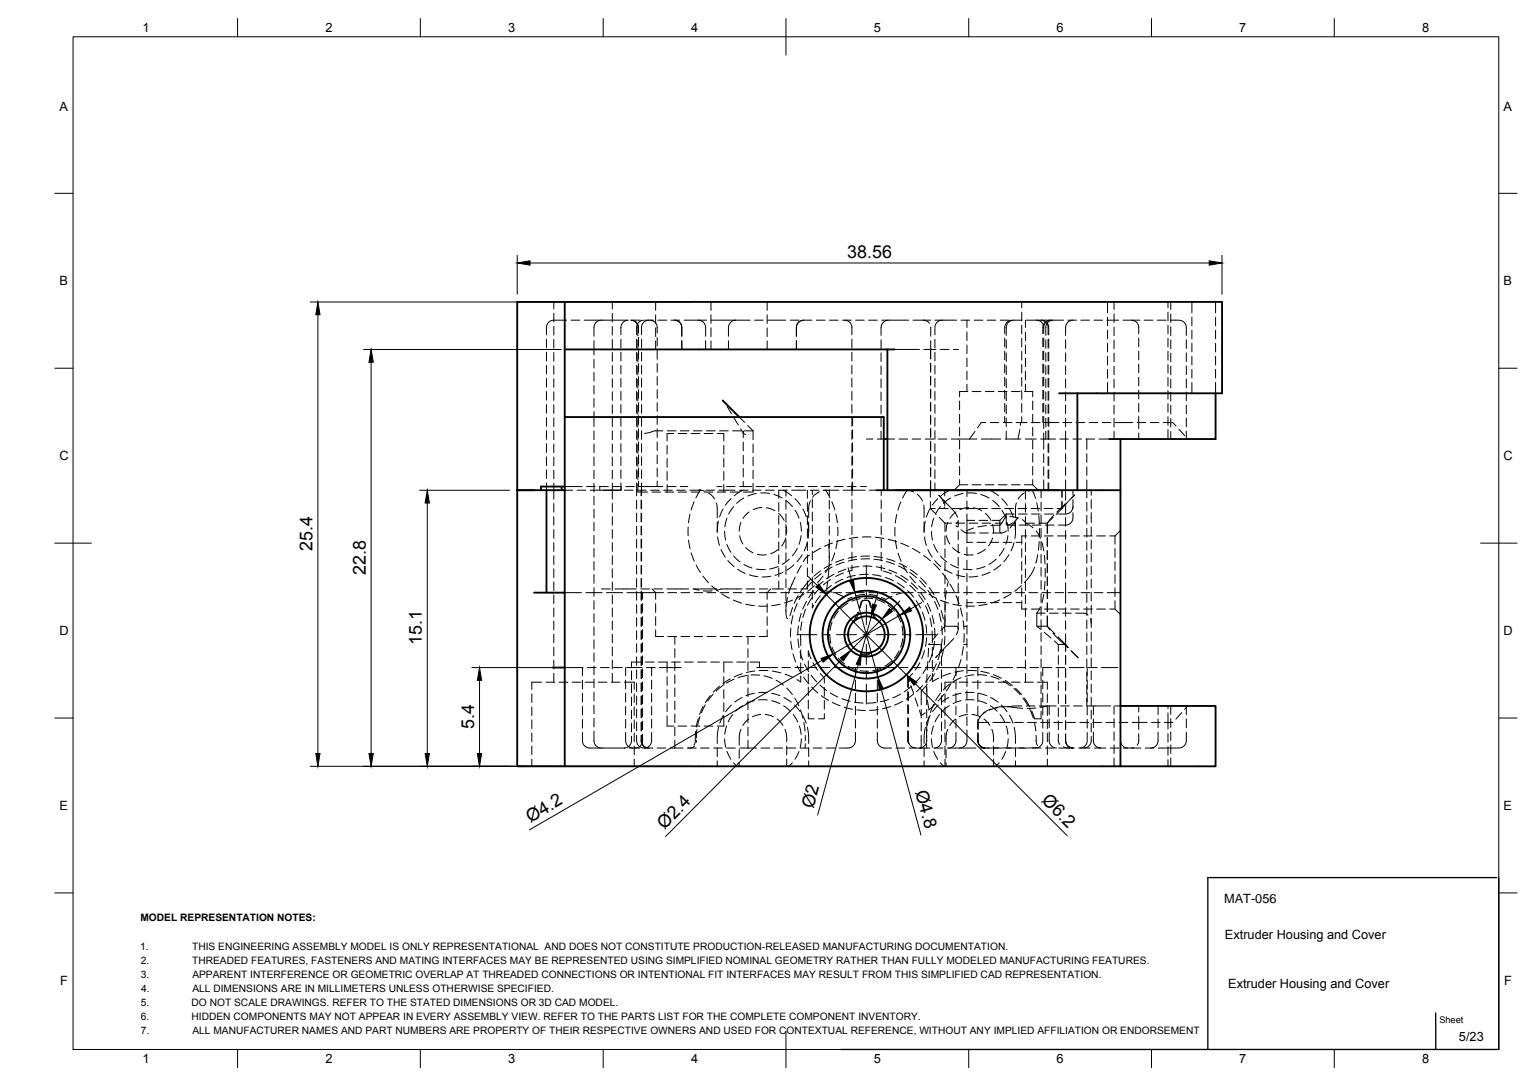
ISO-10303-21;
HEADER;
/* Generated by software containing ST-Developer
 * from STEP Tools, Inc. (www.steptools.com) 
 */

FILE_DESCRIPTION(
/* description */ (''),
/* implementation_level */ '2;1');

FILE_NAME(
/* name */ 'Extruder Housing and Cover.step',
/* time_stamp */ '2026-10-28T16:47:13+01:00',
/* author */ (''),
/* organization */ (''),
/* preprocessor_version */ 'ST-DEVELOPER v20.2',
/* originating_system */ 'Autodesk Translation Framework v15.17.0.0',
/* authorisation */ '');

FILE_SCHEMA (('AUTOMOTIVE_DESIGN { 1 0 10303 214 3 1 1 }'));
ENDSEC;

DATA;
#10=MECHANICAL_DESIGN_GEOMETRIC_PRESENTATION_REPRESENTATION('',(#4569,#4570),#459242);
#135=SPHERICAL_SURFACE('',#96252,3.7);
#136=SPHERICAL_SURFACE('',#96289,0.4);
#137=SPHERICAL_SURFACE('',#96515,3.7);
#138=SPHERICAL_SURFACE('',#96673,2.5);
#139=SPHERICAL_SURFACE('',#96678,2.5);
#140=SPHERICAL_SURFACE('',#96891,0.4);
#141=SPHERICAL_SURFACE('',#96896,0.4);
#156=ELLIPSE('',#96160,1.23559647500717,0.4);
#157=ELLIPSE('',#96173,0.405496303869506,0.4);
#158=ELLIPSE('',#96175,0.680073525436772,0.4);
#159=ELLIPSE('',#96193,0.565685424949236,0.4);
#160=ELLIPSE('',#96250,11.2311262166053,9.2);
#161=ELLIPSE('',#96391,11.2311262166054,9.2);
#162=ELLIPSE('',#96412,0.565685424948761,0.4);
#163=ELLIPSE('',#96519,10.6232449530892,9.2);
#164=ELLIPSE('',#96520,11.2311262166053,9.2);
#165=ELLIPSE('',#96521,11.2311262166053,9.2);
#166=ELLIPSE('',#96562,11.2311262166054,9.2);
#167=ELLIPSE('',#96563,10.6232449530892,9.2);
#168=ELLIPSE('',#96876,12.4909175466738,7.94395207421036);
#169=ELLIPSE('',#97006,2.10877579943506,1.);
#170=ELLIPSE('',#97007,2.46373699895096,1.);
#171=ELLIPSE('',#97009,2.59999999999994,1.3);
#172=ELLIPSE('',#97010,0.230940107675852,0.2);
#173=ELLIPSE('',#97011,0.230940107675852,0.2);
#174=ELLIPSE('',#97015,2.26648083430746,1.3);
#175=ELLIPSE('',#97016,0.24415491775229,0.2);
#176=ELLIPSE('',#97017,0.24415491775229,0.2);
#177=ELLIPSE('',#97027,0.24415491775229,0.2);
#178=ELLIPSE('',#97030,0.24415491775229,0.2);
#179=ELLIPSE('',#97033,0.230940107675851,0.2);
#180=ELLIPSE('',#97035,0.230940107675851,0.2);
#181=ELLIPSE('',#97037,2.59999999999997,1.3);
#182=ELLIPSE('',#97038,2.46373699895092,1.);
#183=ELLIPSE('',#97040,2.10877579943508,1.);
#184=ELLIPSE('',#97042,2.26648083430744,1.3);
#1619=ORIENTED_CLOSED_SHELL('',*,#94627,.F.);
#1620=BREP_WITH_VOIDS('Cover',#94628,(#1619));
#1621=TOROIDAL_SURFACE('',#95348,5.05,0.4);
#1622=TOROIDAL_SURFACE('',#95355,10.4999999997296,0.4);
#1623=TOROIDAL_SURFACE('',#95362,11.6,0.4);
#1624=TOROIDAL_SURFACE('',#95390,3.6,0.4);
#1625=TOROIDAL_SURFACE('',#95404,1.2,0.4);
#1626=TOROIDAL_SURFACE('',#95413,13.6,0.4);
#1627=TOROIDAL_SURFACE('',#95420,3.55,0.4);
#1628=TOROIDAL_SURFACE('',#95445,10.1000000149012,0.4);
#1629=TOROIDAL_SURFACE('',#95463,3.6,0.4);
#1630=TOROIDAL_SURFACE('',#95475,3.55,0.4);
#1631=TOROIDAL_SURFACE('',#95497,10.1000000149012,0.4);
#1632=TOROIDAL_SURFACE('',#95504,4.1,0.4);
#1633=TOROIDAL_SURFACE('',#95508,3.2,0.4);
#1634=TOROIDAL_SURFACE('',#95514,5.80000000000001,0.4);
#1635=TOROIDAL_SURFACE('',#95535,5.2,0.4);
#1636=TOROIDAL_SURFACE('',#95543,5.8,0.4);
#1637=TOROIDAL_SURFACE('',#95547,7.59496173936711,0.4);
#1638=TOROIDAL_SURFACE('',#95556,1.2,0.4);
#1639=TOROIDAL_SURFACE('',#95570,3.5,0.4);
#1640=TOROIDAL_SURFACE('',#95591,9.7949617393671,0.4);
#1641=TOROIDAL_SURFACE('',#95596,3.6,0.4);
#1642=TOROIDAL_SURFACE('',#95603,10.1,0.4);
#1643=TOROIDAL_SURFACE('',#95610,16.9949617393671,0.4);
#1644=TOROIDAL_SURFACE('',#95631,4.,0.4);
#1645=TOROIDAL_SURFACE('',#95639,23.3449617393671,0.4);
#1646=TOROIDAL_SURFACE('',#95643,0.8,0.4);
#1647=TOROIDAL_SURFACE('',#95647,8.2,0.4);
#1648=TOROIDAL_SURFACE('',#95669,19.3949617393671,0.4);
#1649=TOROIDAL_SURFACE('',#95676,10.1,0.4);
#1650=TOROIDAL_SURFACE('',#95699,5.05,0.4);
#1651=TOROIDAL_SURFACE('',#95707,13.,0.4);
#1652=TOROIDAL_SURFACE('',#95716,11.6,0.4);
#1653=TOROIDAL_SURFACE('',#95723,10.4999999997296,0.4);
#1654=TOROIDAL_SURFACE('',#95753,4.,0.4);
#1655=TOROIDAL_SURFACE('',#95760,13.6,0.4);
#1656=TOROIDAL_SURFACE('',#96072,5.05,0.4);
#1657=TOROIDAL_SURFACE('',#96090,11.,0.4);
#1658=TOROIDAL_SURFACE('',#96106,3.6,0.4);
#1659=TOROIDAL_SURFACE('',#96110,2.1,0.4);
#1660=TOROIDAL_SURFACE('',#96116,2.1,0.4);
#1661=TOROIDAL_SURFACE('',#96119,16.9949617393671,0.4);
#1662=TOROIDAL_SURFACE('',#96123,3.6,0.4);
#1663=TOROIDAL_SURFACE('',#96126,9.79496173936711,0.4);
#1664=TOROIDAL_SURFACE('',#96138,11.95,0.4);
#1665=TOROIDAL_SURFACE('',#96145,4.2,0.4);
#1666=TOROIDAL_SURFACE('',#96178,4.2,0.4);
#1667=TOROIDAL_SURFACE('',#96185,25.3449617393673,0.4);
#1668=TOROIDAL_SURFACE('',#96201,4.09750037145961,0.4);
#1669=TOROIDAL_SURFACE('',#96206,3.2,0.4);
#1670=TOROIDAL_SURFACE('',#96209,4.1,0.4);
#1671=TOROIDAL_SURFACE('',#96230,8.8,0.4);
#1672=TOROIDAL_SURFACE('',#96253,4.6,0.4);
#1673=TOROIDAL_SURFACE('',#96263,1.2,0.4);
#1674=TOROIDAL_SURFACE('',#96272,6.1,0.4);
#1675=TOROIDAL_SURFACE('',#96280,5.2,0.4);
#1676=TOROIDAL_SURFACE('',#96286,7.2949617393671,0.4);
#1677=TOROIDAL_SURFACE('',#96310,4.5,0.4);
#1678=TOROIDAL_SURFACE('',#96319,8.2,0.4);
#1679=TOROIDAL_SURFACE('',#96326,19.4949617393671,0.4);
#1680=TOROIDAL_SURFACE('',#96361,4.1,0.4);
#1681=TOROIDAL_SURFACE('',#96365,6.2,0.4);
#1682=TOROIDAL_SURFACE('',#96372,22.1949617393671,0.4);
#1683=TOROIDAL_SURFACE('',#96376,8.8,0.4);
#1684=TOROIDAL_SURFACE('',#96397,12.05,0.4);
#1685=TOROIDAL_SURFACE('',#96404,3.6,0.4);
#1686=TOROIDAL_SURFACE('',#96429,1.2,0.4);
#1687=TOROIDAL_SURFACE('',#96438,8.8,0.4);
#1688=TOROIDAL_SURFACE('',#96450,3.9,0.4);
#1689=TOROIDAL_SURFACE('',#96478,8.8,0.4);
#1690=TOROIDAL_SURFACE('',#96495,3.9,0.4);
#1691=TOROIDAL_SURFACE('',#96506,8.8,0.4);
#1692=TOROIDAL_SURFACE('',#96509,4.0975003714596,0.4);
#1693=TOROIDAL_SURFACE('',#96525,8.8,0.4);
#1694=TOROIDAL_SURFACE('',#96538,3.9,0.4);
#1695=TOROIDAL_SURFACE('',#96884,3.6,0.4);
#1696=TOROIDAL_SURFACE('',#96902,3.6,0.4);
#1697=TOROIDAL_SURFACE('',#96914,4.64877154610377,0.4);
#2221=(
BOUNDED_SURFACE()
B_SPLINE_SURFACE(2,2,((#138725,#138726,#138727,#138728,#138729),(#138730,
#138731,#138732,#138733,#138734),(#138735,#138736,#138737,#138738,#138739)),
 .UNSPECIFIED.,.F.,.F.,.F.)
B_SPLINE_SURFACE_WITH_KNOTS((3,3),(3,2,3),(-1.08356648062379E-15,1.5707963267949),
(-0.78539816339629,0.381098988689,1.54759614077429),.UNSPECIFIED.)
GEOMETRIC_REPRESENTATION_ITEM()
RATIONAL_B_SPLINE_SURFACE(((1.,0.834677941920344,1.,0.834677941920344,1.),
(0.707106781186542,0.590206432838701,0.707106781186542,0.590206432838701,
0.707106781186542),(1.,0.834677941920344,1.,0.834677941920344,1.)))
REPRESENTATION_ITEM('')
SURFACE()
);
#2222=(
BOUNDED_SURFACE()
B_SPLINE_SURFACE(2,2,((#138751,#138752,#138753,#138754,#138755),(#138756,
#138757,#138758,#138759,#138760),(#138761,#138762,#138763,#138764,#138765)),
 .UNSPECIFIED.,.F.,.F.,.F.)
B_SPLINE_SURFACE_WITH_KNOTS((3,3),(3,2,3),(-2.56377862909096E-16,1.5707963267949),
(0.206471222704293,1.13583112104019,2.06519101937609),.UNSPECIFIED.)
GEOMETRIC_REPRESENTATION_ITEM()
RATIONAL_B_SPLINE_SURFACE(((1.,0.89396503791678,1.,0.89396503791678,1.),
(0.707106781186548,0.632128740454645,0.707106781186548,0.632128740454645,
0.707106781186548),(1.,0.89396503791678,1.,0.89396503791678,1.)))
REPRESENTATION_ITEM('')
SURFACE()
);
#2223=(
BOUNDED_SURFACE()
B_SPLINE_SURFACE(2,2,((#138777,#138778,#138779,#138780,#138781),(#138782,
#138783,#138784,#138785,#138786),(#138787,#138788,#138789,#138790,#138791)),
 .UNSPECIFIED.,.F.,.F.,.F.)
B_SPLINE_SURFACE_WITH_KNOTS((3,3),(3,2,3),(-4.13193059734374E-15,1.5707963267949),
(-0.913769759667264,1.11022302462516E-16,0.913769759667264),
 .UNSPECIFIED.)
GEOMETRIC_REPRESENTATION_ITEM()
RATIONAL_B_SPLINE_SURFACE(((1.,0.89743109935827,1.,0.89743109935827,1.),
(0.707106781186553,0.634579616003937,0.707106781186553,0.634579616003937,
0.707106781186553),(1.,0.89743109935827,1.,0.89743109935827,1.)))
REPRESENTATION_ITEM('')
SURFACE()
);
#2224=(
BOUNDED_SURFACE()
B_SPLINE_SURFACE(2,2,((#138803,#138804,#138805),(#138806,#138807,#138808),
(#138809,#138810,#138811)),.UNSPECIFIED.,.F.,.F.,.F.)
B_SPLINE_SURFACE_WITH_KNOTS((3,3),(3,3),(-3.94009957434615E-16,1.5707963267949),
(-2.61567274150278,-1.57079632679301),.UNSPECIFIED.)
GEOMETRIC_REPRESENTATION_ITEM()
RATIONAL_B_SPLINE_SURFACE(((1.,0.866605104543064,1.),(0.707106781186545,
0.612782346033276,0.707106781186545),(1.,0.866605104543064,1.)))
REPRESENTATION_ITEM('')
SURFACE()
);
#2225=(
BOUNDED_SURFACE()
B_SPLINE_SURFACE(2,2,((#138823,#138824,#138825),(#138826,#138827,#138828),
(#138829,#138830,#138831)),.UNSPECIFIED.,.F.,.F.,.F.)
B_SPLINE_SURFACE_WITH_KNOTS((3,3),(3,3),(-1.43399263023479E-17,1.5707963267949),
(-1.57079632679302,-0.785398163396283),.UNSPECIFIED.)
GEOMETRIC_REPRESENTATION_ITEM()
RATIONAL_B_SPLINE_SURFACE(((1.,0.923879532511424,1.),(0.707106781186537,
0.653281482438276,0.707106781186537),(1.,0.923879532511424,1.)))
REPRESENTATION_ITEM('')
SURFACE()
);
#2226=(
BOUNDED_SURFACE()
B_SPLINE_SURFACE(2,2,((#138884,#138885,#138886),(#138887,#138888,#138889),
(#138890,#138891,#138892)),.UNSPECIFIED.,.F.,.F.,.F.)
B_SPLINE_SURFACE_WITH_KNOTS((3,3),(3,3),(-2.92306873924357E-15,1.5707963267949),
(-0.624753868765047,0.624753868765048),.UNSPECIFIED.)
GEOMETRIC_REPRESENTATION_ITEM()
RATIONAL_B_SPLINE_SURFACE(((1.,0.81110710565381,1.),(0.707106781186553,
0.573539334676407,0.707106781186553),(1.,0.81110710565381,1.)))
REPRESENTATION_ITEM('')
SURFACE()
);
#2227=(
BOUNDED_SURFACE()
B_SPLINE_SURFACE(2,2,((#138904,#138905,#138906,#138907,#138908),(#138909,
#138910,#138911,#138912,#138913),(#138914,#138915,#138916,#138917,#138918)),
 .UNSPECIFIED.,.F.,.F.,.F.)
B_SPLINE_SURFACE_WITH_KNOTS((3,3),(3,2,3),(-4.23634106201263E-16,1.5707963267949),
(-0.93774449040515,0.,0.93774449040515),.UNSPECIFIED.)
GEOMETRIC_REPRESENTATION_ITEM()
RATIONAL_B_SPLINE_SURFACE(((1.,0.892078465806108,1.,0.892078465806108,1.),
(0.707106781186543,0.630794732521986,0.707106781186543,0.630794732521986,
0.707106781186543),(1.,0.892078465806108,1.,0.892078465806108,1.)))
REPRESENTATION_ITEM('')
SURFACE()
);
#2228=(
BOUNDED_SURFACE()
B_SPLINE_SURFACE(2,2,((#138930,#138931,#138932),(#138933,#138934,#138935),
(#138936,#138937,#138938)),.UNSPECIFIED.,.F.,.F.,.F.)
B_SPLINE_SURFACE_WITH_KNOTS((3,3),(3,3),(-1.38777878078474E-15,1.5707963267949),
(-1.57079632680232,-0.78539816339745),.UNSPECIFIED.)
GEOMETRIC_REPRESENTATION_ITEM()
RATIONAL_B_SPLINE_SURFACE(((1.,0.923879532509866,1.),(0.707106781186554,
0.653281482437189,0.707106781186554),(1.,0.923879532509866,1.)))
REPRESENTATION_ITEM('')
SURFACE()
);
#2229=(
BOUNDED_SURFACE()
B_SPLINE_SURFACE(2,2,((#138962,#138963,#138964,#138965,#138966),(#138967,
#138968,#138969,#138970,#138971),(#138972,#138973,#138974,#138975,#138976)),
 .UNSPECIFIED.,.F.,.F.,.F.)
B_SPLINE_SURFACE_WITH_KNOTS((3,3),(3,2,3),(-3.22429839320269E-16,1.57079632679491),
(-1.57079632679301,-0.578762685695985,0.413270955399318),.UNSPECIFIED.)
GEOMETRIC_REPRESENTATION_ITEM()
RATIONAL_B_SPLINE_SURFACE(((1.,0.87948523306508,1.,0.87948523306508,1.),
(0.707106781186541,0.621889972253744,0.707106781186541,0.621889972253744,
0.707106781186541),(1.,0.87948523306508,1.,0.87948523306508,1.)))
REPRESENTATION_ITEM('')
SURFACE()
);
#2230=(
BOUNDED_SURFACE()
B_SPLINE_SURFACE(2,2,((#138988,#138989,#138990),(#138991,#138992,#138993),
(#138994,#138995,#138996)),.UNSPECIFIED.,.F.,.F.,.F.)
B_SPLINE_SURFACE_WITH_KNOTS((3,3),(3,3),(-4.80258936466661E-17,1.5707963267949),
(0.338566037798194,1.71521306218255),.UNSPECIFIED.)
GEOMETRIC_REPRESENTATION_ITEM()
RATIONAL_B_SPLINE_SURFACE(((1.,0.772312077486283,1.),(0.707106781186543,
0.546107107182817,0.707106781186543),(1.,0.772312077486283,1.)))
REPRESENTATION_ITEM('')
SURFACE()
);
#2231=(
BOUNDED_SURFACE()
B_SPLINE_SURFACE(2,2,((#139010,#139011,#139012),(#139013,#139014,#139015),
(#139016,#139017,#139018)),.UNSPECIFIED.,.F.,.F.,.F.)
B_SPLINE_SURFACE_WITH_KNOTS((3,3),(3,3),(-2.97223913180379E-15,1.5707963267949),
(0.821121559764502,2.02961305550291),.UNSPECIFIED.)
GEOMETRIC_REPRESENTATION_ITEM()
RATIONAL_B_SPLINE_SURFACE(((1.,0.82293085364046,1.),(0.707106781186547,
0.581899987056804,0.707106781186547),(1.,0.82293085364046,1.)))
REPRESENTATION_ITEM('')
SURFACE()
);
#2232=(
BOUNDED_SURFACE()
B_SPLINE_SURFACE(2,2,((#139080,#139081,#139082),(#139083,#139084,#139085),
(#139086,#139087,#139088)),.UNSPECIFIED.,.F.,.F.,.F.)
B_SPLINE_SURFACE_WITH_KNOTS((3,3),(3,3),(1.36100253158678E-19,1.57079632679491),
(0.135935745545801,1.57038769941725),.UNSPECIFIED.)
GEOMETRIC_REPRESENTATION_ITEM()
RATIONAL_B_SPLINE_SURFACE(((1.,0.753631982435871,1.),(0.707106781186546,
0.532898285299465,0.707106781186546),(1.,0.753631982435871,1.)))
REPRESENTATION_ITEM('')
SURFACE()
);
#2233=(
BOUNDED_SURFACE()
B_SPLINE_SURFACE(2,2,((#139100,#139101,#139102,#139103,#139104),(#139105,
#139106,#139107,#139108,#139109),(#139110,#139111,#139112,#139113,#139114)),
 .UNSPECIFIED.,.F.,.F.,.F.)
B_SPLINE_SURFACE_WITH_KNOTS((3,3),(3,2,3),(-3.39617731412459E-16,1.570796326795),
(1.57038769941725,2.35599017650376,3.14159265359003),.UNSPECIFIED.)
GEOMETRIC_REPRESENTATION_ITEM()
RATIONAL_B_SPLINE_SURFACE(((1.,0.92384043395866,1.,0.92384043395866,1.),
(0.707106781186508,0.653253835586454,0.707106781186508,0.653253835586454,
0.707106781186508),(1.,0.92384043395866,1.,0.92384043395866,1.)))
REPRESENTATION_ITEM('')
SURFACE()
);
#2234=(
BOUNDED_SURFACE()
B_SPLINE_SURFACE(2,2,((#139126,#139127,#139128,#139129,#139130),(#139131,
#139132,#139133,#139134,#139135),(#139136,#139137,#139138,#139139,#139140)),
 .UNSPECIFIED.,.F.,.F.,.F.)
B_SPLINE_SURFACE_WITH_KNOTS((3,3),(3,2,3),(-3.35182484084685E-16,1.5707963267949),
(-3.14159265359013,-2.16753947400706,-1.19348629442367),.UNSPECIFIED.)
GEOMETRIC_REPRESENTATION_ITEM()
RATIONAL_B_SPLINE_SURFACE(((1.,0.883728319944576,1.,0.883728319944576,1.),
(0.707106781186538,0.624890287759396,0.707106781186538,0.624890287759396,
0.707106781186538),(1.,0.883728319944576,1.,0.883728319944576,1.)))
REPRESENTATION_ITEM('')
SURFACE()
);
#2235=(
BOUNDED_SURFACE()
B_SPLINE_SURFACE(2,2,((#139152,#139153,#139154),(#139155,#139156,#139157),
(#139158,#139159,#139160)),.UNSPECIFIED.,.F.,.F.,.F.)
B_SPLINE_SURFACE_WITH_KNOTS((3,3),(3,3),(-2.40560064119055E-16,1.5707963267949),
(-2.36148733561698,-1.11197959808688),.UNSPECIFIED.)
GEOMETRIC_REPRESENTATION_ITEM()
RATIONAL_B_SPLINE_SURFACE(((1.,0.81110710565381,1.),(0.707106781186542,
0.573539334676398,0.707106781186542),(1.,0.81110710565381,1.)))
REPRESENTATION_ITEM('')
SURFACE()
);
#2236=(
BOUNDED_SURFACE()
B_SPLINE_SURFACE(2,2,((#139172,#139173,#139174),(#139175,#139176,#139177),
(#139178,#139179,#139180)),.UNSPECIFIED.,.F.,.F.,.F.)
B_SPLINE_SURFACE_WITH_KNOTS((3,3),(3,3),(-3.67871583187674E-16,1.5707963267949),
(-1.11197959808689,0.13308724141338),.UNSPECIFIED.)
GEOMETRIC_REPRESENTATION_ITEM()
RATIONAL_B_SPLINE_SURFACE(((1.,0.812403840463596,1.),(0.707106781186548,
0.574456264653803,0.707106781186548),(1.,0.812403840463596,1.)))
REPRESENTATION_ITEM('')
SURFACE()
);
#2237=(
BOUNDED_SURFACE()
B_SPLINE_SURFACE(2,2,((#139189,#139190,#139191),(#139192,#139193,#139194),
(#139195,#139196,#139197)),.UNSPECIFIED.,.F.,.F.,.F.)
B_SPLINE_SURFACE_WITH_KNOTS((3,3),(3,3),(-3.62332867476797E-16,1.5707963267949),
(-0.379047751698848,0.883627629924469),.UNSPECIFIED.)
GEOMETRIC_REPRESENTATION_ITEM()
RATIONAL_B_SPLINE_SURFACE(((1.,0.8072386920689,1.),(0.707106781186543,0.570803953198074,
0.707106781186543),(1.,0.8072386920689,1.)))
REPRESENTATION_ITEM('')
SURFACE()
);
#2238=(
BOUNDED_SURFACE()
B_SPLINE_SURFACE(2,2,((#139234,#139235,#139236),(#139237,#139238,#139239),
(#139240,#139241,#139242)),.UNSPECIFIED.,.F.,.F.,.F.)
B_SPLINE_SURFACE_WITH_KNOTS((3,3),(3,3),(-2.78610200478756E-15,1.5707963267949),
(-1.57120495417254,-0.136753000301094),.UNSPECIFIED.)
GEOMETRIC_REPRESENTATION_ITEM()
RATIONAL_B_SPLINE_SURFACE(((1.,0.753631982435872,1.),(0.707106781186546,
0.532898285299465,0.707106781186546),(1.,0.753631982435872,1.)))
REPRESENTATION_ITEM('')
SURFACE()
);
#2239=(
BOUNDED_SURFACE()
B_SPLINE_SURFACE(2,2,((#139254,#139255,#139256),(#139257,#139258,#139259),
(#139260,#139261,#139262)),.UNSPECIFIED.,.F.,.F.,.F.)
B_SPLINE_SURFACE_WITH_KNOTS((3,3),(3,3),(2.55184415889316E-16,1.5707963267949),
(-0.59217173005856,0.724821492103155),.UNSPECIFIED.)
GEOMETRIC_REPRESENTATION_ITEM()
RATIONAL_B_SPLINE_SURFACE(((1.,0.790913091470082,1.),(0.707106781186549,
0.559260010307712,0.707106781186549),(1.,0.790913091470082,1.)))
REPRESENTATION_ITEM('')
SURFACE()
);
#2240=(
BOUNDED_SURFACE()
B_SPLINE_SURFACE(2,2,((#139292,#139293,#139294,#139295,#139296),(#139297,
#139298,#139299,#139300,#139301),(#139302,#139303,#139304,#139305,#139306)),
 .UNSPECIFIED.,.F.,.F.,.F.)
B_SPLINE_SURFACE_WITH_KNOTS((3,3),(3,2,3),(-3.35271616303555E-16,1.57079632679502),
(1.26610367277728,2.20384816318377,3.14159265359003),.UNSPECIFIED.)
GEOMETRIC_REPRESENTATION_ITEM()
RATIONAL_B_SPLINE_SURFACE(((1.,0.892078465805831,1.,0.892078465805831,1.),
(0.707106781186508,0.630794732521759,0.707106781186508,0.630794732521759,
0.707106781186508),(1.,0.892078465805831,1.,0.892078465805831,1.)))
REPRESENTATION_ITEM('')
SURFACE()
);
#2241=(
BOUNDED_SURFACE()
B_SPLINE_SURFACE(2,2,((#139318,#139319,#139320),(#139321,#139322,#139323),
(#139324,#139325,#139326)),.UNSPECIFIED.,.F.,.F.,.F.)
B_SPLINE_SURFACE_WITH_KNOTS((3,3),(3,3),(-3.10863177296109E-15,1.5707963267949),
(-3.14159265359013,-1.57120495417254),.UNSPECIFIED.)
GEOMETRIC_REPRESENTATION_ITEM()
RATIONAL_B_SPLINE_SURFACE(((1.,0.707251238021515,1.),(0.707106781186534,
0.500102146407585,0.707106781186534),(1.,0.707251238021515,1.)))
REPRESENTATION_ITEM('')
SURFACE()
);
#2242=(
BOUNDED_SURFACE()
B_SPLINE_SURFACE(2,2,((#139373,#139374,#139375,#139376,#139377),(#139378,
#139379,#139380,#139381,#139382),(#139383,#139384,#139385,#139386,#139387)),
 .UNSPECIFIED.,.F.,.F.,.F.)
B_SPLINE_SURFACE_WITH_KNOTS((3,3),(3,2,3),(-3.79723113300163E-16,1.5707963267949),
(-2.21649908067713,-1.20577137048503,-0.195043660292926),.UNSPECIFIED.)
GEOMETRIC_REPRESENTATION_ITEM()
RATIONAL_B_SPLINE_SURFACE(((1.,0.874998380695011,1.,0.874998380695011,1.),
(0.707106781186542,0.618717288516686,0.707106781186542,0.618717288516686,
0.707106781186542),(1.,0.874998380695011,1.,0.874998380695011,1.)))
REPRESENTATION_ITEM('')
SURFACE()
);
#2243=(
BOUNDED_SURFACE()
B_SPLINE_SURFACE(2,2,((#139405,#139406,#139407,#139408,#139409),(#139410,
#139411,#139412,#139413,#139414),(#139415,#139416,#139417,#139418,#139419)),
 .UNSPECIFIED.,.F.,.F.,.F.)
B_SPLINE_SURFACE_WITH_KNOTS((3,3),(3,2,3),(-2.33769771306233E-15,1.5707963267949),
(-0.139437550001727,0.715679388398409,1.57079632679678),.UNSPECIFIED.)
GEOMETRIC_REPRESENTATION_ITEM()
RATIONAL_B_SPLINE_SURFACE(((1.,0.909980842363504,1.,0.909980842363504,1.),
(0.707106781186545,0.643453624385078,0.707106781186545,0.643453624385078,
0.707106781186545),(1.,0.909980842363504,1.,0.909980842363504,1.)))
REPRESENTATION_ITEM('')
SURFACE()
);
#2244=(
BOUNDED_SURFACE()
B_SPLINE_SURFACE(2,2,((#139443,#139444,#139445),(#139446,#139447,#139448),
(#139449,#139450,#139451)),.UNSPECIFIED.,.F.,.F.,.F.)
B_SPLINE_SURFACE_WITH_KNOTS((3,3),(3,3),(1.38777878078144E-17,1.5707963267949),
(0.785398163397444,1.5707963267949),.UNSPECIFIED.)
GEOMETRIC_REPRESENTATION_ITEM()
RATIONAL_B_SPLINE_SURFACE(((1.,0.923879532511286,1.),(0.707106781186537,
0.653281482438178,0.707106781186537),(1.,0.923879532511286,1.)))
REPRESENTATION_ITEM('')
SURFACE()
);
#2245=(
BOUNDED_SURFACE()
B_SPLINE_SURFACE(2,2,((#139463,#139464,#139465,#139466,#139467),(#139468,
#139469,#139470,#139471,#139472),(#139473,#139474,#139475,#139476,#139477)),
 .UNSPECIFIED.,.F.,.F.,.F.)
B_SPLINE_SURFACE_WITH_KNOTS((3,3),(3,2,3),(-2.76514922070703E-15,1.5707963267949),
(-1.03943004137575,0.,1.03943004137575),.UNSPECIFIED.)
GEOMETRIC_REPRESENTATION_ITEM()
RATIONAL_B_SPLINE_SURFACE(((1.,0.867960744996435,1.,0.867960744996435,1.),
(0.707106781186546,0.613740928590705,0.707106781186546,0.613740928590705,
0.707106781186546),(1.,0.867960744996435,1.,0.867960744996435,1.)))
REPRESENTATION_ITEM('')
SURFACE()
);
#2246=(
BOUNDED_SURFACE()
B_SPLINE_SURFACE(2,2,((#139489,#139490,#139491,#139492,#139493),(#139494,
#139495,#139496,#139497,#139498),(#139499,#139500,#139501,#139502,#139503)),
 .UNSPECIFIED.,.F.,.F.,.F.)
B_SPLINE_SURFACE_WITH_KNOTS((3,3),(3,2,3),(-4.15746516061636E-16,1.5707963267949),
(-1.31482537730283,-2.22044604925031E-16,1.31482537730283),
 .UNSPECIFIED.)
GEOMETRIC_REPRESENTATION_ITEM()
RATIONAL_B_SPLINE_SURFACE(((1.,0.791575909743,1.,0.791575909743,1.),(0.707106781186554,
0.559728693603191,0.707106781186554,0.559728693603191,0.707106781186554),
(1.,0.791575909743,1.,0.791575909743,1.)))
REPRESENTATION_ITEM('')
SURFACE()
);
#2247=(
BOUNDED_SURFACE()
B_SPLINE_SURFACE(2,2,((#139558,#139559,#139560,#139561,#139562),(#139563,
#139564,#139565,#139566,#139567),(#139568,#139569,#139570,#139571,#139572)),
 .UNSPECIFIED.,.F.,.F.,.F.)
B_SPLINE_SURFACE_WITH_KNOTS((3,3),(3,2,3),(-2.46171489419642E-16,1.5707963267949),
(-2.81803077212777,-1.86696066691245,-0.915890561697128),.UNSPECIFIED.)
GEOMETRIC_REPRESENTATION_ITEM()
RATIONAL_B_SPLINE_SURFACE(((1.,0.889047894212165,1.,0.889047894212165,1.),
(0.707106781186546,0.628651794797041,0.707106781186546,0.628651794797041,
0.707106781186546),(1.,0.889047894212165,1.,0.889047894212165,1.)))
REPRESENTATION_ITEM('')
SURFACE()
);
#2248=(
BOUNDED_SURFACE()
B_SPLINE_SURFACE(2,2,((#139584,#139585,#139586),(#139587,#139588,#139589),
(#139590,#139591,#139592)),.UNSPECIFIED.,.F.,.F.,.F.)
B_SPLINE_SURFACE_WITH_KNOTS((3,3),(3,3),(-4.20649046086306E-17,1.5707963267949),
(-1.66612611099672,-0.292748166464849),.UNSPECIFIED.)
GEOMETRIC_REPRESENTATION_ITEM()
RATIONAL_B_SPLINE_SURFACE(((1.,0.773349375865919,1.),(0.707106781186547,
0.546840587901175,0.707106781186547),(1.,0.773349375865919,1.)))
REPRESENTATION_ITEM('')
SURFACE()
);
#2249=(
BOUNDED_SURFACE()
B_SPLINE_SURFACE(2,2,((#139604,#139605,#139606,#139607,#139608),(#139609,
#139610,#139611,#139612,#139613),(#139614,#139615,#139616,#139617,#139618)),
 .UNSPECIFIED.,.F.,.F.,.F.)
B_SPLINE_SURFACE_WITH_KNOTS((3,3),(3,2,3),(-2.33310191252187E-15,1.5707963267949),
(-0.0602957815162571,0.75525027264115,1.57079632679678),.UNSPECIFIED.)
GEOMETRIC_REPRESENTATION_ITEM()
RATIONAL_B_SPLINE_SURFACE(((1.,0.918006240075228,1.,0.918006240075228,1.),
(0.707106781186546,0.649128437528759,0.707106781186546,0.649128437528759,
0.707106781186546),(1.,0.918006240075228,1.,0.918006240075228,1.)))
REPRESENTATION_ITEM('')
SURFACE()
);
#2250=(
BOUNDED_SURFACE()
B_SPLINE_SURFACE(2,2,((#139630,#139631,#139632),(#139633,#139634,#139635),
(#139636,#139637,#139638)),.UNSPECIFIED.,.F.,.F.,.F.)
B_SPLINE_SURFACE_WITH_KNOTS((3,3),(3,3),(-4.40596164996656E-16,1.5707963267949),
(1.57079632679678,3.04334701619792),.UNSPECIFIED.)
GEOMETRIC_REPRESENTATION_ITEM()
RATIONAL_B_SPLINE_SURFACE(((1.,0.740974920563651,1.),(0.707106781186542,
0.523948391019717,0.707106781186542),(1.,0.740974920563651,1.)))
REPRESENTATION_ITEM('')
SURFACE()
);
#2251=(
BOUNDED_SURFACE()
B_SPLINE_SURFACE(2,2,((#139673,#139674,#139675),(#139676,#139677,#139678),
(#139679,#139680,#139681)),.UNSPECIFIED.,.F.,.F.,.F.)
B_SPLINE_SURFACE_WITH_KNOTS((3,3),(3,3),(-3.19704967403774E-16,1.5707963267949),
(-0.873151522554683,-0.203094574416464),.UNSPECIFIED.)
GEOMETRIC_REPRESENTATION_ITEM()
RATIONAL_B_SPLINE_SURFACE(((1.,0.944400947853729,1.),(0.707106781186549,
0.667792314386376,0.707106781186549),(1.,0.944400947853729,1.)))
REPRESENTATION_ITEM('')
SURFACE()
);
#2252=(
BOUNDED_SURFACE()
B_SPLINE_SURFACE(2,2,((#139705,#139706,#139707),(#139708,#139709,#139710),
(#139711,#139712,#139713)),.UNSPECIFIED.,.F.,.F.,.F.)
B_SPLINE_SURFACE_WITH_KNOTS((3,3),(3,3),(-5.55723799297029E-15,1.5707963267949),
(-1.5533380622009,-0.0271380096021075),.UNSPECIFIED.)
GEOMETRIC_REPRESENTATION_ITEM()
RATIONAL_B_SPLINE_SURFACE(((1.,0.722696856670203,1.),(0.707106781186542,
0.511023848093699,0.707106781186542),(1.,0.722696856670203,1.)))
REPRESENTATION_ITEM('')
SURFACE()
);
#2253=(
BOUNDED_SURFACE()
B_SPLINE_SURFACE(2,2,((#139725,#139726,#139727,#139728,#139729),(#139730,
#139731,#139732,#139733,#139734),(#139735,#139736,#139737,#139738,#139739)),
 .UNSPECIFIED.,.F.,.F.,.F.)
B_SPLINE_SURFACE_WITH_KNOTS((3,3),(3,2,3),(1.04083408558608E-17,1.5707963267949),
(-0.027138009602113,0.771829158596392,1.5707963267949),.UNSPECIFIED.)
GEOMETRIC_REPRESENTATION_ITEM()
RATIONAL_B_SPLINE_SURFACE(((1.,0.921261973001208,1.,0.921261973001208,1.),
(0.707106781186546,0.651430588358451,0.707106781186546,0.651430588358451,
0.707106781186546),(1.,0.921261973001208,1.,0.921261973001208,1.)))
REPRESENTATION_ITEM('')
SURFACE()
);
#2254=(
BOUNDED_SURFACE()
B_SPLINE_SURFACE(2,2,((#139751,#139752,#139753),(#139754,#139755,#139756),
(#139757,#139758,#139759)),.UNSPECIFIED.,.F.,.F.,.F.)
B_SPLINE_SURFACE_WITH_KNOTS((3,3),(3,3),(-3.04212300157278E-16,1.5707963267949),
(1.5707963267949,2.35619449019235),.UNSPECIFIED.)
GEOMETRIC_REPRESENTATION_ITEM()
RATIONAL_B_SPLINE_SURFACE(((1.,0.923879532511286,1.),(0.707106781186548,
0.653281482438189,0.707106781186548),(1.,0.923879532511286,1.)))
REPRESENTATION_ITEM('')
SURFACE()
);
#2255=(
BOUNDED_SURFACE()
B_SPLINE_SURFACE(2,2,((#139771,#139772,#139773),(#139774,#139775,#139776),
(#139777,#139778,#139779)),.UNSPECIFIED.,.F.,.F.,.F.)
B_SPLINE_SURFACE_WITH_KNOTS((3,3),(3,3),(-4.44307714369147E-16,1.5707963267949),
(-0.411322268457341,0.411322268457339),.UNSPECIFIED.)
GEOMETRIC_REPRESENTATION_ITEM()
RATIONAL_B_SPLINE_SURFACE(((1.,0.9165929526849,1.),(0.707106781186543,0.648129092431289,
0.707106781186543),(1.,0.9165929526849,1.)))
REPRESENTATION_ITEM('')
SURFACE()
);
#2256=(
BOUNDED_SURFACE()
B_SPLINE_SURFACE(2,2,((#139791,#139792,#139793),(#139794,#139795,#139796),
(#139797,#139798,#139799)),.UNSPECIFIED.,.F.,.F.,.F.)
B_SPLINE_SURFACE_WITH_KNOTS((3,3),(3,3),(-3.09236869201824E-15,1.57079632679491),
(-0.743192726042517,0.743192726042517),.UNSPECIFIED.)
GEOMETRIC_REPRESENTATION_ITEM()
RATIONAL_B_SPLINE_SURFACE(((1.,0.736311982025157,1.),(0.707106781186541,
0.520651195558891,0.707106781186541),(1.,0.736311982025157,1.)))
REPRESENTATION_ITEM('')
SURFACE()
);
#2257=(
BOUNDED_SURFACE()
B_SPLINE_SURFACE(2,2,((#139811,#139812,#139813,#139814,#139815),(#139816,
#139817,#139818,#139819,#139820),(#139821,#139822,#139823,#139824,#139825)),
 .UNSPECIFIED.,.F.,.F.,.F.)
B_SPLINE_SURFACE_WITH_KNOTS((3,3),(3,2,3),(-3.88201214029742E-16,1.5707963267949),
(-2.21206449869477,-1.24517592036125,-0.278287342027729),.UNSPECIFIED.)
GEOMETRIC_REPRESENTATION_ITEM()
RATIONAL_B_SPLINE_SURFACE(((1.,0.885399163650358,1.,0.885399163650358,1.),
(0.70710678118654,0.626071752674059,0.70710678118654,0.626071752674059,
0.70710678118654),(1.,0.885399163650358,1.,0.885399163650358,1.)))
REPRESENTATION_ITEM('')
SURFACE()
);
#2258=(
BOUNDED_SURFACE()
B_SPLINE_SURFACE(2,2,((#139876,#139877,#139878,#139879,#139880),(#139881,
#139882,#139883,#139884,#139885),(#139886,#139887,#139888,#139889,#139890)),
 .UNSPECIFIED.,.F.,.F.,.F.)
B_SPLINE_SURFACE_WITH_KNOTS((3,3),(3,2,3),(-3.2009740160607E-15,1.5707963267949),
(-2.81763962832209,-1.47992684575006,-0.142214063178028),.UNSPECIFIED.)
GEOMETRIC_REPRESENTATION_ITEM()
RATIONAL_B_SPLINE_SURFACE(((1.,0.784531318155132,1.,0.784531318155132,1.),
(0.707106781186547,0.554747415120714,0.707106781186547,0.554747415120714,
0.707106781186547),(1.,0.784531318155132,1.,0.784531318155132,1.)))
REPRESENTATION_ITEM('')
SURFACE()
);
#2259=(
BOUNDED_SURFACE()
B_SPLINE_SURFACE(2,2,((#139908,#139909,#139910),(#139911,#139912,#139913),
(#139914,#139915,#139916)),.UNSPECIFIED.,.F.,.F.,.F.)
B_SPLINE_SURFACE_WITH_KNOTS((3,3),(3,3),(-9.43679832250494E-16,1.5707963267949),
(-4.54149544011533E-19,1.07849707504375),.UNSPECIFIED.)
GEOMETRIC_REPRESENTATION_ITEM()
RATIONAL_B_SPLINE_SURFACE(((1.,0.858094793061586,1.),(0.707106781186537,
0.606764647074706,0.707106781186537),(1.,0.858094793061586,1.)))
REPRESENTATION_ITEM('')
SURFACE()
);
#2260=(
BOUNDED_SURFACE()
B_SPLINE_SURFACE(2,2,((#139928,#139929,#139930,#139931,#139932),(#139933,
#139934,#139935,#139936,#139937),(#139938,#139939,#139940,#139941,#139942)),
 .UNSPECIFIED.,.F.,.F.,.F.)
B_SPLINE_SURFACE_WITH_KNOTS((3,3),(3,2,3),(-1.37198715633005E-15,1.5707963267949),
(-0.913769759667265,0.,0.913769759667266),.UNSPECIFIED.)
GEOMETRIC_REPRESENTATION_ITEM()
RATIONAL_B_SPLINE_SURFACE(((1.,0.89743109935827,1.,0.89743109935827,1.),
(0.707106781186543,0.634579616003927,0.707106781186543,0.634579616003927,
0.707106781186543),(1.,0.89743109935827,1.,0.89743109935827,1.)))
REPRESENTATION_ITEM('')
SURFACE()
);
#2261=(
BOUNDED_SURFACE()
B_SPLINE_SURFACE(2,2,((#139954,#139955,#139956,#139957,#139958),(#139959,
#139960,#139961,#139962,#139963),(#139964,#139965,#139966,#139967,#139968)),
 .UNSPECIFIED.,.F.,.F.,.F.)
B_SPLINE_SURFACE_WITH_KNOTS((3,3),(3,2,3),(-5.97388390143348E-15,1.5707963267949),
(-0.929359898335899,0.,0.929359898335898),.UNSPECIFIED.)
GEOMETRIC_REPRESENTATION_ITEM()
RATIONAL_B_SPLINE_SURFACE(((1.,0.89396503791678,1.,0.89396503791678,1.),
(0.707106781186544,0.632128740454641,0.707106781186544,0.632128740454641,
0.707106781186544),(1.,0.89396503791678,1.,0.89396503791678,1.)))
REPRESENTATION_ITEM('')
SURFACE()
);
#2262=(
BOUNDED_SURFACE()
B_SPLINE_SURFACE(2,2,((#140011,#140012,#140013),(#140014,#140015,#140016),
(#140017,#140018,#140019)),.UNSPECIFIED.,.F.,.F.,.F.)
B_SPLINE_SURFACE_WITH_KNOTS((3,3),(3,3),(-2.44248335016468E-15,1.5707963267949),
(-1.38777878078145E-17,1.5707963267949),.UNSPECIFIED.)
GEOMETRIC_REPRESENTATION_ITEM()
RATIONAL_B_SPLINE_SURFACE(((1.,0.707106781186547,1.),(0.707106781186554,
0.500000000000004,0.707106781186554),(1.,0.707106781186547,1.)))
REPRESENTATION_ITEM('')
SURFACE()
);
#2263=(
BOUNDED_SURFACE()
B_SPLINE_SURFACE(2,2,((#140031,#140032,#140033,#140034,#140035),(#140036,
#140037,#140038,#140039,#140040),(#140041,#140042,#140043,#140044,#140045)),
 .UNSPECIFIED.,.F.,.F.,.F.)
B_SPLINE_SURFACE_WITH_KNOTS((3,3),(3,2,3),(-2.87162691077515E-16,1.5707963267949),
(-1.06707356455707,0.,1.06707356455707),.UNSPECIFIED.)
GEOMETRIC_REPRESENTATION_ITEM()
RATIONAL_B_SPLINE_SURFACE(((1.,0.86101371653255,1.,0.86101371653255,1.),
(0.707106781186543,0.608828637654794,0.707106781186543,0.608828637654794,
0.707106781186543),(1.,0.86101371653255,1.,0.86101371653255,1.)))
REPRESENTATION_ITEM('')
SURFACE()
);
#2264=(
BOUNDED_SURFACE()
B_SPLINE_SURFACE(2,2,((#140057,#140058,#140059,#140060,#140061),(#140062,
#140063,#140064,#140065,#140066),(#140067,#140068,#140069,#140070,#140071)),
 .UNSPECIFIED.,.F.,.F.,.F.)
B_SPLINE_SURFACE_WITH_KNOTS((3,3),(3,2,3),(-3.12052122059803E-16,1.5707963267949),
(-0.937275919666155,0.,0.937275919666154),.UNSPECIFIED.)
GEOMETRIC_REPRESENTATION_ITEM()
RATIONAL_B_SPLINE_SURFACE(((1.,0.892184310318489,1.,0.892184310318489,1.),
(0.707106781186544,0.630869575894443,0.707106781186544,0.630869575894443,
0.707106781186544),(1.,0.892184310318489,1.,0.892184310318489,1.)))
REPRESENTATION_ITEM('')
SURFACE()
);
#2265=(
BOUNDED_SURFACE()
B_SPLINE_SURFACE(2,2,((#140083,#140084,#140085,#140086,#140087),(#140088,
#140089,#140090,#140091,#140092),(#140093,#140094,#140095,#140096,#140097)),
 .UNSPECIFIED.,.F.,.F.,.F.)
B_SPLINE_SURFACE_WITH_KNOTS((3,3),(3,2,3),(-2.44248335016467E-15,1.5707963267949),
(-1.94884750401252,-0.974423752006261,1.12987552192351E-32),
 .UNSPECIFIED.)
GEOMETRIC_REPRESENTATION_ITEM()
RATIONAL_B_SPLINE_SURFACE(((1.,0.883641590777673,1.,0.883641590777673,1.),
(0.707106781186542,0.624828960977356,0.707106781186542,0.624828960977356,
0.707106781186542),(1.,0.883641590777673,1.,0.883641590777673,1.)))
REPRESENTATION_ITEM('')
SURFACE()
);
#2266=(
BOUNDED_SURFACE()
B_SPLINE_SURFACE(2,2,((#141085,#141086,#141087,#141088,#141089),(#141090,
#141091,#141092,#141093,#141094),(#141095,#141096,#141097,#141098,#141099)),
 .UNSPECIFIED.,.F.,.F.,.F.)
B_SPLINE_SURFACE_WITH_KNOTS((3,3),(3,2,3),(-4.40321821990384E-16,1.5707963267949),
(-1.1664971520853,0.,1.16649715208529),.UNSPECIFIED.)
GEOMETRIC_REPRESENTATION_ITEM()
RATIONAL_B_SPLINE_SURFACE(((1.,0.834677941920342,1.,0.834677941920342,1.),
(0.707106781186555,0.590206432838712,0.707106781186555,0.590206432838712,
0.707106781186555),(1.,0.834677941920342,1.,0.834677941920342,1.)))
REPRESENTATION_ITEM('')
SURFACE()
);
#2267=(
BOUNDED_SURFACE()
B_SPLINE_SURFACE(2,2,((#141108,#141109,#141110),(#141111,#141112,#141113),
(#141114,#141115,#141116)),.UNSPECIFIED.,.F.,.F.,.F.)
B_SPLINE_SURFACE_WITH_KNOTS((3,3),(3,3),(-3.04212300157654E-16,1.5707963267949),
(-2.35619449019351,-1.57079632679678),.UNSPECIFIED.)
GEOMETRIC_REPRESENTATION_ITEM()
RATIONAL_B_SPLINE_SURFACE(((1.,0.923879532511424,1.),(0.707106781186556,
0.653281482438293,0.707106781186556),(1.,0.923879532511424,1.)))
REPRESENTATION_ITEM('')
SURFACE()
);
#2268=(
BOUNDED_SURFACE()
B_SPLINE_SURFACE(2,2,((#141128,#141129,#141130,#141131,#141132),(#141133,
#141134,#141135,#141136,#141137),(#141138,#141139,#141140,#141141,#141142)),
 .UNSPECIFIED.,.F.,.F.,.F.)
B_SPLINE_SURFACE_WITH_KNOTS((3,3),(3,2,3),(1.38777878069775E-17,1.5707963267949),
(-1.57079632679678,-0.570510447746883,0.429775431304741),.UNSPECIFIED.)
GEOMETRIC_REPRESENTATION_ITEM()
RATIONAL_B_SPLINE_SURFACE(((1.,0.877514024066407,1.,0.877514024066407,1.),
(0.70710678118655,0.620496117003654,0.70710678118655,0.620496117003654,
0.70710678118655),(1.,0.877514024066407,1.,0.877514024066407,1.)))
REPRESENTATION_ITEM('')
SURFACE()
);
#2269=(
BOUNDED_SURFACE()
B_SPLINE_SURFACE(2,2,((#141154,#141155,#141156,#141157,#141158),(#141159,
#141160,#141161,#141162,#141163),(#141164,#141165,#141166,#141167,#141168)),
 .UNSPECIFIED.,.F.,.F.,.F.)
B_SPLINE_SURFACE_WITH_KNOTS((3,3),(3,2,3),(-2.04068455613418E-16,1.5707963267949),
(0.317238733765724,1.23836023442364,2.15948173508156),.UNSPECIFIED.)
GEOMETRIC_REPRESENTATION_ITEM()
RATIONAL_B_SPLINE_SURFACE(((1.,0.895803412613763,1.,0.895803412613763,1.),
(0.707106781186556,0.63342866766925,0.707106781186556,0.63342866766925,
0.707106781186556),(1.,0.895803412613763,1.,0.895803412613763,1.)))
REPRESENTATION_ITEM('')
SURFACE()
);
#2270=(
BOUNDED_SURFACE()
B_SPLINE_SURFACE(2,2,((#141344,#141345,#141346,#141347,#141348),(#141349,
#141350,#141351,#141352,#141353),(#141354,#141355,#141356,#141357,#141358)),
 .UNSPECIFIED.,.F.,.F.,.F.)
B_SPLINE_SURFACE_WITH_KNOTS((3,3),(3,2,3),(-2.00928091613498E-16,1.5707963267949),
(0.492169594955417,1.33946582626418,2.18676205757294),.UNSPECIFIED.)
GEOMETRIC_REPRESENTATION_ITEM()
RATIONAL_B_SPLINE_SURFACE(((1.,0.911595310291363,1.,0.911595310291363,1.),
(0.707106781186556,0.644595225604885,0.707106781186556,0.644595225604885,
0.707106781186556),(1.,0.911595310291363,1.,0.911595310291363,1.)))
REPRESENTATION_ITEM('')
SURFACE()
);
#2271=(
BOUNDED_SURFACE()
B_SPLINE_SURFACE(2,2,((#141547,#141548,#141549),(#141550,#141551,#141552),
(#141553,#141554,#141555)),.UNSPECIFIED.,.F.,.F.,.F.)
B_SPLINE_SURFACE_WITH_KNOTS((3,3),(3,3),(-3.40404913931651E-16,1.5707963267949),
(1.57079632679491,3.14159265358979),.UNSPECIFIED.)
GEOMETRIC_REPRESENTATION_ITEM()
RATIONAL_B_SPLINE_SURFACE(((1.,0.707106781186554,1.),(0.707106781186545,
0.500000000000003,0.707106781186545),(1.,0.707106781186554,1.)))
REPRESENTATION_ITEM('')
SURFACE()
);
#2272=(
BOUNDED_SURFACE()
B_SPLINE_SURFACE(2,2,((#141662,#141663,#141664,#141665,#141666),(#141667,
#141668,#141669,#141670,#141671),(#141672,#141673,#141674,#141675,#141676)),
 .UNSPECIFIED.,.F.,.F.,.F.)
B_SPLINE_SURFACE_WITH_KNOTS((3,3),(3,2,3),(9.65265731632566E-18,1.5707963267949),
(-1.57306506263583,-0.715832961083556,0.141399140468717),.UNSPECIFIED.)
GEOMETRIC_REPRESENTATION_ITEM()
RATIONAL_B_SPLINE_SURFACE(((1.,0.909541807036257,1.,0.909541807036257,1.),
(0.707106781186556,0.643143179528011,0.707106781186556,0.643143179528011,
0.707106781186556),(1.,0.909541807036257,1.,0.909541807036257,1.)))
REPRESENTATION_ITEM('')
SURFACE()
);
#2273=(
BOUNDED_SURFACE()
B_SPLINE_SURFACE(2,2,((#141688,#141689,#141690),(#141691,#141692,#141693),
(#141694,#141695,#141696)),.UNSPECIFIED.,.F.,.F.,.F.)
B_SPLINE_SURFACE_WITH_KNOTS((3,3),(3,3),(-1.07735048008271E-14,1.57079632679491),
(0.133494798627492,1.57079632679493),.UNSPECIFIED.)
GEOMETRIC_REPRESENTATION_ITEM()
RATIONAL_B_SPLINE_SURFACE(((1.,0.752694710045445,1.),(0.707106781186546,
0.532235533636375,0.707106781186546),(1.,0.752694710045445,1.)))
REPRESENTATION_ITEM('')
SURFACE()
);
#2274=(
BOUNDED_SURFACE()
B_SPLINE_SURFACE(2,2,((#141811,#141812,#141813),(#141814,#141815,#141816),
(#141817,#141818,#141819)),.UNSPECIFIED.,.F.,.F.,.F.)
B_SPLINE_SURFACE_WITH_KNOTS((3,3),(3,3),(-7.12649760132934E-17,1.20783157419784),
(0.404259769435194,1.75111622640166),.UNSPECIFIED.)
GEOMETRIC_REPRESENTATION_ITEM()
RATIONAL_B_SPLINE_SURFACE(((1.,0.781688182176695,1.),(0.823118273259482,
0.643421826740624,0.823118273259482),(1.,0.781688182176695,1.)))
REPRESENTATION_ITEM('')
SURFACE()
);
#2275=(
BOUNDED_SURFACE()
B_SPLINE_SURFACE(2,2,((#141851,#141852,#141853),(#141854,#141855,#141856),
(#141857,#141858,#141859)),.UNSPECIFIED.,.F.,.F.,.F.)
B_SPLINE_SURFACE_WITH_KNOTS((3,3),(3,3),(-3.40404913931651E-16,1.5707963267949),
(1.5707963267949,3.14159265358979),.UNSPECIFIED.)
GEOMETRIC_REPRESENTATION_ITEM()
RATIONAL_B_SPLINE_SURFACE(((1.,0.707106781186548,1.),(0.707106781186553,
0.500000000000004,0.707106781186553),(1.,0.707106781186548,1.)))
REPRESENTATION_ITEM('')
SURFACE()
);
#2276=(
BOUNDED_SURFACE()
B_SPLINE_SURFACE(2,2,((#141867,#141868,#141869),(#141870,#141871,#141872),
(#141873,#141874,#141875)),.UNSPECIFIED.,.F.,.F.,.F.)
B_SPLINE_SURFACE_WITH_KNOTS((3,3),(3,3),(-3.38850230422209E-16,1.5707963267949),
(-3.14159265358979,-1.5707963267949),.UNSPECIFIED.)
GEOMETRIC_REPRESENTATION_ITEM()
RATIONAL_B_SPLINE_SURFACE(((1.,0.707106781186548,1.),(0.707106781186553,
0.500000000000004,0.707106781186553),(1.,0.707106781186548,1.)))
REPRESENTATION_ITEM('')
SURFACE()
);
#2277=(
BOUNDED_SURFACE()
B_SPLINE_SURFACE(2,2,((#141883,#141884,#141885),(#141886,#141887,#141888),
(#141889,#141890,#141891)),.UNSPECIFIED.,.F.,.F.,.F.)
B_SPLINE_SURFACE_WITH_KNOTS((3,3),(3,3),(1.04083408558608E-17,1.5707963267949),
(-1.5707963267949,-1.21122148599942),.UNSPECIFIED.)
GEOMETRIC_REPRESENTATION_ITEM()
RATIONAL_B_SPLINE_SURFACE(((1.,0.983881728593355,1.),(0.707106781186553,
0.69570944217391,0.707106781186553),(1.,0.983881728593355,1.)))
REPRESENTATION_ITEM('')
SURFACE()
);
#2278=(
BOUNDED_SURFACE()
B_SPLINE_SURFACE(2,2,((#142040,#142041,#142042,#142043,#142044),(#142045,
#142046,#142047,#142048,#142049),(#142050,#142051,#142052,#142053,#142054)),
 .UNSPECIFIED.,.F.,.F.,.F.)
B_SPLINE_SURFACE_WITH_KNOTS((3,3),(3,2,3),(-3.26817438467699E-16,1.5707963267949),
(-0.0112409050907196,1.17247679255081,2.35619449019235),.UNSPECIFIED.)
GEOMETRIC_REPRESENTATION_ITEM()
RATIONAL_B_SPLINE_SURFACE(((1.,0.829905053082259,1.,0.829905053082259,1.),
(0.70710678118655,0.586831490775449,0.70710678118655,0.586831490775449,
0.70710678118655),(1.,0.829905053082259,1.,0.829905053082259,1.)))
REPRESENTATION_ITEM('')
SURFACE()
);
#2279=(
BOUNDED_SURFACE()
B_SPLINE_SURFACE(2,2,((#142078,#142079,#142080,#142081,#142082),(#142083,
#142084,#142085,#142086,#142087),(#142088,#142089,#142090,#142091,#142092)),
 .UNSPECIFIED.,.F.,.F.,.F.)
B_SPLINE_SURFACE_WITH_KNOTS((3,3),(3,2,3),(-4.37390637964367E-16,1.5707963267949),
(-0.858171546837339,1.11022302462516E-16,0.85817154683734),
 .UNSPECIFIED.)
GEOMETRIC_REPRESENTATION_ITEM()
RATIONAL_B_SPLINE_SURFACE(((1.,0.909346484128941,1.,0.909346484128941,1.),
(0.70710678118655,0.643005065375722,0.70710678118655,0.643005065375722,
0.70710678118655),(1.,0.909346484128941,1.,0.909346484128941,1.)))
REPRESENTATION_ITEM('')
SURFACE()
);
#2280=(
BOUNDED_SURFACE()
B_SPLINE_SURFACE(2,2,((#142107,#142108,#142109,#142110,#142111),(#142112,
#142113,#142114,#142115,#142116),(#142117,#142118,#142119,#142120,#142121)),
 .UNSPECIFIED.,.F.,.F.,.F.)
B_SPLINE_SURFACE_WITH_KNOTS((3,3),(3,2,3),(-3.23084773091812E-16,1.5707963267949),
(-2.9253611858372,-1.9555154025201,-0.98566961920299),.UNSPECIFIED.)
GEOMETRIC_REPRESENTATION_ITEM()
RATIONAL_B_SPLINE_SURFACE(((1.,0.884710895031854,1.,0.884710895031854,1.),
(0.707106781186556,0.625585073266651,0.707106781186556,0.625585073266651,
0.707106781186556),(1.,0.884710895031854,1.,0.884710895031854,1.)))
REPRESENTATION_ITEM('')
SURFACE()
);
#2281=(
BOUNDED_SURFACE()
B_SPLINE_SURFACE(2,2,((#142179,#142180,#142181),(#142182,#142183,#142184),
(#142185,#142186,#142187)),.UNSPECIFIED.,.F.,.F.,.F.)
B_SPLINE_SURFACE_WITH_KNOTS((3,3),(3,3),(-3.40404913931651E-16,1.5707963267949),
(1.5707963267949,3.14159265358979),.UNSPECIFIED.)
GEOMETRIC_REPRESENTATION_ITEM()
RATIONAL_B_SPLINE_SURFACE(((1.,0.707106781186548,1.),(0.70710678118655,
0.500000000000002,0.70710678118655),(1.,0.707106781186548,1.)))
REPRESENTATION_ITEM('')
SURFACE()
);
#2282=(
BOUNDED_SURFACE()
B_SPLINE_SURFACE(2,2,((#142205,#142206,#142207,#142208,#142209),(#142210,
#142211,#142212,#142213,#142214),(#142215,#142216,#142217,#142218,#142219)),
 .UNSPECIFIED.,.F.,.F.,.F.)
B_SPLINE_SURFACE_WITH_KNOTS((3,3),(3,2,3),(-3.38916221447103E-16,1.5707963267949),
(-0.993480418549077,0.,0.993480418549077),.UNSPECIFIED.)
GEOMETRIC_REPRESENTATION_ITEM()
RATIONAL_B_SPLINE_SURFACE(((1.,0.879140723351448,1.,0.879140723351448,1.),
(0.707106781186546,0.621646367099054,0.707106781186546,0.621646367099054,
0.707106781186546),(1.,0.879140723351448,1.,0.879140723351448,1.)))
REPRESENTATION_ITEM('')
SURFACE()
);
#2283=(
BOUNDED_SURFACE()
B_SPLINE_SURFACE(2,2,((#142237,#142238,#142239,#142240,#142241),(#142242,
#142243,#142244,#142245,#142246),(#142247,#142248,#142249,#142250,#142251)),
 .UNSPECIFIED.,.F.,.F.,.F.)
B_SPLINE_SURFACE_WITH_KNOTS((3,3),(3,2,3),(-1.80387197830009E-16,1.5707963267949),
(-2.1740397470008,-1.03404943345041,0.105940880099987),.UNSPECIFIED.)
GEOMETRIC_REPRESENTATION_ITEM()
RATIONAL_B_SPLINE_SURFACE(((1.,0.841903588711717,1.,0.841903588711717,1.),
(0.707106781186553,0.59531573668335,0.707106781186553,0.59531573668335,
0.707106781186553),(1.,0.841903588711717,1.,0.841903588711717,1.)))
REPRESENTATION_ITEM('')
SURFACE()
);
#2284=(
BOUNDED_SURFACE()
B_SPLINE_SURFACE(2,2,((#142263,#142264,#142265),(#142266,#142267,#142268),
(#142269,#142270,#142271)),.UNSPECIFIED.,.F.,.F.,.F.)
B_SPLINE_SURFACE_WITH_KNOTS((3,3),(3,3),(3.04212300157275E-16,1.5707963267949),
(-0.0419015857269754,0.785398163397452),.UNSPECIFIED.)
GEOMETRIC_REPRESENTATION_ITEM()
RATIONAL_B_SPLINE_SURFACE(((1.,0.915659843255931,1.),(0.707106781186539,
0.647469284426472,0.707106781186539),(1.,0.915659843255931,1.)))
REPRESENTATION_ITEM('')
SURFACE()
);
#2285=(
BOUNDED_SURFACE()
B_SPLINE_SURFACE(2,2,((#142283,#142284,#142285),(#142286,#142287,#142288),
(#142289,#142290,#142291)),.UNSPECIFIED.,.F.,.F.,.F.)
B_SPLINE_SURFACE_WITH_KNOTS((3,3),(3,3),(-1.43399263032023E-17,1.5707963267949),
(0.78539816339745,1.5707963267949),.UNSPECIFIED.)
GEOMETRIC_REPRESENTATION_ITEM()
RATIONAL_B_SPLINE_SURFACE(((1.,0.923879532511287,1.),(0.707106781186552,
0.653281482438192,0.707106781186552),(1.,0.923879532511287,1.)))
REPRESENTATION_ITEM('')
SURFACE()
);
#2286=(
BOUNDED_SURFACE()
B_SPLINE_SURFACE(2,2,((#142330,#142331,#142332),(#142333,#142334,#142335),
(#142336,#142337,#142338)),.UNSPECIFIED.,.F.,.F.,.F.)
B_SPLINE_SURFACE_WITH_KNOTS((3,3),(3,3),(1.04083408558608E-17,1.5707963267949),
(-1.5707963267949,2.95409308984431E-16),.UNSPECIFIED.)
GEOMETRIC_REPRESENTATION_ITEM()
RATIONAL_B_SPLINE_SURFACE(((1.,0.707106781186547,1.),(0.707106781186553,
0.500000000000004,0.707106781186553),(1.,0.707106781186547,1.)))
REPRESENTATION_ITEM('')
SURFACE()
);
#2287=(
BOUNDED_SURFACE()
B_SPLINE_SURFACE(2,2,((#142350,#142351,#142352),(#142353,#142354,#142355),
(#142356,#142357,#142358)),.UNSPECIFIED.,.F.,.F.,.F.)
B_SPLINE_SURFACE_WITH_KNOTS((3,3),(3,3),(-1.0408340855861E-17,1.5707963267949),
(-2.76167977375508E-15,1.5707963267949),.UNSPECIFIED.)
GEOMETRIC_REPRESENTATION_ITEM()
RATIONAL_B_SPLINE_SURFACE(((1.,0.707106781186546,1.),(0.707106781186553,
0.500000000000003,0.707106781186553),(1.,0.707106781186546,1.)))
REPRESENTATION_ITEM('')
SURFACE()
);
#2288=(
BOUNDED_SURFACE()
B_SPLINE_SURFACE(2,2,((#142382,#142383,#142384,#142385,#142386),(#142387,
#142388,#142389,#142390,#142391),(#142392,#142393,#142394,#142395,#142396)),
 .UNSPECIFIED.,.F.,.F.,.F.)
B_SPLINE_SURFACE_WITH_KNOTS((3,3),(3,2,3),(-3.33132048898093E-16,1.5707963267949),
(-1.09723005759692,0.,1.09723005759692),.UNSPECIFIED.)
GEOMETRIC_REPRESENTATION_ITEM()
RATIONAL_B_SPLINE_SURFACE(((1.,0.85324761095477,1.,0.85324761095477,1.),
(0.707106781186558,0.603337171737348,0.707106781186558,0.603337171737348,
0.707106781186558),(1.,0.85324761095477,1.,0.85324761095477,1.)))
REPRESENTATION_ITEM('')
SURFACE()
);
#2289=(
BOUNDED_SURFACE()
B_SPLINE_SURFACE(2,2,((#142414,#142415,#142416),(#142417,#142418,#142419),
(#142420,#142421,#142422)),.UNSPECIFIED.,.F.,.F.,.F.)
B_SPLINE_SURFACE_WITH_KNOTS((3,3),(3,3),(-1.07755746139668E-16,1.5707963267949),
(-1.93037116759037,-1.5707963267949),.UNSPECIFIED.)
GEOMETRIC_REPRESENTATION_ITEM()
RATIONAL_B_SPLINE_SURFACE(((1.,0.983881728593356,1.),(0.707106781186554,
0.695709442173911,0.707106781186554),(1.,0.983881728593356,1.)))
REPRESENTATION_ITEM('')
SURFACE()
);
#2290=(
BOUNDED_SURFACE()
B_SPLINE_SURFACE(2,2,((#142555,#142556,#142557,#142558,#142559),(#142560,
#142561,#142562,#142563,#142564),(#142565,#142566,#142567,#142568,#142569)),
 .UNSPECIFIED.,.F.,.F.,.F.)
B_SPLINE_SURFACE_WITH_KNOTS((3,3),(3,2,3),(-3.36658337620736E-16,1.5707963267949),
(-0.939955765746386,-1.11022302462516E-16,0.939955765746385),
 .UNSPECIFIED.)
GEOMETRIC_REPRESENTATION_ITEM()
RATIONAL_B_SPLINE_SURFACE(((1.,0.891578304520668,1.,0.891578304520668,1.),
(0.707106781186548,0.63044106508537,0.707106781186548,0.63044106508537,
0.707106781186548),(1.,0.891578304520668,1.,0.891578304520668,1.)))
REPRESENTATION_ITEM('')
SURFACE()
);
#2291=(
BOUNDED_SURFACE()
B_SPLINE_SURFACE(2,2,((#142581,#142582,#142583,#142584,#142585),(#142586,
#142587,#142588,#142589,#142590),(#142591,#142592,#142593,#142594,#142595)),
 .UNSPECIFIED.,.F.,.F.,.F.)
B_SPLINE_SURFACE_WITH_KNOTS((3,3),(3,2,3),(-1.55728298388104E-16,1.5707963267949),
(-1.94810635916574,-0.974053179581248,1.68810521070105E-12),
 .UNSPECIFIED.)
GEOMETRIC_REPRESENTATION_ITEM()
RATIONAL_B_SPLINE_SURFACE(((1.,0.883728319944464,1.,0.883728319944464,1.),
(0.707106781186545,0.624890287759324,0.707106781186545,0.624890287759324,
0.707106781186545),(1.,0.883728319944464,1.,0.883728319944464,1.)))
REPRESENTATION_ITEM('')
SURFACE()
);
#2292=(
BOUNDED_SURFACE()
B_SPLINE_SURFACE(2,2,((#142747,#142748,#142749,#142750,#142751),(#142752,
#142753,#142754,#142755,#142756),(#142757,#142758,#142759,#142760,#142761)),
 .UNSPECIFIED.,.F.,.F.,.F.)
B_SPLINE_SURFACE_WITH_KNOTS((3,3),(3,2,3),(-2.28159225117958E-16,1.5707963267949),
(-2.35619449019236,-1.53123643686414,-0.706278383535922),.UNSPECIFIED.)
GEOMETRIC_REPRESENTATION_ITEM()
RATIONAL_B_SPLINE_SURFACE(((1.,0.916129842560975,1.,0.916129842560975,1.),
(0.707106781186559,0.64780162412224,0.707106781186559,0.64780162412224,
0.707106781186559),(1.,0.916129842560975,1.,0.916129842560975,1.)))
REPRESENTATION_ITEM('')
SURFACE()
);
#2293=(
BOUNDED_SURFACE()
B_SPLINE_SURFACE(2,2,((#142773,#142774,#142775,#142776,#142777),(#142778,
#142779,#142780,#142781,#142782),(#142783,#142784,#142785,#142786,#142787)),
 .UNSPECIFIED.,.F.,.F.,.F.)
B_SPLINE_SURFACE_WITH_KNOTS((3,3),(3,2,3),(1.54818837825044E-16,1.5707963267949),
(-0.663590463352779,0.191803543921911,1.0471975511966),.UNSPECIFIED.)
GEOMETRIC_REPRESENTATION_ITEM()
RATIONAL_B_SPLINE_SURFACE(((1.,0.909923390286242,1.,0.909923390286242,1.),
(0.70710678118655,0.643412999631658,0.70710678118655,0.643412999631658,
0.70710678118655),(1.,0.909923390286242,1.,0.909923390286242,1.)))
REPRESENTATION_ITEM('')
SURFACE()
);
#2294=(
BOUNDED_SURFACE()
B_SPLINE_SURFACE(2,2,((#142799,#142800,#142801),(#142802,#142803,#142804),
(#142805,#142806,#142807)),.UNSPECIFIED.,.F.,.F.,.F.)
B_SPLINE_SURFACE_WITH_KNOTS((3,3),(3,3),(-2.38131079176154E-16,1.5707963267949),
(1.0471975511966,2.32096244656348),.UNSPECIFIED.)
GEOMETRIC_REPRESENTATION_ITEM()
RATIONAL_B_SPLINE_SURFACE(((1.,0.803953645065829,1.),(0.707106781186556,
0.568481074185697,0.707106781186556),(1.,0.803953645065829,1.)))
REPRESENTATION_ITEM('')
SURFACE()
);
#2295=(
BOUNDED_SURFACE()
B_SPLINE_SURFACE(2,2,((#142821,#142822,#142823),(#142824,#142825,#142826),
(#142827,#142828,#142829)),.UNSPECIFIED.,.F.,.F.,.F.)
B_SPLINE_SURFACE_WITH_KNOTS((3,3),(3,3),(-1.75550993291529E-16,1.5707963267949),
(0.820630207026316,2.0943951023932),.UNSPECIFIED.)
GEOMETRIC_REPRESENTATION_ITEM()
RATIONAL_B_SPLINE_SURFACE(((1.,0.803953645065829,1.),(0.707106781186554,
0.568481074185696,0.707106781186554),(1.,0.803953645065829,1.)))
REPRESENTATION_ITEM('')
SURFACE()
);
#2296=(
BOUNDED_SURFACE()
B_SPLINE_SURFACE(2,2,((#142841,#142842,#142843,#142844,#142845),(#142846,
#142847,#142848,#142849,#142850),(#142851,#142852,#142853,#142854,#142855)),
 .UNSPECIFIED.,.F.,.F.,.F.)
B_SPLINE_SURFACE_WITH_KNOTS((3,3),(3,2,3),(-4.26771686360733E-16,1.5707963267949),
(-1.30899693899481,0.,1.30899693899481),.UNSPECIFIED.)
GEOMETRIC_REPRESENTATION_ITEM()
RATIONAL_B_SPLINE_SURFACE(((1.,0.793353340291521,1.,0.793353340291521,1.),
(0.707106781186554,0.560985526797139,0.707106781186554,0.560985526797139,
0.707106781186554),(1.,0.793353340291521,1.,0.793353340291521,1.)))
REPRESENTATION_ITEM('')
SURFACE()
);
#2297=(
BOUNDED_SURFACE()
B_SPLINE_SURFACE(2,2,((#142926,#142927,#142928),(#142929,#142930,#142931),
(#142932,#142933,#142934)),.UNSPECIFIED.,.F.,.F.,.F.)
B_SPLINE_SURFACE_WITH_KNOTS((3,3),(3,3),(-1.04083408558608E-17,1.5707963267949),
(1.24587053304372,1.5707963267949),.UNSPECIFIED.)
GEOMETRIC_REPRESENTATION_ITEM()
RATIONAL_B_SPLINE_SURFACE(((1.,0.986831905268789,1.),(0.707106781186553,
0.697795532106808,0.707106781186553),(1.,0.986831905268789,1.)))
REPRESENTATION_ITEM('')
SURFACE()
);
#2298=(
BOUNDED_SURFACE()
B_SPLINE_SURFACE(2,2,((#142946,#142947,#142948),(#142949,#142950,#142951),
(#142952,#142953,#142954)),.UNSPECIFIED.,.F.,.F.,.F.)
B_SPLINE_SURFACE_WITH_KNOTS((3,3),(3,3),(-3.40404913931651E-16,1.5707963267949),
(1.5707963267949,3.14159265358979),.UNSPECIFIED.)
GEOMETRIC_REPRESENTATION_ITEM()
RATIONAL_B_SPLINE_SURFACE(((1.,0.707106781186548,1.),(0.707106781186553,
0.500000000000004,0.707106781186553),(1.,0.707106781186548,1.)))
REPRESENTATION_ITEM('')
SURFACE()
);
#2299=(
BOUNDED_SURFACE()
B_SPLINE_SURFACE(2,2,((#142966,#142967,#142968),(#142969,#142970,#142971),
(#142972,#142973,#142974)),.UNSPECIFIED.,.F.,.F.,.F.)
B_SPLINE_SURFACE_WITH_KNOTS((3,3),(3,3),(-3.33074211398212E-16,1.5707963267949),
(-3.14159265358979,-1.86782775822291),.UNSPECIFIED.)
GEOMETRIC_REPRESENTATION_ITEM()
RATIONAL_B_SPLINE_SURFACE(((1.,0.80395364506583,1.),(0.707106781186555,
0.568481074185697,0.707106781186555),(1.,0.80395364506583,1.)))
REPRESENTATION_ITEM('')
SURFACE()
);
#2300=(
BOUNDED_SURFACE()
B_SPLINE_SURFACE(2,2,((#142983,#142984,#142985),(#142986,#142987,#142988),
(#142989,#142990,#142991)),.UNSPECIFIED.,.F.,.F.,.F.)
B_SPLINE_SURFACE_WITH_KNOTS((3,3),(3,3),(-3.32755772175793E-16,1.5707963267949),
(-0.636882447683443,0.636882447683442),.UNSPECIFIED.)
GEOMETRIC_REPRESENTATION_ITEM()
RATIONAL_B_SPLINE_SURFACE(((1.,0.803953645065828,1.),(0.707106781186554,
0.568481074185695,0.707106781186554),(1.,0.803953645065828,1.)))
REPRESENTATION_ITEM('')
SURFACE()
);
#2301=(
BOUNDED_SURFACE()
B_SPLINE_SURFACE(2,2,((#143003,#143004,#143005,#143006,#143007),(#143008,
#143009,#143010,#143011,#143012),(#143013,#143014,#143015,#143016,#143017)),
 .UNSPECIFIED.,.F.,.F.,.F.)
B_SPLINE_SURFACE_WITH_KNOTS((3,3),(3,2,3),(-1.64312426003188E-16,1.5707963267949),
(-2.0943951023932,-1.23900109511851,-0.383607087843824),.UNSPECIFIED.)
GEOMETRIC_REPRESENTATION_ITEM()
RATIONAL_B_SPLINE_SURFACE(((1.,0.909923390286242,1.,0.909923390286242,1.),
(0.707106781186545,0.643412999631653,0.707106781186545,0.643412999631653,
0.707106781186545),(1.,0.909923390286242,1.,0.909923390286242,1.)))
REPRESENTATION_ITEM('')
SURFACE()
);
#2302=(
BOUNDED_SURFACE()
B_SPLINE_SURFACE(2,2,((#143187,#143188,#143189,#143190,#143191),(#143192,
#143193,#143194,#143195,#143196),(#143197,#143198,#143199,#143200,#143201)),
 .UNSPECIFIED.,.F.,.F.,.F.)
B_SPLINE_SURFACE_WITH_KNOTS((3,3),(3,2,3),(-3.04971088561005E-16,1.5707963267949),
(-2.75798556574597,-1.90259155847128,-1.0471975511966),.UNSPECIFIED.)
GEOMETRIC_REPRESENTATION_ITEM()
RATIONAL_B_SPLINE_SURFACE(((1.,0.909923390286243,1.,0.909923390286243,1.),
(0.707106781186553,0.643412999631661,0.707106781186553,0.643412999631661,
0.707106781186553),(1.,0.909923390286243,1.,0.909923390286243,1.)))
REPRESENTATION_ITEM('')
SURFACE()
);
#2303=(
BOUNDED_SURFACE()
B_SPLINE_SURFACE(2,2,((#143213,#143214,#143215),(#143216,#143217,#143218),
(#143219,#143220,#143221)),.UNSPECIFIED.,.F.,.F.,.F.)
B_SPLINE_SURFACE_WITH_KNOTS((3,3),(3,3),(1.72872884261539E-16,1.5707963267949),
(-1.0471975511966,0.226567344170284),.UNSPECIFIED.)
GEOMETRIC_REPRESENTATION_ITEM()
RATIONAL_B_SPLINE_SURFACE(((1.,0.803953645065828,1.),(0.707106781186554,
0.568481074185695,0.707106781186554),(1.,0.803953645065828,1.)))
REPRESENTATION_ITEM('')
SURFACE()
);
#2304=(
BOUNDED_SURFACE()
B_SPLINE_SURFACE(2,2,((#143230,#143231,#143232),(#143233,#143234,#143235),
(#143236,#143237,#143238)),.UNSPECIFIED.,.F.,.F.,.F.)
B_SPLINE_SURFACE_WITH_KNOTS((3,3),(3,3),(1.0220704756512E-16,1.5707963267949),
(-1.27376489536688,1.38777878078145E-17),.UNSPECIFIED.)
GEOMETRIC_REPRESENTATION_ITEM()
RATIONAL_B_SPLINE_SURFACE(((1.,0.80395364506583,1.),(0.707106781186553,
0.568481074185696,0.707106781186553),(1.,0.80395364506583,1.)))
REPRESENTATION_ITEM('')
SURFACE()
);
#2305=(
BOUNDED_SURFACE()
B_SPLINE_SURFACE(2,2,((#143250,#143251,#143252),(#143253,#143254,#143255),
(#143256,#143257,#143258)),.UNSPECIFIED.,.F.,.F.,.F.)
B_SPLINE_SURFACE_WITH_KNOTS((3,3),(3,3),(-1.04083408558608E-17,1.5707963267949),
(-6.80011602582909E-16,1.5707963267949),.UNSPECIFIED.)
GEOMETRIC_REPRESENTATION_ITEM()
RATIONAL_B_SPLINE_SURFACE(((1.,0.707106781186547,1.),(0.707106781186555,
0.500000000000005,0.707106781186555),(1.,0.707106781186547,1.)))
REPRESENTATION_ITEM('')
SURFACE()
);
#2306=(
BOUNDED_SURFACE()
B_SPLINE_SURFACE(2,2,((#143270,#143271,#143272),(#143273,#143274,#143275),
(#143276,#143277,#143278)),.UNSPECIFIED.,.F.,.F.,.F.)
B_SPLINE_SURFACE_WITH_KNOTS((3,3),(3,3),(-1.16510060523539E-16,1.5707963267949),
(1.5707963267949,1.89572212054608),.UNSPECIFIED.)
GEOMETRIC_REPRESENTATION_ITEM()
RATIONAL_B_SPLINE_SURFACE(((1.,0.986831905268789,1.),(0.707106781186554,
0.697795532106808,0.707106781186554),(1.,0.986831905268789,1.)))
REPRESENTATION_ITEM('')
SURFACE()
);
#4089=(
BOUNDED_CURVE()
B_SPLINE_CURVE(2,(#140599,#140600,#140601),.UNSPECIFIED.,.F.,.F.)
B_SPLINE_CURVE_WITH_KNOTS((3,3),(0.,0.128077890591623),.UNSPECIFIED.)
CURVE()
GEOMETRIC_REPRESENTATION_ITEM()
RATIONAL_B_SPLINE_CURVE((1.,1.00129982111734,1.))
REPRESENTATION_ITEM('')
);
#4090=(
BOUNDED_CURVE()
B_SPLINE_CURVE(2,(#140616,#140617,#140618),.UNSPECIFIED.,.F.,.F.)
B_SPLINE_CURVE_WITH_KNOTS((3,3),(0.000362946931860339,0.146205519527569),
 .UNSPECIFIED.)
CURVE()
GEOMETRIC_REPRESENTATION_ITEM()
RATIONAL_B_SPLINE_CURVE((1.00000258096586,1.0005198467923,1.00000237765636))
REPRESENTATION_ITEM('')
);
#4091=(
BOUNDED_CURVE()
B_SPLINE_CURVE(2,(#141526,#141527,#141528),.UNSPECIFIED.,.F.,.F.)
B_SPLINE_CURVE_WITH_KNOTS((3,3),(0.00319674958924355,0.00384559926899821),
 .UNSPECIFIED.)
CURVE()
GEOMETRIC_REPRESENTATION_ITEM()
RATIONAL_B_SPLINE_CURVE((1.00001174504467,1.00001239664656,1.00001282889535))
REPRESENTATION_ITEM('')
);
#4092=(
BOUNDED_CURVE()
B_SPLINE_CURVE(2,(#141532,#141533,#141534),.UNSPECIFIED.,.F.,.F.)
B_SPLINE_CURVE_WITH_KNOTS((3,3),(0.235117374689744,0.605037926847431),
 .UNSPECIFIED.)
CURVE()
GEOMETRIC_REPRESENTATION_ITEM()
RATIONAL_B_SPLINE_CURVE((1.05233383959897,1.08689092491703,1.10064057896449))
REPRESENTATION_ITEM('')
);
#4093=(
BOUNDED_CURVE()
B_SPLINE_CURVE(2,(#141570,#141571,#141572),.UNSPECIFIED.,.F.,.F.)
B_SPLINE_CURVE_WITH_KNOTS((3,3),(1.57192299052648,2.14887151832575),
 .UNSPECIFIED.)
CURVE()
GEOMETRIC_REPRESENTATION_ITEM()
RATIONAL_B_SPLINE_CURVE((6.65976698144355,7.49223785412377,8.17335038631666))
REPRESENTATION_ITEM('')
);
#4094=(
BOUNDED_CURVE()
B_SPLINE_CURVE(2,(#141613,#141614,#141615),.UNSPECIFIED.,.F.,.F.)
B_SPLINE_CURVE_WITH_KNOTS((3,3),(0.270860367343992,0.325892472320335),
 .UNSPECIFIED.)
CURVE()
GEOMETRIC_REPRESENTATION_ITEM()
RATIONAL_B_SPLINE_CURVE((1.54730126785002,1.59219194080314,1.63273127384522))
REPRESENTATION_ITEM('')
);
#4095=(
BOUNDED_CURVE()
B_SPLINE_CURVE(2,(#141631,#141632,#141633),.UNSPECIFIED.,.F.,.F.)
B_SPLINE_CURVE_WITH_KNOTS((3,3),(0.,0.29854563440631),.UNSPECIFIED.)
CURVE()
GEOMETRIC_REPRESENTATION_ITEM()
RATIONAL_B_SPLINE_CURVE((1.,1.04264499839507,1.))
REPRESENTATION_ITEM('')
);
#4096=(
BOUNDED_CURVE()
B_SPLINE_CURVE(2,(#141725,#141726,#141727,#141728),.UNSPECIFIED.,.F.,.F.)
B_SPLINE_CURVE_WITH_KNOTS((3,1,3),(1.66167847180388,2.26230069355391,2.27651444205068),
 .UNSPECIFIED.)
CURVE()
GEOMETRIC_REPRESENTATION_ITEM()
RATIONAL_B_SPLINE_CURVE((6.5568621272732,7.34757944538262,7.99897023989561,
8.01394260001255))
REPRESENTATION_ITEM('')
);
#4097=(
BOUNDED_CURVE()
B_SPLINE_CURVE(2,(#143650,#143651,#143652),.UNSPECIFIED.,.F.,.F.)
B_SPLINE_CURVE_WITH_KNOTS((3,3),(0.,0.28311686851659),.UNSPECIFIED.)
CURVE()
GEOMETRIC_REPRESENTATION_ITEM()
RATIONAL_B_SPLINE_CURVE((1.,1.06870093790198,1.))
REPRESENTATION_ITEM('')
);
#4098=(
BOUNDED_CURVE()
B_SPLINE_CURVE(2,(#143653,#143654,#143655),.UNSPECIFIED.,.F.,.F.)
B_SPLINE_CURVE_WITH_KNOTS((3,3),(0.,0.283116868518929),.UNSPECIFIED.)
CURVE()
GEOMETRIC_REPRESENTATION_ITEM()
RATIONAL_B_SPLINE_CURVE((1.,1.0687009379036,1.))
REPRESENTATION_ITEM('')
);
#4099=(
BOUNDED_CURVE()
B_SPLINE_CURVE(2,(#143729,#143730,#143731),.UNSPECIFIED.,.F.,.F.)
B_SPLINE_CURVE_WITH_KNOTS((3,3),(0.185737456128969,0.362789547470562),
 .UNSPECIFIED.)
CURVE()
GEOMETRIC_REPRESENTATION_ITEM()
RATIONAL_B_SPLINE_CURVE((1.,1.13683142662591,1.01279688953851))
REPRESENTATION_ITEM('')
);
#4100=(
BOUNDED_CURVE()
B_SPLINE_CURVE(2,(#143745,#143746,#143747),.UNSPECIFIED.,.F.,.F.)
B_SPLINE_CURVE_WITH_KNOTS((3,3),(0.00868536478737642,0.185737456128969),
 .UNSPECIFIED.)
CURVE()
GEOMETRIC_REPRESENTATION_ITEM()
RATIONAL_B_SPLINE_CURVE((1.01279688953851,1.13683142662591,1.))
REPRESENTATION_ITEM('')
);
#4101=(
BOUNDED_CURVE()
B_SPLINE_CURVE(2,(#143752,#143753,#143754),.UNSPECIFIED.,.F.,.F.)
B_SPLINE_CURVE_WITH_KNOTS((3,3),(0.,0.0101246152898397),.UNSPECIFIED.)
CURVE()
GEOMETRIC_REPRESENTATION_ITEM()
RATIONAL_B_SPLINE_CURVE((1.,1.01194504282515,1.023099278064))
REPRESENTATION_ITEM('')
);
#4102=(
BOUNDED_CURVE()
B_SPLINE_CURVE(2,(#143755,#143756,#143757),.UNSPECIFIED.,.F.,.F.)
B_SPLINE_CURVE_WITH_KNOTS((3,3),(0.29573730439733,0.30586191968717),
 .UNSPECIFIED.)
CURVE()
GEOMETRIC_REPRESENTATION_ITEM()
RATIONAL_B_SPLINE_CURVE((1.02309927806399,1.01194504282515,1.))
REPRESENTATION_ITEM('')
);
#4103=(
BOUNDED_CURVE()
B_SPLINE_CURVE(2,(#143761,#143762,#143763),.UNSPECIFIED.,.F.,.F.)
B_SPLINE_CURVE_WITH_KNOTS((3,3),(0.185737456128969,0.362789547470561),
 .UNSPECIFIED.)
CURVE()
GEOMETRIC_REPRESENTATION_ITEM()
RATIONAL_B_SPLINE_CURVE((1.,1.13683142662589,1.01279688953851))
REPRESENTATION_ITEM('')
);
#4104=(
BOUNDED_CURVE()
B_SPLINE_CURVE(2,(#143777,#143778,#143779),.UNSPECIFIED.,.F.,.F.)
B_SPLINE_CURVE_WITH_KNOTS((3,3),(0.00868536478737701,0.18573745612897),
 .UNSPECIFIED.)
CURVE()
GEOMETRIC_REPRESENTATION_ITEM()
RATIONAL_B_SPLINE_CURVE((1.01279688953851,1.13683142662591,1.))
REPRESENTATION_ITEM('')
);
#4105=(
BOUNDED_CURVE()
B_SPLINE_CURVE(2,(#143784,#143785,#143786),.UNSPECIFIED.,.F.,.F.)
B_SPLINE_CURVE_WITH_KNOTS((3,3),(0.,0.0101246152898398),.UNSPECIFIED.)
CURVE()
GEOMETRIC_REPRESENTATION_ITEM()
RATIONAL_B_SPLINE_CURVE((1.,1.01194504282515,1.023099278064))
REPRESENTATION_ITEM('')
);
#4106=(
BOUNDED_CURVE()
B_SPLINE_CURVE(2,(#143787,#143788,#143789),.UNSPECIFIED.,.F.,.F.)
B_SPLINE_CURVE_WITH_KNOTS((3,3),(0.29573730439733,0.30586191968717),
 .UNSPECIFIED.)
CURVE()
GEOMETRIC_REPRESENTATION_ITEM()
RATIONAL_B_SPLINE_CURVE((1.023099278064,1.01194504282515,1.))
REPRESENTATION_ITEM('')
);
#4107=(
BOUNDED_CURVE()
B_SPLINE_CURVE(2,(#143926,#143927,#143928),.UNSPECIFIED.,.F.,.F.)
B_SPLINE_CURVE_WITH_KNOTS((3,3),(0.281942572226475,0.665668068688164),
 .UNSPECIFIED.)
CURVE()
GEOMETRIC_REPRESENTATION_ITEM()
RATIONAL_B_SPLINE_CURVE((1.10320422134355,1.12183288632099,1.))
REPRESENTATION_ITEM('')
);
#4108=(
BOUNDED_CURVE()
B_SPLINE_CURVE(2,(#143930,#143931,#143932),.UNSPECIFIED.,.F.,.F.)
B_SPLINE_CURVE_WITH_KNOTS((3,3),(0.,0.283207139377398),.UNSPECIFIED.)
CURVE()
GEOMETRIC_REPRESENTATION_ITEM()
RATIONAL_B_SPLINE_CURVE((1.,1.06875639213164,1.00010378144267))
REPRESENTATION_ITEM('')
);
#4109=(
BOUNDED_CURVE()
B_SPLINE_CURVE(2,(#144536,#144537,#144538),.UNSPECIFIED.,.F.,.F.)
B_SPLINE_CURVE_WITH_KNOTS((3,3),(0.,0.128077890592173),.UNSPECIFIED.)
CURVE()
GEOMETRIC_REPRESENTATION_ITEM()
RATIONAL_B_SPLINE_CURVE((1.,1.001299821138,1.))
REPRESENTATION_ITEM('')
);
#4110=(
BOUNDED_CURVE()
B_SPLINE_CURVE(2,(#144636,#144637,#144638),.UNSPECIFIED.,.F.,.F.)
B_SPLINE_CURVE_WITH_KNOTS((3,3),(0.,0.0065572501027407),.UNSPECIFIED.)
CURVE()
GEOMETRIC_REPRESENTATION_ITEM()
RATIONAL_B_SPLINE_CURVE((1.,1.00078068132504,1.00149559186922))
REPRESENTATION_ITEM('')
);
#4111=(
BOUNDED_CURVE()
B_SPLINE_CURVE(2,(#144967,#144968,#144969),.UNSPECIFIED.,.F.,.F.)
B_SPLINE_CURVE_WITH_KNOTS((3,3),(0.000566681709996598,0.146427783245033),
 .UNSPECIFIED.)
CURVE()
GEOMETRIC_REPRESENTATION_ITEM()
RATIONAL_B_SPLINE_CURVE((1.00000402002378,1.00051937724566,1.))
REPRESENTATION_ITEM('')
);
#4407=SHAPE_REPRESENTATION_RELATIONSHIP('SRR','None',#459332,#4428);
#4428=ADVANCED_BREP_SHAPE_REPRESENTATION('',(#4450,#1620),#459221);
#4450=MANIFOLD_SOLID_BREP('Body',#94626);
#4569=STYLED_ITEM('',(#459505),#4450);
#4570=STYLED_ITEM('',(#459505),#1620);
#4672=CONICAL_SURFACE('',#95787,2.35,0.785398163397448);
#4673=CONICAL_SURFACE('',#95933,17.8449617393671,0.785398163397452);
#4674=CONICAL_SURFACE('',#95988,4.45,0.785398163397449);
#4675=CONICAL_SURFACE('',#96034,8.94496173936711,0.785398163397449);
#4676=CONICAL_SURFACE('',#96037,2.15,0.785398163397448);
#4677=CONICAL_SURFACE('',#96648,1.70000000000068,0.785398163409378);
#4678=CONICAL_SURFACE('',#96655,1.70000000000068,0.785398163385518);
#4679=CONICAL_SURFACE('',#96656,3.3,0.785398163405255);
#4680=CONICAL_SURFACE('',#96688,1.7,0.785398163397448);
#4681=CONICAL_SURFACE('',#96694,1.7,0.785398163397448);
#4682=CONICAL_SURFACE('',#96712,3.3,0.785398163417184);
#4683=CONICAL_SURFACE('',#96758,3.025,0.785398163397444);
#4684=CONICAL_SURFACE('',#96777,3.95,0.78539816339745);
#4685=CONICAL_SURFACE('',#96784,2.25,0.982793723247329);
#4686=CONICAL_SURFACE('',#96794,2.15000000000002,0.78539816339767);
#4687=CONICAL_SURFACE('',#96823,4.45,0.785398163397449);
#4688=CONICAL_SURFACE('',#96825,4.45,0.785398163397449);
#4689=CONICAL_SURFACE('',#96840,8.94496173936711,0.78539816339745);
#4690=CONICAL_SURFACE('',#96849,3.625,0.483447001567199);
#4691=CONICAL_SURFACE('',#96853,1.1,0.588002603547571);
#4692=CONICAL_SURFACE('',#96856,4.43137084989847,0.78539816339745);
#4693=CONICAL_SURFACE('',#96858,4.43137084989847,0.78539816339745);
#4694=CONICAL_SURFACE('',#96860,4.43137084989847,0.78539816339745);
#4695=CONICAL_SURFACE('',#96871,2.75,0.785398163397449);
#4696=CONICAL_SURFACE('',#96872,2.75,0.785398163397449);
#4697=CONICAL_SURFACE('',#96910,3.2,0.785398163397448);
#4698=CONICAL_SURFACE('',#96934,17.8449617393671,0.785398163397452);
#4699=CONICAL_SURFACE('',#96987,3.15,0.785398163397448);
#4700=CONICAL_SURFACE('',#97073,4.68747748340553,0.483447001567199);
#4701=CONICAL_SURFACE('',#97074,4.325,0.785398163397448);
#5126=FACE_BOUND('',#12581,.T.);
#5127=FACE_BOUND('',#12584,.T.);
#5128=FACE_BOUND('',#12585,.T.);
#5129=FACE_BOUND('',#12590,.T.);
#5130=FACE_BOUND('',#12591,.T.);
#5131=FACE_BOUND('',#12592,.T.);
#5132=FACE_BOUND('',#12593,.T.);
#5133=FACE_BOUND('',#12594,.T.);
#5134=FACE_BOUND('',#12605,.T.);
#5135=FACE_BOUND('',#12648,.T.);
#5136=FACE_BOUND('',#12676,.T.);
#5137=FACE_BOUND('',#12677,.T.);
#5138=FACE_BOUND('',#12689,.T.);
#5139=FACE_BOUND('',#12708,.T.);
#5140=FACE_BOUND('',#12768,.T.);
#5141=FACE_BOUND('',#12943,.T.);
#5142=FACE_BOUND('',#12965,.T.);
#5143=FACE_BOUND('',#12969,.T.);
#5144=FACE_BOUND('',#13002,.T.);
#5145=FACE_BOUND('',#13027,.T.);
#5146=FACE_BOUND('',#13029,.T.);
#5147=FACE_BOUND('',#13030,.T.);
#5148=FACE_BOUND('',#13031,.T.);
#5149=FACE_BOUND('',#13045,.T.);
#5150=FACE_BOUND('',#13069,.T.);
#5151=FACE_BOUND('',#13071,.T.);
#5152=FACE_BOUND('',#13080,.T.);
#5153=FACE_BOUND('',#13083,.T.);
#5154=FACE_BOUND('',#13089,.T.);
#5155=FACE_BOUND('',#13123,.T.);
#5156=FACE_BOUND('',#13130,.T.);
#5157=FACE_BOUND('',#13147,.T.);
#5158=FACE_BOUND('',#13199,.T.);
#5159=FACE_BOUND('',#13213,.T.);
#5160=FACE_BOUND('',#13214,.T.);
#5161=FACE_BOUND('',#13215,.T.);
#5352=PLANE('',#95379);
#5353=PLANE('',#95382);
#5354=PLANE('',#95383);
#5355=PLANE('',#95427);
#5356=PLANE('',#95443);
#5357=PLANE('',#95444);
#5358=PLANE('',#95483);
#5359=PLANE('',#95490);
#5360=PLANE('',#95525);
#5361=PLANE('',#95530);
#5362=PLANE('',#95533);
#5363=PLANE('',#95534);
#5364=PLANE('',#95580);
#5365=PLANE('',#95587);
#5366=PLANE('',#95590);
#5367=PLANE('',#95625);
#5368=PLANE('',#95630);
#5369=PLANE('',#95684);
#5370=PLANE('',#95698);
#5371=PLANE('',#95741);
#5372=PLANE('',#95772);
#5373=PLANE('',#95773);
#5374=PLANE('',#95791);
#5375=PLANE('',#95795);
#5376=PLANE('',#95799);
#5377=PLANE('',#95817);
#5378=PLANE('',#95836);
#5379=PLANE('',#95839);
#5380=PLANE('',#95840);
#5381=PLANE('',#95860);
#5382=PLANE('',#95865);
#5383=PLANE('',#95866);
#5384=PLANE('',#95877);
#5385=PLANE('',#95880);
#5386=PLANE('',#95894);
#5387=PLANE('',#95895);
#5388=PLANE('',#95899);
#5389=PLANE('',#95901);
#5390=PLANE('',#95915);
#5391=PLANE('',#95917);
#5392=PLANE('',#95918);
#5393=PLANE('',#95923);
#5394=PLANE('',#95925);
#5395=PLANE('',#95932);
#5396=PLANE('',#95935);
#5397=PLANE('',#95936);
#5398=PLANE('',#95938);
#5399=PLANE('',#95945);
#5400=PLANE('',#95951);
#5401=PLANE('',#95958);
#5402=PLANE('',#95966);
#5403=PLANE('',#95968);
#5404=PLANE('',#95973);
#5405=PLANE('',#95981);
#5406=PLANE('',#95993);
#5407=PLANE('',#95995);
#5408=PLANE('',#95997);
#5409=PLANE('',#95998);
#5410=PLANE('',#96002);
#5411=PLANE('',#96007);
#5412=PLANE('',#96012);
#5413=PLANE('',#96015);
#5414=PLANE('',#96016);
#5415=PLANE('',#96025);
#5416=PLANE('',#96031);
#5417=PLANE('',#96039);
#5418=PLANE('',#96041);
#5419=PLANE('',#96043);
#5420=PLANE('',#96044);
#5421=PLANE('',#96046);
#5422=PLANE('',#96047);
#5423=PLANE('',#96055);
#5424=PLANE('',#96071);
#5425=PLANE('',#96105);
#5426=PLANE('',#96134);
#5427=PLANE('',#96137);
#5428=PLANE('',#96157);
#5429=PLANE('',#96159);
#5430=PLANE('',#96165);
#5431=PLANE('',#96170);
#5432=PLANE('',#96176);
#5433=PLANE('',#96177);
#5434=PLANE('',#96195);
#5435=PLANE('',#96197);
#5436=PLANE('',#96200);
#5437=PLANE('',#96213);
#5438=PLANE('',#96238);
#5439=PLANE('',#96241);
#5440=PLANE('',#96244);
#5441=PLANE('',#96291);
#5442=PLANE('',#96294);
#5443=PLANE('',#96301);
#5444=PLANE('',#96343);
#5445=PLANE('',#96346);
#5446=PLANE('',#96347);
#5447=PLANE('',#96395);
#5448=PLANE('',#96396);
#5449=PLANE('',#96417);
#5450=PLANE('',#96422);
#5451=PLANE('',#96473);
#5452=PLANE('',#96476);
#5453=PLANE('',#96477);
#5454=PLANE('',#96512);
#5455=PLANE('',#96524);
#5456=PLANE('',#96553);
#5457=PLANE('',#96556);
#5458=PLANE('',#96565);
#5459=PLANE('',#96568);
#5460=PLANE('',#96578);
#5461=PLANE('',#96579);
#5462=PLANE('',#96594);
#5463=PLANE('',#96598);
#5464=PLANE('',#96605);
#5465=PLANE('',#96618);
#5466=PLANE('',#96621);
#5467=PLANE('',#96645);
#5468=PLANE('',#96652);
#5469=PLANE('',#96657);
#5470=PLANE('',#96660);
#5471=PLANE('',#96663);
#5472=PLANE('',#96667);
#5473=PLANE('',#96668);
#5474=PLANE('',#96672);
#5475=PLANE('',#96683);
#5476=PLANE('',#96687);
#5477=PLANE('',#96689);
#5478=PLANE('',#96693);
#5479=PLANE('',#96695);
#5480=PLANE('',#96696);
#5481=PLANE('',#96698);
#5482=PLANE('',#96699);
#5483=PLANE('',#96702);
#5484=PLANE('',#96704);
#5485=PLANE('',#96707);
#5486=PLANE('',#96714);
#5487=PLANE('',#96717);
#5488=PLANE('',#96723);
#5489=PLANE('',#96732);
#5490=PLANE('',#96734);
#5491=PLANE('',#96739);
#5492=PLANE('',#96744);
#5493=PLANE('',#96752);
#5494=PLANE('',#96753);
#5495=PLANE('',#96780);
#5496=PLANE('',#96810);
#5497=PLANE('',#96818);
#5498=PLANE('',#96829);
#5499=PLANE('',#96831);
#5500=PLANE('',#96838);
#5501=PLANE('',#96839);
#5502=PLANE('',#96848);
#5503=PLANE('',#96850);
#5504=PLANE('',#96861);
#5505=PLANE('',#96875);
#5506=PLANE('',#96879);
#5507=PLANE('',#96880);
#5508=PLANE('',#96916);
#5509=PLANE('',#96923);
#5510=PLANE('',#96930);
#5511=PLANE('',#96937);
#5512=PLANE('',#96944);
#5513=PLANE('',#96947);
#5514=PLANE('',#96951);
#5515=PLANE('',#96954);
#5516=PLANE('',#96957);
#5517=PLANE('',#96960);
#5518=PLANE('',#96968);
#5519=PLANE('',#96984);
#5520=PLANE('',#96988);
#5521=PLANE('',#96989);
#5522=PLANE('',#97008);
#5523=PLANE('',#97012);
#5524=PLANE('',#97013);
#5525=PLANE('',#97014);
#5526=PLANE('',#97018);
#5527=PLANE('',#97031);
#5528=PLANE('',#97036);
#5529=PLANE('',#97041);
#5530=PLANE('',#97047);
#5531=PLANE('',#97056);
#5532=PLANE('',#97062);
#5533=PLANE('',#97064);
#5534=PLANE('',#97068);
#5535=PLANE('',#97070);
#5536=PLANE('',#97071);
#5537=PLANE('',#97075);
#5538=PLANE('',#97076);
#5539=PLANE('',#97077);
#5540=PLANE('',#97081);
#5541=PLANE('',#97083);
#5542=PLANE('',#97085);
#5543=PLANE('',#97089);
#5544=PLANE('',#97090);
#5545=PLANE('',#97091);
#5546=PLANE('',#97092);
#6205=B_SPLINE_SURFACE_WITH_KNOTS('',3,3,((#140119,#140120,#140121,#140122,
#140123,#140124,#140125,#140126,#140127),(#140128,#140129,#140130,#140131,
#140132,#140133,#140134,#140135,#140136),(#140137,#140138,#140139,#140140,
#140141,#140142,#140143,#140144,#140145),(#140146,#140147,#140148,#140149,
#140150,#140151,#140152,#140153,#140154),(#140155,#140156,#140157,#140158,
#140159,#140160,#140161,#140162,#140163)),.UNSPECIFIED.,.F.,.F.,.F.,(4,
1,4),(4,1,1,1,1,1,4),(0.,0.571428571428571,1.),(0.461365642517441,0.594297668650691,
0.72722969478394,0.793695707850564,0.860161720917189,0.893394727450501,
0.926627733983813),.UNSPECIFIED.);
#6206=B_SPLINE_SURFACE_WITH_KNOTS('',3,3,((#140218,#140219,#140220,#140221,
#140222,#140223),(#140224,#140225,#140226,#140227,#140228,#140229),(#140230,
#140231,#140232,#140233,#140234,#140235),(#140236,#140237,#140238,#140239,
#140240,#140241)),.UNSPECIFIED.,.F.,.F.,.F.,(4,4),(4,1,1,4),(0.,1.),(8.11743420200643E-14,
0.0357756929344898,0.0596261548907622,0.0834766168470346),.UNSPECIFIED.);
#6207=B_SPLINE_SURFACE_WITH_KNOTS('',3,3,((#140256,#140257,#140258,#140259,
#140260,#140261,#140262),(#140263,#140264,#140265,#140266,#140267,#140268,
#140269),(#140270,#140271,#140272,#140273,#140274,#140275,#140276),(#140277,
#140278,#140279,#140280,#140281,#140282,#140283),(#140284,#140285,#140286,
#140287,#140288,#140289,#140290)),.UNSPECIFIED.,.F.,.F.,.F.,(4,1,4),(4,
1,1,1,4),(0.,0.571428571428571,1.),(0.,0.0576772753326012,0.115354550665202,
0.173031825997804,0.403740927328209),.UNSPECIFIED.);
#6208=B_SPLINE_SURFACE_WITH_KNOTS('',3,3,((#144750,#144751,#144752,#144753,
#144754),(#144755,#144756,#144757,#144758,#144759),(#144760,#144761,#144762,
#144763,#144764),(#144765,#144766,#144767,#144768,#144769),(#144770,#144771,
#144772,#144773,#144774)),.UNSPECIFIED.,.F.,.F.,.F.,(4,1,4),(4,1,4),(0.,
0.5,1.),(0.,0.0637546478056962,0.148760844879958),.UNSPECIFIED.);
#6209=B_SPLINE_SURFACE_WITH_KNOTS('',3,3,((#144837,#144838,#144839,#144840,
#144841,#144842,#144843,#144844,#144845,#144846,#144847,#144848,#144849),
(#144850,#144851,#144852,#144853,#144854,#144855,#144856,#144857,#144858,
#144859,#144860,#144861,#144862),(#144863,#144864,#144865,#144866,#144867,
#144868,#144869,#144870,#144871,#144872,#144873,#144874,#144875),(#144876,
#144877,#144878,#144879,#144880,#144881,#144882,#144883,#144884,#144885,
#144886,#144887,#144888),(#144889,#144890,#144891,#144892,#144893,#144894,
#144895,#144896,#144897,#144898,#144899,#144900,#144901)),.UNSPECIFIED.,
 .F.,.F.,.F.,(4,1,4),(4,1,1,1,1,1,1,1,1,1,4),(0.,0.5,1.),(-0.195457271730056,
-0.191966963306305,-0.188476654882554,-0.181496038035052,-0.167534804340048,
-0.13961233695004,-0.125651103255036,-0.111689869560032,-0.0837674021700239,
-0.0558449347800159,0.),.UNSPECIFIED.);
#6210=B_SPLINE_SURFACE_WITH_KNOTS('',3,3,((#145209,#145210,#145211,#145212),
(#145213,#145214,#145215,#145216),(#145217,#145218,#145219,#145220),(#145221,
#145222,#145223,#145224)),.UNSPECIFIED.,.F.,.F.,.F.,(4,4),(4,4),(0.,1.),
(-0.185221475089327,0.29949531162374),.UNSPECIFIED.);
#6211=B_SPLINE_SURFACE_WITH_KNOTS('',3,3,((#145225,#145226,#145227,#145228),
(#145229,#145230,#145231,#145232),(#145233,#145234,#145235,#145236),(#145237,
#145238,#145239,#145240)),.UNSPECIFIED.,.F.,.F.,.F.,(4,4),(4,4),(0.,1.),
(-0.35010463104534,0.22917017018593),.UNSPECIFIED.);
#6212=B_SPLINE_SURFACE_WITH_KNOTS('',3,3,((#145242,#145243,#145244,#145245,
#145246,#145247),(#145248,#145249,#145250,#145251,#145252,#145253),(#145254,
#145255,#145256,#145257,#145258,#145259),(#145260,#145261,#145262,#145263,
#145264,#145265)),.UNSPECIFIED.,.F.,.F.,.F.,(4,4),(4,1,1,4),(0.,1.),(-0.346299380282928,
-0.321815335614959,-0.312633818864471,-0.303452302113982),.UNSPECIFIED.);
#6213=B_SPLINE_SURFACE_WITH_KNOTS('',3,3,((#145274,#145275,#145276,#145277,
#145278),(#145279,#145280,#145281,#145282,#145283),(#145284,#145285,#145286,
#145287,#145288),(#145289,#145290,#145291,#145292,#145293)),
 .UNSPECIFIED.,.F.,.F.,.F.,(4,4),(4,1,4),(0.,1.),(-0.700638140826161,-0.192826413836344,
0.484255888816744),.UNSPECIFIED.);
#6214=B_SPLINE_SURFACE_WITH_KNOTS('',3,3,((#145297,#145298,#145299,#145300,
#145301),(#145302,#145303,#145304,#145305,#145306),(#145307,#145308,#145309,
#145310,#145311),(#145312,#145313,#145314,#145315,#145316)),
 .UNSPECIFIED.,.F.,.F.,.F.,(4,4),(4,1,4),(0.,1.),(-0.780128599420792,-0.0310350531663454,
0.53078510652449),.UNSPECIFIED.);
#6585=FACE_OUTER_BOUND('',#12406,.T.);
#6586=FACE_OUTER_BOUND('',#12407,.T.);
#6587=FACE_OUTER_BOUND('',#12408,.T.);
#6588=FACE_OUTER_BOUND('',#12409,.T.);
#6589=FACE_OUTER_BOUND('',#12410,.T.);
#6590=FACE_OUTER_BOUND('',#12411,.T.);
#6591=FACE_OUTER_BOUND('',#12412,.T.);
#6592=FACE_OUTER_BOUND('',#12413,.T.);
#6593=FACE_OUTER_BOUND('',#12414,.T.);
#6594=FACE_OUTER_BOUND('',#12415,.T.);
#6595=FACE_OUTER_BOUND('',#12416,.T.);
#6596=FACE_OUTER_BOUND('',#12417,.T.);
#6597=FACE_OUTER_BOUND('',#12418,.T.);
#6598=FACE_OUTER_BOUND('',#12419,.T.);
#6599=FACE_OUTER_BOUND('',#12420,.T.);
#6600=FACE_OUTER_BOUND('',#12421,.T.);
#6601=FACE_OUTER_BOUND('',#12422,.T.);
#6602=FACE_OUTER_BOUND('',#12423,.T.);
#6603=FACE_OUTER_BOUND('',#12424,.T.);
#6604=FACE_OUTER_BOUND('',#12425,.T.);
#6605=FACE_OUTER_BOUND('',#12426,.T.);
#6606=FACE_OUTER_BOUND('',#12427,.T.);
#6607=FACE_OUTER_BOUND('',#12428,.T.);
#6608=FACE_OUTER_BOUND('',#12429,.T.);
#6609=FACE_OUTER_BOUND('',#12430,.T.);
#6610=FACE_OUTER_BOUND('',#12431,.T.);
#6611=FACE_OUTER_BOUND('',#12432,.T.);
#6612=FACE_OUTER_BOUND('',#12433,.T.);
#6613=FACE_OUTER_BOUND('',#12434,.T.);
#6614=FACE_OUTER_BOUND('',#12435,.T.);
#6615=FACE_OUTER_BOUND('',#12436,.T.);
#6616=FACE_OUTER_BOUND('',#12437,.T.);
#6617=FACE_OUTER_BOUND('',#12438,.T.);
#6618=FACE_OUTER_BOUND('',#12439,.T.);
#6619=FACE_OUTER_BOUND('',#12440,.T.);
#6620=FACE_OUTER_BOUND('',#12441,.T.);
#6621=FACE_OUTER_BOUND('',#12442,.T.);
#6622=FACE_OUTER_BOUND('',#12443,.T.);
#6623=FACE_OUTER_BOUND('',#12444,.T.);
#6624=FACE_OUTER_BOUND('',#12445,.T.);
#6625=FACE_OUTER_BOUND('',#12446,.T.);
#6626=FACE_OUTER_BOUND('',#12447,.T.);
#6627=FACE_OUTER_BOUND('',#12448,.T.);
#6628=FACE_OUTER_BOUND('',#12449,.T.);
#6629=FACE_OUTER_BOUND('',#12450,.T.);
#6630=FACE_OUTER_BOUND('',#12451,.T.);
#6631=FACE_OUTER_BOUND('',#12452,.T.);
#6632=FACE_OUTER_BOUND('',#12453,.T.);
#6633=FACE_OUTER_BOUND('',#12454,.T.);
#6634=FACE_OUTER_BOUND('',#12455,.T.);
#6635=FACE_OUTER_BOUND('',#12456,.T.);
#6636=FACE_OUTER_BOUND('',#12457,.T.);
#6637=FACE_OUTER_BOUND('',#12458,.T.);
#6638=FACE_OUTER_BOUND('',#12459,.T.);
#6639=FACE_OUTER_BOUND('',#12460,.T.);
#6640=FACE_OUTER_BOUND('',#12461,.T.);
#6641=FACE_OUTER_BOUND('',#12462,.T.);
#6642=FACE_OUTER_BOUND('',#12463,.T.);
#6643=FACE_OUTER_BOUND('',#12464,.T.);
#6644=FACE_OUTER_BOUND('',#12465,.T.);
#6645=FACE_OUTER_BOUND('',#12466,.T.);
#6646=FACE_OUTER_BOUND('',#12467,.T.);
#6647=FACE_OUTER_BOUND('',#12468,.T.);
#6648=FACE_OUTER_BOUND('',#12469,.T.);
#6649=FACE_OUTER_BOUND('',#12470,.T.);
#6650=FACE_OUTER_BOUND('',#12471,.T.);
#6651=FACE_OUTER_BOUND('',#12472,.T.);
#6652=FACE_OUTER_BOUND('',#12473,.T.);
#6653=FACE_OUTER_BOUND('',#12474,.T.);
#6654=FACE_OUTER_BOUND('',#12475,.T.);
#6655=FACE_OUTER_BOUND('',#12476,.T.);
#6656=FACE_OUTER_BOUND('',#12477,.T.);
#6657=FACE_OUTER_BOUND('',#12478,.T.);
#6658=FACE_OUTER_BOUND('',#12479,.T.);
#6659=FACE_OUTER_BOUND('',#12480,.T.);
#6660=FACE_OUTER_BOUND('',#12481,.T.);
#6661=FACE_OUTER_BOUND('',#12482,.T.);
#6662=FACE_OUTER_BOUND('',#12483,.T.);
#6663=FACE_OUTER_BOUND('',#12484,.T.);
#6664=FACE_OUTER_BOUND('',#12485,.T.);
#6665=FACE_OUTER_BOUND('',#12486,.T.);
#6666=FACE_OUTER_BOUND('',#12487,.T.);
#6667=FACE_OUTER_BOUND('',#12488,.T.);
#6668=FACE_OUTER_BOUND('',#12489,.T.);
#6669=FACE_OUTER_BOUND('',#12490,.T.);
#6670=FACE_OUTER_BOUND('',#12491,.T.);
#6671=FACE_OUTER_BOUND('',#12492,.T.);
#6672=FACE_OUTER_BOUND('',#12493,.T.);
#6673=FACE_OUTER_BOUND('',#12494,.T.);
#6674=FACE_OUTER_BOUND('',#12495,.T.);
#6675=FACE_OUTER_BOUND('',#12496,.T.);
#6676=FACE_OUTER_BOUND('',#12497,.T.);
#6677=FACE_OUTER_BOUND('',#12498,.T.);
#6678=FACE_OUTER_BOUND('',#12499,.T.);
#6679=FACE_OUTER_BOUND('',#12500,.T.);
#6680=FACE_OUTER_BOUND('',#12501,.T.);
#6681=FACE_OUTER_BOUND('',#12502,.T.);
#6682=FACE_OUTER_BOUND('',#12503,.T.);
#6683=FACE_OUTER_BOUND('',#12504,.T.);
#6684=FACE_OUTER_BOUND('',#12505,.T.);
#6685=FACE_OUTER_BOUND('',#12506,.T.);
#6686=FACE_OUTER_BOUND('',#12507,.T.);
#6687=FACE_OUTER_BOUND('',#12508,.T.);
#6688=FACE_OUTER_BOUND('',#12509,.T.);
#6689=FACE_OUTER_BOUND('',#12510,.T.);
#6690=FACE_OUTER_BOUND('',#12511,.T.);
#6691=FACE_OUTER_BOUND('',#12512,.T.);
#6692=FACE_OUTER_BOUND('',#12513,.T.);
#6693=FACE_OUTER_BOUND('',#12514,.T.);
#6694=FACE_OUTER_BOUND('',#12515,.T.);
#6695=FACE_OUTER_BOUND('',#12516,.T.);
#6696=FACE_OUTER_BOUND('',#12517,.T.);
#6697=FACE_OUTER_BOUND('',#12518,.T.);
#6698=FACE_OUTER_BOUND('',#12519,.T.);
#6699=FACE_OUTER_BOUND('',#12520,.T.);
#6700=FACE_OUTER_BOUND('',#12521,.T.);
#6701=FACE_OUTER_BOUND('',#12522,.T.);
#6702=FACE_OUTER_BOUND('',#12523,.T.);
#6703=FACE_OUTER_BOUND('',#12524,.T.);
#6704=FACE_OUTER_BOUND('',#12525,.T.);
#6705=FACE_OUTER_BOUND('',#12526,.T.);
#6706=FACE_OUTER_BOUND('',#12527,.T.);
#6707=FACE_OUTER_BOUND('',#12528,.T.);
#6708=FACE_OUTER_BOUND('',#12529,.T.);
#6709=FACE_OUTER_BOUND('',#12530,.T.);
#6710=FACE_OUTER_BOUND('',#12531,.T.);
#6711=FACE_OUTER_BOUND('',#12532,.T.);
#6712=FACE_OUTER_BOUND('',#12533,.T.);
#6713=FACE_OUTER_BOUND('',#12534,.T.);
#6714=FACE_OUTER_BOUND('',#12535,.T.);
#6715=FACE_OUTER_BOUND('',#12536,.T.);
#6716=FACE_OUTER_BOUND('',#12537,.T.);
#6717=FACE_OUTER_BOUND('',#12538,.T.);
#6718=FACE_OUTER_BOUND('',#12539,.T.);
#6719=FACE_OUTER_BOUND('',#12540,.T.);
#6720=FACE_OUTER_BOUND('',#12541,.T.);
#6721=FACE_OUTER_BOUND('',#12542,.T.);
#6722=FACE_OUTER_BOUND('',#12543,.T.);
#6723=FACE_OUTER_BOUND('',#12544,.T.);
#6724=FACE_OUTER_BOUND('',#12545,.T.);
#6725=FACE_OUTER_BOUND('',#12546,.T.);
#6726=FACE_OUTER_BOUND('',#12547,.T.);
#6727=FACE_OUTER_BOUND('',#12548,.T.);
#6728=FACE_OUTER_BOUND('',#12549,.T.);
#6729=FACE_OUTER_BOUND('',#12550,.T.);
#6730=FACE_OUTER_BOUND('',#12551,.T.);
#6731=FACE_OUTER_BOUND('',#12552,.T.);
#6732=FACE_OUTER_BOUND('',#12553,.T.);
#6733=FACE_OUTER_BOUND('',#12554,.T.);
#6734=FACE_OUTER_BOUND('',#12555,.T.);
#6735=FACE_OUTER_BOUND('',#12556,.T.);
#6736=FACE_OUTER_BOUND('',#12557,.T.);
#6737=FACE_OUTER_BOUND('',#12558,.T.);
#6738=FACE_OUTER_BOUND('',#12559,.T.);
#6739=FACE_OUTER_BOUND('',#12560,.T.);
#6740=FACE_OUTER_BOUND('',#12561,.T.);
#6741=FACE_OUTER_BOUND('',#12562,.T.);
#6742=FACE_OUTER_BOUND('',#12563,.T.);
#6743=FACE_OUTER_BOUND('',#12564,.T.);
#6744=FACE_OUTER_BOUND('',#12565,.T.);
#6745=FACE_OUTER_BOUND('',#12566,.T.);
#6746=FACE_OUTER_BOUND('',#12567,.T.);
#6747=FACE_OUTER_BOUND('',#12568,.T.);
#6748=FACE_OUTER_BOUND('',#12569,.T.);
#6749=FACE_OUTER_BOUND('',#12570,.T.);
#6750=FACE_OUTER_BOUND('',#12571,.T.);
#6751=FACE_OUTER_BOUND('',#12572,.T.);
#6752=FACE_OUTER_BOUND('',#12573,.T.);
#6753=FACE_OUTER_BOUND('',#12574,.T.);
#6754=FACE_OUTER_BOUND('',#12575,.T.);
#6755=FACE_OUTER_BOUND('',#12576,.T.);
#6756=FACE_OUTER_BOUND('',#12577,.T.);
#6757=FACE_OUTER_BOUND('',#12578,.T.);
#6758=FACE_OUTER_BOUND('',#12579,.T.);
#6759=FACE_OUTER_BOUND('',#12580,.T.);
#6760=FACE_OUTER_BOUND('',#12582,.T.);
#6761=FACE_OUTER_BOUND('',#12583,.T.);
#6762=FACE_OUTER_BOUND('',#12586,.T.);
#6763=FACE_OUTER_BOUND('',#12587,.T.);
#6764=FACE_OUTER_BOUND('',#12588,.T.);
#6765=FACE_OUTER_BOUND('',#12589,.T.);
#6766=FACE_OUTER_BOUND('',#12595,.T.);
#6767=FACE_OUTER_BOUND('',#12596,.T.);
#6768=FACE_OUTER_BOUND('',#12597,.T.);
#6769=FACE_OUTER_BOUND('',#12598,.T.);
#6770=FACE_OUTER_BOUND('',#12599,.T.);
#6771=FACE_OUTER_BOUND('',#12600,.T.);
#6772=FACE_OUTER_BOUND('',#12601,.T.);
#6773=FACE_OUTER_BOUND('',#12602,.T.);
#6774=FACE_OUTER_BOUND('',#12603,.T.);
#6775=FACE_OUTER_BOUND('',#12604,.T.);
#6776=FACE_OUTER_BOUND('',#12606,.T.);
#6777=FACE_OUTER_BOUND('',#12607,.T.);
#6778=FACE_OUTER_BOUND('',#12608,.T.);
#6779=FACE_OUTER_BOUND('',#12609,.T.);
#6780=FACE_OUTER_BOUND('',#12610,.T.);
#6781=FACE_OUTER_BOUND('',#12611,.T.);
#6782=FACE_OUTER_BOUND('',#12612,.T.);
#6783=FACE_OUTER_BOUND('',#12613,.T.);
#6784=FACE_OUTER_BOUND('',#12614,.T.);
#6785=FACE_OUTER_BOUND('',#12615,.T.);
#6786=FACE_OUTER_BOUND('',#12616,.T.);
#6787=FACE_OUTER_BOUND('',#12617,.T.);
#6788=FACE_OUTER_BOUND('',#12618,.T.);
#6789=FACE_OUTER_BOUND('',#12619,.T.);
#6790=FACE_OUTER_BOUND('',#12620,.T.);
#6791=FACE_OUTER_BOUND('',#12621,.T.);
#6792=FACE_OUTER_BOUND('',#12622,.T.);
#6793=FACE_OUTER_BOUND('',#12623,.T.);
#6794=FACE_OUTER_BOUND('',#12624,.T.);
#6795=FACE_OUTER_BOUND('',#12625,.T.);
#6796=FACE_OUTER_BOUND('',#12626,.T.);
#6797=FACE_OUTER_BOUND('',#12627,.T.);
#6798=FACE_OUTER_BOUND('',#12628,.T.);
#6799=FACE_OUTER_BOUND('',#12629,.T.);
#6800=FACE_OUTER_BOUND('',#12630,.T.);
#6801=FACE_OUTER_BOUND('',#12631,.T.);
#6802=FACE_OUTER_BOUND('',#12632,.T.);
#6803=FACE_OUTER_BOUND('',#12633,.T.);
#6804=FACE_OUTER_BOUND('',#12634,.T.);
#6805=FACE_OUTER_BOUND('',#12635,.T.);
#6806=FACE_OUTER_BOUND('',#12636,.T.);
#6807=FACE_OUTER_BOUND('',#12637,.T.);
#6808=FACE_OUTER_BOUND('',#12638,.T.);
#6809=FACE_OUTER_BOUND('',#12639,.T.);
#6810=FACE_OUTER_BOUND('',#12640,.T.);
#6811=FACE_OUTER_BOUND('',#12641,.T.);
#6812=FACE_OUTER_BOUND('',#12642,.T.);
#6813=FACE_OUTER_BOUND('',#12643,.T.);
#6814=FACE_OUTER_BOUND('',#12644,.T.);
#6815=FACE_OUTER_BOUND('',#12645,.T.);
#6816=FACE_OUTER_BOUND('',#12646,.T.);
#6817=FACE_OUTER_BOUND('',#12647,.T.);
#6818=FACE_OUTER_BOUND('',#12649,.T.);
#6819=FACE_OUTER_BOUND('',#12650,.T.);
#6820=FACE_OUTER_BOUND('',#12651,.T.);
#6821=FACE_OUTER_BOUND('',#12652,.T.);
#6822=FACE_OUTER_BOUND('',#12653,.T.);
#6823=FACE_OUTER_BOUND('',#12654,.T.);
#6824=FACE_OUTER_BOUND('',#12655,.T.);
#6825=FACE_OUTER_BOUND('',#12656,.T.);
#6826=FACE_OUTER_BOUND('',#12657,.T.);
#6827=FACE_OUTER_BOUND('',#12658,.T.);
#6828=FACE_OUTER_BOUND('',#12659,.T.);
#6829=FACE_OUTER_BOUND('',#12660,.T.);
#6830=FACE_OUTER_BOUND('',#12661,.T.);
#6831=FACE_OUTER_BOUND('',#12662,.T.);
#6832=FACE_OUTER_BOUND('',#12663,.T.);
#6833=FACE_OUTER_BOUND('',#12664,.T.);
#6834=FACE_OUTER_BOUND('',#12665,.T.);
#6835=FACE_OUTER_BOUND('',#12666,.T.);
#6836=FACE_OUTER_BOUND('',#12667,.T.);
#6837=FACE_OUTER_BOUND('',#12668,.T.);
#6838=FACE_OUTER_BOUND('',#12669,.T.);
#6839=FACE_OUTER_BOUND('',#12670,.T.);
#6840=FACE_OUTER_BOUND('',#12671,.T.);
#6841=FACE_OUTER_BOUND('',#12672,.T.);
#6842=FACE_OUTER_BOUND('',#12673,.T.);
#6843=FACE_OUTER_BOUND('',#12674,.T.);
#6844=FACE_OUTER_BOUND('',#12675,.T.);
#6845=FACE_OUTER_BOUND('',#12678,.T.);
#6846=FACE_OUTER_BOUND('',#12679,.T.);
#6847=FACE_OUTER_BOUND('',#12680,.T.);
#6848=FACE_OUTER_BOUND('',#12681,.T.);
#6849=FACE_OUTER_BOUND('',#12682,.T.);
#6850=FACE_OUTER_BOUND('',#12683,.T.);
#6851=FACE_OUTER_BOUND('',#12684,.T.);
#6852=FACE_OUTER_BOUND('',#12685,.T.);
#6853=FACE_OUTER_BOUND('',#12686,.T.);
#6854=FACE_OUTER_BOUND('',#12687,.T.);
#6855=FACE_OUTER_BOUND('',#12688,.T.);
#6856=FACE_OUTER_BOUND('',#12690,.T.);
#6857=FACE_OUTER_BOUND('',#12691,.T.);
#6858=FACE_OUTER_BOUND('',#12692,.T.);
#6859=FACE_OUTER_BOUND('',#12693,.T.);
#6860=FACE_OUTER_BOUND('',#12694,.T.);
#6861=FACE_OUTER_BOUND('',#12695,.T.);
#6862=FACE_OUTER_BOUND('',#12696,.T.);
#6863=FACE_OUTER_BOUND('',#12697,.T.);
#6864=FACE_OUTER_BOUND('',#12698,.T.);
#6865=FACE_OUTER_BOUND('',#12699,.T.);
#6866=FACE_OUTER_BOUND('',#12700,.T.);
#6867=FACE_OUTER_BOUND('',#12701,.T.);
#6868=FACE_OUTER_BOUND('',#12702,.T.);
#6869=FACE_OUTER_BOUND('',#12703,.T.);
#6870=FACE_OUTER_BOUND('',#12704,.T.);
#6871=FACE_OUTER_BOUND('',#12705,.T.);
#6872=FACE_OUTER_BOUND('',#12706,.T.);
#6873=FACE_OUTER_BOUND('',#12707,.T.);
#6874=FACE_OUTER_BOUND('',#12709,.T.);
#6875=FACE_OUTER_BOUND('',#12710,.T.);
#6876=FACE_OUTER_BOUND('',#12711,.T.);
#6877=FACE_OUTER_BOUND('',#12712,.T.);
#6878=FACE_OUTER_BOUND('',#12713,.T.);
#6879=FACE_OUTER_BOUND('',#12714,.T.);
#6880=FACE_OUTER_BOUND('',#12715,.T.);
#6881=FACE_OUTER_BOUND('',#12716,.T.);
#6882=FACE_OUTER_BOUND('',#12717,.T.);
#6883=FACE_OUTER_BOUND('',#12718,.T.);
#6884=FACE_OUTER_BOUND('',#12719,.T.);
#6885=FACE_OUTER_BOUND('',#12720,.T.);
#6886=FACE_OUTER_BOUND('',#12721,.T.);
#6887=FACE_OUTER_BOUND('',#12722,.T.);
#6888=FACE_OUTER_BOUND('',#12723,.T.);
#6889=FACE_OUTER_BOUND('',#12724,.T.);
#6890=FACE_OUTER_BOUND('',#12725,.T.);
#6891=FACE_OUTER_BOUND('',#12726,.T.);
#6892=FACE_OUTER_BOUND('',#12727,.T.);
#6893=FACE_OUTER_BOUND('',#12728,.T.);
#6894=FACE_OUTER_BOUND('',#12729,.T.);
#6895=FACE_OUTER_BOUND('',#12730,.T.);
#6896=FACE_OUTER_BOUND('',#12731,.T.);
#6897=FACE_OUTER_BOUND('',#12732,.T.);
#6898=FACE_OUTER_BOUND('',#12733,.T.);
#6899=FACE_OUTER_BOUND('',#12734,.T.);
#6900=FACE_OUTER_BOUND('',#12735,.T.);
#6901=FACE_OUTER_BOUND('',#12736,.T.);
#6902=FACE_OUTER_BOUND('',#12737,.T.);
#6903=FACE_OUTER_BOUND('',#12738,.T.);
#6904=FACE_OUTER_BOUND('',#12739,.T.);
#6905=FACE_OUTER_BOUND('',#12740,.T.);
#6906=FACE_OUTER_BOUND('',#12741,.T.);
#6907=FACE_OUTER_BOUND('',#12742,.T.);
#6908=FACE_OUTER_BOUND('',#12743,.T.);
#6909=FACE_OUTER_BOUND('',#12744,.T.);
#6910=FACE_OUTER_BOUND('',#12745,.T.);
#6911=FACE_OUTER_BOUND('',#12746,.T.);
#6912=FACE_OUTER_BOUND('',#12747,.T.);
#6913=FACE_OUTER_BOUND('',#12748,.T.);
#6914=FACE_OUTER_BOUND('',#12749,.T.);
#6915=FACE_OUTER_BOUND('',#12750,.T.);
#6916=FACE_OUTER_BOUND('',#12751,.T.);
#6917=FACE_OUTER_BOUND('',#12752,.T.);
#6918=FACE_OUTER_BOUND('',#12753,.T.);
#6919=FACE_OUTER_BOUND('',#12754,.T.);
#6920=FACE_OUTER_BOUND('',#12755,.T.);
#6921=FACE_OUTER_BOUND('',#12756,.T.);
#6922=FACE_OUTER_BOUND('',#12757,.T.);
#6923=FACE_OUTER_BOUND('',#12758,.T.);
#6924=FACE_OUTER_BOUND('',#12759,.T.);
#6925=FACE_OUTER_BOUND('',#12760,.T.);
#6926=FACE_OUTER_BOUND('',#12761,.T.);
#6927=FACE_OUTER_BOUND('',#12762,.T.);
#6928=FACE_OUTER_BOUND('',#12763,.T.);
#6929=FACE_OUTER_BOUND('',#12764,.T.);
#6930=FACE_OUTER_BOUND('',#12765,.T.);
#6931=FACE_OUTER_BOUND('',#12766,.T.);
#6932=FACE_OUTER_BOUND('',#12767,.T.);
#6933=FACE_OUTER_BOUND('',#12769,.T.);
#6934=FACE_OUTER_BOUND('',#12770,.T.);
#6935=FACE_OUTER_BOUND('',#12771,.T.);
#6936=FACE_OUTER_BOUND('',#12772,.T.);
#6937=FACE_OUTER_BOUND('',#12773,.T.);
#6938=FACE_OUTER_BOUND('',#12774,.T.);
#6939=FACE_OUTER_BOUND('',#12775,.T.);
#6940=FACE_OUTER_BOUND('',#12776,.T.);
#6941=FACE_OUTER_BOUND('',#12777,.T.);
#6942=FACE_OUTER_BOUND('',#12778,.T.);
#6943=FACE_OUTER_BOUND('',#12779,.T.);
#6944=FACE_OUTER_BOUND('',#12780,.T.);
#6945=FACE_OUTER_BOUND('',#12781,.T.);
#6946=FACE_OUTER_BOUND('',#12782,.T.);
#6947=FACE_OUTER_BOUND('',#12783,.T.);
#6948=FACE_OUTER_BOUND('',#12784,.T.);
#6949=FACE_OUTER_BOUND('',#12785,.T.);
#6950=FACE_OUTER_BOUND('',#12786,.T.);
#6951=FACE_OUTER_BOUND('',#12787,.T.);
#6952=FACE_OUTER_BOUND('',#12788,.T.);
#6953=FACE_OUTER_BOUND('',#12789,.T.);
#6954=FACE_OUTER_BOUND('',#12790,.T.);
#6955=FACE_OUTER_BOUND('',#12791,.T.);
#6956=FACE_OUTER_BOUND('',#12792,.T.);
#6957=FACE_OUTER_BOUND('',#12793,.T.);
#6958=FACE_OUTER_BOUND('',#12794,.T.);
#6959=FACE_OUTER_BOUND('',#12795,.T.);
#6960=FACE_OUTER_BOUND('',#12796,.T.);
#6961=FACE_OUTER_BOUND('',#12797,.T.);
#6962=FACE_OUTER_BOUND('',#12798,.T.);
#6963=FACE_OUTER_BOUND('',#12799,.T.);
#6964=FACE_OUTER_BOUND('',#12800,.T.);
#6965=FACE_OUTER_BOUND('',#12801,.T.);
#6966=FACE_OUTER_BOUND('',#12802,.T.);
#6967=FACE_OUTER_BOUND('',#12803,.T.);
#6968=FACE_OUTER_BOUND('',#12804,.T.);
#6969=FACE_OUTER_BOUND('',#12805,.T.);
#6970=FACE_OUTER_BOUND('',#12806,.T.);
#6971=FACE_OUTER_BOUND('',#12807,.T.);
#6972=FACE_OUTER_BOUND('',#12808,.T.);
#6973=FACE_OUTER_BOUND('',#12809,.T.);
#6974=FACE_OUTER_BOUND('',#12810,.T.);
#6975=FACE_OUTER_BOUND('',#12811,.T.);
#6976=FACE_OUTER_BOUND('',#12812,.T.);
#6977=FACE_OUTER_BOUND('',#12813,.T.);
#6978=FACE_OUTER_BOUND('',#12814,.T.);
#6979=FACE_OUTER_BOUND('',#12815,.T.);
#6980=FACE_OUTER_BOUND('',#12816,.T.);
#6981=FACE_OUTER_BOUND('',#12817,.T.);
#6982=FACE_OUTER_BOUND('',#12818,.T.);
#6983=FACE_OUTER_BOUND('',#12819,.T.);
#6984=FACE_OUTER_BOUND('',#12820,.T.);
#6985=FACE_OUTER_BOUND('',#12821,.T.);
#6986=FACE_OUTER_BOUND('',#12822,.T.);
#6987=FACE_OUTER_BOUND('',#12823,.T.);
#6988=FACE_OUTER_BOUND('',#12824,.T.);
#6989=FACE_OUTER_BOUND('',#12825,.T.);
#6990=FACE_OUTER_BOUND('',#12826,.T.);
#6991=FACE_OUTER_BOUND('',#12827,.T.);
#6992=FACE_OUTER_BOUND('',#12828,.T.);
#6993=FACE_OUTER_BOUND('',#12829,.T.);
#6994=FACE_OUTER_BOUND('',#12830,.T.);
#6995=FACE_OUTER_BOUND('',#12831,.T.);
#6996=FACE_OUTER_BOUND('',#12832,.T.);
#6997=FACE_OUTER_BOUND('',#12833,.T.);
#6998=FACE_OUTER_BOUND('',#12834,.T.);
#6999=FACE_OUTER_BOUND('',#12835,.T.);
#7000=FACE_OUTER_BOUND('',#12836,.T.);
#7001=FACE_OUTER_BOUND('',#12837,.T.);
#7002=FACE_OUTER_BOUND('',#12838,.T.);
#7003=FACE_OUTER_BOUND('',#12839,.T.);
#7004=FACE_OUTER_BOUND('',#12840,.T.);
#7005=FACE_OUTER_BOUND('',#12841,.T.);
#7006=FACE_OUTER_BOUND('',#12842,.T.);
#7007=FACE_OUTER_BOUND('',#12843,.T.);
#7008=FACE_OUTER_BOUND('',#12844,.T.);
#7009=FACE_OUTER_BOUND('',#12845,.T.);
#7010=FACE_OUTER_BOUND('',#12846,.T.);
#7011=FACE_OUTER_BOUND('',#12847,.T.);
#7012=FACE_OUTER_BOUND('',#12848,.T.);
#7013=FACE_OUTER_BOUND('',#12849,.T.);
#7014=FACE_OUTER_BOUND('',#12850,.T.);
#7015=FACE_OUTER_BOUND('',#12851,.T.);
#7016=FACE_OUTER_BOUND('',#12852,.T.);
#7017=FACE_OUTER_BOUND('',#12853,.T.);
#7018=FACE_OUTER_BOUND('',#12854,.T.);
#7019=FACE_OUTER_BOUND('',#12855,.T.);
#7020=FACE_OUTER_BOUND('',#12856,.T.);
#7021=FACE_OUTER_BOUND('',#12857,.T.);
#7022=FACE_OUTER_BOUND('',#12858,.T.);
#7023=FACE_OUTER_BOUND('',#12859,.T.);
#7024=FACE_OUTER_BOUND('',#12860,.T.);
#7025=FACE_OUTER_BOUND('',#12861,.T.);
#7026=FACE_OUTER_BOUND('',#12862,.T.);
#7027=FACE_OUTER_BOUND('',#12863,.T.);
#7028=FACE_OUTER_BOUND('',#12864,.T.);
#7029=FACE_OUTER_BOUND('',#12865,.T.);
#7030=FACE_OUTER_BOUND('',#12866,.T.);
#7031=FACE_OUTER_BOUND('',#12867,.T.);
#7032=FACE_OUTER_BOUND('',#12868,.T.);
#7033=FACE_OUTER_BOUND('',#12869,.T.);
#7034=FACE_OUTER_BOUND('',#12870,.T.);
#7035=FACE_OUTER_BOUND('',#12871,.T.);
#7036=FACE_OUTER_BOUND('',#12872,.T.);
#7037=FACE_OUTER_BOUND('',#12873,.T.);
#7038=FACE_OUTER_BOUND('',#12874,.T.);
#7039=FACE_OUTER_BOUND('',#12875,.T.);
#7040=FACE_OUTER_BOUND('',#12876,.T.);
#7041=FACE_OUTER_BOUND('',#12877,.T.);
#7042=FACE_OUTER_BOUND('',#12878,.T.);
#7043=FACE_OUTER_BOUND('',#12879,.T.);
#7044=FACE_OUTER_BOUND('',#12880,.T.);
#7045=FACE_OUTER_BOUND('',#12881,.T.);
#7046=FACE_OUTER_BOUND('',#12882,.T.);
#7047=FACE_OUTER_BOUND('',#12883,.T.);
#7048=FACE_OUTER_BOUND('',#12884,.T.);
#7049=FACE_OUTER_BOUND('',#12885,.T.);
#7050=FACE_OUTER_BOUND('',#12886,.T.);
#7051=FACE_OUTER_BOUND('',#12887,.T.);
#7052=FACE_OUTER_BOUND('',#12888,.T.);
#7053=FACE_OUTER_BOUND('',#12889,.T.);
#7054=FACE_OUTER_BOUND('',#12890,.T.);
#7055=FACE_OUTER_BOUND('',#12891,.T.);
#7056=FACE_OUTER_BOUND('',#12892,.T.);
#7057=FACE_OUTER_BOUND('',#12893,.T.);
#7058=FACE_OUTER_BOUND('',#12894,.T.);
#7059=FACE_OUTER_BOUND('',#12895,.T.);
#7060=FACE_OUTER_BOUND('',#12896,.T.);
#7061=FACE_OUTER_BOUND('',#12897,.T.);
#7062=FACE_OUTER_BOUND('',#12898,.T.);
#7063=FACE_OUTER_BOUND('',#12899,.T.);
#7064=FACE_OUTER_BOUND('',#12900,.T.);
#7065=FACE_OUTER_BOUND('',#12901,.T.);
#7066=FACE_OUTER_BOUND('',#12902,.T.);
#7067=FACE_OUTER_BOUND('',#12903,.T.);
#7068=FACE_OUTER_BOUND('',#12904,.T.);
#7069=FACE_OUTER_BOUND('',#12905,.T.);
#7070=FACE_OUTER_BOUND('',#12906,.T.);
#7071=FACE_OUTER_BOUND('',#12907,.T.);
#7072=FACE_OUTER_BOUND('',#12908,.T.);
#7073=FACE_OUTER_BOUND('',#12909,.T.);
#7074=FACE_OUTER_BOUND('',#12910,.T.);
#7075=FACE_OUTER_BOUND('',#12911,.T.);
#7076=FACE_OUTER_BOUND('',#12912,.T.);
#7077=FACE_OUTER_BOUND('',#12913,.T.);
#7078=FACE_OUTER_BOUND('',#12914,.T.);
#7079=FACE_OUTER_BOUND('',#12915,.T.);
#7080=FACE_OUTER_BOUND('',#12916,.T.);
#7081=FACE_OUTER_BOUND('',#12917,.T.);
#7082=FACE_OUTER_BOUND('',#12918,.T.);
#7083=FACE_OUTER_BOUND('',#12919,.T.);
#7084=FACE_OUTER_BOUND('',#12920,.T.);
#7085=FACE_OUTER_BOUND('',#12921,.T.);
#7086=FACE_OUTER_BOUND('',#12922,.T.);
#7087=FACE_OUTER_BOUND('',#12923,.T.);
#7088=FACE_OUTER_BOUND('',#12924,.T.);
#7089=FACE_OUTER_BOUND('',#12925,.T.);
#7090=FACE_OUTER_BOUND('',#12926,.T.);
#7091=FACE_OUTER_BOUND('',#12927,.T.);
#7092=FACE_OUTER_BOUND('',#12928,.T.);
#7093=FACE_OUTER_BOUND('',#12929,.T.);
#7094=FACE_OUTER_BOUND('',#12930,.T.);
#7095=FACE_OUTER_BOUND('',#12931,.T.);
#7096=FACE_OUTER_BOUND('',#12932,.T.);
#7097=FACE_OUTER_BOUND('',#12933,.T.);
#7098=FACE_OUTER_BOUND('',#12934,.T.);
#7099=FACE_OUTER_BOUND('',#12935,.T.);
#7100=FACE_OUTER_BOUND('',#12936,.T.);
#7101=FACE_OUTER_BOUND('',#12937,.T.);
#7102=FACE_OUTER_BOUND('',#12938,.T.);
#7103=FACE_OUTER_BOUND('',#12939,.T.);
#7104=FACE_OUTER_BOUND('',#12940,.T.);
#7105=FACE_OUTER_BOUND('',#12941,.T.);
#7106=FACE_OUTER_BOUND('',#12942,.T.);
#7107=FACE_OUTER_BOUND('',#12944,.T.);
#7108=FACE_OUTER_BOUND('',#12945,.T.);
#7109=FACE_OUTER_BOUND('',#12946,.T.);
#7110=FACE_OUTER_BOUND('',#12947,.T.);
#7111=FACE_OUTER_BOUND('',#12948,.T.);
#7112=FACE_OUTER_BOUND('',#12949,.T.);
#7113=FACE_OUTER_BOUND('',#12950,.T.);
#7114=FACE_OUTER_BOUND('',#12951,.T.);
#7115=FACE_OUTER_BOUND('',#12952,.T.);
#7116=FACE_OUTER_BOUND('',#12953,.T.);
#7117=FACE_OUTER_BOUND('',#12954,.T.);
#7118=FACE_OUTER_BOUND('',#12955,.T.);
#7119=FACE_OUTER_BOUND('',#12956,.T.);
#7120=FACE_OUTER_BOUND('',#12957,.T.);
#7121=FACE_OUTER_BOUND('',#12958,.T.);
#7122=FACE_OUTER_BOUND('',#12959,.T.);
#7123=FACE_OUTER_BOUND('',#12960,.T.);
#7124=FACE_OUTER_BOUND('',#12961,.T.);
#7125=FACE_OUTER_BOUND('',#12962,.T.);
#7126=FACE_OUTER_BOUND('',#12963,.T.);
#7127=FACE_OUTER_BOUND('',#12964,.T.);
#7128=FACE_OUTER_BOUND('',#12966,.T.);
#7129=FACE_OUTER_BOUND('',#12967,.T.);
#7130=FACE_OUTER_BOUND('',#12968,.T.);
#7131=FACE_OUTER_BOUND('',#12970,.T.);
#7132=FACE_OUTER_BOUND('',#12971,.T.);
#7133=FACE_OUTER_BOUND('',#12972,.T.);
#7134=FACE_OUTER_BOUND('',#12973,.T.);
#7135=FACE_OUTER_BOUND('',#12974,.T.);
#7136=FACE_OUTER_BOUND('',#12975,.T.);
#7137=FACE_OUTER_BOUND('',#12976,.T.);
#7138=FACE_OUTER_BOUND('',#12977,.T.);
#7139=FACE_OUTER_BOUND('',#12978,.T.);
#7140=FACE_OUTER_BOUND('',#12979,.T.);
#7141=FACE_OUTER_BOUND('',#12980,.T.);
#7142=FACE_OUTER_BOUND('',#12981,.T.);
#7143=FACE_OUTER_BOUND('',#12982,.T.);
#7144=FACE_OUTER_BOUND('',#12983,.T.);
#7145=FACE_OUTER_BOUND('',#12984,.T.);
#7146=FACE_OUTER_BOUND('',#12985,.T.);
#7147=FACE_OUTER_BOUND('',#12986,.T.);
#7148=FACE_OUTER_BOUND('',#12987,.T.);
#7149=FACE_OUTER_BOUND('',#12988,.T.);
#7150=FACE_OUTER_BOUND('',#12989,.T.);
#7151=FACE_OUTER_BOUND('',#12990,.T.);
#7152=FACE_OUTER_BOUND('',#12991,.T.);
#7153=FACE_OUTER_BOUND('',#12992,.T.);
#7154=FACE_OUTER_BOUND('',#12993,.T.);
#7155=FACE_OUTER_BOUND('',#12994,.T.);
#7156=FACE_OUTER_BOUND('',#12995,.T.);
#7157=FACE_OUTER_BOUND('',#12996,.T.);
#7158=FACE_OUTER_BOUND('',#12997,.T.);
#7159=FACE_OUTER_BOUND('',#12998,.T.);
#7160=FACE_OUTER_BOUND('',#12999,.T.);
#7161=FACE_OUTER_BOUND('',#13000,.T.);
#7162=FACE_OUTER_BOUND('',#13001,.T.);
#7163=FACE_OUTER_BOUND('',#13003,.T.);
#7164=FACE_OUTER_BOUND('',#13004,.T.);
#7165=FACE_OUTER_BOUND('',#13005,.T.);
#7166=FACE_OUTER_BOUND('',#13006,.T.);
#7167=FACE_OUTER_BOUND('',#13007,.T.);
#7168=FACE_OUTER_BOUND('',#13008,.T.);
#7169=FACE_OUTER_BOUND('',#13009,.T.);
#7170=FACE_OUTER_BOUND('',#13010,.T.);
#7171=FACE_OUTER_BOUND('',#13011,.T.);
#7172=FACE_OUTER_BOUND('',#13012,.T.);
#7173=FACE_OUTER_BOUND('',#13013,.T.);
#7174=FACE_OUTER_BOUND('',#13014,.T.);
#7175=FACE_OUTER_BOUND('',#13015,.T.);
#7176=FACE_OUTER_BOUND('',#13016,.T.);
#7177=FACE_OUTER_BOUND('',#13017,.T.);
#7178=FACE_OUTER_BOUND('',#13018,.T.);
#7179=FACE_OUTER_BOUND('',#13019,.T.);
#7180=FACE_OUTER_BOUND('',#13020,.T.);
#7181=FACE_OUTER_BOUND('',#13021,.T.);
#7182=FACE_OUTER_BOUND('',#13022,.T.);
#7183=FACE_OUTER_BOUND('',#13023,.T.);
#7184=FACE_OUTER_BOUND('',#13024,.T.);
#7185=FACE_OUTER_BOUND('',#13025,.T.);
#7186=FACE_OUTER_BOUND('',#13026,.T.);
#7187=FACE_OUTER_BOUND('',#13028,.T.);
#7188=FACE_OUTER_BOUND('',#13032,.T.);
#7189=FACE_OUTER_BOUND('',#13033,.T.);
#7190=FACE_OUTER_BOUND('',#13034,.T.);
#7191=FACE_OUTER_BOUND('',#13035,.T.);
#7192=FACE_OUTER_BOUND('',#13036,.T.);
#7193=FACE_OUTER_BOUND('',#13037,.T.);
#7194=FACE_OUTER_BOUND('',#13038,.T.);
#7195=FACE_OUTER_BOUND('',#13039,.T.);
#7196=FACE_OUTER_BOUND('',#13040,.T.);
#7197=FACE_OUTER_BOUND('',#13041,.T.);
#7198=FACE_OUTER_BOUND('',#13042,.T.);
#7199=FACE_OUTER_BOUND('',#13043,.T.);
#7200=FACE_OUTER_BOUND('',#13044,.T.);
#7201=FACE_OUTER_BOUND('',#13046,.T.);
#7202=FACE_OUTER_BOUND('',#13047,.T.);
#7203=FACE_OUTER_BOUND('',#13048,.T.);
#7204=FACE_OUTER_BOUND('',#13049,.T.);
#7205=FACE_OUTER_BOUND('',#13050,.T.);
#7206=FACE_OUTER_BOUND('',#13051,.T.);
#7207=FACE_OUTER_BOUND('',#13052,.T.);
#7208=FACE_OUTER_BOUND('',#13053,.T.);
#7209=FACE_OUTER_BOUND('',#13054,.T.);
#7210=FACE_OUTER_BOUND('',#13055,.T.);
#7211=FACE_OUTER_BOUND('',#13056,.T.);
#7212=FACE_OUTER_BOUND('',#13057,.T.);
#7213=FACE_OUTER_BOUND('',#13058,.T.);
#7214=FACE_OUTER_BOUND('',#13059,.T.);
#7215=FACE_OUTER_BOUND('',#13060,.T.);
#7216=FACE_OUTER_BOUND('',#13061,.T.);
#7217=FACE_OUTER_BOUND('',#13062,.T.);
#7218=FACE_OUTER_BOUND('',#13063,.T.);
#7219=FACE_OUTER_BOUND('',#13064,.T.);
#7220=FACE_OUTER_BOUND('',#13065,.T.);
#7221=FACE_OUTER_BOUND('',#13066,.T.);
#7222=FACE_OUTER_BOUND('',#13067,.T.);
#7223=FACE_OUTER_BOUND('',#13068,.T.);
#7224=FACE_OUTER_BOUND('',#13070,.T.);
#7225=FACE_OUTER_BOUND('',#13072,.T.);
#7226=FACE_OUTER_BOUND('',#13073,.T.);
#7227=FACE_OUTER_BOUND('',#13074,.T.);
#7228=FACE_OUTER_BOUND('',#13075,.T.);
#7229=FACE_OUTER_BOUND('',#13076,.T.);
#7230=FACE_OUTER_BOUND('',#13077,.T.);
#7231=FACE_OUTER_BOUND('',#13078,.T.);
#7232=FACE_OUTER_BOUND('',#13079,.T.);
#7233=FACE_OUTER_BOUND('',#13081,.T.);
#7234=FACE_OUTER_BOUND('',#13082,.T.);
#7235=FACE_OUTER_BOUND('',#13084,.T.);
#7236=FACE_OUTER_BOUND('',#13085,.T.);
#7237=FACE_OUTER_BOUND('',#13086,.T.);
#7238=FACE_OUTER_BOUND('',#13087,.T.);
#7239=FACE_OUTER_BOUND('',#13088,.T.);
#7240=FACE_OUTER_BOUND('',#13090,.T.);
#7241=FACE_OUTER_BOUND('',#13091,.T.);
#7242=FACE_OUTER_BOUND('',#13092,.T.);
#7243=FACE_OUTER_BOUND('',#13093,.T.);
#7244=FACE_OUTER_BOUND('',#13094,.T.);
#7245=FACE_OUTER_BOUND('',#13095,.T.);
#7246=FACE_OUTER_BOUND('',#13096,.T.);
#7247=FACE_OUTER_BOUND('',#13097,.T.);
#7248=FACE_OUTER_BOUND('',#13098,.T.);
#7249=FACE_OUTER_BOUND('',#13099,.T.);
#7250=FACE_OUTER_BOUND('',#13100,.T.);
#7251=FACE_OUTER_BOUND('',#13101,.T.);
#7252=FACE_OUTER_BOUND('',#13102,.T.);
#7253=FACE_OUTER_BOUND('',#13103,.T.);
#7254=FACE_OUTER_BOUND('',#13104,.T.);
#7255=FACE_OUTER_BOUND('',#13105,.T.);
#7256=FACE_OUTER_BOUND('',#13106,.T.);
#7257=FACE_OUTER_BOUND('',#13107,.T.);
#7258=FACE_OUTER_BOUND('',#13108,.T.);
#7259=FACE_OUTER_BOUND('',#13109,.T.);
#7260=FACE_OUTER_BOUND('',#13110,.T.);
#7261=FACE_OUTER_BOUND('',#13111,.T.);
#7262=FACE_OUTER_BOUND('',#13112,.T.);
#7263=FACE_OUTER_BOUND('',#13113,.T.);
#7264=FACE_OUTER_BOUND('',#13114,.T.);
#7265=FACE_OUTER_BOUND('',#13115,.T.);
#7266=FACE_OUTER_BOUND('',#13116,.T.);
#7267=FACE_OUTER_BOUND('',#13117,.T.);
#7268=FACE_OUTER_BOUND('',#13118,.T.);
#7269=FACE_OUTER_BOUND('',#13119,.T.);
#7270=FACE_OUTER_BOUND('',#13120,.T.);
#7271=FACE_OUTER_BOUND('',#13121,.T.);
#7272=FACE_OUTER_BOUND('',#13122,.T.);
#7273=FACE_OUTER_BOUND('',#13124,.T.);
#7274=FACE_OUTER_BOUND('',#13125,.T.);
#7275=FACE_OUTER_BOUND('',#13126,.T.);
#7276=FACE_OUTER_BOUND('',#13127,.T.);
#7277=FACE_OUTER_BOUND('',#13128,.T.);
#7278=FACE_OUTER_BOUND('',#13129,.T.);
#7279=FACE_OUTER_BOUND('',#13131,.T.);
#7280=FACE_OUTER_BOUND('',#13132,.T.);
#7281=FACE_OUTER_BOUND('',#13133,.T.);
#7282=FACE_OUTER_BOUND('',#13134,.T.);
#7283=FACE_OUTER_BOUND('',#13135,.T.);
#7284=FACE_OUTER_BOUND('',#13136,.T.);
#7285=FACE_OUTER_BOUND('',#13137,.T.);
#7286=FACE_OUTER_BOUND('',#13138,.T.);
#7287=FACE_OUTER_BOUND('',#13139,.T.);
#7288=FACE_OUTER_BOUND('',#13140,.T.);
#7289=FACE_OUTER_BOUND('',#13141,.T.);
#7290=FACE_OUTER_BOUND('',#13142,.T.);
#7291=FACE_OUTER_BOUND('',#13143,.T.);
#7292=FACE_OUTER_BOUND('',#13144,.T.);
#7293=FACE_OUTER_BOUND('',#13145,.T.);
#7294=FACE_OUTER_BOUND('',#13146,.T.);
#7295=FACE_OUTER_BOUND('',#13148,.T.);
#7296=FACE_OUTER_BOUND('',#13149,.T.);
#7297=FACE_OUTER_BOUND('',#13150,.T.);
#7298=FACE_OUTER_BOUND('',#13151,.T.);
#7299=FACE_OUTER_BOUND('',#13152,.T.);
#7300=FACE_OUTER_BOUND('',#13153,.T.);
#7301=FACE_OUTER_BOUND('',#13154,.T.);
#7302=FACE_OUTER_BOUND('',#13155,.T.);
#7303=FACE_OUTER_BOUND('',#13156,.T.);
#7304=FACE_OUTER_BOUND('',#13157,.T.);
#7305=FACE_OUTER_BOUND('',#13158,.T.);
#7306=FACE_OUTER_BOUND('',#13159,.T.);
#7307=FACE_OUTER_BOUND('',#13160,.T.);
#7308=FACE_OUTER_BOUND('',#13161,.T.);
#7309=FACE_OUTER_BOUND('',#13162,.T.);
#7310=FACE_OUTER_BOUND('',#13163,.T.);
#7311=FACE_OUTER_BOUND('',#13164,.T.);
#7312=FACE_OUTER_BOUND('',#13165,.T.);
#7313=FACE_OUTER_BOUND('',#13166,.T.);
#7314=FACE_OUTER_BOUND('',#13167,.T.);
#7315=FACE_OUTER_BOUND('',#13168,.T.);
#7316=FACE_OUTER_BOUND('',#13169,.T.);
#7317=FACE_OUTER_BOUND('',#13170,.T.);
#7318=FACE_OUTER_BOUND('',#13171,.T.);
#7319=FACE_OUTER_BOUND('',#13172,.T.);
#7320=FACE_OUTER_BOUND('',#13173,.T.);
#7321=FACE_OUTER_BOUND('',#13174,.T.);
#7322=FACE_OUTER_BOUND('',#13175,.T.);
#7323=FACE_OUTER_BOUND('',#13176,.T.);
#7324=FACE_OUTER_BOUND('',#13177,.T.);
#7325=FACE_OUTER_BOUND('',#13178,.T.);
#7326=FACE_OUTER_BOUND('',#13179,.T.);
#7327=FACE_OUTER_BOUND('',#13180,.T.);
#7328=FACE_OUTER_BOUND('',#13181,.T.);
#7329=FACE_OUTER_BOUND('',#13182,.T.);
#7330=FACE_OUTER_BOUND('',#13183,.T.);
#7331=FACE_OUTER_BOUND('',#13184,.T.);
#7332=FACE_OUTER_BOUND('',#13185,.T.);
#7333=FACE_OUTER_BOUND('',#13186,.T.);
#7334=FACE_OUTER_BOUND('',#13187,.T.);
#7335=FACE_OUTER_BOUND('',#13188,.T.);
#7336=FACE_OUTER_BOUND('',#13189,.T.);
#7337=FACE_OUTER_BOUND('',#13190,.T.);
#7338=FACE_OUTER_BOUND('',#13191,.T.);
#7339=FACE_OUTER_BOUND('',#13192,.T.);
#7340=FACE_OUTER_BOUND('',#13193,.T.);
#7341=FACE_OUTER_BOUND('',#13194,.T.);
#7342=FACE_OUTER_BOUND('',#13195,.T.);
#7343=FACE_OUTER_BOUND('',#13196,.T.);
#7344=FACE_OUTER_BOUND('',#13197,.T.);
#7345=FACE_OUTER_BOUND('',#13198,.T.);
#7346=FACE_OUTER_BOUND('',#13200,.T.);
#7347=FACE_OUTER_BOUND('',#13201,.T.);
#7348=FACE_OUTER_BOUND('',#13202,.T.);
#7349=FACE_OUTER_BOUND('',#13203,.T.);
#7350=FACE_OUTER_BOUND('',#13204,.T.);
#7351=FACE_OUTER_BOUND('',#13205,.T.);
#7352=FACE_OUTER_BOUND('',#13206,.T.);
#7353=FACE_OUTER_BOUND('',#13207,.T.);
#7354=FACE_OUTER_BOUND('',#13208,.T.);
#7355=FACE_OUTER_BOUND('',#13209,.T.);
#7356=FACE_OUTER_BOUND('',#13210,.T.);
#7357=FACE_OUTER_BOUND('',#13211,.T.);
#7358=FACE_OUTER_BOUND('',#13212,.T.);
#7359=FACE_OUTER_BOUND('',#13216,.T.);
#7360=FACE_OUTER_BOUND('',#13217,.T.);
#7361=FACE_OUTER_BOUND('',#13218,.T.);
#7362=FACE_OUTER_BOUND('',#13219,.T.);
#7363=FACE_OUTER_BOUND('',#13220,.T.);
#12406=EDGE_LOOP('',(#59316,#59317,#59318,#59319));
#12407=EDGE_LOOP('',(#59320,#59321,#59322,#59323));
#12408=EDGE_LOOP('',(#59324,#59325,#59326,#59327));
#12409=EDGE_LOOP('',(#59328,#59329,#59330,#59331));
#12410=EDGE_LOOP('',(#59332,#59333,#59334,#59335));
#12411=EDGE_LOOP('',(#59336,#59337,#59338,#59339));
#12412=EDGE_LOOP('',(#59340,#59341,#59342,#59343));
#12413=EDGE_LOOP('',(#59344,#59345,#59346,#59347));
#12414=EDGE_LOOP('',(#59348,#59349,#59350,#59351));
#12415=EDGE_LOOP('',(#59352,#59353,#59354,#59355));
#12416=EDGE_LOOP('',(#59356,#59357,#59358,#59359,#59360,#59361,#59362,#59363,
#59364,#59365));
#12417=EDGE_LOOP('',(#59366,#59367,#59368,#59369));
#12418=EDGE_LOOP('',(#59370,#59371,#59372,#59373));
#12419=EDGE_LOOP('',(#59374,#59375,#59376,#59377));
#12420=EDGE_LOOP('',(#59378,#59379,#59380,#59381));
#12421=EDGE_LOOP('',(#59382,#59383,#59384,#59385,#59386,#59387,#59388,#59389,
#59390,#59391));
#12422=EDGE_LOOP('',(#59392,#59393,#59394,#59395));
#12423=EDGE_LOOP('',(#59396,#59397,#59398,#59399));
#12424=EDGE_LOOP('',(#59400,#59401,#59402,#59403));
#12425=EDGE_LOOP('',(#59404,#59405,#59406,#59407));
#12426=EDGE_LOOP('',(#59408,#59409,#59410,#59411));
#12427=EDGE_LOOP('',(#59412,#59413,#59414,#59415));
#12428=EDGE_LOOP('',(#59416,#59417,#59418,#59419));
#12429=EDGE_LOOP('',(#59420,#59421,#59422,#59423));
#12430=EDGE_LOOP('',(#59424,#59425,#59426,#59427));
#12431=EDGE_LOOP('',(#59428,#59429,#59430,#59431));
#12432=EDGE_LOOP('',(#59432,#59433,#59434,#59435));
#12433=EDGE_LOOP('',(#59436,#59437,#59438,#59439));
#12434=EDGE_LOOP('',(#59440,#59441,#59442,#59443,#59444));
#12435=EDGE_LOOP('',(#59445,#59446,#59447,#59448));
#12436=EDGE_LOOP('',(#59449,#59450,#59451,#59452));
#12437=EDGE_LOOP('',(#59453,#59454,#59455,#59456));
#12438=EDGE_LOOP('',(#59457,#59458,#59459,#59460));
#12439=EDGE_LOOP('',(#59461,#59462,#59463,#59464));
#12440=EDGE_LOOP('',(#59465,#59466,#59467,#59468,#59469,#59470,#59471,#59472,
#59473,#59474,#59475,#59476,#59477,#59478,#59479,#59480));
#12441=EDGE_LOOP('',(#59481,#59482,#59483,#59484));
#12442=EDGE_LOOP('',(#59485,#59486,#59487,#59488));
#12443=EDGE_LOOP('',(#59489,#59490,#59491,#59492,#59493,#59494,#59495,#59496,
#59497,#59498,#59499,#59500,#59501,#59502));
#12444=EDGE_LOOP('',(#59503,#59504,#59505,#59506));
#12445=EDGE_LOOP('',(#59507,#59508,#59509,#59510));
#12446=EDGE_LOOP('',(#59511,#59512,#59513,#59514));
#12447=EDGE_LOOP('',(#59515,#59516,#59517,#59518));
#12448=EDGE_LOOP('',(#59519,#59520,#59521,#59522));
#12449=EDGE_LOOP('',(#59523,#59524,#59525,#59526));
#12450=EDGE_LOOP('',(#59527,#59528,#59529,#59530));
#12451=EDGE_LOOP('',(#59531,#59532,#59533,#59534));
#12452=EDGE_LOOP('',(#59535,#59536,#59537,#59538));
#12453=EDGE_LOOP('',(#59539,#59540,#59541,#59542));
#12454=EDGE_LOOP('',(#59543,#59544,#59545,#59546));
#12455=EDGE_LOOP('',(#59547,#59548,#59549,#59550));
#12456=EDGE_LOOP('',(#59551,#59552,#59553,#59554,#59555,#59556));
#12457=EDGE_LOOP('',(#59557,#59558,#59559,#59560));
#12458=EDGE_LOOP('',(#59561,#59562,#59563,#59564));
#12459=EDGE_LOOP('',(#59565,#59566,#59567,#59568));
#12460=EDGE_LOOP('',(#59569,#59570,#59571,#59572));
#12461=EDGE_LOOP('',(#59573,#59574,#59575,#59576,#59577,#59578,#59579,#59580,
#59581,#59582,#59583,#59584));
#12462=EDGE_LOOP('',(#59585,#59586,#59587,#59588));
#12463=EDGE_LOOP('',(#59589,#59590,#59591,#59592));
#12464=EDGE_LOOP('',(#59593,#59594,#59595,#59596));
#12465=EDGE_LOOP('',(#59597,#59598,#59599,#59600));
#12466=EDGE_LOOP('',(#59601,#59602,#59603,#59604));
#12467=EDGE_LOOP('',(#59605,#59606,#59607,#59608));
#12468=EDGE_LOOP('',(#59609,#59610,#59611,#59612));
#12469=EDGE_LOOP('',(#59613,#59614,#59615,#59616));
#12470=EDGE_LOOP('',(#59617,#59618,#59619,#59620));
#12471=EDGE_LOOP('',(#59621,#59622,#59623,#59624));
#12472=EDGE_LOOP('',(#59625,#59626,#59627,#59628));
#12473=EDGE_LOOP('',(#59629,#59630,#59631,#59632,#59633,#59634));
#12474=EDGE_LOOP('',(#59635,#59636,#59637,#59638));
#12475=EDGE_LOOP('',(#59639,#59640,#59641,#59642));
#12476=EDGE_LOOP('',(#59643,#59644,#59645,#59646));
#12477=EDGE_LOOP('',(#59647,#59648,#59649,#59650));
#12478=EDGE_LOOP('',(#59651,#59652,#59653,#59654,#59655,#59656));
#12479=EDGE_LOOP('',(#59657,#59658,#59659,#59660,#59661,#59662,#59663,#59664,
#59665,#59666,#59667));
#12480=EDGE_LOOP('',(#59668,#59669,#59670,#59671));
#12481=EDGE_LOOP('',(#59672,#59673,#59674,#59675));
#12482=EDGE_LOOP('',(#59676,#59677,#59678,#59679));
#12483=EDGE_LOOP('',(#59680,#59681,#59682,#59683));
#12484=EDGE_LOOP('',(#59684,#59685,#59686,#59687));
#12485=EDGE_LOOP('',(#59688,#59689,#59690,#59691));
#12486=EDGE_LOOP('',(#59692,#59693,#59694,#59695));
#12487=EDGE_LOOP('',(#59696,#59697,#59698,#59699));
#12488=EDGE_LOOP('',(#59700,#59701,#59702,#59703));
#12489=EDGE_LOOP('',(#59704,#59705,#59706,#59707));
#12490=EDGE_LOOP('',(#59708,#59709,#59710,#59711));
#12491=EDGE_LOOP('',(#59712,#59713,#59714,#59715));
#12492=EDGE_LOOP('',(#59716,#59717,#59718,#59719));
#12493=EDGE_LOOP('',(#59720,#59721,#59722,#59723));
#12494=EDGE_LOOP('',(#59724,#59725,#59726,#59727));
#12495=EDGE_LOOP('',(#59728,#59729,#59730,#59731));
#12496=EDGE_LOOP('',(#59732,#59733,#59734,#59735));
#12497=EDGE_LOOP('',(#59736,#59737,#59738,#59739));
#12498=EDGE_LOOP('',(#59740,#59741,#59742,#59743));
#12499=EDGE_LOOP('',(#59744,#59745,#59746,#59747));
#12500=EDGE_LOOP('',(#59748,#59749,#59750,#59751));
#12501=EDGE_LOOP('',(#59752,#59753,#59754,#59755,#59756,#59757,#59758,#59759,
#59760,#59761,#59762,#59763,#59764,#59765));
#12502=EDGE_LOOP('',(#59766,#59767,#59768,#59769));
#12503=EDGE_LOOP('',(#59770,#59771,#59772,#59773));
#12504=EDGE_LOOP('',(#59774,#59775,#59776,#59777));
#12505=EDGE_LOOP('',(#59778,#59779,#59780,#59781));
#12506=EDGE_LOOP('',(#59782,#59783,#59784,#59785));
#12507=EDGE_LOOP('',(#59786,#59787,#59788,#59789));
#12508=EDGE_LOOP('',(#59790,#59791,#59792,#59793));
#12509=EDGE_LOOP('',(#59794,#59795,#59796,#59797));
#12510=EDGE_LOOP('',(#59798,#59799,#59800,#59801));
#12511=EDGE_LOOP('',(#59802,#59803,#59804,#59805));
#12512=EDGE_LOOP('',(#59806,#59807,#59808,#59809));
#12513=EDGE_LOOP('',(#59810,#59811,#59812,#59813));
#12514=EDGE_LOOP('',(#59814,#59815,#59816,#59817));
#12515=EDGE_LOOP('',(#59818,#59819,#59820,#59821));
#12516=EDGE_LOOP('',(#59822,#59823,#59824,#59825,#59826,#59827,#59828,#59829,
#59830));
#12517=EDGE_LOOP('',(#59831,#59832,#59833,#59834));
#12518=EDGE_LOOP('',(#59835,#59836,#59837,#59838));
#12519=EDGE_LOOP('',(#59839,#59840,#59841,#59842));
#12520=EDGE_LOOP('',(#59843,#59844,#59845,#59846));
#12521=EDGE_LOOP('',(#59847,#59848,#59849,#59850));
#12522=EDGE_LOOP('',(#59851,#59852,#59853,#59854));
#12523=EDGE_LOOP('',(#59855,#59856,#59857,#59858));
#12524=EDGE_LOOP('',(#59859,#59860,#59861,#59862));
#12525=EDGE_LOOP('',(#59863,#59864,#59865,#59866));
#12526=EDGE_LOOP('',(#59867,#59868,#59869,#59870));
#12527=EDGE_LOOP('',(#59871,#59872,#59873,#59874));
#12528=EDGE_LOOP('',(#59875,#59876,#59877,#59878));
#12529=EDGE_LOOP('',(#59879,#59880,#59881,#59882));
#12530=EDGE_LOOP('',(#59883,#59884,#59885,#59886));
#12531=EDGE_LOOP('',(#59887,#59888,#59889,#59890));
#12532=EDGE_LOOP('',(#59891,#59892,#59893,#59894));
#12533=EDGE_LOOP('',(#59895,#59896,#59897,#59898));
#12534=EDGE_LOOP('',(#59899,#59900,#59901,#59902));
#12535=EDGE_LOOP('',(#59903,#59904,#59905,#59906));
#12536=EDGE_LOOP('',(#59907,#59908,#59909,#59910));
#12537=EDGE_LOOP('',(#59911,#59912,#59913,#59914));
#12538=EDGE_LOOP('',(#59915,#59916,#59917,#59918));
#12539=EDGE_LOOP('',(#59919,#59920,#59921,#59922));
#12540=EDGE_LOOP('',(#59923,#59924,#59925,#59926,#59927,#59928));
#12541=EDGE_LOOP('',(#59929,#59930,#59931,#59932,#59933,#59934,#59935,#59936,
#59937,#59938,#59939,#59940,#59941,#59942,#59943,#59944));
#12542=EDGE_LOOP('',(#59945,#59946,#59947,#59948));
#12543=EDGE_LOOP('',(#59949,#59950,#59951,#59952));
#12544=EDGE_LOOP('',(#59953,#59954,#59955,#59956));
#12545=EDGE_LOOP('',(#59957,#59958,#59959,#59960));
#12546=EDGE_LOOP('',(#59961,#59962,#59963,#59964));
#12547=EDGE_LOOP('',(#59965,#59966,#59967,#59968));
#12548=EDGE_LOOP('',(#59969,#59970,#59971,#59972));
#12549=EDGE_LOOP('',(#59973,#59974,#59975,#59976));
#12550=EDGE_LOOP('',(#59977,#59978,#59979,#59980));
#12551=EDGE_LOOP('',(#59981,#59982,#59983,#59984,#59985,#59986,#59987,#59988));
#12552=EDGE_LOOP('',(#59989,#59990,#59991,#59992));
#12553=EDGE_LOOP('',(#59993,#59994,#59995,#59996));
#12554=EDGE_LOOP('',(#59997,#59998,#59999,#60000));
#12555=EDGE_LOOP('',(#60001,#60002,#60003,#60004));
#12556=EDGE_LOOP('',(#60005,#60006,#60007,#60008,#60009,#60010,#60011,#60012,
#60013));
#12557=EDGE_LOOP('',(#60014,#60015,#60016,#60017));
#12558=EDGE_LOOP('',(#60018,#60019,#60020,#60021));
#12559=EDGE_LOOP('',(#60022,#60023,#60024,#60025));
#12560=EDGE_LOOP('',(#60026,#60027,#60028,#60029));
#12561=EDGE_LOOP('',(#60030,#60031,#60032,#60033));
#12562=EDGE_LOOP('',(#60034,#60035,#60036,#60037));
#12563=EDGE_LOOP('',(#60038,#60039,#60040,#60041));
#12564=EDGE_LOOP('',(#60042,#60043,#60044,#60045));
#12565=EDGE_LOOP('',(#60046,#60047,#60048,#60049));
#12566=EDGE_LOOP('',(#60050,#60051,#60052,#60053));
#12567=EDGE_LOOP('',(#60054,#60055,#60056,#60057));
#12568=EDGE_LOOP('',(#60058,#60059,#60060,#60061));
#12569=EDGE_LOOP('',(#60062,#60063,#60064,#60065,#60066,#60067,#60068,#60069));
#12570=EDGE_LOOP('',(#60070,#60071,#60072,#60073));
#12571=EDGE_LOOP('',(#60074,#60075,#60076,#60077));
#12572=EDGE_LOOP('',(#60078,#60079,#60080,#60081));
#12573=EDGE_LOOP('',(#60082,#60083,#60084,#60085));
#12574=EDGE_LOOP('',(#60086,#60087,#60088,#60089,#60090,#60091,#60092,#60093,
#60094,#60095,#60096,#60097,#60098,#60099,#60100,#60101,#60102,#60103));
#12575=EDGE_LOOP('',(#60104,#60105,#60106,#60107,#60108,#60109));
#12576=EDGE_LOOP('',(#60110,#60111,#60112,#60113));
#12577=EDGE_LOOP('',(#60114,#60115,#60116,#60117,#60118,#60119,#60120,#60121,
#60122,#60123,#60124,#60125,#60126,#60127));
#12578=EDGE_LOOP('',(#60128,#60129,#60130,#60131,#60132,#60133));
#12579=EDGE_LOOP('',(#60134,#60135,#60136,#60137));
#12580=EDGE_LOOP('',(#60138,#60139,#60140,#60141,#60142,#60143,#60144,#60145,
#60146,#60147,#60148,#60149,#60150,#60151,#60152,#60153,#60154,#60155,#60156,
#60157,#60158,#60159,#60160,#60161,#60162,#60163,#60164,#60165,#60166,#60167,
#60168,#60169));
#12581=EDGE_LOOP('',(#60170));
#12582=EDGE_LOOP('',(#60171,#60172,#60173,#60174));
#12583=EDGE_LOOP('',(#60175,#60176,#60177,#60178,#60179,#60180,#60181,#60182,
#60183,#60184,#60185,#60186,#60187,#60188,#60189,#60190,#60191,#60192,#60193,
#60194,#60195,#60196,#60197));
#12584=EDGE_LOOP('',(#60198,#60199,#60200,#60201,#60202,#60203,#60204,#60205,
#60206,#60207,#60208,#60209,#60210,#60211));
#12585=EDGE_LOOP('',(#60212));
#12586=EDGE_LOOP('',(#60213,#60214,#60215,#60216,#60217,#60218));
#12587=EDGE_LOOP('',(#60219,#60220,#60221,#60222));
#12588=EDGE_LOOP('',(#60223,#60224,#60225,#60226));
#12589=EDGE_LOOP('',(#60227,#60228,#60229,#60230,#60231,#60232,#60233,#60234,
#60235,#60236,#60237,#60238,#60239,#60240,#60241,#60242,#60243,#60244,#60245,
#60246,#60247,#60248,#60249,#60250,#60251,#60252));
#12590=EDGE_LOOP('',(#60253));
#12591=EDGE_LOOP('',(#60254,#60255,#60256,#60257));
#12592=EDGE_LOOP('',(#60258));
#12593=EDGE_LOOP('',(#60259));
#12594=EDGE_LOOP('',(#60260));
#12595=EDGE_LOOP('',(#60261,#60262,#60263,#60264));
#12596=EDGE_LOOP('',(#60265,#60266,#60267,#60268,#60269,#60270));
#12597=EDGE_LOOP('',(#60271,#60272,#60273,#60274));
#12598=EDGE_LOOP('',(#60275,#60276,#60277,#60278));
#12599=EDGE_LOOP('',(#60279,#60280,#60281,#60282,#60283,#60284));
#12600=EDGE_LOOP('',(#60285,#60286,#60287,#60288,#60289,#60290,#60291,#60292,
#60293,#60294,#60295,#60296,#60297,#60298,#60299,#60300,#60301,#60302,#60303,
#60304,#60305,#60306,#60307,#60308,#60309));
#12601=EDGE_LOOP('',(#60310,#60311,#60312,#60313));
#12602=EDGE_LOOP('',(#60314,#60315,#60316,#60317));
#12603=EDGE_LOOP('',(#60318,#60319,#60320,#60321));
#12604=EDGE_LOOP('',(#60322,#60323,#60324,#60325,#60326,#60327,#60328,#60329,
#60330,#60331,#60332,#60333,#60334,#60335,#60336,#60337,#60338,#60339,#60340,
#60341,#60342,#60343,#60344,#60345,#60346,#60347,#60348,#60349,#60350,#60351,
#60352,#60353));
#12605=EDGE_LOOP('',(#60354));
#12606=EDGE_LOOP('',(#60355,#60356,#60357,#60358));
#12607=EDGE_LOOP('',(#60359,#60360,#60361,#60362));
#12608=EDGE_LOOP('',(#60363,#60364,#60365,#60366,#60367,#60368));
#12609=EDGE_LOOP('',(#60369,#60370,#60371,#60372));
#12610=EDGE_LOOP('',(#60373,#60374,#60375,#60376));
#12611=EDGE_LOOP('',(#60377,#60378,#60379,#60380));
#12612=EDGE_LOOP('',(#60381,#60382,#60383,#60384));
#12613=EDGE_LOOP('',(#60385,#60386,#60387,#60388));
#12614=EDGE_LOOP('',(#60389,#60390,#60391,#60392));
#12615=EDGE_LOOP('',(#60393,#60394,#60395,#60396));
#12616=EDGE_LOOP('',(#60397,#60398,#60399,#60400));
#12617=EDGE_LOOP('',(#60401,#60402,#60403,#60404));
#12618=EDGE_LOOP('',(#60405,#60406,#60407,#60408));
#12619=EDGE_LOOP('',(#60409,#60410,#60411,#60412));
#12620=EDGE_LOOP('',(#60413,#60414,#60415,#60416));
#12621=EDGE_LOOP('',(#60417,#60418,#60419,#60420,#60421,#60422));
#12622=EDGE_LOOP('',(#60423,#60424,#60425,#60426));
#12623=EDGE_LOOP('',(#60427,#60428,#60429,#60430));
#12624=EDGE_LOOP('',(#60431,#60432,#60433,#60434));
#12625=EDGE_LOOP('',(#60435,#60436,#60437,#60438));
#12626=EDGE_LOOP('',(#60439,#60440,#60441,#60442,#60443,#60444,#60445,#60446));
#12627=EDGE_LOOP('',(#60447,#60448,#60449,#60450));
#12628=EDGE_LOOP('',(#60451,#60452,#60453,#60454));
#12629=EDGE_LOOP('',(#60455,#60456,#60457,#60458));
#12630=EDGE_LOOP('',(#60459,#60460,#60461,#60462));
#12631=EDGE_LOOP('',(#60463,#60464,#60465,#60466,#60467,#60468));
#12632=EDGE_LOOP('',(#60469,#60470,#60471,#60472));
#12633=EDGE_LOOP('',(#60473,#60474,#60475,#60476));
#12634=EDGE_LOOP('',(#60477,#60478,#60479,#60480));
#12635=EDGE_LOOP('',(#60481,#60482,#60483,#60484));
#12636=EDGE_LOOP('',(#60485,#60486,#60487,#60488));
#12637=EDGE_LOOP('',(#60489,#60490,#60491,#60492));
#12638=EDGE_LOOP('',(#60493,#60494,#60495,#60496));
#12639=EDGE_LOOP('',(#60497,#60498,#60499,#60500,#60501,#60502));
#12640=EDGE_LOOP('',(#60503,#60504,#60505,#60506));
#12641=EDGE_LOOP('',(#60507,#60508,#60509,#60510,#60511,#60512));
#12642=EDGE_LOOP('',(#60513,#60514,#60515,#60516));
#12643=EDGE_LOOP('',(#60517,#60518,#60519,#60520,#60521,#60522,#60523,#60524));
#12644=EDGE_LOOP('',(#60525,#60526,#60527,#60528));
#12645=EDGE_LOOP('',(#60529,#60530,#60531,#60532,#60533));
#12646=EDGE_LOOP('',(#60534,#60535,#60536,#60537,#60538));
#12647=EDGE_LOOP('',(#60539));
#12648=EDGE_LOOP('',(#60540));
#12649=EDGE_LOOP('',(#60541,#60542,#60543,#60544));
#12650=EDGE_LOOP('',(#60545,#60546,#60547,#60548));
#12651=EDGE_LOOP('',(#60549,#60550,#60551,#60552,#60553,#60554,#60555,#60556,
#60557));
#12652=EDGE_LOOP('',(#60558,#60559,#60560,#60561,#60562,#60563));
#12653=EDGE_LOOP('',(#60564,#60565,#60566,#60567));
#12654=EDGE_LOOP('',(#60568,#60569,#60570,#60571));
#12655=EDGE_LOOP('',(#60572,#60573,#60574,#60575));
#12656=EDGE_LOOP('',(#60576,#60577,#60578,#60579));
#12657=EDGE_LOOP('',(#60580,#60581,#60582,#60583));
#12658=EDGE_LOOP('',(#60584,#60585,#60586,#60587));
#12659=EDGE_LOOP('',(#60588,#60589,#60590,#60591));
#12660=EDGE_LOOP('',(#60592,#60593,#60594,#60595));
#12661=EDGE_LOOP('',(#60596,#60597,#60598,#60599,#60600,#60601));
#12662=EDGE_LOOP('',(#60602,#60603,#60604,#60605));
#12663=EDGE_LOOP('',(#60606,#60607,#60608,#60609));
#12664=EDGE_LOOP('',(#60610,#60611,#60612,#60613));
#12665=EDGE_LOOP('',(#60614,#60615,#60616,#60617));
#12666=EDGE_LOOP('',(#60618,#60619,#60620,#60621));
#12667=EDGE_LOOP('',(#60622,#60623,#60624,#60625));
#12668=EDGE_LOOP('',(#60626,#60627,#60628,#60629));
#12669=EDGE_LOOP('',(#60630,#60631,#60632,#60633));
#12670=EDGE_LOOP('',(#60634,#60635,#60636,#60637));
#12671=EDGE_LOOP('',(#60638,#60639,#60640,#60641));
#12672=EDGE_LOOP('',(#60642,#60643,#60644,#60645));
#12673=EDGE_LOOP('',(#60646,#60647,#60648,#60649));
#12674=EDGE_LOOP('',(#60650,#60651,#60652,#60653,#60654,#60655));
#12675=EDGE_LOOP('',(#60656,#60657,#60658,#60659,#60660,#60661,#60662,#60663,
#60664,#60665,#60666,#60667,#60668,#60669,#60670,#60671,#60672));
#12676=EDGE_LOOP('',(#60673,#60674,#60675,#60676,#60677,#60678,#60679,#60680));
#12677=EDGE_LOOP('',(#60681));
#12678=EDGE_LOOP('',(#60682,#60683,#60684,#60685,#60686));
#12679=EDGE_LOOP('',(#60687,#60688,#60689,#60690));
#12680=EDGE_LOOP('',(#60691,#60692,#60693,#60694));
#12681=EDGE_LOOP('',(#60695,#60696,#60697,#60698));
#12682=EDGE_LOOP('',(#60699,#60700,#60701,#60702));
#12683=EDGE_LOOP('',(#60703,#60704,#60705,#60706));
#12684=EDGE_LOOP('',(#60707,#60708,#60709,#60710));
#12685=EDGE_LOOP('',(#60711,#60712,#60713,#60714,#60715,#60716));
#12686=EDGE_LOOP('',(#60717));
#12687=EDGE_LOOP('',(#60718,#60719,#60720,#60721));
#12688=EDGE_LOOP('',(#60722));
#12689=EDGE_LOOP('',(#60723));
#12690=EDGE_LOOP('',(#60724,#60725,#60726,#60727));
#12691=EDGE_LOOP('',(#60728,#60729,#60730,#60731));
#12692=EDGE_LOOP('',(#60732,#60733,#60734,#60735));
#12693=EDGE_LOOP('',(#60736,#60737,#60738,#60739));
#12694=EDGE_LOOP('',(#60740,#60741,#60742,#60743));
#12695=EDGE_LOOP('',(#60744,#60745,#60746,#60747));
#12696=EDGE_LOOP('',(#60748,#60749,#60750,#60751));
#12697=EDGE_LOOP('',(#60752,#60753,#60754,#60755));
#12698=EDGE_LOOP('',(#60756));
#12699=EDGE_LOOP('',(#60757,#60758,#60759,#60760));
#12700=EDGE_LOOP('',(#60761,#60762,#60763,#60764));
#12701=EDGE_LOOP('',(#60765,#60766,#60767,#60768));
#12702=EDGE_LOOP('',(#60769,#60770,#60771,#60772));
#12703=EDGE_LOOP('',(#60773,#60774,#60775,#60776));
#12704=EDGE_LOOP('',(#60777,#60778,#60779,#60780));
#12705=EDGE_LOOP('',(#60781,#60782,#60783,#60784));
#12706=EDGE_LOOP('',(#60785,#60786,#60787,#60788));
#12707=EDGE_LOOP('',(#60789,#60790,#60791,#60792,#60793,#60794,#60795,#60796,
#60797,#60798,#60799,#60800,#60801,#60802));
#12708=EDGE_LOOP('',(#60803,#60804,#60805,#60806));
#12709=EDGE_LOOP('',(#60807,#60808,#60809,#60810,#60811));
#12710=EDGE_LOOP('',(#60812,#60813,#60814,#60815));
#12711=EDGE_LOOP('',(#60816,#60817,#60818,#60819));
#12712=EDGE_LOOP('',(#60820,#60821,#60822,#60823));
#12713=EDGE_LOOP('',(#60824,#60825,#60826,#60827));
#12714=EDGE_LOOP('',(#60828,#60829,#60830,#60831,#60832,#60833,#60834,#60835));
#12715=EDGE_LOOP('',(#60836,#60837,#60838,#60839));
#12716=EDGE_LOOP('',(#60840,#60841,#60842,#60843));
#12717=EDGE_LOOP('',(#60844,#60845,#60846,#60847));
#12718=EDGE_LOOP('',(#60848,#60849,#60850,#60851,#60852,#60853));
#12719=EDGE_LOOP('',(#60854,#60855,#60856,#60857));
#12720=EDGE_LOOP('',(#60858,#60859,#60860));
#12721=EDGE_LOOP('',(#60861,#60862,#60863,#60864));
#12722=EDGE_LOOP('',(#60865,#60866,#60867));
#12723=EDGE_LOOP('',(#60868,#60869,#60870,#60871));
#12724=EDGE_LOOP('',(#60872,#60873,#60874,#60875));
#12725=EDGE_LOOP('',(#60876,#60877,#60878,#60879));
#12726=EDGE_LOOP('',(#60880,#60881,#60882,#60883,#60884,#60885,#60886,#60887,
#60888,#60889,#60890,#60891,#60892,#60893,#60894,#60895,#60896,#60897,#60898,
#60899));
#12727=EDGE_LOOP('',(#60900,#60901,#60902,#60903));
#12728=EDGE_LOOP('',(#60904,#60905,#60906,#60907));
#12729=EDGE_LOOP('',(#60908,#60909,#60910,#60911,#60912,#60913));
#12730=EDGE_LOOP('',(#60914,#60915,#60916,#60917));
#12731=EDGE_LOOP('',(#60918,#60919,#60920,#60921));
#12732=EDGE_LOOP('',(#60922,#60923,#60924,#60925));
#12733=EDGE_LOOP('',(#60926,#60927,#60928,#60929));
#12734=EDGE_LOOP('',(#60930,#60931,#60932,#60933));
#12735=EDGE_LOOP('',(#60934,#60935,#60936,#60937));
#12736=EDGE_LOOP('',(#60938,#60939,#60940,#60941));
#12737=EDGE_LOOP('',(#60942,#60943,#60944,#60945));
#12738=EDGE_LOOP('',(#60946,#60947,#60948,#60949));
#12739=EDGE_LOOP('',(#60950,#60951,#60952,#60953));
#12740=EDGE_LOOP('',(#60954,#60955,#60956,#60957));
#12741=EDGE_LOOP('',(#60958,#60959,#60960,#60961,#60962,#60963));
#12742=EDGE_LOOP('',(#60964,#60965,#60966,#60967,#60968,#60969,#60970,#60971));
#12743=EDGE_LOOP('',(#60972,#60973,#60974,#60975));
#12744=EDGE_LOOP('',(#60976,#60977,#60978,#60979));
#12745=EDGE_LOOP('',(#60980,#60981,#60982,#60983));
#12746=EDGE_LOOP('',(#60984,#60985,#60986,#60987));
#12747=EDGE_LOOP('',(#60988,#60989,#60990,#60991));
#12748=EDGE_LOOP('',(#60992,#60993,#60994,#60995));
#12749=EDGE_LOOP('',(#60996,#60997,#60998,#60999));
#12750=EDGE_LOOP('',(#61000,#61001,#61002,#61003));
#12751=EDGE_LOOP('',(#61004,#61005,#61006,#61007));
#12752=EDGE_LOOP('',(#61008,#61009,#61010,#61011));
#12753=EDGE_LOOP('',(#61012,#61013,#61014,#61015));
#12754=EDGE_LOOP('',(#61016,#61017,#61018,#61019));
#12755=EDGE_LOOP('',(#61020,#61021,#61022,#61023,#61024,#61025,#61026,#61027));
#12756=EDGE_LOOP('',(#61028,#61029,#61030,#61031,#61032));
#12757=EDGE_LOOP('',(#61033,#61034,#61035,#61036));
#12758=EDGE_LOOP('',(#61037,#61038,#61039,#61040,#61041,#61042,#61043));
#12759=EDGE_LOOP('',(#61044,#61045,#61046,#61047,#61048,#61049,#61050,#61051,
#61052,#61053,#61054,#61055,#61056));
#12760=EDGE_LOOP('',(#61057,#61058,#61059,#61060));
#12761=EDGE_LOOP('',(#61061,#61062,#61063,#61064,#61065,#61066,#61067));
#12762=EDGE_LOOP('',(#61068,#61069,#61070,#61071));
#12763=EDGE_LOOP('',(#61072,#61073,#61074,#61075,#61076));
#12764=EDGE_LOOP('',(#61077,#61078,#61079,#61080,#61081,#61082,#61083,#61084,
#61085,#61086));
#12765=EDGE_LOOP('',(#61087,#61088,#61089,#61090));
#12766=EDGE_LOOP('',(#61091,#61092,#61093,#61094));
#12767=EDGE_LOOP('',(#61095,#61096,#61097,#61098,#61099,#61100,#61101));
#12768=EDGE_LOOP('',(#61102));
#12769=EDGE_LOOP('',(#61103,#61104,#61105,#61106));
#12770=EDGE_LOOP('',(#61107,#61108,#61109,#61110,#61111,#61112,#61113,#61114,
#61115,#61116,#61117,#61118,#61119,#61120,#61121,#61122));
#12771=EDGE_LOOP('',(#61123,#61124,#61125,#61126,#61127));
#12772=EDGE_LOOP('',(#61128,#61129,#61130,#61131,#61132));
#12773=EDGE_LOOP('',(#61133,#61134,#61135,#61136));
#12774=EDGE_LOOP('',(#61137,#61138,#61139,#61140));
#12775=EDGE_LOOP('',(#61141,#61142,#61143,#61144));
#12776=EDGE_LOOP('',(#61145,#61146,#61147,#61148));
#12777=EDGE_LOOP('',(#61149,#61150,#61151,#61152));
#12778=EDGE_LOOP('',(#61153,#61154,#61155,#61156));
#12779=EDGE_LOOP('',(#61157,#61158,#61159,#61160));
#12780=EDGE_LOOP('',(#61161,#61162,#61163,#61164));
#12781=EDGE_LOOP('',(#61165,#61166,#61167,#61168,#61169,#61170));
#12782=EDGE_LOOP('',(#61171,#61172,#61173,#61174,#61175,#61176,#61177));
#12783=EDGE_LOOP('',(#61178,#61179,#61180,#61181));
#12784=EDGE_LOOP('',(#61182,#61183,#61184,#61185,#61186,#61187));
#12785=EDGE_LOOP('',(#61188,#61189,#61190,#61191,#61192,#61193,#61194,#61195));
#12786=EDGE_LOOP('',(#61196,#61197,#61198));
#12787=EDGE_LOOP('',(#61199,#61200,#61201,#61202));
#12788=EDGE_LOOP('',(#61203,#61204,#61205,#61206,#61207));
#12789=EDGE_LOOP('',(#61208,#61209,#61210,#61211,#61212,#61213,#61214,#61215,
#61216));
#12790=EDGE_LOOP('',(#61217,#61218,#61219,#61220));
#12791=EDGE_LOOP('',(#61221,#61222,#61223,#61224));
#12792=EDGE_LOOP('',(#61225,#61226,#61227,#61228));
#12793=EDGE_LOOP('',(#61229,#61230,#61231,#61232));
#12794=EDGE_LOOP('',(#61233,#61234,#61235,#61236));
#12795=EDGE_LOOP('',(#61237,#61238,#61239,#61240));
#12796=EDGE_LOOP('',(#61241,#61242,#61243,#61244));
#12797=EDGE_LOOP('',(#61245,#61246,#61247,#61248,#61249,#61250));
#12798=EDGE_LOOP('',(#61251,#61252,#61253,#61254));
#12799=EDGE_LOOP('',(#61255,#61256,#61257,#61258));
#12800=EDGE_LOOP('',(#61259,#61260,#61261,#61262));
#12801=EDGE_LOOP('',(#61263,#61264,#61265,#61266));
#12802=EDGE_LOOP('',(#61267,#61268,#61269,#61270));
#12803=EDGE_LOOP('',(#61271,#61272,#61273,#61274));
#12804=EDGE_LOOP('',(#61275,#61276,#61277,#61278));
#12805=EDGE_LOOP('',(#61279,#61280,#61281,#61282));
#12806=EDGE_LOOP('',(#61283,#61284,#61285,#61286,#61287,#61288,#61289,#61290,
#61291,#61292,#61293,#61294,#61295,#61296,#61297));
#12807=EDGE_LOOP('',(#61298,#61299,#61300));
#12808=EDGE_LOOP('',(#61301,#61302,#61303,#61304));
#12809=EDGE_LOOP('',(#61305,#61306,#61307,#61308));
#12810=EDGE_LOOP('',(#61309,#61310,#61311,#61312));
#12811=EDGE_LOOP('',(#61313,#61314,#61315,#61316));
#12812=EDGE_LOOP('',(#61317,#61318,#61319,#61320));
#12813=EDGE_LOOP('',(#61321,#61322,#61323,#61324));
#12814=EDGE_LOOP('',(#61325,#61326,#61327,#61328));
#12815=EDGE_LOOP('',(#61329,#61330,#61331,#61332));
#12816=EDGE_LOOP('',(#61333,#61334,#61335,#61336));
#12817=EDGE_LOOP('',(#61337,#61338,#61339,#61340));
#12818=EDGE_LOOP('',(#61341,#61342,#61343,#61344));
#12819=EDGE_LOOP('',(#61345,#61346,#61347));
#12820=EDGE_LOOP('',(#61348,#61349,#61350,#61351));
#12821=EDGE_LOOP('',(#61352,#61353,#61354,#61355));
#12822=EDGE_LOOP('',(#61356,#61357,#61358,#61359));
#12823=EDGE_LOOP('',(#61360,#61361,#61362,#61363));
#12824=EDGE_LOOP('',(#61364,#61365,#61366,#61367));
#12825=EDGE_LOOP('',(#61368,#61369,#61370,#61371));
#12826=EDGE_LOOP('',(#61372,#61373,#61374,#61375,#61376,#61377,#61378,#61379,
#61380,#61381,#61382));
#12827=EDGE_LOOP('',(#61383,#61384,#61385,#61386));
#12828=EDGE_LOOP('',(#61387,#61388,#61389,#61390));
#12829=EDGE_LOOP('',(#61391,#61392,#61393,#61394));
#12830=EDGE_LOOP('',(#61395,#61396,#61397,#61398));
#12831=EDGE_LOOP('',(#61399,#61400,#61401,#61402));
#12832=EDGE_LOOP('',(#61403,#61404,#61405,#61406));
#12833=EDGE_LOOP('',(#61407,#61408,#61409,#61410));
#12834=EDGE_LOOP('',(#61411,#61412,#61413,#61414));
#12835=EDGE_LOOP('',(#61415,#61416,#61417,#61418));
#12836=EDGE_LOOP('',(#61419,#61420,#61421,#61422));
#12837=EDGE_LOOP('',(#61423,#61424,#61425,#61426));
#12838=EDGE_LOOP('',(#61427,#61428,#61429,#61430));
#12839=EDGE_LOOP('',(#61431,#61432,#61433,#61434));
#12840=EDGE_LOOP('',(#61435,#61436,#61437,#61438));
#12841=EDGE_LOOP('',(#61439,#61440,#61441,#61442));
#12842=EDGE_LOOP('',(#61443,#61444,#61445,#61446));
#12843=EDGE_LOOP('',(#61447,#61448,#61449,#61450));
#12844=EDGE_LOOP('',(#61451,#61452,#61453,#61454));
#12845=EDGE_LOOP('',(#61455,#61456,#61457,#61458,#61459,#61460,#61461,#61462,
#61463,#61464,#61465,#61466));
#12846=EDGE_LOOP('',(#61467,#61468,#61469,#61470));
#12847=EDGE_LOOP('',(#61471,#61472,#61473,#61474));
#12848=EDGE_LOOP('',(#61475,#61476,#61477,#61478));
#12849=EDGE_LOOP('',(#61479,#61480,#61481,#61482));
#12850=EDGE_LOOP('',(#61483,#61484,#61485,#61486));
#12851=EDGE_LOOP('',(#61487,#61488,#61489,#61490));
#12852=EDGE_LOOP('',(#61491,#61492,#61493,#61494));
#12853=EDGE_LOOP('',(#61495,#61496,#61497,#61498));
#12854=EDGE_LOOP('',(#61499,#61500,#61501,#61502));
#12855=EDGE_LOOP('',(#61503,#61504,#61505,#61506));
#12856=EDGE_LOOP('',(#61507,#61508,#61509,#61510));
#12857=EDGE_LOOP('',(#61511,#61512,#61513,#61514));
#12858=EDGE_LOOP('',(#61515,#61516,#61517,#61518));
#12859=EDGE_LOOP('',(#61519,#61520,#61521,#61522,#61523,#61524));
#12860=EDGE_LOOP('',(#61525,#61526,#61527,#61528,#61529,#61530,#61531,#61532,
#61533,#61534,#61535));
#12861=EDGE_LOOP('',(#61536,#61537,#61538,#61539));
#12862=EDGE_LOOP('',(#61540,#61541,#61542,#61543));
#12863=EDGE_LOOP('',(#61544,#61545,#61546,#61547,#61548,#61549,#61550,#61551,
#61552,#61553,#61554));
#12864=EDGE_LOOP('',(#61555,#61556,#61557,#61558));
#12865=EDGE_LOOP('',(#61559,#61560,#61561,#61562));
#12866=EDGE_LOOP('',(#61563,#61564,#61565,#61566));
#12867=EDGE_LOOP('',(#61567,#61568,#61569,#61570));
#12868=EDGE_LOOP('',(#61571,#61572,#61573,#61574));
#12869=EDGE_LOOP('',(#61575,#61576,#61577,#61578,#61579,#61580));
#12870=EDGE_LOOP('',(#61581,#61582,#61583,#61584));
#12871=EDGE_LOOP('',(#61585,#61586,#61587,#61588,#61589,#61590,#61591,#61592,
#61593,#61594));
#12872=EDGE_LOOP('',(#61595,#61596,#61597,#61598));
#12873=EDGE_LOOP('',(#61599,#61600,#61601,#61602,#61603,#61604));
#12874=EDGE_LOOP('',(#61605,#61606,#61607,#61608,#61609,#61610,#61611,#61612,
#61613,#61614,#61615,#61616,#61617,#61618));
#12875=EDGE_LOOP('',(#61619,#61620,#61621,#61622));
#12876=EDGE_LOOP('',(#61623,#61624,#61625,#61626));
#12877=EDGE_LOOP('',(#61627,#61628,#61629,#61630));
#12878=EDGE_LOOP('',(#61631,#61632,#61633,#61634));
#12879=EDGE_LOOP('',(#61635,#61636,#61637,#61638));
#12880=EDGE_LOOP('',(#61639,#61640,#61641,#61642));
#12881=EDGE_LOOP('',(#61643,#61644,#61645,#61646));
#12882=EDGE_LOOP('',(#61647,#61648,#61649,#61650));
#12883=EDGE_LOOP('',(#61651,#61652,#61653,#61654,#61655));
#12884=EDGE_LOOP('',(#61656,#61657,#61658,#61659));
#12885=EDGE_LOOP('',(#61660,#61661,#61662,#61663));
#12886=EDGE_LOOP('',(#61664,#61665,#61666,#61667));
#12887=EDGE_LOOP('',(#61668,#61669,#61670,#61671));
#12888=EDGE_LOOP('',(#61672,#61673,#61674,#61675,#61676,#61677,#61678,#61679,
#61680,#61681,#61682,#61683,#61684,#61685,#61686,#61687));
#12889=EDGE_LOOP('',(#61688,#61689,#61690,#61691));
#12890=EDGE_LOOP('',(#61692,#61693,#61694,#61695));
#12891=EDGE_LOOP('',(#61696,#61697,#61698,#61699));
#12892=EDGE_LOOP('',(#61700,#61701,#61702,#61703));
#12893=EDGE_LOOP('',(#61704,#61705,#61706,#61707,#61708,#61709,#61710,#61711,
#61712,#61713,#61714,#61715));
#12894=EDGE_LOOP('',(#61716,#61717,#61718,#61719));
#12895=EDGE_LOOP('',(#61720,#61721,#61722,#61723));
#12896=EDGE_LOOP('',(#61724,#61725,#61726,#61727));
#12897=EDGE_LOOP('',(#61728,#61729,#61730,#61731));
#12898=EDGE_LOOP('',(#61732,#61733,#61734,#61735));
#12899=EDGE_LOOP('',(#61736,#61737,#61738,#61739));
#12900=EDGE_LOOP('',(#61740,#61741,#61742,#61743));
#12901=EDGE_LOOP('',(#61744,#61745,#61746,#61747));
#12902=EDGE_LOOP('',(#61748,#61749,#61750,#61751));
#12903=EDGE_LOOP('',(#61752,#61753,#61754,#61755));
#12904=EDGE_LOOP('',(#61756,#61757,#61758,#61759));
#12905=EDGE_LOOP('',(#61760,#61761,#61762,#61763,#61764,#61765));
#12906=EDGE_LOOP('',(#61766,#61767,#61768,#61769));
#12907=EDGE_LOOP('',(#61770,#61771,#61772,#61773));
#12908=EDGE_LOOP('',(#61774,#61775));
#12909=EDGE_LOOP('',(#61776,#61777,#61778,#61779,#61780,#61781,#61782,#61783,
#61784,#61785,#61786,#61787,#61788,#61789,#61790,#61791,#61792,#61793,#61794,
#61795,#61796,#61797,#61798,#61799));
#12910=EDGE_LOOP('',(#61800,#61801,#61802,#61803,#61804,#61805,#61806,#61807,
#61808,#61809,#61810,#61811));
#12911=EDGE_LOOP('',(#61812,#61813,#61814,#61815));
#12912=EDGE_LOOP('',(#61816,#61817,#61818,#61819));
#12913=EDGE_LOOP('',(#61820,#61821,#61822,#61823));
#12914=EDGE_LOOP('',(#61824,#61825,#61826,#61827));
#12915=EDGE_LOOP('',(#61828,#61829,#61830,#61831));
#12916=EDGE_LOOP('',(#61832,#61833,#61834,#61835));
#12917=EDGE_LOOP('',(#61836,#61837,#61838,#61839));
#12918=EDGE_LOOP('',(#61840,#61841,#61842,#61843));
#12919=EDGE_LOOP('',(#61844,#61845,#61846,#61847));
#12920=EDGE_LOOP('',(#61848,#61849,#61850,#61851));
#12921=EDGE_LOOP('',(#61852,#61853,#61854,#61855));
#12922=EDGE_LOOP('',(#61856,#61857,#61858,#61859));
#12923=EDGE_LOOP('',(#61860,#61861,#61862,#61863));
#12924=EDGE_LOOP('',(#61864,#61865,#61866,#61867));
#12925=EDGE_LOOP('',(#61868,#61869,#61870,#61871,#61872,#61873,#61874,#61875,
#61876,#61877,#61878,#61879,#61880,#61881,#61882));
#12926=EDGE_LOOP('',(#61883,#61884,#61885,#61886,#61887,#61888,#61889,#61890,
#61891,#61892));
#12927=EDGE_LOOP('',(#61893,#61894,#61895,#61896));
#12928=EDGE_LOOP('',(#61897,#61898,#61899,#61900));
#12929=EDGE_LOOP('',(#61901,#61902,#61903,#61904));
#12930=EDGE_LOOP('',(#61905,#61906,#61907,#61908));
#12931=EDGE_LOOP('',(#61909,#61910,#61911,#61912));
#12932=EDGE_LOOP('',(#61913,#61914,#61915,#61916));
#12933=EDGE_LOOP('',(#61917,#61918,#61919,#61920,#61921,#61922,#61923,#61924));
#12934=EDGE_LOOP('',(#61925,#61926,#61927,#61928));
#12935=EDGE_LOOP('',(#61929,#61930,#61931,#61932));
#12936=EDGE_LOOP('',(#61933,#61934,#61935,#61936));
#12937=EDGE_LOOP('',(#61937,#61938,#61939,#61940));
#12938=EDGE_LOOP('',(#61941,#61942,#61943,#61944));
#12939=EDGE_LOOP('',(#61945,#61946,#61947,#61948));
#12940=EDGE_LOOP('',(#61949,#61950,#61951,#61952));
#12941=EDGE_LOOP('',(#61953,#61954,#61955,#61956));
#12942=EDGE_LOOP('',(#61957));
#12943=EDGE_LOOP('',(#61958));
#12944=EDGE_LOOP('',(#61959,#61960,#61961,#61962));
#12945=EDGE_LOOP('',(#61963,#61964,#61965,#61966));
#12946=EDGE_LOOP('',(#61967,#61968,#61969,#61970,#61971,#61972,#61973,#61974,
#61975,#61976));
#12947=EDGE_LOOP('',(#61977,#61978,#61979,#61980));
#12948=EDGE_LOOP('',(#61981,#61982,#61983,#61984));
#12949=EDGE_LOOP('',(#61985,#61986,#61987,#61988));
#12950=EDGE_LOOP('',(#61989,#61990,#61991,#61992));
#12951=EDGE_LOOP('',(#61993,#61994,#61995,#61996));
#12952=EDGE_LOOP('',(#61997,#61998,#61999,#62000));
#12953=EDGE_LOOP('',(#62001,#62002,#62003,#62004));
#12954=EDGE_LOOP('',(#62005,#62006,#62007,#62008));
#12955=EDGE_LOOP('',(#62009,#62010,#62011,#62012));
#12956=EDGE_LOOP('',(#62013,#62014,#62015,#62016));
#12957=EDGE_LOOP('',(#62017,#62018,#62019,#62020));
#12958=EDGE_LOOP('',(#62021,#62022,#62023,#62024));
#12959=EDGE_LOOP('',(#62025,#62026,#62027,#62028));
#12960=EDGE_LOOP('',(#62029,#62030,#62031,#62032));
#12961=EDGE_LOOP('',(#62033,#62034,#62035,#62036));
#12962=EDGE_LOOP('',(#62037,#62038,#62039,#62040));
#12963=EDGE_LOOP('',(#62041,#62042,#62043,#62044));
#12964=EDGE_LOOP('',(#62045,#62046));
#12965=EDGE_LOOP('',(#62047));
#12966=EDGE_LOOP('',(#62048,#62049,#62050,#62051));
#12967=EDGE_LOOP('',(#62052,#62053,#62054,#62055));
#12968=EDGE_LOOP('',(#62056,#62057));
#12969=EDGE_LOOP('',(#62058));
#12970=EDGE_LOOP('',(#62059,#62060,#62061,#62062));
#12971=EDGE_LOOP('',(#62063,#62064,#62065,#62066));
#12972=EDGE_LOOP('',(#62067,#62068,#62069,#62070,#62071,#62072));
#12973=EDGE_LOOP('',(#62073,#62074,#62075,#62076,#62077,#62078));
#12974=EDGE_LOOP('',(#62079,#62080,#62081,#62082));
#12975=EDGE_LOOP('',(#62083,#62084,#62085,#62086,#62087));
#12976=EDGE_LOOP('',(#62088,#62089,#62090,#62091));
#12977=EDGE_LOOP('',(#62092,#62093,#62094,#62095));
#12978=EDGE_LOOP('',(#62096,#62097,#62098,#62099,#62100));
#12979=EDGE_LOOP('',(#62101,#62102,#62103,#62104));
#12980=EDGE_LOOP('',(#62105,#62106,#62107,#62108,#62109));
#12981=EDGE_LOOP('',(#62110,#62111,#62112,#62113));
#12982=EDGE_LOOP('',(#62114,#62115,#62116,#62117,#62118));
#12983=EDGE_LOOP('',(#62119,#62120,#62121,#62122));
#12984=EDGE_LOOP('',(#62123,#62124,#62125,#62126));
#12985=EDGE_LOOP('',(#62127,#62128,#62129,#62130));
#12986=EDGE_LOOP('',(#62131,#62132,#62133,#62134));
#12987=EDGE_LOOP('',(#62135,#62136,#62137,#62138,#62139,#62140));
#12988=EDGE_LOOP('',(#62141,#62142,#62143,#62144));
#12989=EDGE_LOOP('',(#62145,#62146,#62147,#62148));
#12990=EDGE_LOOP('',(#62149,#62150,#62151,#62152));
#12991=EDGE_LOOP('',(#62153,#62154,#62155,#62156,#62157,#62158));
#12992=EDGE_LOOP('',(#62159,#62160,#62161,#62162));
#12993=EDGE_LOOP('',(#62163,#62164,#62165,#62166));
#12994=EDGE_LOOP('',(#62167,#62168,#62169,#62170,#62171,#62172));
#12995=EDGE_LOOP('',(#62173,#62174,#62175,#62176));
#12996=EDGE_LOOP('',(#62177,#62178,#62179,#62180));
#12997=EDGE_LOOP('',(#62181,#62182,#62183,#62184));
#12998=EDGE_LOOP('',(#62185,#62186,#62187,#62188));
#12999=EDGE_LOOP('',(#62189,#62190,#62191,#62192));
#13000=EDGE_LOOP('',(#62193,#62194,#62195,#62196,#62197,#62198));
#13001=EDGE_LOOP('',(#62199));
#13002=EDGE_LOOP('',(#62200));
#13003=EDGE_LOOP('',(#62201,#62202,#62203,#62204));
#13004=EDGE_LOOP('',(#62205,#62206,#62207,#62208,#62209));
#13005=EDGE_LOOP('',(#62210,#62211,#62212,#62213));
#13006=EDGE_LOOP('',(#62214,#62215,#62216,#62217));
#13007=EDGE_LOOP('',(#62218,#62219,#62220,#62221,#62222,#62223,#62224,#62225));
#13008=EDGE_LOOP('',(#62226,#62227,#62228,#62229,#62230,#62231));
#13009=EDGE_LOOP('',(#62232,#62233,#62234,#62235,#62236,#62237));
#13010=EDGE_LOOP('',(#62238,#62239,#62240,#62241));
#13011=EDGE_LOOP('',(#62242,#62243,#62244,#62245));
#13012=EDGE_LOOP('',(#62246,#62247,#62248,#62249));
#13013=EDGE_LOOP('',(#62250,#62251,#62252,#62253,#62254,#62255));
#13014=EDGE_LOOP('',(#62256,#62257,#62258,#62259));
#13015=EDGE_LOOP('',(#62260,#62261,#62262,#62263,#62264));
#13016=EDGE_LOOP('',(#62265,#62266,#62267,#62268));
#13017=EDGE_LOOP('',(#62269,#62270,#62271,#62272,#62273,#62274,#62275,#62276,
#62277,#62278,#62279,#62280));
#13018=EDGE_LOOP('',(#62281,#62282,#62283,#62284));
#13019=EDGE_LOOP('',(#62285,#62286,#62287,#62288));
#13020=EDGE_LOOP('',(#62289,#62290,#62291,#62292,#62293,#62294,#62295,#62296,
#62297,#62298));
#13021=EDGE_LOOP('',(#62299,#62300,#62301,#62302));
#13022=EDGE_LOOP('',(#62303,#62304,#62305,#62306,#62307,#62308,#62309,#62310,
#62311,#62312));
#13023=EDGE_LOOP('',(#62313,#62314,#62315,#62316));
#13024=EDGE_LOOP('',(#62317,#62318,#62319,#62320));
#13025=EDGE_LOOP('',(#62321,#62322,#62323,#62324));
#13026=EDGE_LOOP('',(#62325,#62326,#62327,#62328,#62329,#62330,#62331,#62332,
#62333,#62334,#62335,#62336,#62337,#62338,#62339,#62340,#62341,#62342,#62343,
#62344,#62345,#62346,#62347,#62348,#62349,#62350,#62351,#62352,#62353,#62354,
#62355,#62356,#62357,#62358,#62359,#62360,#62361,#62362,#62363,#62364,#62365,
#62366,#62367,#62368,#62369,#62370,#62371));
#13027=EDGE_LOOP('',(#62372));
#13028=EDGE_LOOP('',(#62373,#62374,#62375,#62376,#62377,#62378,#62379,#62380,
#62381,#62382,#62383,#62384,#62385,#62386));
#13029=EDGE_LOOP('',(#62387));
#13030=EDGE_LOOP('',(#62388));
#13031=EDGE_LOOP('',(#62389));
#13032=EDGE_LOOP('',(#62390,#62391,#62392,#62393));
#13033=EDGE_LOOP('',(#62394,#62395,#62396,#62397));
#13034=EDGE_LOOP('',(#62398,#62399,#62400,#62401,#62402,#62403,#62404));
#13035=EDGE_LOOP('',(#62405,#62406,#62407,#62408,#62409));
#13036=EDGE_LOOP('',(#62410,#62411,#62412,#62413));
#13037=EDGE_LOOP('',(#62414,#62415,#62416,#62417,#62418));
#13038=EDGE_LOOP('',(#62419,#62420,#62421,#62422,#62423));
#13039=EDGE_LOOP('',(#62424,#62425,#62426,#62427));
#13040=EDGE_LOOP('',(#62428,#62429,#62430,#62431,#62432,#62433,#62434));
#13041=EDGE_LOOP('',(#62435,#62436,#62437,#62438));
#13042=EDGE_LOOP('',(#62439,#62440,#62441,#62442,#62443,#62444));
#13043=EDGE_LOOP('',(#62445,#62446,#62447,#62448));
#13044=EDGE_LOOP('',(#62449));
#13045=EDGE_LOOP('',(#62450));
#13046=EDGE_LOOP('',(#62451,#62452,#62453,#62454));
#13047=EDGE_LOOP('',(#62455,#62456,#62457,#62458));
#13048=EDGE_LOOP('',(#62459,#62460,#62461,#62462));
#13049=EDGE_LOOP('',(#62463,#62464,#62465,#62466));
#13050=EDGE_LOOP('',(#62467,#62468,#62469,#62470));
#13051=EDGE_LOOP('',(#62471,#62472,#62473,#62474));
#13052=EDGE_LOOP('',(#62475,#62476,#62477,#62478));
#13053=EDGE_LOOP('',(#62479,#62480,#62481,#62482));
#13054=EDGE_LOOP('',(#62483,#62484,#62485,#62486));
#13055=EDGE_LOOP('',(#62487,#62488,#62489,#62490));
#13056=EDGE_LOOP('',(#62491,#62492,#62493,#62494));
#13057=EDGE_LOOP('',(#62495,#62496,#62497,#62498));
#13058=EDGE_LOOP('',(#62499,#62500,#62501,#62502));
#13059=EDGE_LOOP('',(#62503,#62504,#62505,#62506));
#13060=EDGE_LOOP('',(#62507,#62508,#62509,#62510,#62511,#62512,#62513));
#13061=EDGE_LOOP('',(#62514,#62515,#62516,#62517));
#13062=EDGE_LOOP('',(#62518,#62519,#62520,#62521));
#13063=EDGE_LOOP('',(#62522,#62523,#62524,#62525,#62526,#62527));
#13064=EDGE_LOOP('',(#62528,#62529,#62530,#62531));
#13065=EDGE_LOOP('',(#62532,#62533,#62534));
#13066=EDGE_LOOP('',(#62535,#62536,#62537,#62538,#62539));
#13067=EDGE_LOOP('',(#62540,#62541,#62542,#62543));
#13068=EDGE_LOOP('',(#62544));
#13069=EDGE_LOOP('',(#62545));
#13070=EDGE_LOOP('',(#62546));
#13071=EDGE_LOOP('',(#62547));
#13072=EDGE_LOOP('',(#62548,#62549,#62550,#62551));
#13073=EDGE_LOOP('',(#62552,#62553,#62554,#62555));
#13074=EDGE_LOOP('',(#62556));
#13075=EDGE_LOOP('',(#62557));
#13076=EDGE_LOOP('',(#62558,#62559,#62560,#62561,#62562));
#13077=EDGE_LOOP('',(#62563,#62564,#62565,#62566));
#13078=EDGE_LOOP('',(#62567,#62568,#62569,#62570));
#13079=EDGE_LOOP('',(#62571));
#13080=EDGE_LOOP('',(#62572));
#13081=EDGE_LOOP('',(#62573,#62574,#62575,#62576));
#13082=EDGE_LOOP('',(#62577));
#13083=EDGE_LOOP('',(#62578));
#13084=EDGE_LOOP('',(#62579,#62580,#62581,#62582,#62583));
#13085=EDGE_LOOP('',(#62584,#62585,#62586,#62587));
#13086=EDGE_LOOP('',(#62588,#62589,#62590,#62591,#62592,#62593,#62594));
#13087=EDGE_LOOP('',(#62595,#62596,#62597,#62598,#62599,#62600));
#13088=EDGE_LOOP('',(#62601));
#13089=EDGE_LOOP('',(#62602));
#13090=EDGE_LOOP('',(#62603,#62604,#62605,#62606));
#13091=EDGE_LOOP('',(#62607,#62608,#62609,#62610,#62611,#62612,#62613,#62614));
#13092=EDGE_LOOP('',(#62615,#62616,#62617,#62618,#62619,#62620,#62621,#62622));
#13093=EDGE_LOOP('',(#62623,#62624,#62625));
#13094=EDGE_LOOP('',(#62626,#62627,#62628,#62629));
#13095=EDGE_LOOP('',(#62630,#62631,#62632,#62633));
#13096=EDGE_LOOP('',(#62634,#62635,#62636,#62637));
#13097=EDGE_LOOP('',(#62638,#62639,#62640,#62641,#62642));
#13098=EDGE_LOOP('',(#62643,#62644,#62645,#62646));
#13099=EDGE_LOOP('',(#62647,#62648,#62649,#62650));
#13100=EDGE_LOOP('',(#62651,#62652,#62653,#62654));
#13101=EDGE_LOOP('',(#62655,#62656,#62657,#62658));
#13102=EDGE_LOOP('',(#62659,#62660,#62661,#62662,#62663,#62664,#62665,#62666,
#62667));
#13103=EDGE_LOOP('',(#62668,#62669,#62670,#62671));
#13104=EDGE_LOOP('',(#62672,#62673,#62674));
#13105=EDGE_LOOP('',(#62675,#62676,#62677,#62678));
#13106=EDGE_LOOP('',(#62679,#62680,#62681));
#13107=EDGE_LOOP('',(#62682,#62683,#62684,#62685));
#13108=EDGE_LOOP('',(#62686,#62687,#62688,#62689));
#13109=EDGE_LOOP('',(#62690,#62691,#62692,#62693));
#13110=EDGE_LOOP('',(#62694,#62695,#62696,#62697));
#13111=EDGE_LOOP('',(#62698,#62699,#62700,#62701,#62702,#62703,#62704,#62705,
#62706));
#13112=EDGE_LOOP('',(#62707,#62708,#62709,#62710));
#13113=EDGE_LOOP('',(#62711,#62712,#62713,#62714,#62715,#62716,#62717,#62718));
#13114=EDGE_LOOP('',(#62719,#62720,#62721,#62722,#62723,#62724,#62725,#62726,
#62727,#62728,#62729,#62730,#62731));
#13115=EDGE_LOOP('',(#62732,#62733,#62734,#62735));
#13116=EDGE_LOOP('',(#62736,#62737,#62738,#62739));
#13117=EDGE_LOOP('',(#62740,#62741,#62742,#62743));
#13118=EDGE_LOOP('',(#62744,#62745,#62746,#62747));
#13119=EDGE_LOOP('',(#62748,#62749,#62750,#62751));
#13120=EDGE_LOOP('',(#62752,#62753,#62754,#62755));
#13121=EDGE_LOOP('',(#62756,#62757,#62758,#62759));
#13122=EDGE_LOOP('',(#62760,#62761,#62762,#62763,#62764,#62765));
#13123=EDGE_LOOP('',(#62766));
#13124=EDGE_LOOP('',(#62767,#62768,#62769,#62770));
#13125=EDGE_LOOP('',(#62771,#62772,#62773,#62774));
#13126=EDGE_LOOP('',(#62775,#62776,#62777,#62778));
#13127=EDGE_LOOP('',(#62779,#62780,#62781,#62782));
#13128=EDGE_LOOP('',(#62783,#62784,#62785,#62786,#62787,#62788,#62789));
#13129=EDGE_LOOP('',(#62790,#62791,#62792,#62793,#62794,#62795,#62796,#62797,
#62798,#62799,#62800,#62801,#62802,#62803,#62804,#62805,#62806,#62807,#62808,
#62809,#62810,#62811,#62812));
#13130=EDGE_LOOP('',(#62813));
#13131=EDGE_LOOP('',(#62814,#62815,#62816,#62817));
#13132=EDGE_LOOP('',(#62818,#62819,#62820,#62821));
#13133=EDGE_LOOP('',(#62822,#62823,#62824,#62825));
#13134=EDGE_LOOP('',(#62826,#62827,#62828,#62829));
#13135=EDGE_LOOP('',(#62830,#62831,#62832,#62833));
#13136=EDGE_LOOP('',(#62834,#62835,#62836,#62837));
#13137=EDGE_LOOP('',(#62838,#62839,#62840,#62841,#62842,#62843,#62844,#62845));
#13138=EDGE_LOOP('',(#62846,#62847,#62848,#62849));
#13139=EDGE_LOOP('',(#62850,#62851,#62852,#62853));
#13140=EDGE_LOOP('',(#62854,#62855,#62856,#62857));
#13141=EDGE_LOOP('',(#62858,#62859,#62860,#62861,#62862,#62863,#62864,#62865,
#62866,#62867,#62868,#62869,#62870,#62871,#62872,#62873,#62874,#62875,#62876));
#13142=EDGE_LOOP('',(#62877,#62878,#62879,#62880));
#13143=EDGE_LOOP('',(#62881,#62882,#62883,#62884));
#13144=EDGE_LOOP('',(#62885,#62886,#62887,#62888));
#13145=EDGE_LOOP('',(#62889,#62890,#62891,#62892));
#13146=EDGE_LOOP('',(#62893,#62894,#62895,#62896,#62897,#62898,#62899,#62900,
#62901,#62902,#62903,#62904,#62905,#62906,#62907,#62908,#62909,#62910,#62911,
#62912,#62913,#62914,#62915,#62916,#62917,#62918,#62919,#62920,#62921,#62922,
#62923,#62924,#62925,#62926,#62927,#62928));
#13147=EDGE_LOOP('',(#62929));
#13148=EDGE_LOOP('',(#62930,#62931,#62932,#62933));
#13149=EDGE_LOOP('',(#62934,#62935,#62936,#62937,#62938,#62939,#62940,#62941));
#13150=EDGE_LOOP('',(#62942,#62943,#62944,#62945));
#13151=EDGE_LOOP('',(#62946,#62947,#62948,#62949,#62950));
#13152=EDGE_LOOP('',(#62951,#62952,#62953,#62954,#62955,#62956,#62957,#62958,
#62959,#62960,#62961,#62962,#62963,#62964,#62965,#62966,#62967,#62968));
#13153=EDGE_LOOP('',(#62969,#62970,#62971,#62972,#62973,#62974,#62975));
#13154=EDGE_LOOP('',(#62976,#62977,#62978,#62979));
#13155=EDGE_LOOP('',(#62980,#62981,#62982,#62983,#62984,#62985,#62986,#62987,
#62988,#62989,#62990,#62991,#62992,#62993,#62994,#62995,#62996,#62997,#62998,
#62999,#63000,#63001,#63002,#63003,#63004,#63005,#63006,#63007,#63008,#63009,
#63010,#63011,#63012,#63013,#63014,#63015,#63016,#63017,#63018,#63019,#63020,
#63021,#63022,#63023,#63024,#63025,#63026,#63027,#63028,#63029));
#13156=EDGE_LOOP('',(#63030,#63031,#63032,#63033));
#13157=EDGE_LOOP('',(#63034,#63035,#63036,#63037,#63038,#63039,#63040,#63041,
#63042));
#13158=EDGE_LOOP('',(#63043,#63044,#63045,#63046,#63047));
#13159=EDGE_LOOP('',(#63048,#63049,#63050,#63051));
#13160=EDGE_LOOP('',(#63052,#63053,#63054,#63055));
#13161=EDGE_LOOP('',(#63056,#63057,#63058,#63059,#63060,#63061));
#13162=EDGE_LOOP('',(#63062,#63063,#63064,#63065));
#13163=EDGE_LOOP('',(#63066,#63067,#63068,#63069));
#13164=EDGE_LOOP('',(#63070,#63071,#63072,#63073,#63074));
#13165=EDGE_LOOP('',(#63075,#63076,#63077,#63078));
#13166=EDGE_LOOP('',(#63079,#63080,#63081,#63082));
#13167=EDGE_LOOP('',(#63083,#63084,#63085,#63086));
#13168=EDGE_LOOP('',(#63087,#63088,#63089,#63090));
#13169=EDGE_LOOP('',(#63091,#63092,#63093,#63094));
#13170=EDGE_LOOP('',(#63095,#63096,#63097,#63098));
#13171=EDGE_LOOP('',(#63099,#63100,#63101,#63102,#63103));
#13172=EDGE_LOOP('',(#63104,#63105,#63106,#63107,#63108));
#13173=EDGE_LOOP('',(#63109,#63110,#63111,#63112,#63113));
#13174=EDGE_LOOP('',(#63114,#63115,#63116,#63117,#63118));
#13175=EDGE_LOOP('',(#63119,#63120,#63121,#63122));
#13176=EDGE_LOOP('',(#63123,#63124,#63125,#63126));
#13177=EDGE_LOOP('',(#63127,#63128,#63129,#63130,#63131,#63132));
#13178=EDGE_LOOP('',(#63133,#63134,#63135,#63136));
#13179=EDGE_LOOP('',(#63137,#63138,#63139,#63140));
#13180=EDGE_LOOP('',(#63141,#63142,#63143,#63144));
#13181=EDGE_LOOP('',(#63145,#63146,#63147,#63148));
#13182=EDGE_LOOP('',(#63149,#63150,#63151,#63152));
#13183=EDGE_LOOP('',(#63153,#63154,#63155,#63156));
#13184=EDGE_LOOP('',(#63157,#63158,#63159,#63160));
#13185=EDGE_LOOP('',(#63161,#63162,#63163,#63164));
#13186=EDGE_LOOP('',(#63165,#63166,#63167,#63168));
#13187=EDGE_LOOP('',(#63169,#63170,#63171,#63172,#63173,#63174,#63175,#63176,
#63177,#63178,#63179,#63180,#63181,#63182,#63183,#63184,#63185,#63186,#63187,
#63188,#63189,#63190,#63191,#63192));
#13188=EDGE_LOOP('',(#63193,#63194,#63195,#63196));
#13189=EDGE_LOOP('',(#63197,#63198,#63199,#63200));
#13190=EDGE_LOOP('',(#63201,#63202,#63203,#63204));
#13191=EDGE_LOOP('',(#63205,#63206,#63207,#63208));
#13192=EDGE_LOOP('',(#63209,#63210,#63211,#63212));
#13193=EDGE_LOOP('',(#63213,#63214,#63215,#63216));
#13194=EDGE_LOOP('',(#63217,#63218,#63219,#63220,#63221,#63222,#63223));
#13195=EDGE_LOOP('',(#63224,#63225,#63226,#63227));
#13196=EDGE_LOOP('',(#63228,#63229,#63230,#63231));
#13197=EDGE_LOOP('',(#63232,#63233,#63234,#63235,#63236,#63237,#63238,#63239,
#63240,#63241,#63242));
#13198=EDGE_LOOP('',(#63243,#63244,#63245,#63246,#63247,#63248,#63249,#63250));
#13199=EDGE_LOOP('',(#63251));
#13200=EDGE_LOOP('',(#63252,#63253,#63254,#63255,#63256,#63257));
#13201=EDGE_LOOP('',(#63258,#63259,#63260,#63261));
#13202=EDGE_LOOP('',(#63262,#63263,#63264,#63265,#63266,#63267,#63268,#63269));
#13203=EDGE_LOOP('',(#63270,#63271,#63272,#63273,#63274,#63275,#63276,#63277,
#63278));
#13204=EDGE_LOOP('',(#63279,#63280,#63281,#63282,#63283));
#13205=EDGE_LOOP('',(#63284,#63285,#63286,#63287,#63288));
#13206=EDGE_LOOP('',(#63289,#63290,#63291,#63292,#63293,#63294));
#13207=EDGE_LOOP('',(#63295,#63296,#63297,#63298));
#13208=EDGE_LOOP('',(#63299,#63300,#63301,#63302,#63303,#63304));
#13209=EDGE_LOOP('',(#63305,#63306,#63307,#63308));
#13210=EDGE_LOOP('',(#63309,#63310,#63311,#63312,#63313,#63314));
#13211=EDGE_LOOP('',(#63315,#63316,#63317,#63318,#63319,#63320,#63321,#63322,
#63323));
#13212=EDGE_LOOP('',(#63324,#63325,#63326,#63327,#63328,#63329,#63330,#63331,
#63332,#63333,#63334,#63335,#63336,#63337,#63338,#63339,#63340,#63341,#63342,
#63343,#63344,#63345,#63346,#63347,#63348,#63349,#63350,#63351,#63352,#63353,
#63354,#63355,#63356,#63357,#63358,#63359,#63360,#63361,#63362,#63363,#63364,
#63365,#63366,#63367,#63368,#63369));
#13213=EDGE_LOOP('',(#63370));
#13214=EDGE_LOOP('',(#63371));
#13215=EDGE_LOOP('',(#63372));
#13216=EDGE_LOOP('',(#63373,#63374,#63375,#63376));
#13217=EDGE_LOOP('',(#63377,#63378,#63379,#63380,#63381,#63382,#63383,#63384,
#63385,#63386,#63387,#63388,#63389,#63390,#63391,#63392,#63393,#63394));
#13218=EDGE_LOOP('',(#63395,#63396,#63397,#63398));
#13219=EDGE_LOOP('',(#63399,#63400,#63401,#63402,#63403,#63404,#63405,#63406));
#13220=EDGE_LOOP('',(#63407,#63408,#63409,#63410,#63411,#63412,#63413,#63414,
#63415,#63416,#63417,#63418,#63419,#63420,#63421,#63422,#63423,#63424,#63425));
#18355=CIRCLE('',#95343,0.4);
#18356=CIRCLE('',#95344,0.4);
#18357=CIRCLE('',#95345,0.4);
#18358=CIRCLE('',#95346,0.8);
#18359=CIRCLE('',#95347,0.4);
#18360=CIRCLE('',#95349,0.4);
#18361=CIRCLE('',#95350,4.65);
#18362=CIRCLE('',#95351,5.05);
#18363=CIRCLE('',#95352,0.400000000000001);
#18364=CIRCLE('',#95353,0.8);
#18365=CIRCLE('',#95354,0.4);
#18366=CIRCLE('',#95356,0.400000000000002);
#18367=CIRCLE('',#95357,10.0999999997296);
#18368=CIRCLE('',#95358,10.4999999997296);
#18369=CIRCLE('',#95359,0.4);
#18370=CIRCLE('',#95360,0.8);
#18371=CIRCLE('',#95361,0.4);
#18372=CIRCLE('',#95363,0.4);
#18373=CIRCLE('',#95364,12.);
#18374=CIRCLE('',#95365,11.6);
#18375=CIRCLE('',#95366,0.4);
#18376=CIRCLE('',#95367,0.8);
#18377=CIRCLE('',#95368,0.4);
#18378=CIRCLE('',#95370,0.4);
#18379=CIRCLE('',#95371,0.8);
#18380=CIRCLE('',#95372,0.4);
#18381=CIRCLE('',#95374,12.);
#18382=CIRCLE('',#95375,12.);
#18383=CIRCLE('',#95376,12.);
#18384=CIRCLE('',#95378,0.8);
#18385=CIRCLE('',#95381,0.8);
#18386=CIRCLE('',#95385,0.399999999999998);
#18387=CIRCLE('',#95386,0.400000000000001);
#18388=CIRCLE('',#95387,0.4);
#18389=CIRCLE('',#95388,0.6);
#18390=CIRCLE('',#95389,0.2);
#18391=CIRCLE('',#95391,0.4);
#18392=CIRCLE('',#95392,3.2);
#18393=CIRCLE('',#95393,3.6);
#18394=CIRCLE('',#95394,0.4);
#18395=CIRCLE('',#95395,0.8);
#18396=CIRCLE('',#95396,0.4);
#18397=CIRCLE('',#95398,0.4);
#18398=CIRCLE('',#95399,0.399999999999999);
#18399=CIRCLE('',#95400,0.8);
#18400=CIRCLE('',#95401,0.4);
#18401=CIRCLE('',#95403,0.4);
#18402=CIRCLE('',#95405,0.4);
#18403=CIRCLE('',#95406,0.8);
#18404=CIRCLE('',#95407,1.2);
#18405=CIRCLE('',#95409,0.4);
#18406=CIRCLE('',#95410,0.399999999999999);
#18407=CIRCLE('',#95411,0.8);
#18408=CIRCLE('',#95412,0.4);
#18409=CIRCLE('',#95414,0.399999999999999);
#18410=CIRCLE('',#95415,13.2);
#18411=CIRCLE('',#95416,13.6);
#18412=CIRCLE('',#95417,0.4);
#18413=CIRCLE('',#95418,0.6);
#18414=CIRCLE('',#95419,0.2);
#18415=CIRCLE('',#95421,0.4);
#18416=CIRCLE('',#95422,3.15);
#18417=CIRCLE('',#95423,3.15);
#18418=CIRCLE('',#95424,3.55);
#18419=CIRCLE('',#95425,0.8);
#18420=CIRCLE('',#95426,0.4);
#18421=CIRCLE('',#95429,0.8);
#18422=CIRCLE('',#95431,13.2);
#18423=CIRCLE('',#95433,0.6);
#18424=CIRCLE('',#95435,3.15);
#18425=CIRCLE('',#95436,3.15);
#18426=CIRCLE('',#95437,3.15);
#18427=CIRCLE('',#95438,3.15);
#18428=CIRCLE('',#95439,3.15);
#18429=CIRCLE('',#95440,3.15);
#18430=CIRCLE('',#95442,0.8);
#18431=CIRCLE('',#95446,0.4);
#18432=CIRCLE('',#95447,10.1000000149012);
#18433=CIRCLE('',#95448,0.4);
#18434=CIRCLE('',#95449,9.70000001490116);
#18435=CIRCLE('',#95450,0.4);
#18436=CIRCLE('',#95451,0.6);
#18437=CIRCLE('',#95452,0.2);
#18438=CIRCLE('',#95454,0.399999999999999);
#18439=CIRCLE('',#95455,0.399999999999999);
#18440=CIRCLE('',#95456,0.6);
#18441=CIRCLE('',#95457,0.2);
#18442=CIRCLE('',#95459,0.4);
#18443=CIRCLE('',#95460,0.4);
#18444=CIRCLE('',#95461,0.6);
#18445=CIRCLE('',#95462,0.2);
#18446=CIRCLE('',#95464,0.4);
#18447=CIRCLE('',#95465,3.2);
#18448=CIRCLE('',#95466,3.6);
#18449=CIRCLE('',#95467,0.400000000000001);
#18450=CIRCLE('',#95468,0.6);
#18451=CIRCLE('',#95469,0.2);
#18452=CIRCLE('',#95471,0.4);
#18453=CIRCLE('',#95472,0.4);
#18454=CIRCLE('',#95473,0.6);
#18455=CIRCLE('',#95474,0.2);
#18456=CIRCLE('',#95476,0.399999999999999);
#18457=CIRCLE('',#95477,3.55);
#18458=CIRCLE('',#95478,0.6);
#18459=CIRCLE('',#95479,0.2);
#18460=CIRCLE('',#95481,0.6);
#18461=CIRCLE('',#95482,0.6);
#18462=CIRCLE('',#95485,0.6);
#18463=CIRCLE('',#95487,0.6);
#18464=CIRCLE('',#95489,9.70000001490116);
#18465=CIRCLE('',#95492,0.400000000000001);
#18466=CIRCLE('',#95493,0.399999999999999);
#18467=CIRCLE('',#95494,0.399999999999999);
#18468=CIRCLE('',#95495,0.6);
#18469=CIRCLE('',#95496,0.2);
#18470=CIRCLE('',#95498,0.4);
#18471=CIRCLE('',#95499,9.70000001490116);
#18472=CIRCLE('',#95500,10.1000000149012);
#18473=CIRCLE('',#95501,0.4);
#18474=CIRCLE('',#95502,0.6);
#18475=CIRCLE('',#95503,0.2);
#18476=CIRCLE('',#95505,0.4);
#18477=CIRCLE('',#95506,3.7);
#18478=CIRCLE('',#95507,4.1);
#18479=CIRCLE('',#95509,0.399999999999999);
#18480=CIRCLE('',#95510,3.6);
#18481=CIRCLE('',#95511,3.2);
#18482=CIRCLE('',#95513,0.4);
#18483=CIRCLE('',#95515,0.399999999999999);
#18484=CIRCLE('',#95516,5.40000000000001);
#18485=CIRCLE('',#95517,5.80000000000001);
#18486=CIRCLE('',#95518,0.4);
#18487=CIRCLE('',#95519,0.6);
#18488=CIRCLE('',#95520,0.2);
#18489=CIRCLE('',#95522,0.4);
#18490=CIRCLE('',#95523,0.6);
#18491=CIRCLE('',#95524,0.2);
#18492=CIRCLE('',#95527,5.40000000000001);
#18493=CIRCLE('',#95529,0.6);
#18494=CIRCLE('',#95532,0.6);
#18495=CIRCLE('',#95536,0.4);
#18496=CIRCLE('',#95537,5.2);
#18497=CIRCLE('',#95538,0.4);
#18498=CIRCLE('',#95539,4.8);
#18499=CIRCLE('',#95540,0.4);
#18500=CIRCLE('',#95541,0.6);
#18501=CIRCLE('',#95542,0.2);
#18502=CIRCLE('',#95544,0.399999999999999);
#18503=CIRCLE('',#95545,5.4);
#18504=CIRCLE('',#95546,5.8);
#18505=CIRCLE('',#95548,0.4);
#18506=CIRCLE('',#95549,7.99496173936711);
#18507=CIRCLE('',#95550,7.59496173936711);
#18508=CIRCLE('',#95551,0.4);
#18509=CIRCLE('',#95552,0.8);
#18510=CIRCLE('',#95553,0.4);
#18511=CIRCLE('',#95555,0.4);
#18512=CIRCLE('',#95557,0.4);
#18513=CIRCLE('',#95558,0.8);
#18514=CIRCLE('',#95559,1.2);
#18515=CIRCLE('',#95561,0.4);
#18516=CIRCLE('',#95562,0.4);
#18517=CIRCLE('',#95563,0.8);
#18518=CIRCLE('',#95564,0.4);
#18519=CIRCLE('',#95566,0.4);
#18520=CIRCLE('',#95567,0.4);
#18521=CIRCLE('',#95568,0.6);
#18522=CIRCLE('',#95569,0.2);
#18523=CIRCLE('',#95571,0.4);
#18524=CIRCLE('',#95572,3.1);
#18525=CIRCLE('',#95573,3.5);
#18526=CIRCLE('',#95574,0.400000000000001);
#18527=CIRCLE('',#95575,0.800000000000001);
#18528=CIRCLE('',#95576,0.400000000000001);
#18529=CIRCLE('',#95579,0.8);
#18530=CIRCLE('',#95582,0.6);
#18531=CIRCLE('',#95584,3.1);
#18532=CIRCLE('',#95586,0.800000000000001);
#18533=CIRCLE('',#95589,4.8);
#18534=CIRCLE('',#95592,0.400000000000002);
#18535=CIRCLE('',#95593,9.79496173936711);
#18536=CIRCLE('',#95594,0.400000000000001);
#18537=CIRCLE('',#95595,9.3949617393671);
#18538=CIRCLE('',#95597,0.4);
#18539=CIRCLE('',#95598,4.);
#18540=CIRCLE('',#95599,3.6);
#18541=CIRCLE('',#95600,0.4);
#18542=CIRCLE('',#95601,0.6);
#18543=CIRCLE('',#95602,0.2);
#18544=CIRCLE('',#95604,0.4);
#18545=CIRCLE('',#95605,9.7);
#18546=CIRCLE('',#95606,10.1);
#18547=CIRCLE('',#95607,0.400000000000001);
#18548=CIRCLE('',#95608,0.6);
#18549=CIRCLE('',#95609,0.2);
#18550=CIRCLE('',#95611,0.400000000000001);
#18551=CIRCLE('',#95612,17.3949617393671);
#18552=CIRCLE('',#95613,16.9949617393671);
#18553=CIRCLE('',#95614,0.4);
#18554=CIRCLE('',#95615,0.8);
#18555=CIRCLE('',#95616,0.4);
#18556=CIRCLE('',#95618,0.4);
#18557=CIRCLE('',#95619,0.8);
#18558=CIRCLE('',#95620,0.4);
#18559=CIRCLE('',#95622,17.3949617393671);
#18560=CIRCLE('',#95624,0.8);
#18561=CIRCLE('',#95627,0.8);
#18562=CIRCLE('',#95629,9.3949617393671);
#18563=CIRCLE('',#95632,0.400000000000001);
#18564=CIRCLE('',#95633,4.);
#18565=CIRCLE('',#95634,0.4);
#18566=CIRCLE('',#95635,3.6);
#18567=CIRCLE('',#95636,0.400000000000003);
#18568=CIRCLE('',#95637,0.8);
#18569=CIRCLE('',#95638,0.4);
#18570=CIRCLE('',#95640,0.399999999999998);
#18571=CIRCLE('',#95641,23.7449617393671);
#18572=CIRCLE('',#95642,23.3449617393671);
#18573=CIRCLE('',#95644,0.400000000000003);
#18574=CIRCLE('',#95645,0.4);
#18575=CIRCLE('',#95646,0.8);
#18576=CIRCLE('',#95648,0.4);
#18577=CIRCLE('',#95649,7.8);
#18578=CIRCLE('',#95650,8.2);
#18579=CIRCLE('',#95651,0.399999999999998);
#18580=CIRCLE('',#95652,0.8);
#18581=CIRCLE('',#95653,0.4);
#18582=CIRCLE('',#95655,0.4);
#18583=CIRCLE('',#95656,0.4);
#18584=CIRCLE('',#95657,0.6);
#18585=CIRCLE('',#95658,0.2);
#18586=CIRCLE('',#95660,0.4);
#18587=CIRCLE('',#95661,0.4);
#18588=CIRCLE('',#95662,0.8);
#18589=CIRCLE('',#95663,0.4);
#18590=CIRCLE('',#95665,0.4);
#18591=CIRCLE('',#95666,0.4);
#18592=CIRCLE('',#95667,0.8);
#18593=CIRCLE('',#95668,0.4);
#18594=CIRCLE('',#95670,0.4);
#18595=CIRCLE('',#95671,18.9949617393671);
#18596=CIRCLE('',#95672,19.3949617393671);
#18597=CIRCLE('',#95673,0.399999999999999);
#18598=CIRCLE('',#95674,0.6);
#18599=CIRCLE('',#95675,0.2);
#18600=CIRCLE('',#95677,0.4);
#18601=CIRCLE('',#95678,9.7);
#18602=CIRCLE('',#95679,10.1);
#18603=CIRCLE('',#95680,0.6);
#18604=CIRCLE('',#95681,0.2);
#18605=CIRCLE('',#95683,0.8);
#18606=CIRCLE('',#95686,0.8);
#18607=CIRCLE('',#95688,18.9949617393671);
#18608=CIRCLE('',#95690,0.6);
#18609=CIRCLE('',#95692,9.7);
#18610=CIRCLE('',#95694,0.6);
#18611=CIRCLE('',#95696,3.6);
#18612=CIRCLE('',#95697,3.6);
#18613=CIRCLE('',#95700,0.4);
#18614=CIRCLE('',#95701,5.05);
#18615=CIRCLE('',#95702,0.4);
#18616=CIRCLE('',#95703,4.65);
#18617=CIRCLE('',#95704,0.399999999999998);
#18618=CIRCLE('',#95705,0.8);
#18619=CIRCLE('',#95706,0.4);
#18620=CIRCLE('',#95708,0.400000000000001);
#18621=CIRCLE('',#95709,13.4);
#18622=CIRCLE('',#95710,13.);
#18623=CIRCLE('',#95712,0.4);
#18624=CIRCLE('',#95713,0.4);
#18625=CIRCLE('',#95714,0.8);
#18626=CIRCLE('',#95715,0.4);
#18627=CIRCLE('',#95717,0.4);
#18628=CIRCLE('',#95718,12.);
#18629=CIRCLE('',#95719,11.6);
#18630=CIRCLE('',#95720,0.4);
#18631=CIRCLE('',#95721,0.8);
#18632=CIRCLE('',#95722,0.4);
#18633=CIRCLE('',#95724,0.400000000000002);
#18634=CIRCLE('',#95725,10.0999999997296);
#18635=CIRCLE('',#95726,10.4999999997296);
#18636=CIRCLE('',#95727,0.8);
#18637=CIRCLE('',#95728,0.4);
#18638=CIRCLE('',#95730,12.);
#18639=CIRCLE('',#95731,12.);
#18640=CIRCLE('',#95732,12.);
#18641=CIRCLE('',#95734,0.8);
#18642=CIRCLE('',#95736,10.0999999997296);
#18643=CIRCLE('',#95738,0.8);
#18644=CIRCLE('',#95740,4.65);
#18645=CIRCLE('',#95743,0.4);
#18646=CIRCLE('',#95744,0.4);
#18647=CIRCLE('',#95745,0.399999999999999);
#18648=CIRCLE('',#95746,0.6);
#18649=CIRCLE('',#95747,0.2);
#18650=CIRCLE('',#95749,0.4);
#18651=CIRCLE('',#95750,0.4);
#18652=CIRCLE('',#95751,0.6);
#18653=CIRCLE('',#95752,0.2);
#18654=CIRCLE('',#95754,0.399999999999999);
#18655=CIRCLE('',#95755,3.6);
#18656=CIRCLE('',#95756,4.);
#18657=CIRCLE('',#95757,0.4);
#18658=CIRCLE('',#95758,0.6);
#18659=CIRCLE('',#95759,0.2);
#18660=CIRCLE('',#95761,0.4);
#18661=CIRCLE('',#95762,13.2);
#18662=CIRCLE('',#95763,13.6);
#18663=CIRCLE('',#95764,0.6);
#18664=CIRCLE('',#95765,0.2);
#18665=CIRCLE('',#95767,0.6);
#18666=CIRCLE('',#95769,13.2);
#18667=CIRCLE('',#95771,0.6);
#18668=CIRCLE('',#95774,0.200000000000001);
#18669=CIRCLE('',#95775,0.2);
#18670=CIRCLE('',#95777,0.4);
#18671=CIRCLE('',#95779,8.5);
#18672=CIRCLE('',#95780,8.5);
#18673=CIRCLE('',#95781,8.5);
#18674=CIRCLE('',#95782,8.5);
#18675=CIRCLE('',#95783,8.5);
#18676=CIRCLE('',#95784,8.5);
#18677=CIRCLE('',#95785,8.5);
#18678=CIRCLE('',#95786,8.5);
#18679=CIRCLE('',#95789,0.4);
#18680=CIRCLE('',#95790,0.4);
#18681=CIRCLE('',#95792,0.8);
#18682=CIRCLE('',#95793,0.8);
#18683=CIRCLE('',#95794,0.6);
#18684=CIRCLE('',#95797,0.8);
#18685=CIRCLE('',#95798,0.8);
#18686=CIRCLE('',#95800,4.2);
#18687=CIRCLE('',#95801,0.4);
#18688=CIRCLE('',#95802,0.79999999999745);
#18689=CIRCLE('',#95803,0.6);
#18690=CIRCLE('',#95804,0.6);
#18691=CIRCLE('',#95805,3.2);
#18692=CIRCLE('',#95806,10.45);
#18693=CIRCLE('',#95807,3.43614417320658);
#18694=CIRCLE('',#95808,0.6);
#18695=CIRCLE('',#95809,3.2);
#18696=CIRCLE('',#95810,0.8);
#18697=CIRCLE('',#95811,0.8);
#18698=CIRCLE('',#95812,0.8);
#18699=CIRCLE('',#95813,3.60000000004514);
#18700=CIRCLE('',#95814,1.6);
#18701=CIRCLE('',#95816,4.2);
#18702=CIRCLE('',#95818,4.);
#18703=CIRCLE('',#95819,0.8);
#18704=CIRCLE('',#95820,0.8);
#18705=CIRCLE('',#95821,8.4949617393671);
#18706=CIRCLE('',#95822,4.9);
#18707=CIRCLE('',#95823,0.8);
#18708=CIRCLE('',#95824,0.6);
#18709=CIRCLE('',#95825,9.70000001490116);
#18710=CIRCLE('',#95826,0.6);
#18711=CIRCLE('',#95827,3.7);
#18712=CIRCLE('',#95828,3.6);
#18713=CIRCLE('',#95829,0.4);
#18714=CIRCLE('',#95830,0.8);
#18715=CIRCLE('',#95831,0.6);
#18716=CIRCLE('',#95832,5.4);
#18717=CIRCLE('',#95833,7.99496173936711);
#18718=CIRCLE('',#95834,0.8);
#18719=CIRCLE('',#95835,1.55);
#18720=CIRCLE('',#95838,0.8);
#18721=CIRCLE('',#95841,4.);
#18722=CIRCLE('',#95842,3.60000000004514);
#18723=CIRCLE('',#95843,0.8);
#18724=CIRCLE('',#95844,0.8);
#18725=CIRCLE('',#95845,0.8);
#18726=CIRCLE('',#95846,0.8);
#18727=CIRCLE('',#95847,1.58);
#18728=CIRCLE('',#95848,3.25);
#18729=CIRCLE('',#95849,3.25);
#18730=CIRCLE('',#95850,10.9);
#18731=CIRCLE('',#95851,0.8);
#18732=CIRCLE('',#95852,0.8);
#18733=CIRCLE('',#95853,0.8);
#18734=CIRCLE('',#95854,1.6);
#18735=CIRCLE('',#95855,1.6);
#18736=CIRCLE('',#95856,1.6);
#18737=CIRCLE('',#95857,1.55);
#18738=CIRCLE('',#95858,3.05);
#18739=CIRCLE('',#95862,0.8);
#18740=CIRCLE('',#95864,0.8);
#18741=CIRCLE('',#95867,1.);
#18742=CIRCLE('',#95868,2.);
#18743=CIRCLE('',#95869,7.8);
#18744=CIRCLE('',#95870,0.8);
#18745=CIRCLE('',#95871,0.6);
#18746=CIRCLE('',#95872,100.);
#18747=CIRCLE('',#95873,0.8);
#18748=CIRCLE('',#95874,18.2949617393671);
#18749=CIRCLE('',#95876,0.8);
#18750=CIRCLE('',#95879,0.8);
#18751=CIRCLE('',#95881,0.8);
#18752=CIRCLE('',#95882,4.65);
#18753=CIRCLE('',#95883,0.8);
#18754=CIRCLE('',#95884,10.0999999997296);
#18755=CIRCLE('',#95885,0.8);
#18756=CIRCLE('',#95886,3.75);
#18757=CIRCLE('',#95887,0.8);
#18758=CIRCLE('',#95888,13.4);
#18759=CIRCLE('',#95889,0.8);
#18760=CIRCLE('',#95890,0.4);
#18761=CIRCLE('',#95891,3.05);
#18762=CIRCLE('',#95903,0.6);
#18763=CIRCLE('',#95905,9.7);
#18764=CIRCLE('',#95907,0.6);
#18765=CIRCLE('',#95909,23.7449617393671);
#18766=CIRCLE('',#95911,0.4);
#18767=CIRCLE('',#95913,7.8);
#18768=CIRCLE('',#95919,17.3949617393671);
#18769=CIRCLE('',#95920,9.3949617393671);
#18770=CIRCLE('',#95934,17.3949617393671);
#18771=CIRCLE('',#95939,0.79999999999745);
#18772=CIRCLE('',#95940,0.6);
#18773=CIRCLE('',#95941,0.6);
#18774=CIRCLE('',#95946,1.55);
#18775=CIRCLE('',#95948,3.43614417320658);
#18776=CIRCLE('',#95950,10.45);
#18777=CIRCLE('',#95952,0.6);
#18778=CIRCLE('',#95955,100.);
#18779=CIRCLE('',#95957,0.8);
#18780=CIRCLE('',#95960,0.6);
#18781=CIRCLE('',#95962,3.6);
#18782=CIRCLE('',#95976,0.6);
#18783=CIRCLE('',#95982,0.8);
#18784=CIRCLE('',#95983,2.);
#18785=CIRCLE('',#95984,1.);
#18786=CIRCLE('',#95985,0.4);
#18787=CIRCLE('',#95986,3.75);
#18788=CIRCLE('',#95987,2.3);
#18789=CIRCLE('',#95989,4.);
#18790=CIRCLE('',#95990,4.);
#18791=CIRCLE('',#95999,1.6);
#18792=CIRCLE('',#96001,1.6);
#18793=CIRCLE('',#96003,2.);
#18794=CIRCLE('',#96006,3.25);
#18795=CIRCLE('',#96009,3.25);
#18796=CIRCLE('',#96011,1.6);
#18797=CIRCLE('',#96014,1.6);
#18798=CIRCLE('',#96017,1.55);
#18799=CIRCLE('',#96020,2.);
#18800=CIRCLE('',#96022,1.58);
#18801=CIRCLE('',#96024,2.);
#18802=CIRCLE('',#96027,10.9);
#18803=CIRCLE('',#96030,1.);
#18804=CIRCLE('',#96032,2.);
#18805=CIRCLE('',#96033,1.);
#18806=CIRCLE('',#96048,11.65);
#18807=CIRCLE('',#96049,6.4499999999938);
#18808=CIRCLE('',#96053,0.8);
#18809=CIRCLE('',#96054,0.8);
#18810=CIRCLE('',#96056,5.);
#18811=CIRCLE('',#96057,0.8);
#18812=CIRCLE('',#96058,0.8);
#18813=CIRCLE('',#96059,0.4);
#18814=CIRCLE('',#96060,10.6);
#18815=CIRCLE('',#96061,0.4);
#18816=CIRCLE('',#96062,0.8);
#18817=CIRCLE('',#96063,0.8);
#18818=CIRCLE('',#96064,0.4);
#18819=CIRCLE('',#96065,10.);
#18820=CIRCLE('',#96066,0.8);
#18821=CIRCLE('',#96068,5.);
#18822=CIRCLE('',#96070,0.8);
#18823=CIRCLE('',#96073,0.4);
#18824=CIRCLE('',#96074,5.05);
#18825=CIRCLE('',#96075,0.4);
#18826=CIRCLE('',#96076,4.65);
#18827=CIRCLE('',#96077,0.4);
#18828=CIRCLE('',#96078,0.8);
#18829=CIRCLE('',#96079,0.4);
#18830=CIRCLE('',#96081,0.4);
#18831=CIRCLE('',#96082,0.4);
#18832=CIRCLE('',#96083,0.8);
#18833=CIRCLE('',#96084,0.4);
#18834=CIRCLE('',#96086,0.4);
#18835=CIRCLE('',#96087,0.4);
#18836=CIRCLE('',#96088,0.8);
#18837=CIRCLE('',#96089,0.4);
#18838=CIRCLE('',#96091,0.399999999999996);
#18839=CIRCLE('',#96092,10.6);
#18840=CIRCLE('',#96093,11.);
#18841=CIRCLE('',#96094,0.6);
#18842=CIRCLE('',#96095,0.2);
#18843=CIRCLE('',#96097,0.8);
#18844=CIRCLE('',#96099,10.6);
#18845=CIRCLE('',#96101,0.6);
#18846=CIRCLE('',#96103,4.64999999999989);
#18847=CIRCLE('',#96104,4.64999999999989);
#18848=CIRCLE('',#96107,3.6);
#18849=CIRCLE('',#96108,0.4);
#18850=CIRCLE('',#96109,4.);
#18851=CIRCLE('',#96111,2.1);
#18852=CIRCLE('',#96112,0.4);
#18853=CIRCLE('',#96113,2.5);
#18854=CIRCLE('',#96115,0.4);
#18855=CIRCLE('',#96117,2.5);
#18856=CIRCLE('',#96118,2.1);
#18857=CIRCLE('',#96120,16.9949617393671);
#18858=CIRCLE('',#96121,0.4);
#18859=CIRCLE('',#96122,17.3949617393671);
#18860=CIRCLE('',#96124,4.);
#18861=CIRCLE('',#96125,3.6);
#18862=CIRCLE('',#96127,9.3949617393671);
#18863=CIRCLE('',#96128,9.79496173936711);
#18864=CIRCLE('',#96131,4.);
#18865=CIRCLE('',#96133,9.3949617393671);
#18866=CIRCLE('',#96136,17.3949617393671);
#18867=CIRCLE('',#96139,11.95);
#18868=CIRCLE('',#96140,0.399999999999996);
#18869=CIRCLE('',#96141,11.55);
#18870=CIRCLE('',#96142,0.4);
#18871=CIRCLE('',#96143,0.599999999999999);
#18872=CIRCLE('',#96144,0.199999999999999);
#18873=CIRCLE('',#96146,4.2);
#18874=CIRCLE('',#96147,3.8);
#18875=CIRCLE('',#96148,4.2);
#18876=CIRCLE('',#96150,11.55);
#18877=CIRCLE('',#96153,3.8);
#18878=CIRCLE('',#96154,3.8);
#18879=CIRCLE('',#96156,0.4);
#18880=CIRCLE('',#96158,0.2);
#18881=CIRCLE('',#96161,0.4);
#18882=CIRCLE('',#96162,0.4);
#18883=CIRCLE('',#96163,0.6);
#18884=CIRCLE('',#96166,0.4);
#18885=CIRCLE('',#96167,2.85);
#18886=CIRCLE('',#96168,1.65);
#18887=CIRCLE('',#96171,4.64877154610377);
#18888=CIRCLE('',#96179,4.2);
#18889=CIRCLE('',#96180,0.4);
#18890=CIRCLE('',#96181,3.8);
#18891=CIRCLE('',#96182,0.4);
#18892=CIRCLE('',#96183,0.6);
#18893=CIRCLE('',#96184,0.2);
#18894=CIRCLE('',#96186,0.400000000000005);
#18895=CIRCLE('',#96187,24.9449617393673);
#18896=CIRCLE('',#96188,25.3449617393673);
#18897=CIRCLE('',#96189,0.4);
#18898=CIRCLE('',#96190,0.6);
#18899=CIRCLE('',#96191,0.2);
#18900=CIRCLE('',#96196,3.6);
#18901=CIRCLE('',#96199,3.8);
#18902=CIRCLE('',#96202,3.69774423765867);
#18903=CIRCLE('',#96203,4.09750037145961);
#18904=CIRCLE('',#96204,0.4);
#18905=CIRCLE('',#96205,0.600000000000001);
#18906=CIRCLE('',#96207,0.4);
#18907=CIRCLE('',#96208,3.6);
#18908=CIRCLE('',#96210,4.1);
#18909=CIRCLE('',#96211,0.4);
#18910=CIRCLE('',#96212,3.7);
#18911=CIRCLE('',#96214,8.8);
#18912=CIRCLE('',#96215,0.2);
#18913=CIRCLE('',#96216,0.2);
#18914=CIRCLE('',#96217,0.2);
#18915=CIRCLE('',#96219,0.4);
#18916=CIRCLE('',#96220,0.4);
#18917=CIRCLE('',#96221,0.6);
#18918=CIRCLE('',#96223,0.4);
#18919=CIRCLE('',#96224,0.4);
#18920=CIRCLE('',#96225,0.6);
#18921=CIRCLE('',#96227,0.4);
#18922=CIRCLE('',#96228,0.4);
#18923=CIRCLE('',#96229,0.6);
#18924=CIRCLE('',#96231,9.2);
#18925=CIRCLE('',#96233,0.600000000000001);
#18926=CIRCLE('',#96235,3.6);
#18927=CIRCLE('',#96237,3.7);
#18928=CIRCLE('',#96240,0.6);
#18929=CIRCLE('',#96243,0.6);
#18930=CIRCLE('',#96246,0.6);
#18931=CIRCLE('',#96248,9.2);
#18932=CIRCLE('',#96249,9.2);
#18933=CIRCLE('',#96251,9.2);
#18934=CIRCLE('',#96254,0.399999999999999);
#18935=CIRCLE('',#96255,4.6);
#18936=CIRCLE('',#96256,0.399999999999996);
#18937=CIRCLE('',#96257,4.2);
#18938=CIRCLE('',#96258,0.4);
#18939=CIRCLE('',#96259,0.800000000000001);
#18940=CIRCLE('',#96260,0.400000000000001);
#18941=CIRCLE('',#96262,0.4);
#18942=CIRCLE('',#96264,0.4);
#18943=CIRCLE('',#96265,0.8);
#18944=CIRCLE('',#96266,1.2);
#18945=CIRCLE('',#96268,0.4);
#18946=CIRCLE('',#96269,0.4);
#18947=CIRCLE('',#96270,0.8);
#18948=CIRCLE('',#96271,0.4);
#18949=CIRCLE('',#96273,0.400000000000001);
#18950=CIRCLE('',#96274,6.1);
#18951=CIRCLE('',#96275,0.4);
#18952=CIRCLE('',#96276,5.7);
#18953=CIRCLE('',#96277,0.4);
#18954=CIRCLE('',#96278,0.6);
#18955=CIRCLE('',#96279,0.2);
#18956=CIRCLE('',#96281,0.4);
#18957=CIRCLE('',#96282,4.8);
#18958=CIRCLE('',#96283,5.2);
#18959=CIRCLE('',#96285,0.4);
#18960=CIRCLE('',#96287,7.69496173936711);
#18961=CIRCLE('',#96288,7.2949617393671);
#18962=CIRCLE('',#96290,0.399999999999999);
#18963=CIRCLE('',#96293,0.8);
#18964=CIRCLE('',#96296,0.8);
#18965=CIRCLE('',#96298,7.69496173936711);
#18966=CIRCLE('',#96300,5.7);
#18967=CIRCLE('',#96303,0.400000000000003);
#18968=CIRCLE('',#96304,0.4);
#18969=CIRCLE('',#96305,0.400000000000005);
#18970=CIRCLE('',#96306,0.6);
#18971=CIRCLE('',#96307,0.2);
#18972=CIRCLE('',#96309,0.4);
#18973=CIRCLE('',#96311,0.400000000000005);
#18974=CIRCLE('',#96312,4.1);
#18975=CIRCLE('',#96313,4.5);
#18976=CIRCLE('',#96314,0.400000000000005);
#18977=CIRCLE('',#96315,0.6);
#18978=CIRCLE('',#96316,0.2);
#18979=CIRCLE('',#96318,0.4);
#18980=CIRCLE('',#96320,0.4);
#18981=CIRCLE('',#96321,7.8);
#18982=CIRCLE('',#96322,8.2);
#18983=CIRCLE('',#96323,0.4);
#18984=CIRCLE('',#96324,0.6);
#18985=CIRCLE('',#96325,0.2);
#18986=CIRCLE('',#96327,0.399999999999996);
#18987=CIRCLE('',#96328,19.0949617393671);
#18988=CIRCLE('',#96329,19.4949617393671);
#18989=CIRCLE('',#96330,0.4);
#18990=CIRCLE('',#96331,0.8);
#18991=CIRCLE('',#96332,0.4);
#18992=CIRCLE('',#96334,0.4);
#18993=CIRCLE('',#96335,0.8);
#18994=CIRCLE('',#96336,0.4);
#18995=CIRCLE('',#96338,0.6);
#18996=CIRCLE('',#96340,19.0949617393671);
#18997=CIRCLE('',#96342,0.8);
#18998=CIRCLE('',#96345,0.8);
#18999=CIRCLE('',#96349,0.4);
#19000=CIRCLE('',#96350,0.4);
#19001=CIRCLE('',#96351,0.4);
#19002=CIRCLE('',#96352,0.6);
#19003=CIRCLE('',#96353,0.2);
#19004=CIRCLE('',#96355,0.4);
#19005=CIRCLE('',#96356,0.4);
#19006=CIRCLE('',#96357,0.6);
#19007=CIRCLE('',#96358,0.2);
#19008=CIRCLE('',#96360,0.4);
#19009=CIRCLE('',#96362,0.4);
#19010=CIRCLE('',#96363,3.7);
#19011=CIRCLE('',#96364,4.1);
#19012=CIRCLE('',#96366,0.4);
#19013=CIRCLE('',#96367,6.6);
#19014=CIRCLE('',#96368,6.2);
#19015=CIRCLE('',#96369,0.4);
#19016=CIRCLE('',#96370,0.6);
#19017=CIRCLE('',#96371,0.2);
#19018=CIRCLE('',#96373,0.4);
#19019=CIRCLE('',#96374,22.5949617393671);
#19020=CIRCLE('',#96375,22.1949617393671);
#19021=CIRCLE('',#96377,0.4);
#19022=CIRCLE('',#96378,9.2);
#19023=CIRCLE('',#96379,8.8);
#19024=CIRCLE('',#96380,0.6);
#19025=CIRCLE('',#96381,0.2);
#19026=CIRCLE('',#96383,6.6);
#19027=CIRCLE('',#96385,0.6);
#19028=CIRCLE('',#96387,22.5949617393671);
#19029=CIRCLE('',#96388,22.5949617393671);
#19030=CIRCLE('',#96390,9.2);
#19031=CIRCLE('',#96392,9.2);
#19032=CIRCLE('',#96394,0.6);
#19033=CIRCLE('',#96398,12.05);
#19034=CIRCLE('',#96399,0.400000000000005);
#19035=CIRCLE('',#96400,11.65);
#19036=CIRCLE('',#96401,0.4);
#19037=CIRCLE('',#96402,0.6);
#19038=CIRCLE('',#96403,0.2);
#19039=CIRCLE('',#96405,0.4);
#19040=CIRCLE('',#96406,3.2);
#19041=CIRCLE('',#96407,3.6);
#19042=CIRCLE('',#96408,0.4);
#19043=CIRCLE('',#96409,0.6);
#19044=CIRCLE('',#96410,0.2);
#19045=CIRCLE('',#96414,0.4);
#19046=CIRCLE('',#96416,0.6);
#19047=CIRCLE('',#96418,3.7);
#19048=CIRCLE('',#96419,3.6);
#19049=CIRCLE('',#96420,4.1);
#19050=CIRCLE('',#96424,11.65);
#19051=CIRCLE('',#96425,11.65);
#19052=CIRCLE('',#96427,0.399999999999998);
#19053=CIRCLE('',#96428,0.4);
#19054=CIRCLE('',#96430,0.4);
#19055=CIRCLE('',#96431,0.8);
#19056=CIRCLE('',#96432,1.2);
#19057=CIRCLE('',#96434,0.4);
#19058=CIRCLE('',#96435,0.4);
#19059=CIRCLE('',#96436,0.6);
#19060=CIRCLE('',#96437,0.2);
#19061=CIRCLE('',#96439,0.4);
#19062=CIRCLE('',#96440,9.2);
#19063=CIRCLE('',#96441,8.8);
#19064=CIRCLE('',#96442,0.4);
#19065=CIRCLE('',#96443,0.6);
#19066=CIRCLE('',#96444,0.2);
#19067=CIRCLE('',#96446,0.4);
#19068=CIRCLE('',#96447,0.4);
#19069=CIRCLE('',#96448,0.6);
#19070=CIRCLE('',#96449,0.2);
#19071=CIRCLE('',#96451,0.4);
#19072=CIRCLE('',#96452,3.5);
#19073=CIRCLE('',#96453,3.5);
#19074=CIRCLE('',#96454,3.9);
#19075=CIRCLE('',#96455,0.4);
#19076=CIRCLE('',#96456,0.6);
#19077=CIRCLE('',#96457,0.2);
#19078=CIRCLE('',#96459,0.4);
#19079=CIRCLE('',#96460,0.800000000000001);
#19080=CIRCLE('',#96461,0.400000000000001);
#19081=CIRCLE('',#96463,0.6);
#19082=CIRCLE('',#96465,3.5);
#19083=CIRCLE('',#96466,3.5);
#19084=CIRCLE('',#96467,3.5);
#19085=CIRCLE('',#96468,3.5);
#19086=CIRCLE('',#96469,3.5);
#19087=CIRCLE('',#96470,3.5);
#19088=CIRCLE('',#96472,0.6);
#19089=CIRCLE('',#96475,0.800000000000001);
#19090=CIRCLE('',#96479,8.8);
#19091=CIRCLE('',#96480,0.4);
#19092=CIRCLE('',#96481,9.2);
#19093=CIRCLE('',#96482,0.4);
#19094=CIRCLE('',#96483,0.6);
#19095=CIRCLE('',#96484,0.2);
#19096=CIRCLE('',#96486,0.4);
#19097=CIRCLE('',#96487,0.4);
#19098=CIRCLE('',#96488,0.6);
#19099=CIRCLE('',#96489,0.2);
#19100=CIRCLE('',#96491,0.4);
#19101=CIRCLE('',#96492,0.4);
#19102=CIRCLE('',#96493,0.6);
#19103=CIRCLE('',#96494,0.2);
#19104=CIRCLE('',#96496,0.4);
#19105=CIRCLE('',#96497,3.9);
#19106=CIRCLE('',#96498,0.4);
#19107=CIRCLE('',#96499,0.6);
#19108=CIRCLE('',#96500,0.2);
#19109=CIRCLE('',#96502,0.4);
#19110=CIRCLE('',#96503,0.4);
#19111=CIRCLE('',#96504,0.6);
#19112=CIRCLE('',#96505,0.2);
#19113=CIRCLE('',#96507,9.2);
#19114=CIRCLE('',#96508,8.8);
#19115=CIRCLE('',#96510,3.69774423765867);
#19116=CIRCLE('',#96511,4.0975003714596);
#19117=CIRCLE('',#96514,0.6);
#19118=CIRCLE('',#96517,9.2);
#19119=CIRCLE('',#96518,9.2);
#19120=CIRCLE('',#96522,9.2);
#19121=CIRCLE('',#96523,9.2);
#19122=CIRCLE('',#96526,0.4);
#19123=CIRCLE('',#96527,8.8);
#19124=CIRCLE('',#96528,0.4);
#19125=CIRCLE('',#96529,9.2);
#19126=CIRCLE('',#96530,0.4);
#19127=CIRCLE('',#96531,0.6);
#19128=CIRCLE('',#96532,0.2);
#19129=CIRCLE('',#96534,0.4);
#19130=CIRCLE('',#96535,0.4);
#19131=CIRCLE('',#96536,0.6);
#19132=CIRCLE('',#96537,0.2);
#19133=CIRCLE('',#96539,0.4);
#19134=CIRCLE('',#96540,3.9);
#19135=CIRCLE('',#96541,0.4);
#19136=CIRCLE('',#96542,0.6);
#19137=CIRCLE('',#96543,0.2);
#19138=CIRCLE('',#96545,0.4);
#19139=CIRCLE('',#96546,0.4);
#19140=CIRCLE('',#96547,0.6);
#19141=CIRCLE('',#96548,0.2);
#19142=CIRCLE('',#96550,0.4);
#19143=CIRCLE('',#96551,0.6);
#19144=CIRCLE('',#96552,0.2);
#19145=CIRCLE('',#96555,0.6);
#19146=CIRCLE('',#96558,0.6);
#19147=CIRCLE('',#96560,9.2);
#19148=CIRCLE('',#96561,9.2);
#19149=CIRCLE('',#96564,9.2);
#19150=CIRCLE('',#96567,0.8);
#19151=CIRCLE('',#96570,0.6);
#19152=CIRCLE('',#96572,0.6);
#19153=CIRCLE('',#96574,3.2);
#19154=CIRCLE('',#96576,0.399999999999999);
#19155=CIRCLE('',#96577,0.399999999999999);
#19156=CIRCLE('',#96581,0.4);
#19157=CIRCLE('',#96582,0.4);
#19158=CIRCLE('',#96584,0.6);
#19159=CIRCLE('',#96586,0.8);
#19160=CIRCLE('',#96587,0.8);
#19161=CIRCLE('',#96589,0.8);
#19162=CIRCLE('',#96590,0.8);
#19163=CIRCLE('',#96592,3.43614417320659);
#19164=CIRCLE('',#96593,3.43614417320659);
#19165=CIRCLE('',#96596,3.60000000004514);
#19166=CIRCLE('',#96597,3.60000000004514);
#19167=CIRCLE('',#96599,2.8);
#19168=CIRCLE('',#96600,1.6);
#19169=CIRCLE('',#96602,1.6);
#19170=CIRCLE('',#96604,2.8);
#19171=CIRCLE('',#96607,0.4);
#19172=CIRCLE('',#96609,4.2);
#19173=CIRCLE('',#96611,0.800000000000001);
#19174=CIRCLE('',#96613,0.4);
#19175=CIRCLE('',#96614,0.4);
#19176=CIRCLE('',#96616,0.8);
#19177=CIRCLE('',#96617,0.8);
#19178=CIRCLE('',#96620,0.6);
#19179=CIRCLE('',#96623,4.);
#19180=CIRCLE('',#96624,4.);
#19181=CIRCLE('',#96626,0.8);
#19182=CIRCLE('',#96627,0.8);
#19183=CIRCLE('',#96629,4.2);
#19184=CIRCLE('',#96630,4.2);
#19185=CIRCLE('',#96632,1.55);
#19186=CIRCLE('',#96633,1.55);
#19187=CIRCLE('',#96635,0.4);
#19188=CIRCLE('',#96636,0.4);
#19189=CIRCLE('',#96638,0.75);
#19190=CIRCLE('',#96639,0.75);
#19191=CIRCLE('',#96643,1.3);
#19192=CIRCLE('',#96644,1.3);
#19193=CIRCLE('',#96646,2.5);
#19194=CIRCLE('',#96647,2.10000000000135);
#19195=CIRCLE('',#96650,1.3);
#19196=CIRCLE('',#96651,1.3);
#19197=CIRCLE('',#96653,2.5);
#19198=CIRCLE('',#96654,2.10000000000135);
#19199=CIRCLE('',#96658,2.09999999998101);
#19200=CIRCLE('',#96659,2.5);
#19201=CIRCLE('',#96661,2.09999999998101);
#19202=CIRCLE('',#96662,2.5);
#19203=CIRCLE('',#96665,2.5);
#19204=CIRCLE('',#96666,2.5);
#19205=CIRCLE('',#96670,2.5);
#19206=CIRCLE('',#96671,2.5);
#19207=CIRCLE('',#96674,2.5);
#19208=CIRCLE('',#96675,2.5);
#19209=CIRCLE('',#96677,2.5);
#19210=CIRCLE('',#96679,2.5);
#19211=CIRCLE('',#96680,2.5);
#19212=CIRCLE('',#96682,2.5);
#19213=CIRCLE('',#96685,1.3);
#19214=CIRCLE('',#96686,1.3);
#19215=CIRCLE('',#96691,1.3);
#19216=CIRCLE('',#96692,1.3);
#19217=CIRCLE('',#96701,0.6);
#19218=CIRCLE('',#96703,11.55);
#19219=CIRCLE('',#96706,3.6);
#19220=CIRCLE('',#96708,2.);
#19221=CIRCLE('',#96709,1.);
#19222=CIRCLE('',#96711,2.);
#19223=CIRCLE('',#96713,4.1);
#19224=CIRCLE('',#96716,0.6);
#19225=CIRCLE('',#96718,3.7);
#19226=CIRCLE('',#96721,0.6);
#19227=CIRCLE('',#96722,0.6);
#19228=CIRCLE('',#96724,0.6);
#19229=CIRCLE('',#96725,5.79999999999998);
#19230=CIRCLE('',#96727,0.6);
#19231=CIRCLE('',#96729,5.79999999999998);
#19232=CIRCLE('',#96731,0.6);
#19233=CIRCLE('',#96736,11.55);
#19234=CIRCLE('',#96738,0.6);
#19235=CIRCLE('',#96741,10.45);
#19236=CIRCLE('',#96742,10.45);
#19237=CIRCLE('',#96743,10.45);
#19238=CIRCLE('',#96746,10.35);
#19239=CIRCLE('',#96747,10.35);
#19240=CIRCLE('',#96748,10.35);
#19241=CIRCLE('',#96755,0.6);
#19242=CIRCLE('',#96757,0.599999999999999);
#19243=CIRCLE('',#96759,2.85);
#19244=CIRCLE('',#96760,3.2);
#19245=CIRCLE('',#96762,2.8);
#19246=CIRCLE('',#96763,2.8);
#19247=CIRCLE('',#96765,3.6);
#19248=CIRCLE('',#96766,3.6);
#19249=CIRCLE('',#96770,0.6);
#19250=CIRCLE('',#96772,6.4499999999938);
#19251=CIRCLE('',#96774,1.);
#19252=CIRCLE('',#96776,11.65);
#19253=CIRCLE('',#96778,4.15);
#19254=CIRCLE('',#96779,3.75);
#19255=CIRCLE('',#96781,2.4);
#19256=CIRCLE('',#96783,4.15);
#19257=CIRCLE('',#96785,2.1);
#19258=CIRCLE('',#96787,2.8);
#19259=CIRCLE('',#96788,2.8);
#19260=CIRCLE('',#96791,1.6);
#19261=CIRCLE('',#96792,1.6);
#19262=CIRCLE('',#96795,2.30000000000004);
#19263=CIRCLE('',#96796,2.);
#19264=CIRCLE('',#96798,2.);
#19265=CIRCLE('',#96800,0.4);
#19266=CIRCLE('',#96801,0.4);
#19267=CIRCLE('',#96803,10.35);
#19268=CIRCLE('',#96804,10.35);
#19269=CIRCLE('',#96806,0.75);
#19270=CIRCLE('',#96807,0.75);
#19271=CIRCLE('',#96809,10.);
#19272=CIRCLE('',#96812,0.4);
#19273=CIRCLE('',#96814,2.5);
#19274=CIRCLE('',#96816,3.1);
#19275=CIRCLE('',#96817,3.1);
#19276=CIRCLE('',#96820,2.5);
#19277=CIRCLE('',#96822,0.6);
#19278=CIRCLE('',#96824,4.);
#19279=CIRCLE('',#96826,4.9);
#19280=CIRCLE('',#96828,0.6);
#19281=CIRCLE('',#96830,1.55);
#19282=CIRCLE('',#96832,3.05);
#19283=CIRCLE('',#96833,2.);
#19284=CIRCLE('',#96835,1.55);
#19285=CIRCLE('',#96837,2.);
#19286=CIRCLE('',#96841,8.4949617393671);
#19287=CIRCLE('',#96842,9.3949617393671);
#19288=CIRCLE('',#96844,23.7449617393671);
#19289=CIRCLE('',#96845,23.7449617393671);
#19290=CIRCLE('',#96847,1.65);
#19291=CIRCLE('',#96851,2.1);
#19292=CIRCLE('',#96852,1.2);
#19293=CIRCLE('',#96854,1.);
#19294=CIRCLE('',#96855,1.);
#19295=CIRCLE('',#96857,2.8);
#19296=CIRCLE('',#96859,2.8);
#19297=CIRCLE('',#96864,5.35);
#19298=CIRCLE('',#96865,5.35);
#19299=CIRCLE('',#96866,5.35);
#19300=CIRCLE('',#96868,3.3);
#19301=CIRCLE('',#96869,3.3);
#19302=CIRCLE('',#96870,3.3);
#19303=CIRCLE('',#96873,2.2);
#19304=CIRCLE('',#96878,0.75);
#19305=CIRCLE('',#96881,3.6);
#19306=CIRCLE('',#96883,0.5);
#19307=CIRCLE('',#96885,0.4);
#19308=CIRCLE('',#96886,3.2);
#19309=CIRCLE('',#96888,3.2);
#19310=CIRCLE('',#96890,0.4);
#19311=CIRCLE('',#96892,0.400000000000005);
#19312=CIRCLE('',#96893,0.399999999999949);
#19313=CIRCLE('',#96895,0.4);
#19314=CIRCLE('',#96897,0.400000000000001);
#19315=CIRCLE('',#96898,0.4);
#19316=CIRCLE('',#96900,0.4);
#19317=CIRCLE('',#96901,0.400000000000003);
#19318=CIRCLE('',#96904,0.4);
#19319=CIRCLE('',#96906,2.8);
#19320=CIRCLE('',#96909,24.9449617393673);
#19321=CIRCLE('',#96912,0.399999999999997);
#19322=CIRCLE('',#96913,4.3);
#19323=CIRCLE('',#96915,4.3);
#19324=CIRCLE('',#96918,0.6);
#19325=CIRCLE('',#96920,4.1);
#19326=CIRCLE('',#96922,0.6);
#19327=CIRCLE('',#96925,1.);
#19328=CIRCLE('',#96926,1.);
#19329=CIRCLE('',#96928,2.5);
#19330=CIRCLE('',#96929,2.5);
#19331=CIRCLE('',#96932,1.);
#19332=CIRCLE('',#96933,1.);
#19333=CIRCLE('',#96935,17.3949617393671);
#19334=CIRCLE('',#96936,18.2949617393671);
#19335=CIRCLE('',#96938,4.8);
#19336=CIRCLE('',#96939,0.8);
#19337=CIRCLE('',#96941,0.6);
#19338=CIRCLE('',#96943,0.8);
#19339=CIRCLE('',#96946,0.800000000000001);
#19340=CIRCLE('',#96949,0.800000000000003);
#19341=CIRCLE('',#96950,0.8);
#19342=CIRCLE('',#96953,0.8);
#19343=CIRCLE('',#96956,0.8);
#19344=CIRCLE('',#96958,0.8);
#19345=CIRCLE('',#96959,7.8);
#19346=CIRCLE('',#96962,0.8);
#19347=CIRCLE('',#96964,0.8);
#19348=CIRCLE('',#96966,5.25);
#19349=CIRCLE('',#96967,5.25);
#19350=CIRCLE('',#96969,0.4);
#19351=CIRCLE('',#96970,7.8);
#19352=CIRCLE('',#96971,10.45);
#19353=CIRCLE('',#96973,0.4);
#19354=CIRCLE('',#96975,10.45);
#19355=CIRCLE('',#96976,10.45);
#19356=CIRCLE('',#96977,10.45);
#19357=CIRCLE('',#96979,0.4);
#19358=CIRCLE('',#96980,0.4);
#19359=CIRCLE('',#96982,3.05);
#19360=CIRCLE('',#96983,3.05);
#19361=CIRCLE('',#96985,3.25);
#19362=CIRCLE('',#96986,3.25);
#19363=CIRCLE('',#96990,0.2);
#19364=CIRCLE('',#96991,0.2);
#19365=CIRCLE('',#96992,0.6);
#19366=CIRCLE('',#96993,0.6);
#19367=CIRCLE('',#96994,0.6);
#19368=CIRCLE('',#96995,0.2);
#19369=CIRCLE('',#96996,0.2);
#19370=CIRCLE('',#96997,0.6);
#19371=CIRCLE('',#96998,0.6);
#19372=CIRCLE('',#96999,3.7);
#19373=CIRCLE('',#97000,0.4);
#19374=CIRCLE('',#97001,7.8);
#19375=CIRCLE('',#97002,4.8);
#19376=CIRCLE('',#97004,0.6);
#19377=CIRCLE('',#97022,0.2);
#19378=CIRCLE('',#97024,0.2);
#19379=CIRCLE('',#97026,0.2);
#19380=CIRCLE('',#97029,0.2);
#19381=CIRCLE('',#97039,0.299999999999997);
#19382=CIRCLE('',#97044,0.4);
#19383=CIRCLE('',#97049,0.6);
#19384=CIRCLE('',#97051,0.4);
#19385=CIRCLE('',#97053,10.6);
#19386=CIRCLE('',#97055,0.4);
#19387=CIRCLE('',#97057,0.4);
#19388=CIRCLE('',#97058,7.8);
#19389=CIRCLE('',#97060,0.4);
#19390=CIRCLE('',#97079,0.8);
#19391=CIRCLE('',#97080,0.800000000000001);
#19392=CIRCLE('',#97086,0.8);
#19393=CIRCLE('',#97088,0.8);
#23610=B_SPLINE_CURVE_WITH_KNOTS('',3,(#138846,#138847,#138848,#138849,
#138850,#138851,#138852),.UNSPECIFIED.,.F.,.F.,(4,1,1,1,4),(0.,0.0576772753326012,
0.115354550665202,0.173031825997804,0.403740927328209),.UNSPECIFIED.);
#23611=B_SPLINE_CURVE_WITH_KNOTS('',3,(#140166,#140167,#140168,#140169,
#140170,#140171,#140172,#140173,#140174,#140175,#140176,#140177,#140178,
#140179,#140180,#140181,#140182,#140183,#140184,#140185,#140186,#140187,
#140188,#140189,#140190,#140191,#140192,#140193,#140194,#140195,#140196),
 .UNSPECIFIED.,.F.,.F.,(4,3,3,3,3,3,3,3,3,3,4),(0.,0.00461311763943398,
0.0108962108513953,0.0174429809772217,0.0241024188265093,0.025565721040406,
0.0266315692284618,0.0334300723314571,0.0405906131676447,0.0477511540038322,
0.0479851889522872),.UNSPECIFIED.);
#23612=B_SPLINE_CURVE_WITH_KNOTS('',3,(#140198,#140199,#140200,#140201,
#140202,#140203,#140204,#140205,#140206),.UNSPECIFIED.,.F.,.F.,(4,1,1,1,
1,1,4),(0.461365642517441,0.594297668650691,0.72722969478394,0.793695707850564,
0.860161720917189,0.893394727450501,0.926627733983813),.UNSPECIFIED.);
#23613=B_SPLINE_CURVE_WITH_KNOTS('',3,(#140209,#140210,#140211,#140212,
#140213,#140214,#140215,#140216,#140217),.UNSPECIFIED.,.F.,.F.,(4,1,1,1,
1,1,4),(-0.926627733983813,-0.893394727450501,-0.860161720917189,-0.793695707850564,
-0.72722969478394,-0.594297668650691,-0.500154675194955),.UNSPECIFIED.);
#23614=B_SPLINE_CURVE_WITH_KNOTS('',3,(#140244,#140245,#140246,#140247,
#140248,#140249),.UNSPECIFIED.,.F.,.F.,(4,1,1,4),(-0.0834766168470346,-0.0596261548907622,
-0.0357756929344898,-8.11743420200643E-14),.UNSPECIFIED.);
#23615=B_SPLINE_CURVE_WITH_KNOTS('',3,(#140250,#140251,#140252,#140253,
#140254,#140255),.UNSPECIFIED.,.F.,.F.,(4,1,1,4),(8.11743420200643E-14,
0.0357756929344898,0.0596261548907622,0.0834766168470346),.UNSPECIFIED.);
#23616=B_SPLINE_CURVE_WITH_KNOTS('',3,(#140292,#140293,#140294,#140295,
#140296,#140297,#140298,#140299,#140300,#140301,#140302,#140303,#140304,
#140305,#140306,#140307,#140308,#140309,#140310,#140311,#140312,#140313,
#140314,#140315,#140316,#140317,#140318,#140319),.UNSPECIFIED.,.F.,.F.,
(4,3,3,3,3,3,3,3,3,4),(-0.000214859095644161,0.,0.00693142052454231,0.0137691687551713,
0.0194026267134537,0.0225967132655498,0.0291207852027703,0.0354961538326274,
0.0414739990602825,0.0439088685276748),.UNSPECIFIED.);
#23617=B_SPLINE_CURVE_WITH_KNOTS('',3,(#140320,#140321,#140322,#140323,
#140324,#140325,#140326),.UNSPECIFIED.,.F.,.F.,(4,1,1,1,4),(-0.368376389772111,
-0.173031825997804,-0.115354550665202,-0.0576772753326012,0.),
 .UNSPECIFIED.);
#23618=B_SPLINE_CURVE_WITH_KNOTS('',3,(#140341,#140342,#140343,#140344,
#140345,#140346),.UNSPECIFIED.,.F.,.F.,(4,2,4),(2.16893938526046,2.18932185224566,
2.29478437652477),.UNSPECIFIED.);
#23619=B_SPLINE_CURVE_WITH_KNOTS('',3,(#140350,#140351,#140352,#140353,
#140354,#140355,#140356),.UNSPECIFIED.,.F.,.F.,(4,3,4),(1.53576065525224,
1.55048490763555,1.65559071935948),.UNSPECIFIED.);
#23620=B_SPLINE_CURVE_WITH_KNOTS('',3,(#140372,#140373,#140374,#140375,
#140376,#140377),.UNSPECIFIED.,.F.,.F.,(4,2,4),(0.341286253546736,0.361143619795883,
0.363320956651565),.UNSPECIFIED.);
#23621=B_SPLINE_CURVE_WITH_KNOTS('',3,(#140378,#140379,#140380,#140381,
#140382,#140383),.UNSPECIFIED.,.F.,.F.,(4,2,4),(0.313750555620341,0.321428887297588,
0.341286253546736),.UNSPECIFIED.);
#23622=B_SPLINE_CURVE_WITH_KNOTS('',3,(#140980,#140981,#140982,#140983,
#140984,#140985,#140986,#140987,#140988,#140989),.UNSPECIFIED.,.F.,.F.,
(4,2,2,2,4),(1.67380554977791,1.72330946760875,1.82115803507338,1.91900660253801,
1.92968955045032),.UNSPECIFIED.);
#23623=B_SPLINE_CURVE_WITH_KNOTS('',3,(#140991,#140992,#140993,#140994,
#140995,#140996,#140997,#140998),.UNSPECIFIED.,.F.,.F.,(4,2,2,4),(1.16203916326871,
1.24446130754331,1.33480896870603,1.33871262848189),.UNSPECIFIED.);
#23624=B_SPLINE_CURVE_WITH_KNOTS('',3,(#141202,#141203,#141204,#141205,
#141206,#141207,#141208,#141209,#141210,#141211,#141212,#141213,#141214,
#141215),.UNSPECIFIED.,.F.,.F.,(4,2,2,2,2,2,4),(-0.0644438520828007,-0.049420098065367,
-0.0340805324627365,-0.0180381900027908,-0.00905381728536003,0.,0.000302476647115217),
 .UNSPECIFIED.);
#23625=B_SPLINE_CURVE_WITH_KNOTS('',3,(#141224,#141225,#141226,#141227,
#141228,#141229,#141230,#141231,#141232,#141233,#141234,#141235,#141236,
#141237),.UNSPECIFIED.,.F.,.F.,(4,2,2,2,2,2,4),(-0.0645192623114328,-0.0495220659688513,
-0.034197838940368,-0.0181427477062707,-0.00910662411509301,0.,0.000307206838262488),
 .UNSPECIFIED.);
#23626=B_SPLINE_CURVE_WITH_KNOTS('',3,(#141255,#141256,#141257,#141258,
#141259,#141260,#141261,#141262,#141263,#141264,#141265,#141266,#141267,
#141268),.UNSPECIFIED.,.F.,.F.,(4,2,2,2,2,2,4),(-0.076933286852498,-0.0656628947840389,
-0.0527777497222598,-0.0355412965898649,-0.0182549906540077,0.,0.000407112356477986),
 .UNSPECIFIED.);
#23627=B_SPLINE_CURVE_WITH_KNOTS('',3,(#141277,#141278,#141279,#141280,
#141281,#141282,#141283,#141284,#141285,#141286,#141287,#141288,#141289,
#141290,#141291,#141292),.UNSPECIFIED.,.F.,.F.,(4,2,2,2,2,2,2,4),(-0.17484883404941,
-0.17438352547713,-0.154057828687025,-0.134514112676025,-0.113669604374028,
-0.0979724065437587,-0.0842463799815946,-0.0840619732027956),
 .UNSPECIFIED.);
#23628=B_SPLINE_CURVE_WITH_KNOTS('',3,(#141318,#141319,#141320,#141321,
#141322,#141323,#141324,#141325,#141326,#141327,#141328,#141329),
 .UNSPECIFIED.,.F.,.F.,(4,2,2,2,2,4),(-0.000388459955655831,0.,0.0324366524825953,
0.0672148594225315,0.0883338786734475,0.0887070234931564),.UNSPECIFIED.);
#23629=B_SPLINE_CURVE_WITH_KNOTS('',3,(#141336,#141337,#141338,#141339,
#141340,#141341,#141342,#141343),.UNSPECIFIED.,.F.,.F.,(4,2,2,4),(0.209727352355126,
0.221639359053507,0.227267824689401,0.231641458293049),.UNSPECIFIED.);
#23630=B_SPLINE_CURVE_WITH_KNOTS('',3,(#141367,#141368,#141369,#141370,
#141371,#141372),.UNSPECIFIED.,.F.,.F.,(4,2,4),(-0.085422632899438,-0.0599779172305395,
-0.00660946384348909),.UNSPECIFIED.);
#23631=B_SPLINE_CURVE_WITH_KNOTS('',3,(#141376,#141377,#141378,#141379,
#141380,#141381,#141382,#141383,#141384,#141385,#141386,#141387,#141388,
#141389),.UNSPECIFIED.,.F.,.F.,(4,2,2,2,2,2,4),(0.000112134656694737,0.0132030014333664,
0.0271656495376335,0.0434063776045854,0.0557452168635409,0.0681403897390113,
0.0684503648574364),.UNSPECIFIED.);
#23632=B_SPLINE_CURVE_WITH_KNOTS('',3,(#141393,#141394,#141395,#141396,
#141397,#141398),.UNSPECIFIED.,.F.,.F.,(4,2,4),(0.0919390414530091,0.15020057139645,
0.150889093198151),.UNSPECIFIED.);
#23633=B_SPLINE_CURVE_WITH_KNOTS('',3,(#141403,#141404,#141405,#141406),
 .UNSPECIFIED.,.F.,.F.,(4,4),(0.324870734299899,0.389015211548213),
 .UNSPECIFIED.);
#23634=B_SPLINE_CURVE_WITH_KNOTS('',3,(#141410,#141411,#141412,#141413),
 .UNSPECIFIED.,.F.,.F.,(4,4),(1.82536907488932,1.86305287236042),
 .UNSPECIFIED.);
#23635=B_SPLINE_CURVE_WITH_KNOTS('',3,(#141421,#141422,#141423,#141424,
#141425,#141426),.UNSPECIFIED.,.F.,.F.,(4,2,4),(0.746025828133808,0.777852575214063,
0.79046455586539),.UNSPECIFIED.);
#23636=B_SPLINE_CURVE_WITH_KNOTS('',3,(#141428,#141429,#141430,#141431,
#141432,#141433),.UNSPECIFIED.,.F.,.F.,(4,2,4),(0.303437751782123,0.312479563833371,
0.470690179622201),.UNSPECIFIED.);
#23637=B_SPLINE_CURVE_WITH_KNOTS('',3,(#141435,#141436,#141437,#141438,
#141439,#141440,#141441,#141442,#141443,#141444,#141445,#141446,#141447,
#141448),.UNSPECIFIED.,.F.,.F.,(4,2,2,2,2,2,4),(1.16336684881612,1.24052856460303,
1.33090755793504,1.42128655126704,1.51166554459905,1.60204453793105,1.67920625371796),
 .UNSPECIFIED.);
#23638=B_SPLINE_CURVE_WITH_KNOTS('',3,(#141450,#141451,#141452,#141453),
 .UNSPECIFIED.,.F.,.F.,(4,4),(1.24043822694661,1.24960607382757),
 .UNSPECIFIED.);
#23639=B_SPLINE_CURVE_WITH_KNOTS('',3,(#141458,#141459,#141460,#141461,
#141462,#141463,#141464,#141465,#141466,#141467,#141468,#141469),
 .UNSPECIFIED.,.F.,.F.,(4,2,2,2,2,4),(0.10066778259603,0.120892907264577,
0.141118031933124,0.171226798562592,0.201335565192059,0.222479033048159),
 .UNSPECIFIED.);
#23640=B_SPLINE_CURVE_WITH_KNOTS('',3,(#141476,#141477,#141478,#141479,
#141480,#141481,#141482,#141483,#141484,#141485,#141486,#141487,#141488,
#141489,#141490),.UNSPECIFIED.,.F.,.F.,(4,2,2,3,2,2,4),(1.95413674175165,
1.9749623939079,2.06883224877398,2.18440456807724,2.27009756469335,2.3998891015239,
2.43069177712689),.UNSPECIFIED.);
#23641=B_SPLINE_CURVE_WITH_KNOTS('',3,(#141492,#141493,#141494,#141495,
#141496,#141497,#141498,#141499,#141500,#141501,#141502,#141503,#141504,
#141505,#141506),.UNSPECIFIED.,.F.,.F.,(4,2,2,3,2,2,4),(0.132343968988449,
0.206008897163555,0.279486022780957,0.290162010211257,0.448048634858984,
0.517599926787915,0.527299151805233),.UNSPECIFIED.);
#23642=B_SPLINE_CURVE_WITH_KNOTS('',3,(#141536,#141537,#141538,#141539,
#141540,#141541,#141542,#141543),.UNSPECIFIED.,.F.,.F.,(4,2,2,4),(-0.117541017236412,
-0.105671481013589,-0.0875214169518554,-0.0677213667893671),
 .UNSPECIFIED.);
#23643=B_SPLINE_CURVE_WITH_KNOTS('',3,(#141578,#141579,#141580,#141581,
#141582,#141583,#141584,#141585,#141586,#141587,#141588,#141589,#141590,
#141591),.UNSPECIFIED.,.F.,.F.,(4,2,2,2,2,2,4),(0.18312537356055,0.188512137502322,
0.20364370582247,0.220110749285725,0.236577792748981,0.260891780441132,
0.285205768133283),.UNSPECIFIED.);
#23644=B_SPLINE_CURVE_WITH_KNOTS('',3,(#141646,#141647,#141648,#141649,
#141650,#141651,#141652,#141653,#141654,#141655,#141656,#141657,#141658,
#141659,#141660,#141661),.UNSPECIFIED.,.F.,.F.,(4,2,2,2,2,2,2,4),(-0.000477658155061879,
0.,0.0247302092914747,0.0480741684085018,0.0685297927666644,0.0821332220389815,
0.0925411876291308,0.0950579615863738),.UNSPECIFIED.);
#23645=B_SPLINE_CURVE_WITH_KNOTS('',3,(#141733,#141734,#141735,#141736,
#141737,#141738,#141739,#141740,#141741,#141742),.UNSPECIFIED.,.F.,.F.,
(4,2,2,2,4),(0.13732942536332,0.150614929788285,0.166747654183265,0.186151203326564,
0.207424187379634),.UNSPECIFIED.);
#23646=B_SPLINE_CURVE_WITH_KNOTS('',3,(#141751,#141752,#141753,#141754),
 .UNSPECIFIED.,.F.,.F.,(4,4),(0.142599130795278,0.144346706380812),
 .UNSPECIFIED.);
#23647=B_SPLINE_CURVE_WITH_KNOTS('',3,(#141758,#141759,#141760,#141761),
 .UNSPECIFIED.,.F.,.F.,(4,4),(0.00025811192102492,0.00165664283540655),
 .UNSPECIFIED.);
#23648=B_SPLINE_CURVE_WITH_KNOTS('',3,(#141763,#141764,#141765,#141766,
#141767,#141768,#141769,#141770,#141771,#141772,#141773,#141774,#141775,
#141776),.UNSPECIFIED.,.F.,.F.,(4,2,2,2,2,2,4),(-0.000346312484341596,0.,
0.0150312784786187,0.0297106940471177,0.0467215668210816,0.0602423017367392,
0.0722722728378001),.UNSPECIFIED.);
#23649=B_SPLINE_CURVE_WITH_KNOTS('',3,(#141780,#141781,#141782,#141783,
#141784,#141785,#141786,#141787),.UNSPECIFIED.,.F.,.F.,(4,2,2,4),(0.0136627898201133,
0.125132828407067,0.152540787048518,0.156243805314172),.UNSPECIFIED.);
#23650=B_SPLINE_CURVE_WITH_KNOTS('',3,(#141789,#141790,#141791,#141792,
#141793,#141794,#141795,#141796),.UNSPECIFIED.,.F.,.F.,(4,2,2,4),(0.00660661411091279,
0.14470344735553,0.251350868103014,0.347057593360392),.UNSPECIFIED.);
#23651=B_SPLINE_CURVE_WITH_KNOTS('',3,(#141797,#141798,#141799,#141800,
#141801,#141802,#141803,#141804,#141805,#141806,#141807,#141808,#141809,
#141810),.UNSPECIFIED.,.F.,.F.,(4,2,2,2,2,2,4),(-0.107017806276282,-0.0978369539163657,
-0.0882519488889954,-0.0704169759838092,-0.0478776048900307,-0.0237745956474009,
-0.0129771129663482),.UNSPECIFIED.);
#23652=B_SPLINE_CURVE_WITH_KNOTS('',3,(#141904,#141905,#141906,#141907,
#141908,#141909,#141910,#141911,#141912),.UNSPECIFIED.,.F.,.F.,(4,2,3,4),
(0.828293167562194,0.869881225451604,0.954778354838245,0.973139317003065),
 .UNSPECIFIED.);
#23653=B_SPLINE_CURVE_WITH_KNOTS('',3,(#141946,#141947,#141948,#141949,
#141950,#141951,#141952,#141953,#141954,#141955,#141956,#141957,#141958,
#141959,#141960,#141961,#141962,#141963,#141964,#141965,#141966,#141967,
#141968,#141969,#141970),.UNSPECIFIED.,.F.,.F.,(4,2,2,2,2,2,2,2,2,2,3,4),
(1.15977853242372,1.20026581496982,1.28836339099528,1.37646096702074,1.45628348069954,
1.53610599437834,1.61592850805714,1.69575102173595,1.78384859776141,1.87194617378687,
2.04246365813963,2.06103131106925),.UNSPECIFIED.);
#23654=B_SPLINE_CURVE_WITH_KNOTS('',3,(#141982,#141983,#141984,#141985,
#141986,#141987),.UNSPECIFIED.,.F.,.F.,(4,2,4),(0.,0.0366955352357751,0.0584007125994646),
 .UNSPECIFIED.);
#23655=B_SPLINE_CURVE_WITH_KNOTS('',3,(#141989,#141990,#141991,#141992,
#141993,#141994,#141995,#141996,#141997,#141998,#141999,#142000,#142001,
#142002,#142003,#142004,#142005,#142006,#142007,#142008,#142009,#142010,
#142011,#142012),.UNSPECIFIED.,.F.,.F.,(4,2,2,2,2,2,2,2,2,2,2,4),(0.603586482438603,
0.690548157104178,0.7776775531107,0.814909478184255,0.841789702690823,0.855229814944108,
0.868669927197392,0.882110039450676,0.89555015170396,0.922430376210528,
0.959662301284084,0.988423011761695),.UNSPECIFIED.);
#23656=B_SPLINE_CURVE_WITH_KNOTS('',3,(#142014,#142015,#142016,#142017,
#142018,#142019,#142020,#142021,#142022,#142023,#142024,#142025,#142026),
 .UNSPECIFIED.,.F.,.F.,(4,3,3,3,4),(0.,0.00510825104781711,0.00881483564204352,
0.0138582618694087,0.0184324970853374),.UNSPECIFIED.);
#23657=B_SPLINE_CURVE_WITH_KNOTS('',3,(#142451,#142452,#142453,#142454,
#142455,#142456,#142457,#142458,#142459,#142460,#142461,#142462,#142463),
 .UNSPECIFIED.,.F.,.F.,(4,3,3,3,4),(0.,0.00495757901231158,0.00803114212030837,
0.0131782094120615,0.0156274267007913),.UNSPECIFIED.);
#23658=B_SPLINE_CURVE_WITH_KNOTS('',3,(#142465,#142466,#142467,#142468,
#142469,#142470,#142471,#142472,#142473,#142474,#142475,#142476,#142477,
#142478,#142479,#142480,#142481,#142482,#142483,#142484,#142485,#142486,
#142487,#142488,#142489,#142490,#142491,#142492),.UNSPECIFIED.,.F.,.F.,
(4,2,2,2,2,3,2,2,2,2,3,2,4),(1.57820587984966,1.64634748030809,1.68357940538165,
1.71045962988822,1.7238997421415,1.73733985439478,1.75515538094126,1.77739368952689,
1.81480798197786,1.90628850472617,1.92355226704702,1.99122268110966,2.03565025170069),
 .UNSPECIFIED.);
#23659=B_SPLINE_CURVE_WITH_KNOTS('',3,(#142494,#142495,#142496,#142497,
#142498,#142499,#142500,#142501,#142502,#142503,#142504,#142505,#142506,
#142507,#142508,#142509,#142510,#142511,#142512,#142513,#142514,#142515,
#142516,#142517,#142518),.UNSPECIFIED.,.F.,.F.,(4,3,3,3,3,3,3,3,4),(0.,
0.00579507786607313,0.00734016029473464,0.0138775194884377,0.0157142860932645,
0.0230358256114078,0.0255587459307486,0.0326896693983427,0.0375637041363583),
 .UNSPECIFIED.);
#23660=B_SPLINE_CURVE_WITH_KNOTS('',3,(#142541,#142542,#142543,#142544,
#142545,#142546,#142547,#142548,#142549,#142550,#142551,#142552,#142553,
#142554),.UNSPECIFIED.,.F.,.F.,(4,2,2,2,2,2,4),(-0.0758814738778919,-0.0645512346483667,
-0.0515933744670232,-0.0342983873642865,-0.0175181259639588,0.,0.000393270258763866),
 .UNSPECIFIED.);
#23661=B_SPLINE_CURVE_WITH_KNOTS('',3,(#142610,#142611,#142612,#142613),
 .UNSPECIFIED.,.F.,.F.,(4,4),(0.239784037589408,0.24117260623475),
 .UNSPECIFIED.);
#23662=B_SPLINE_CURVE_WITH_KNOTS('',3,(#142639,#142640,#142641,#142642,
#142643,#142644,#142645,#142646,#142647,#142648,#142649,#142650,#142651,
#142652,#142653,#142654,#142655),.UNSPECIFIED.,.F.,.F.,(4,3,2,2,2,2,2,4),
(-0.0128577538036982,0.00567052604397339,0.139467562250634,0.278935124501267,
0.421402366816533,0.563869609131798,0.720032639200108,0.790946603218797),
 .UNSPECIFIED.);
#23663=B_SPLINE_CURVE_WITH_KNOTS('',3,(#142664,#142665,#142666,#142667,
#142668,#142669,#142670,#142671,#142672,#142673),.UNSPECIFIED.,.F.,.F.,
(4,2,2,2,4),(0.603059033985991,0.640749534408183,0.678440034830375,0.716154939786789,
0.753869844743204),.UNSPECIFIED.);
#23664=B_SPLINE_CURVE_WITH_KNOTS('',3,(#142677,#142678,#142679,#142680,
#142681,#142682,#142683,#142684,#142685,#142686,#142687,#142688,#142689,
#142690,#142691,#142692,#142693,#142694),.UNSPECIFIED.,.F.,.F.,(4,2,2,2,
2,2,2,2,4),(0.,0.0939769400668632,0.187953880133726,0.285086724461635,0.382219568789543,
0.485399452153548,0.588579335517553,0.683402310815935,0.778225286114316),
 .UNSPECIFIED.);
#23665=B_SPLINE_CURVE_WITH_KNOTS('',3,(#142698,#142699,#142700,#142701,
#142702,#142703,#142704,#142705,#142706,#142707),.UNSPECIFIED.,.F.,.F.,
(4,2,2,2,4),(-0.168397624102938,-0.121332479144638,-0.074267334186339,-0.0371336670931696,
0.),.UNSPECIFIED.);
#23666=B_SPLINE_CURVE_WITH_KNOTS('',3,(#142713,#142714,#142715,#142716,
#142717,#142718,#142719,#142720,#142721,#142722,#142723,#142724),
 .UNSPECIFIED.,.F.,.F.,(4,2,2,2,2,4),(1.37984672511584,1.40611061616659,
1.50164662943263,1.59718264269866,1.71238091394357,1.79261814476496),
 .UNSPECIFIED.);
#23667=B_SPLINE_CURVE_WITH_KNOTS('',3,(#142912,#142913,#142914,#142915,
#142916,#142917,#142918,#142919,#142920,#142921,#142922,#142923,#142924,
#142925),.UNSPECIFIED.,.F.,.F.,(4,2,2,2,2,2,4),(-0.142919155679814,-0.142584878197208,
-0.131628599743153,-0.109600735717745,-0.0922149909757629,-0.0785268178472592,
-0.0721276294223837),.UNSPECIFIED.);
#23668=B_SPLINE_CURVE_WITH_KNOTS('',3,(#143028,#143029,#143030,#143031,
#143032,#143033,#143034,#143035,#143036,#143037,#143038,#143039,#143040,
#143041),.UNSPECIFIED.,.F.,.F.,(4,2,2,2,2,2,4),(-0.144508400855472,-0.144147613097621,
-0.129519379467225,-0.115275397220758,-0.098017254785151,-0.0843295892561403,
-0.0720738065488153),.UNSPECIFIED.);
#23669=B_SPLINE_CURVE_WITH_KNOTS('',3,(#143046,#143047,#143048,#143049),
 .UNSPECIFIED.,.F.,.F.,(4,4),(0.126555917274389,0.127955709526028),
 .UNSPECIFIED.);
#23670=B_SPLINE_CURVE_WITH_KNOTS('',3,(#143051,#143052,#143053,#143054,
#143055,#143056),.UNSPECIFIED.,.F.,.F.,(4,2,4),(0.12515823369475,0.125586430963453,
0.12655591727435),.UNSPECIFIED.);
#23671=B_SPLINE_CURVE_WITH_KNOTS('',3,(#143068,#143069,#143070,#143071,
#143072,#143073,#143074,#143075,#143076,#143077,#143078,#143079,#143080,
#143081,#143082,#143083,#143084,#143085,#143086,#143087,#143088,#143089,
#143090,#143091,#143092,#143093,#143094,#143095),.UNSPECIFIED.,.F.,.F.,
(4,3,2,2,2,2,2,2,2,2,2,3,4),(1.00649313055325,1.02506097707024,1.19486303676886,
1.28260286113604,1.37034268550322,1.44970888377749,1.52907508205176,1.60844128032603,
1.68780747860031,1.77554730296748,1.86328712733466,2.03308918703329,2.05164843706349),
 .UNSPECIFIED.);
#23672=B_SPLINE_CURVE_WITH_KNOTS('',3,(#143109,#143110,#143111,#143112,
#143113,#143114,#143115,#143116,#143117,#143118,#143119,#143120,#143121,
#143122,#143123,#143124,#143125,#143126,#143127),.UNSPECIFIED.,.F.,.F.,
(4,3,3,3,3,3,4),(0.,0.00601946685722754,0.0114877407859627,0.0130556988279324,
0.0185846512727586,0.0238133106387385,0.0241136037175848),.UNSPECIFIED.);
#23673=B_SPLINE_CURVE_WITH_KNOTS('',3,(#143129,#143130,#143131,#143132,
#143133,#143134,#143135,#143136,#143137,#143138,#143139,#143140,#143141,
#143142),.UNSPECIFIED.,.F.,.F.,(4,2,2,2,2,2,4),(2.23207184191967,2.29687645546178,
2.38015427484409,2.41565949974496,2.44114532275338,2.45388823425759,2.4666311457618),
 .UNSPECIFIED.);
#23674=B_SPLINE_CURVE_WITH_KNOTS('',3,(#143144,#143145,#143146,#143147,
#143148,#143149,#143150,#143151,#143152,#143153,#143154,#143155),
 .UNSPECIFIED.,.F.,.F.,(4,2,2,2,2,4),(2.4666311457618,2.47937405726601,
2.49211696877022,2.51760279177863,2.55310801667951,2.57292617100586),
 .UNSPECIFIED.);
#23675=B_SPLINE_CURVE_WITH_KNOTS('',3,(#143157,#143158,#143159,#143160,
#143161,#143162,#143163),.UNSPECIFIED.,.F.,.F.,(4,3,4),(-2.6313632032836E-5,
0.00282304343927375,0.00571245680678869),.UNSPECIFIED.);
#23676=B_SPLINE_CURVE_WITH_KNOTS('',3,(#143313,#143314,#143315,#143316,
#143317,#143318),.UNSPECIFIED.,.F.,.F.,(4,2,4),(0.,0.0412614986637767,0.0652763436524788),
 .UNSPECIFIED.);
#23677=B_SPLINE_CURVE_WITH_KNOTS('',3,(#143320,#143321,#143322,#143323,
#143324,#143325,#143326,#143327,#143328,#143329,#143330,#143331),
 .UNSPECIFIED.,.F.,.F.,(4,2,2,2,2,4),(1.53706718335664,1.55794389292349,
1.59344911782436,1.61893494083278,1.63167785233699,1.6444207638412),
 .UNSPECIFIED.);
#23678=B_SPLINE_CURVE_WITH_KNOTS('',3,(#143333,#143334,#143335,#143336,
#143337,#143338,#143339,#143340,#143341,#143342,#143343,#143344,#143345,
#143346),.UNSPECIFIED.,.F.,.F.,(4,2,2,2,2,2,4),(1.6444207638412,1.65716367534541,
1.66990658684962,1.69539240985803,1.73089763475891,1.81417545414122,1.90238360165616),
 .UNSPECIFIED.);
#23679=B_SPLINE_CURVE_WITH_KNOTS('',3,(#143348,#143349,#143350,#143351,
#143352,#143353),.UNSPECIFIED.,.F.,.F.,(4,2,4),(0.,0.00532881829401623,
0.0217063037167981),.UNSPECIFIED.);
#23680=B_SPLINE_CURVE_WITH_KNOTS('',3,(#143556,#143557,#143558,#143559,
#143560,#143561,#143562,#143563,#143564,#143565,#143566,#143567,#143568,
#143569,#143570,#143571,#143572,#143573),.UNSPECIFIED.,.F.,.F.,(4,2,2,2,
2,2,2,2,4),(0.,0.0948259003515225,0.189651800703045,0.292563142700536,0.395474484698028,
0.492438634253719,0.589402783809411,0.683398079037316,0.777393374265221),
 .UNSPECIFIED.);
#23681=B_SPLINE_CURVE_WITH_KNOTS('',3,(#143577,#143578,#143579,#143580,
#143581,#143582,#143583,#143584,#143585,#143586,#143587,#143588,#143589,
#143590,#143591,#143592,#143593,#143594),.UNSPECIFIED.,.F.,.F.,(4,2,2,2,
2,2,2,2,4),(0.,0.0944195222117657,0.188839044423531,0.286064822200348,0.383290599977165,
0.488790377679475,0.594290155381785,0.689433686163349,0.784577216944913),
 .UNSPECIFIED.);
#23682=B_SPLINE_CURVE_WITH_KNOTS('',3,(#143600,#143601,#143602,#143603,
#143604,#143605,#143606,#143607,#143608,#143609,#143610,#143611,#143612,
#143613,#143614,#143615,#143616,#143617),.UNSPECIFIED.,.F.,.F.,(4,2,2,2,
2,2,2,2,4),(0.,0.098362147606416,0.196724295212832,0.299373551861381,0.40202280850993,
0.499926681532627,0.597830554555324,0.691757138564027,0.785683722572729),
 .UNSPECIFIED.);
#23683=B_SPLINE_CURVE_WITH_KNOTS('',3,(#143801,#143802,#143803,#143804,
#143805,#143806,#143807,#143808,#143809,#143810),.UNSPECIFIED.,.F.,.F.,
(4,2,2,2,4),(0.189270674477839,0.211763257145919,0.234255839813999,0.258231413480196,
0.282206987146393),.UNSPECIFIED.);
#23684=B_SPLINE_CURVE_WITH_KNOTS('',3,(#143813,#143814,#143815,#143816,
#143817,#143818,#143819,#143820,#143821,#143822,#143823,#143824,#143825,
#143826),.UNSPECIFIED.,.F.,.F.,(4,2,2,2,2,2,4),(0.18925639316843,0.212017765594377,
0.234779138020324,0.258485907400251,0.282192676780179,0.306887761301932,
0.326562144225016),.UNSPECIFIED.);
#23685=B_SPLINE_CURVE_WITH_KNOTS('',3,(#143842,#143843,#143844,#143845,
#143846,#143847,#143848,#143849,#143850,#143851,#143852,#143853,#143854,
#143855),.UNSPECIFIED.,.F.,.F.,(4,2,2,2,2,2,4),(0.241932234759915,0.261279320323699,
0.286037147223808,0.309784118650402,0.333531090076996,0.356299951830059,
0.379068813583121),.UNSPECIFIED.);
#23686=B_SPLINE_CURVE_WITH_KNOTS('',3,(#143875,#143876,#143877,#143878,
#143879,#143880,#143881,#143882,#143883,#143884),.UNSPECIFIED.,.F.,.F.,
(4,2,2,2,4),(0.286037128270882,0.310064366617074,0.334091604963267,0.3565802092733,
0.379068813583334),.UNSPECIFIED.);
#23687=B_SPLINE_CURVE_WITH_KNOTS('',3,(#143886,#143887,#143888,#143889,
#143890,#143891,#143892,#143893,#143894,#143895),.UNSPECIFIED.,.F.,.F.,
(4,2,2,2,4),(1.01847209163261,1.09614224834082,1.21102278725762,1.30659119635196,
1.40215960544631),.UNSPECIFIED.);
#23688=B_SPLINE_CURVE_WITH_KNOTS('',3,(#143909,#143910,#143911,#143912,
#143913,#143914,#143915,#143916,#143917,#143918,#143919,#143920,#143921,
#143922,#143923,#143924,#143925),.UNSPECIFIED.,.F.,.F.,(4,2,2,2,3,2,2,4),
(0.928216827061862,0.932389730285405,0.992769022880904,1.0531483154764,
1.1739069006674,1.2946654858584,1.3550447784539,1.39738911925677),
 .UNSPECIFIED.);
#23689=B_SPLINE_CURVE_WITH_KNOTS('',3,(#143951,#143952,#143953,#143954,
#143955,#143956),.UNSPECIFIED.,.F.,.F.,(4,2,4),(0.104086067281323,0.108489006128221,
0.168304783933614),.UNSPECIFIED.);
#23690=B_SPLINE_CURVE_WITH_KNOTS('',3,(#143958,#143959,#143960,#143961,
#143962,#143963,#143964,#143965,#143966,#143967,#143968,#143969),
 .UNSPECIFIED.,.F.,.F.,(4,2,2,2,2,4),(0.371222277774226,0.439583636064719,
0.595306530197309,0.737554434553936,0.879802338910563,0.949739845591811),
 .UNSPECIFIED.);
#23691=B_SPLINE_CURVE_WITH_KNOTS('',3,(#143970,#143971,#143972,#143973,
#143974,#143975),.UNSPECIFIED.,.F.,.F.,(4,2,4),(0.0529943431633899,0.0577411969641437,
0.162437857102921),.UNSPECIFIED.);
#23692=B_SPLINE_CURVE_WITH_KNOTS('',3,(#143995,#143996,#143997,#143998,
#143999,#144000,#144001,#144002),.UNSPECIFIED.,.F.,.F.,(4,2,2,4),(0.454924391717627,
0.46478463553666,0.487557239675925,0.503332474617141),.UNSPECIFIED.);
#23693=B_SPLINE_CURVE_WITH_KNOTS('',3,(#144013,#144014,#144015,#144016,
#144017,#144018,#144019,#144020,#144021,#144022),.UNSPECIFIED.,.F.,.F.,
(4,2,2,2,4),(0.301557475483223,0.33925269209598,0.376947908708738,0.414656148075488,
0.452364387442238),.UNSPECIFIED.);
#23694=B_SPLINE_CURVE_WITH_KNOTS('',3,(#144024,#144025,#144026,#144027,
#144028,#144029,#144030,#144031),.UNSPECIFIED.,.F.,.F.,(4,2,2,4),(-0.108303883771064,
-0.0753798988372107,-0.0376899494186054,0.),.UNSPECIFIED.);
#23695=B_SPLINE_CURVE_WITH_KNOTS('',3,(#144040,#144041,#144042,#144043,
#144044,#144045,#144046,#144047,#144048,#144049),.UNSPECIFIED.,.F.,.F.,
(4,2,2,2,4),(0.344103183736344,0.381242716027575,0.418382248318806,0.465288723179234,
0.512195198039662),.UNSPECIFIED.);
#23696=B_SPLINE_CURVE_WITH_KNOTS('',3,(#144061,#144062,#144063,#144064,
#144065,#144066,#144067,#144068,#144069,#144070),.UNSPECIFIED.,.F.,.F.,
(4,2,2,2,4),(0.363197033462642,0.4031110869448,0.443025140426958,0.490684930222813,
0.538344720018669),.UNSPECIFIED.);
#23697=B_SPLINE_CURVE_WITH_KNOTS('',3,(#144074,#144075,#144076,#144077,
#144078,#144079,#144080,#144081,#144082,#144083),.UNSPECIFIED.,.F.,.F.,
(4,2,2,2,4),(0.150729427408656,0.188455603969964,0.226181780531272,0.263877644175159,
0.301573507819046),.UNSPECIFIED.);
#23698=B_SPLINE_CURVE_WITH_KNOTS('',3,(#144089,#144090,#144091,#144092,
#144093,#144094,#144095,#144096,#144097,#144098),.UNSPECIFIED.,.F.,.F.,
(4,2,2,2,4),(0.550254856554737,0.59775876613801,0.645262675721284,0.685134618848566,
0.725006561975848),.UNSPECIFIED.);
#23699=B_SPLINE_CURVE_WITH_KNOTS('',3,(#144118,#144119,#144120,#144121,
#144122,#144123,#144124,#144125,#144126,#144127,#144128,#144129,#144130),
 .UNSPECIFIED.,.F.,.F.,(4,2,2,2,3,4),(-0.100223122044128,-0.0800989314803924,
-0.0599747409166565,-0.0299873704583282,0.,0.0243767134003336),
 .UNSPECIFIED.);
#23700=B_SPLINE_CURVE_WITH_KNOTS('',3,(#144138,#144139,#144140,#144141,
#144142,#144143,#144144,#144145,#144146,#144147,#144148,#144149),
 .UNSPECIFIED.,.F.,.F.,(4,2,2,2,2,4),(0.21639017325191,0.239839563382432,
0.26982693384076,0.299814304299088,0.319938494862824,0.34006268542656),
 .UNSPECIFIED.);
#23701=B_SPLINE_CURVE_WITH_KNOTS('',3,(#144156,#144157,#144158,#144159,
#144160,#144161),.UNSPECIFIED.,.F.,.F.,(4,2,4),(1.4463380141481,1.46636753961024,
1.5045533789501),.UNSPECIFIED.);
#23702=B_SPLINE_CURVE_WITH_KNOTS('',3,(#144163,#144164,#144165,#144166),
 .UNSPECIFIED.,.F.,.F.,(4,4),(2.02040063642927,2.03639014323659),
 .UNSPECIFIED.);
#23703=B_SPLINE_CURVE_WITH_KNOTS('',3,(#144169,#144170,#144171,#144172,
#144173,#144174,#144175,#144176,#144177,#144178,#144179,#144180,#144181,
#144182,#144183),.UNSPECIFIED.,.F.,.F.,(4,2,2,2,3,2,4),(0.225773787410195,
0.239394753865059,0.253015720319924,0.273253708378096,0.293491696436268,
0.315181887462217,0.333911176073498),.UNSPECIFIED.);
#23704=B_SPLINE_CURVE_WITH_KNOTS('',3,(#144185,#144186,#144187,#144188,
#144189,#144190,#144191,#144192,#144193,#144194,#144195,#144196,#144197,
#144198,#144199),.UNSPECIFIED.,.F.,.F.,(4,2,2,2,3,2,4),(-0.068263214221219,
-0.0545185069182086,-0.0407737996151983,-0.0203868998075991,0.,0.0215381797259622,
0.0362085650374704),.UNSPECIFIED.);
#23705=B_SPLINE_CURVE_WITH_KNOTS('',3,(#144207,#144208,#144209,#144210,
#144211,#144212,#144213,#144214,#144215,#144216,#144217,#144218,#144219,
#144220,#144221,#144222),.UNSPECIFIED.,.F.,.F.,(4,2,2,2,2,2,2,4),(0.763245415685139,
0.772656167228652,0.890067929002265,1.00747969077588,1.12489145254949,1.2423032143231,
1.34066137334052,1.34318636064082),.UNSPECIFIED.);
#23706=B_SPLINE_CURVE_WITH_KNOTS('',3,(#144234,#144235,#144236,#144237),
 .UNSPECIFIED.,.F.,.F.,(4,4),(1.52365417396437,1.52591840699516),
 .UNSPECIFIED.);
#23707=B_SPLINE_CURVE_WITH_KNOTS('',3,(#144238,#144239,#144240,#144241),
 .UNSPECIFIED.,.F.,.F.,(4,4),(1.80468312171546,1.87869184978489),
 .UNSPECIFIED.);
#23708=B_SPLINE_CURVE_WITH_KNOTS('',3,(#144242,#144243,#144244,#144245),
 .UNSPECIFIED.,.F.,.F.,(4,4),(6.05153047053036,6.12780351388147),
 .UNSPECIFIED.);
#23709=B_SPLINE_CURVE_WITH_KNOTS('',3,(#144249,#144250,#144251,#144252,
#144253,#144254,#144255,#144256,#144257,#144258,#144259,#144260,#144261,
#144262,#144263,#144264),.UNSPECIFIED.,.F.,.F.,(4,2,2,2,2,2,2,4),(0.156606736308253,
0.180805448767024,0.20508734783811,0.217228297373654,0.229369246909197,
0.24151019644474,0.253651145980283,0.264578837334174),.UNSPECIFIED.);
#23710=B_SPLINE_CURVE_WITH_KNOTS('',3,(#144276,#144277,#144278,#144279,
#144280,#144281),.UNSPECIFIED.,.F.,.F.,(4,2,4),(2.05087433026329,2.07604853698334,
2.22480786223231),.UNSPECIFIED.);
#23711=B_SPLINE_CURVE_WITH_KNOTS('',3,(#144283,#144284,#144285,#144286,
#144287,#144288),.UNSPECIFIED.,.F.,.F.,(4,2,4),(3.23765002225092,3.43215209198459,
3.58086556096453),.UNSPECIFIED.);
#23712=B_SPLINE_CURVE_WITH_KNOTS('',3,(#144290,#144291,#144292,#144293,
#144294,#144295,#144296,#144297),.UNSPECIFIED.,.F.,.F.,(4,2,2,4),(0.193941715876439,
0.365833717405826,0.459726527436784,0.496146962294632),.UNSPECIFIED.);
#23713=B_SPLINE_CURVE_WITH_KNOTS('',3,(#144298,#144299,#144300,#144301,
#144302,#144303,#144304,#144305),.UNSPECIFIED.,.F.,.F.,(4,2,2,4),(1.19119064358888,
1.25304900366289,1.35089757112752,1.40777544238509),.UNSPECIFIED.);
#23714=B_SPLINE_CURVE_WITH_KNOTS('',3,(#144308,#144309,#144310,#144311,
#144312,#144313,#144314,#144315,#144316,#144317,#144318,#144319,#144320,
#144321),.UNSPECIFIED.,.F.,.F.,(4,2,2,2,2,2,4),(0.0724967244197842,0.0766714820213276,
0.114986644138398,0.153301806255469,0.19149984850442,0.229697890753371,
0.234669900956502),.UNSPECIFIED.);
#23715=B_SPLINE_CURVE_WITH_KNOTS('',3,(#144327,#144328,#144329,#144330),
 .UNSPECIFIED.,.F.,.F.,(4,4),(1.62317914932141,1.69306789581112),
 .UNSPECIFIED.);
#23716=B_SPLINE_CURVE_WITH_KNOTS('',3,(#144332,#144333,#144334,#144335,
#144336,#144337),.UNSPECIFIED.,.F.,.F.,(4,2,4),(0.410526643667809,0.556855217300137,
0.576452875080128),.UNSPECIFIED.);
#23717=B_SPLINE_CURVE_WITH_KNOTS('',3,(#144338,#144339,#144340,#144341,
#144342,#144343),.UNSPECIFIED.,.F.,.F.,(4,2,4),(0.257017510558728,0.263940899519207,
0.300168261034611),.UNSPECIFIED.);
#23718=B_SPLINE_CURVE_WITH_KNOTS('',3,(#144369,#144370,#144371,#144372,
#144373,#144374,#144375,#144376,#144377,#144378),.UNSPECIFIED.,.F.,.F.,
(4,2,2,2,4),(1.31489350131146,1.33456157653928,1.41236011898755,1.49015866143582,
1.50084837281906),.UNSPECIFIED.);
#23719=B_SPLINE_CURVE_WITH_KNOTS('',3,(#144388,#144389,#144390,#144391,
#144392,#144393,#144394,#144395,#144396,#144397,#144398,#144399,#144400),
 .UNSPECIFIED.,.F.,.F.,(4,3,2,2,2,4),(0.417573720644144,0.440269087673341,
0.470377854302809,0.500486620932276,0.520711745600823,0.540936870269371),
 .UNSPECIFIED.);
#23720=B_SPLINE_CURVE_WITH_KNOTS('',3,(#144455,#144456,#144457,#144458,
#144459,#144460),.UNSPECIFIED.,.F.,.F.,(4,2,4),(1.28130036614749,1.3304475484929,
1.37533827653421),.UNSPECIFIED.);
#23721=B_SPLINE_CURVE_WITH_KNOTS('',3,(#144462,#144463,#144464,#144465,
#144466,#144467,#144468,#144469),.UNSPECIFIED.,.F.,.F.,(4,2,2,4),(0.372364396932915,
0.435374241191316,0.532988843711153,0.599542108482719),.UNSPECIFIED.);
#23722=B_SPLINE_CURVE_WITH_KNOTS('',3,(#144483,#144484,#144485,#144486,
#144487,#144488,#144489,#144490,#144491,#144492,#144493),.UNSPECIFIED.,
 .F.,.F.,(4,2,3,2,4),(-0.149195468638109,-0.0954898081619349,0.,0.105194370875322,
0.138905665786208),.UNSPECIFIED.);
#23723=B_SPLINE_CURVE_WITH_KNOTS('',3,(#144509,#144510,#144511,#144512),
 .UNSPECIFIED.,.F.,.F.,(4,4),(2.8612825744839,2.89469550090435),
 .UNSPECIFIED.);
#23724=B_SPLINE_CURVE_WITH_KNOTS('',3,(#144565,#144566,#144567,#144568,
#144569,#144570),.UNSPECIFIED.,.F.,.F.,(4,2,4),(2.59711974020287,2.67846990390876,
2.74436889115826),.UNSPECIFIED.);
#23725=B_SPLINE_CURVE_WITH_KNOTS('',3,(#144573,#144574,#144575,#144576,
#144577,#144578,#144579,#144580,#144581,#144582,#144583,#144584,#144585),
 .UNSPECIFIED.,.F.,.F.,(4,2,2,2,3,4),(0.3424697429409,0.362070187841933,
0.381670632742966,0.411028407725618,0.440386182708269,0.473071910942229),
 .UNSPECIFIED.);
#23726=B_SPLINE_CURVE_WITH_KNOTS('',3,(#144587,#144588,#144589,#144590,
#144591,#144592),.UNSPECIFIED.,.F.,.F.,(4,2,4),(6.1917354885447,6.24887728986414,
6.34659932277937),.UNSPECIFIED.);
#23727=B_SPLINE_CURVE_WITH_KNOTS('',3,(#144596,#144597,#144598,#144599,
#144600,#144601,#144602,#144603,#144604,#144605,#144606,#144607,#144608),
 .UNSPECIFIED.,.F.,.F.,(4,3,2,2,2,4),(0.40770045386894,0.440386182708269,
0.46974395769092,0.499101732673572,0.518702177574605,0.538302622475638),
 .UNSPECIFIED.);
#23728=B_SPLINE_CURVE_WITH_KNOTS('',3,(#144609,#144610,#144611,#144612),
 .UNSPECIFIED.,.F.,.F.,(4,4),(7.0054188597794,7.15111856184614),
 .UNSPECIFIED.);
#23729=B_SPLINE_CURVE_WITH_KNOTS('',3,(#144618,#144619,#144620,#144621,
#144622,#144623,#144624,#144625,#144626,#144627),.UNSPECIFIED.,.F.,.F.,
(4,2,2,2,4),(0.959941045056019,1.01793558590819,1.10632333107227,1.1957800913699,
1.2405102505028),.UNSPECIFIED.);
#23730=B_SPLINE_CURVE_WITH_KNOTS('',3,(#144650,#144651,#144652,#144653,
#144654,#144655,#144656,#144657,#144658,#144659,#144660,#144661,#144662),
 .UNSPECIFIED.,.F.,.F.,(4,1,1,1,1,1,1,1,1,1,4),(-0.194615646314672,-0.191966963306305,
-0.188476654882554,-0.181496038035052,-0.167534804340048,-0.13961233695004,
-0.125651103255036,-0.111689869560032,-0.0837674021700239,-0.0558449347800159,
0.),.UNSPECIFIED.);
#23731=B_SPLINE_CURVE_WITH_KNOTS('',3,(#144663,#144664,#144665,#144666,
#144667,#144668,#144669,#144670,#144671,#144672,#144673,#144674,#144675,
#144676,#144677,#144678,#144679,#144680,#144681,#144682,#144683),
 .UNSPECIFIED.,.F.,.F.,(4,2,2,2,2,3,2,2,2,4),(-0.184532964552272,-0.110069111897134,
-0.0293037936841922,-0.0146518968420961,-0.00732594842104806,0.,0.00444223893322424,
0.00888447786644848,0.017768955732897,0.0282169626580737),.UNSPECIFIED.);
#23732=B_SPLINE_CURVE_WITH_KNOTS('',3,(#144704,#144705,#144706,#144707,
#144708),.UNSPECIFIED.,.F.,.F.,(4,1,4),(-0.148760844879958,-0.0637546478056962,
0.),.UNSPECIFIED.);
#23733=B_SPLINE_CURVE_WITH_KNOTS('',3,(#144719,#144720,#144721,#144722,
#144723),.UNSPECIFIED.,.F.,.F.,(4,1,4),(0.,0.0637546478056962,0.148760844879958),
 .UNSPECIFIED.);
#23734=B_SPLINE_CURVE_WITH_KNOTS('',3,(#144725,#144726,#144727,#144728,
#144729,#144730,#144731,#144732,#144733,#144734,#144735,#144736),
 .UNSPECIFIED.,.F.,.F.,(4,2,2,2,2,4),(0.125732173566188,0.141264421553229,
0.170878065072357,0.200491708591485,0.260959450514356,0.268438600062818),
 .UNSPECIFIED.);
#23735=B_SPLINE_CURVE_WITH_KNOTS('',3,(#144782,#144783,#144784,#144785,
#144786,#144787,#144788,#144789,#144790,#144791,#144792,#144793),
 .UNSPECIFIED.,.F.,.F.,(4,2,2,2,2,4),(0.449858469158036,0.479607229821293,
0.553740396055668,0.642656295652044,0.695378146353882,0.704137329267106),
 .UNSPECIFIED.);
#23736=B_SPLINE_CURVE_WITH_KNOTS('',3,(#144796,#144797,#144798,#144799,
#144800,#144801,#144802,#144803,#144804,#144805,#144806,#144807,#144808),
 .UNSPECIFIED.,.F.,.F.,(4,3,2,2,2,4),(0.407700454474756,0.44038618270827,
0.469743957690921,0.499101732673573,0.518702177574606,0.538302622475639),
 .UNSPECIFIED.);
#23737=B_SPLINE_CURVE_WITH_KNOTS('',3,(#144814,#144815,#144816,#144817,
#144818,#144819,#144820),.UNSPECIFIED.,.F.,.F.,(4,3,4),(2.40353495487923,
2.40579815042619,2.52067239352636),.UNSPECIFIED.);
#23738=B_SPLINE_CURVE_WITH_KNOTS('',3,(#144823,#144824,#144825,#144826,
#144827,#144828,#144829,#144830,#144831,#144832,#144833,#144834,#144835),
 .UNSPECIFIED.,.F.,.F.,(4,2,2,2,3,4),(0.342469742940901,0.362070187841934,
0.381670632742967,0.411028407725619,0.44038618270827,0.473071910941784),
 .UNSPECIFIED.);
#23739=B_SPLINE_CURVE_WITH_KNOTS('',3,(#144903,#144904,#144905,#144906,
#144907,#144908,#144909),.UNSPECIFIED.,.F.,.F.,(4,3,4),(0.,0.00387940189952665,
0.00751236288843331),.UNSPECIFIED.);
#23740=B_SPLINE_CURVE_WITH_KNOTS('',3,(#144972,#144973,#144974,#144975,
#144976,#144977),.UNSPECIFIED.,.F.,.F.,(4,2,4),(1.82331017716016,1.90750204863416,
2.02800814763992),.UNSPECIFIED.);
#23741=B_SPLINE_CURVE_WITH_KNOTS('',3,(#145072,#145073,#145074,#145075,
#145076,#145077),.UNSPECIFIED.,.F.,.F.,(4,2,4),(2.32014740388574,2.402277537928,
2.48440767197027),.UNSPECIFIED.);
#23742=B_SPLINE_CURVE_WITH_KNOTS('',3,(#145178,#145179,#145180,#145181),
 .UNSPECIFIED.,.F.,.F.,(4,4),(0.,0.00120017992069814),.UNSPECIFIED.);
#23743=B_SPLINE_CURVE_WITH_KNOTS('',3,(#145202,#145203,#145204,#145205),
 .UNSPECIFIED.,.F.,.F.,(4,4),(0.,0.00271678269554457),.UNSPECIFIED.);
#23744=B_SPLINE_CURVE_WITH_KNOTS('',3,(#145267,#145268,#145269,#145270,
#145271,#145272),.UNSPECIFIED.,.F.,.F.,(4,1,1,4),(0.304018832611615,0.312633818864471,
0.321815335614959,0.346299380282928),.UNSPECIFIED.);
#27340=LINE('',#138721,#31142);
#27341=LINE('',#138724,#31143);
#27342=LINE('',#138821,#31144);
#27343=LINE('',#138822,#31145);
#27344=LINE('',#138836,#31146);
#27345=LINE('',#138840,#31147);
#27346=LINE('',#138844,#31148);
#27347=LINE('',#138854,#31149);
#27348=LINE('',#138857,#31150);
#27349=LINE('',#138860,#31151);
#27350=LINE('',#138864,#31152);
#27351=LINE('',#138865,#31153);
#27352=LINE('',#138868,#31154);
#27353=LINE('',#138872,#31155);
#27354=LINE('',#138873,#31156);
#27355=LINE('',#138880,#31157);
#27356=LINE('',#138883,#31158);
#27357=LINE('',#138928,#31159);
#27358=LINE('',#138929,#31160);
#27359=LINE('',#138948,#31161);
#27360=LINE('',#138949,#31162);
#27361=LINE('',#138960,#31163);
#27362=LINE('',#138961,#31164);
#27363=LINE('',#139023,#31165);
#27364=LINE('',#139025,#31166);
#27365=LINE('',#139026,#31167);
#27366=LINE('',#139029,#31168);
#27367=LINE('',#139033,#31169);
#27368=LINE('',#139037,#31170);
#27369=LINE('',#139042,#31171);
#27370=LINE('',#139044,#31172);
#27371=LINE('',#139048,#31173);
#27372=LINE('',#139052,#31174);
#27373=LINE('',#139056,#31175);
#27374=LINE('',#139060,#31176);
#27375=LINE('',#139064,#31177);
#27376=LINE('',#139068,#31178);
#27377=LINE('',#139069,#31179);
#27378=LINE('',#139098,#31180);
#27379=LINE('',#139099,#31181);
#27380=LINE('',#139124,#31182);
#27381=LINE('',#139125,#31183);
#27382=LINE('',#139170,#31184);
#27383=LINE('',#139171,#31185);
#27384=LINE('',#139202,#31186);
#27385=LINE('',#139206,#31187);
#27386=LINE('',#139209,#31188);
#27387=LINE('',#139212,#31189);
#27388=LINE('',#139213,#31190);
#27389=LINE('',#139218,#31191);
#27390=LINE('',#139222,#31192);
#27391=LINE('',#139230,#31193);
#27392=LINE('',#139233,#31194);
#27393=LINE('',#139284,#31195);
#27394=LINE('',#139285,#31196);
#27395=LINE('',#139316,#31197);
#27396=LINE('',#139317,#31198);
#27397=LINE('',#139331,#31199);
#27398=LINE('',#139333,#31200);
#27399=LINE('',#139335,#31201);
#27400=LINE('',#139337,#31202);
#27401=LINE('',#139338,#31203);
#27402=LINE('',#139341,#31204);
#27403=LINE('',#139345,#31205);
#27404=LINE('',#139349,#31206);
#27405=LINE('',#139350,#31207);
#27406=LINE('',#139353,#31208);
#27407=LINE('',#139357,#31209);
#27408=LINE('',#139359,#31210);
#27409=LINE('',#139361,#31211);
#27410=LINE('',#139362,#31212);
#27411=LINE('',#139429,#31213);
#27412=LINE('',#139430,#31214);
#27413=LINE('',#139441,#31215);
#27414=LINE('',#139442,#31216);
#27415=LINE('',#139461,#31217);
#27416=LINE('',#139462,#31218);
#27417=LINE('',#139510,#31219);
#27418=LINE('',#139511,#31220);
#27419=LINE('',#139514,#31221);
#27420=LINE('',#139517,#31222);
#27421=LINE('',#139520,#31223);
#27422=LINE('',#139521,#31224);
#27423=LINE('',#139524,#31225);
#27424=LINE('',#139528,#31226);
#27425=LINE('',#139532,#31227);
#27426=LINE('',#139536,#31228);
#27427=LINE('',#139537,#31229);
#27428=LINE('',#139540,#31230);
#27429=LINE('',#139628,#31231);
#27430=LINE('',#139629,#31232);
#27431=LINE('',#139643,#31233);
#27432=LINE('',#139646,#31234);
#27433=LINE('',#139649,#31235);
#27434=LINE('',#139653,#31236);
#27435=LINE('',#139654,#31237);
#27436=LINE('',#139657,#31238);
#27437=LINE('',#139661,#31239);
#27438=LINE('',#139723,#31240);
#27439=LINE('',#139724,#31241);
#27440=LINE('',#139749,#31242);
#27441=LINE('',#139750,#31243);
#27442=LINE('',#139769,#31244);
#27443=LINE('',#139770,#31245);
#27444=LINE('',#139830,#31246);
#27445=LINE('',#139833,#31247);
#27446=LINE('',#139836,#31248);
#27447=LINE('',#139837,#31249);
#27448=LINE('',#139840,#31250);
#27449=LINE('',#139844,#31251);
#27450=LINE('',#139848,#31252);
#27451=LINE('',#139852,#31253);
#27452=LINE('',#139856,#31254);
#27453=LINE('',#139860,#31255);
#27454=LINE('',#139864,#31256);
#27455=LINE('',#139906,#31257);
#27456=LINE('',#139907,#31258);
#27457=LINE('',#139973,#31259);
#27458=LINE('',#139977,#31260);
#27459=LINE('',#139981,#31261);
#27460=LINE('',#139984,#31262);
#27461=LINE('',#139987,#31263);
#27462=LINE('',#139991,#31264);
#27463=LINE('',#139995,#31265);
#27464=LINE('',#139999,#31266);
#27465=LINE('',#140007,#31267);
#27466=LINE('',#140010,#31268);
#27467=LINE('',#140029,#31269);
#27468=LINE('',#140030,#31270);
#27469=LINE('',#140102,#31271);
#27470=LINE('',#140105,#31272);
#27471=LINE('',#140108,#31273);
#27472=LINE('',#140112,#31274);
#27473=LINE('',#140116,#31275);
#27474=LINE('',#140117,#31276);
#27475=LINE('',#140329,#31277);
#27476=LINE('',#140333,#31278);
#27477=LINE('',#140337,#31279);
#27478=LINE('',#140360,#31280);
#27479=LINE('',#140364,#31281);
#27480=LINE('',#140368,#31282);
#27481=LINE('',#140389,#31283);
#27482=LINE('',#140392,#31284);
#27483=LINE('',#140396,#31285);
#27484=LINE('',#140398,#31286);
#27485=LINE('',#140400,#31287);
#27486=LINE('',#140405,#31288);
#27487=LINE('',#140407,#31289);
#27488=LINE('',#140409,#31290);
#27489=LINE('',#140410,#31291);
#27490=LINE('',#140416,#31292);
#27491=LINE('',#140419,#31293);
#27492=LINE('',#140424,#31294);
#27493=LINE('',#140427,#31295);
#27494=LINE('',#140431,#31296);
#27495=LINE('',#140435,#31297);
#27496=LINE('',#140450,#31298);
#27497=LINE('',#140454,#31299);
#27498=LINE('',#140456,#31300);
#27499=LINE('',#140458,#31301);
#27500=LINE('',#140462,#31302);
#27501=LINE('',#140465,#31303);
#27502=LINE('',#140471,#31304);
#27503=LINE('',#140474,#31305);
#27504=LINE('',#140478,#31306);
#27505=LINE('',#140482,#31307);
#27506=LINE('',#140486,#31308);
#27507=LINE('',#140501,#31309);
#27508=LINE('',#140504,#31310);
#27509=LINE('',#140508,#31311);
#27510=LINE('',#140517,#31312);
#27511=LINE('',#140522,#31313);
#27512=LINE('',#140524,#31314);
#27513=LINE('',#140525,#31315);
#27514=LINE('',#140528,#31316);
#27515=LINE('',#140531,#31317);
#27516=LINE('',#140534,#31318);
#27517=LINE('',#140535,#31319);
#27518=LINE('',#140538,#31320);
#27519=LINE('',#140543,#31321);
#27520=LINE('',#140547,#31322);
#27521=LINE('',#140552,#31323);
#27522=LINE('',#140556,#31324);
#27523=LINE('',#140562,#31325);
#27524=LINE('',#140568,#31326);
#27525=LINE('',#140572,#31327);
#27526=LINE('',#140576,#31328);
#27527=LINE('',#140580,#31329);
#27528=LINE('',#140584,#31330);
#27529=LINE('',#140593,#31331);
#27530=LINE('',#140596,#31332);
#27531=LINE('',#140598,#31333);
#27532=LINE('',#140605,#31334);
#27533=LINE('',#140608,#31335);
#27534=LINE('',#140611,#31336);
#27535=LINE('',#140614,#31337);
#27536=LINE('',#140619,#31338);
#27537=LINE('',#140622,#31339);
#27538=LINE('',#140626,#31340);
#27539=LINE('',#140630,#31341);
#27540=LINE('',#140632,#31342);
#27541=LINE('',#140638,#31343);
#27542=LINE('',#140641,#31344);
#27543=LINE('',#140648,#31345);
#27544=LINE('',#140651,#31346);
#27545=LINE('',#140654,#31347);
#27546=LINE('',#140655,#31348);
#27547=LINE('',#140674,#31349);
#27548=LINE('',#140678,#31350);
#27549=LINE('',#140682,#31351);
#27550=LINE('',#140684,#31352);
#27551=LINE('',#140685,#31353);
#27552=LINE('',#140687,#31354);
#27553=LINE('',#140689,#31355);
#27554=LINE('',#140691,#31356);
#27555=LINE('',#140692,#31357);
#27556=LINE('',#140694,#31358);
#27557=LINE('',#140696,#31359);
#27558=LINE('',#140698,#31360);
#27559=LINE('',#140700,#31361);
#27560=LINE('',#140704,#31362);
#27561=LINE('',#140707,#31363);
#27562=LINE('',#140710,#31364);
#27563=LINE('',#140716,#31365);
#27564=LINE('',#140719,#31366);
#27565=LINE('',#140722,#31367);
#27566=LINE('',#140725,#31368);
#27567=LINE('',#140727,#31369);
#27568=LINE('',#140730,#31370);
#27569=LINE('',#140732,#31371);
#27570=LINE('',#140734,#31372);
#27571=LINE('',#140740,#31373);
#27572=LINE('',#140741,#31374);
#27573=LINE('',#140743,#31375);
#27574=LINE('',#140745,#31376);
#27575=LINE('',#140747,#31377);
#27576=LINE('',#140749,#31378);
#27577=LINE('',#140752,#31379);
#27578=LINE('',#140753,#31380);
#27579=LINE('',#140755,#31381);
#27580=LINE('',#140758,#31382);
#27581=LINE('',#140761,#31383);
#27582=LINE('',#140765,#31384);
#27583=LINE('',#140768,#31385);
#27584=LINE('',#140770,#31386);
#27585=LINE('',#140771,#31387);
#27586=LINE('',#140779,#31388);
#27587=LINE('',#140781,#31389);
#27588=LINE('',#140789,#31390);
#27589=LINE('',#140792,#31391);
#27590=LINE('',#140801,#31392);
#27591=LINE('',#140806,#31393);
#27592=LINE('',#140808,#31394);
#27593=LINE('',#140809,#31395);
#27594=LINE('',#140812,#31396);
#27595=LINE('',#140817,#31397);
#27596=LINE('',#140818,#31398);
#27597=LINE('',#140820,#31399);
#27598=LINE('',#140823,#31400);
#27599=LINE('',#140824,#31401);
#27600=LINE('',#140826,#31402);
#27601=LINE('',#140828,#31403);
#27602=LINE('',#140830,#31404);
#27603=LINE('',#140833,#31405);
#27604=LINE('',#140835,#31406);
#27605=LINE('',#140837,#31407);
#27606=LINE('',#140843,#31408);
#27607=LINE('',#140849,#31409);
#27608=LINE('',#140851,#31410);
#27609=LINE('',#140855,#31411);
#27610=LINE('',#140859,#31412);
#27611=LINE('',#140867,#31413);
#27612=LINE('',#140871,#31414);
#27613=LINE('',#140873,#31415);
#27614=LINE('',#140883,#31416);
#27615=LINE('',#140888,#31417);
#27616=LINE('',#140891,#31418);
#27617=LINE('',#140894,#31419);
#27618=LINE('',#140897,#31420);
#27619=LINE('',#140898,#31421);
#27620=LINE('',#140901,#31422);
#27621=LINE('',#140907,#31423);
#27622=LINE('',#140908,#31424);
#27623=LINE('',#140911,#31425);
#27624=LINE('',#140912,#31426);
#27625=LINE('',#140916,#31427);
#27626=LINE('',#140918,#31428);
#27627=LINE('',#140923,#31429);
#27628=LINE('',#140927,#31430);
#27629=LINE('',#140931,#31431);
#27630=LINE('',#140936,#31432);
#27631=LINE('',#140937,#31433);
#27632=LINE('',#140940,#31434);
#27633=LINE('',#140941,#31435);
#27634=LINE('',#140951,#31436);
#27635=LINE('',#140953,#31437);
#27636=LINE('',#140956,#31438);
#27637=LINE('',#140959,#31439);
#27638=LINE('',#140961,#31440);
#27639=LINE('',#140963,#31441);
#27640=LINE('',#140965,#31442);
#27641=LINE('',#140967,#31443);
#27642=LINE('',#140969,#31444);
#27643=LINE('',#140971,#31445);
#27644=LINE('',#140973,#31446);
#27645=LINE('',#140975,#31447);
#27646=LINE('',#140999,#31448);
#27647=LINE('',#141002,#31449);
#27648=LINE('',#141004,#31450);
#27649=LINE('',#141005,#31451);
#27650=LINE('',#141011,#31452);
#27651=LINE('',#141018,#31453);
#27652=LINE('',#141021,#31454);
#27653=LINE('',#141028,#31455);
#27654=LINE('',#141032,#31456);
#27655=LINE('',#141040,#31457);
#27656=LINE('',#141044,#31458);
#27657=LINE('',#141048,#31459);
#27658=LINE('',#141052,#31460);
#27659=LINE('',#141056,#31461);
#27660=LINE('',#141059,#31462);
#27661=LINE('',#141063,#31463);
#27662=LINE('',#141067,#31464);
#27663=LINE('',#141070,#31465);
#27664=LINE('',#141072,#31466);
#27665=LINE('',#141074,#31467);
#27666=LINE('',#141075,#31468);
#27667=LINE('',#141107,#31469);
#27668=LINE('',#141126,#31470);
#27669=LINE('',#141127,#31471);
#27670=LINE('',#141173,#31472);
#27671=LINE('',#141176,#31473);
#27672=LINE('',#141179,#31474);
#27673=LINE('',#141183,#31475);
#27674=LINE('',#141187,#31476);
#27675=LINE('',#141191,#31477);
#27676=LINE('',#141242,#31478);
#27677=LINE('',#141243,#31479);
#27678=LINE('',#141294,#31480);
#27679=LINE('',#141295,#31481);
#27680=LINE('',#141298,#31482);
#27681=LINE('',#141301,#31483);
#27682=LINE('',#141304,#31484);
#27683=LINE('',#141308,#31485);
#27684=LINE('',#141309,#31486);
#27685=LINE('',#141312,#31487);
#27686=LINE('',#141401,#31488);
#27687=LINE('',#141408,#31489);
#27688=LINE('',#141415,#31490);
#27689=LINE('',#141419,#31491);
#27690=LINE('',#141454,#31492);
#27691=LINE('',#141457,#31493);
#27692=LINE('',#141472,#31494);
#27693=LINE('',#141510,#31495);
#27694=LINE('',#141513,#31496);
#27695=LINE('',#141516,#31497);
#27696=LINE('',#141518,#31498);
#27697=LINE('',#141524,#31499);
#27698=LINE('',#141530,#31500);
#27699=LINE('',#141545,#31501);
#27700=LINE('',#141560,#31502);
#27701=LINE('',#141563,#31503);
#27702=LINE('',#141569,#31504);
#27703=LINE('',#141577,#31505);
#27704=LINE('',#141596,#31506);
#27705=LINE('',#141598,#31507);
#27706=LINE('',#141600,#31508);
#27707=LINE('',#141602,#31509);
#27708=LINE('',#141603,#31510);
#27709=LINE('',#141605,#31511);
#27710=LINE('',#141607,#31512);
#27711=LINE('',#141609,#31513);
#27712=LINE('',#141611,#31514);
#27713=LINE('',#141616,#31515);
#27714=LINE('',#141619,#31516);
#27715=LINE('',#141622,#31517);
#27716=LINE('',#141626,#31518);
#27717=LINE('',#141627,#31519);
#27718=LINE('',#141630,#31520);
#27719=LINE('',#141636,#31521);
#27720=LINE('',#141637,#31522);
#27721=LINE('',#141704,#31523);
#27722=LINE('',#141706,#31524);
#27723=LINE('',#141709,#31525);
#27724=LINE('',#141710,#31526);
#27725=LINE('',#141713,#31527);
#27726=LINE('',#141717,#31528);
#27727=LINE('',#141719,#31529);
#27728=LINE('',#141720,#31530);
#27729=LINE('',#141723,#31531);
#27730=LINE('',#141730,#31532);
#27731=LINE('',#141732,#31533);
#27732=LINE('',#141745,#31534);
#27733=LINE('',#141839,#31535);
#27734=LINE('',#141843,#31536);
#27735=LINE('',#141846,#31537);
#27736=LINE('',#141850,#31538);
#27737=LINE('',#141866,#31539);
#27738=LINE('',#141882,#31540);
#27739=LINE('',#141899,#31541);
#27740=LINE('',#141903,#31542);
#27741=LINE('',#141915,#31543);
#27742=LINE('',#141919,#31544);
#27743=LINE('',#141923,#31545);
#27744=LINE('',#141924,#31546);
#27745=LINE('',#141927,#31547);
#27746=LINE('',#141931,#31548);
#27747=LINE('',#141932,#31549);
#27748=LINE('',#141935,#31550);
#27749=LINE('',#141939,#31551);
#27750=LINE('',#141940,#31552);
#27751=LINE('',#141943,#31553);
#27752=LINE('',#141974,#31554);
#27753=LINE('',#141978,#31555);
#27754=LINE('',#142028,#31556);
#27755=LINE('',#142064,#31557);
#27756=LINE('',#142065,#31558);
#27757=LINE('',#142076,#31559);
#27758=LINE('',#142077,#31560);
#27759=LINE('',#142136,#31561);
#27760=LINE('',#142137,#31562);
#27761=LINE('',#142145,#31563);
#27762=LINE('',#142147,#31564);
#27763=LINE('',#142148,#31565);
#27764=LINE('',#142151,#31566);
#27765=LINE('',#142155,#31567);
#27766=LINE('',#142156,#31568);
#27767=LINE('',#142159,#31569);
#27768=LINE('',#142163,#31570);
#27769=LINE('',#142167,#31571);
#27770=LINE('',#142175,#31572);
#27771=LINE('',#142178,#31573);
#27772=LINE('',#142197,#31574);
#27773=LINE('',#142198,#31575);
#27774=LINE('',#142229,#31576);
#27775=LINE('',#142230,#31577);
#27776=LINE('',#142281,#31578);
#27777=LINE('',#142282,#31579);
#27778=LINE('',#142296,#31580);
#27779=LINE('',#142299,#31581);
#27780=LINE('',#142302,#31582);
#27781=LINE('',#142306,#31583);
#27782=LINE('',#142310,#31584);
#27783=LINE('',#142311,#31585);
#27784=LINE('',#142314,#31586);
#27785=LINE('',#142318,#31587);
#27786=LINE('',#142319,#31588);
#27787=LINE('',#142326,#31589);
#27788=LINE('',#142329,#31590);
#27789=LINE('',#142348,#31591);
#27790=LINE('',#142349,#31592);
#27791=LINE('',#142368,#31593);
#27792=LINE('',#142369,#31594);
#27793=LINE('',#142427,#31595);
#27794=LINE('',#142430,#31596);
#27795=LINE('',#142433,#31597);
#27796=LINE('',#142437,#31598);
#27797=LINE('',#142441,#31599);
#27798=LINE('',#142445,#31600);
#27799=LINE('',#142449,#31601);
#27800=LINE('',#142522,#31602);
#27801=LINE('',#142526,#31603);
#27802=LINE('',#142530,#31604);
#27803=LINE('',#142531,#31605);
#27804=LINE('',#142603,#31606);
#27805=LINE('',#142605,#31607);
#27806=LINE('',#142608,#31608);
#27807=LINE('',#142615,#31609);
#27808=LINE('',#142619,#31610);
#27809=LINE('',#142622,#31611);
#27810=LINE('',#142627,#31612);
#27811=LINE('',#142631,#31613);
#27812=LINE('',#142633,#31614);
#27813=LINE('',#142636,#31615);
#27814=LINE('',#142656,#31616);
#27815=LINE('',#142660,#31617);
#27816=LINE('',#142675,#31618);
#27817=LINE('',#142696,#31619);
#27818=LINE('',#142711,#31620);
#27819=LINE('',#142725,#31621);
#27820=LINE('',#142731,#31622);
#27821=LINE('',#142734,#31623);
#27822=LINE('',#142745,#31624);
#27823=LINE('',#142746,#31625);
#27824=LINE('',#142797,#31626);
#27825=LINE('',#142798,#31627);
#27826=LINE('',#142839,#31628);
#27827=LINE('',#142840,#31629);
#27828=LINE('',#142860,#31630);
#27829=LINE('',#142863,#31631);
#27830=LINE('',#142867,#31632);
#27831=LINE('',#142869,#31633);
#27832=LINE('',#142873,#31634);
#27833=LINE('',#142877,#31635);
#27834=LINE('',#142881,#31636);
#27835=LINE('',#142885,#31637);
#27836=LINE('',#142889,#31638);
#27837=LINE('',#142893,#31639);
#27838=LINE('',#142894,#31640);
#27839=LINE('',#142897,#31641);
#27840=LINE('',#142901,#31642);
#27841=LINE('',#142902,#31643);
#27842=LINE('',#142944,#31644);
#27843=LINE('',#142945,#31645);
#27844=LINE('',#142964,#31646);
#27845=LINE('',#142965,#31647);
#27846=LINE('',#143001,#31648);
#27847=LINE('',#143002,#31649);
#27848=LINE('',#143059,#31650);
#27849=LINE('',#143061,#31651);
#27850=LINE('',#143062,#31652);
#27851=LINE('',#143065,#31653);
#27852=LINE('',#143098,#31654);
#27853=LINE('',#143101,#31655);
#27854=LINE('',#143105,#31656);
#27855=LINE('',#143169,#31657);
#27856=LINE('',#143173,#31658);
#27857=LINE('',#143176,#31659);
#27858=LINE('',#143211,#31660);
#27859=LINE('',#143212,#31661);
#27860=LINE('',#143248,#31662);
#27861=LINE('',#143249,#31663);
#27862=LINE('',#143268,#31664);
#27863=LINE('',#143269,#31665);
#27864=LINE('',#143283,#31666);
#27865=LINE('',#143285,#31667);
#27866=LINE('',#143286,#31668);
#27867=LINE('',#143289,#31669);
#27868=LINE('',#143293,#31670);
#27869=LINE('',#143294,#31671);
#27870=LINE('',#143297,#31672);
#27871=LINE('',#143301,#31673);
#27872=LINE('',#143305,#31674);
#27873=LINE('',#143309,#31675);
#27874=LINE('',#143357,#31676);
#27875=LINE('',#143362,#31677);
#27876=LINE('',#143366,#31678);
#27877=LINE('',#143367,#31679);
#27878=LINE('',#143372,#31680);
#27879=LINE('',#143381,#31681);
#27880=LINE('',#143384,#31682);
#27881=LINE('',#143387,#31683);
#27882=LINE('',#143389,#31684);
#27883=LINE('',#143391,#31685);
#27884=LINE('',#143393,#31686);
#27885=LINE('',#143395,#31687);
#27886=LINE('',#143397,#31688);
#27887=LINE('',#143398,#31689);
#27888=LINE('',#143401,#31690);
#27889=LINE('',#143403,#31691);
#27890=LINE('',#143404,#31692);
#27891=LINE('',#143410,#31693);
#27892=LINE('',#143416,#31694);
#27893=LINE('',#143422,#31695);
#27894=LINE('',#143428,#31696);
#27895=LINE('',#143432,#31697);
#27896=LINE('',#143434,#31698);
#27897=LINE('',#143435,#31699);
#27898=LINE('',#143441,#31700);
#27899=LINE('',#143450,#31701);
#27900=LINE('',#143454,#31702);
#27901=LINE('',#143457,#31703);
#27902=LINE('',#143459,#31704);
#27903=LINE('',#143461,#31705);
#27904=LINE('',#143463,#31706);
#27905=LINE('',#143465,#31707);
#27906=LINE('',#143467,#31708);
#27907=LINE('',#143469,#31709);
#27908=LINE('',#143471,#31710);
#27909=LINE('',#143472,#31711);
#27910=LINE('',#143475,#31712);
#27911=LINE('',#143479,#31713);
#27912=LINE('',#143487,#31714);
#27913=LINE('',#143494,#31715);
#27914=LINE('',#143497,#31716);
#27915=LINE('',#143500,#31717);
#27916=LINE('',#143502,#31718);
#27917=LINE('',#143503,#31719);
#27918=LINE('',#143506,#31720);
#27919=LINE('',#143510,#31721);
#27920=LINE('',#143512,#31722);
#27921=LINE('',#143513,#31723);
#27922=LINE('',#143518,#31724);
#27923=LINE('',#143525,#31725);
#27924=LINE('',#143528,#31726);
#27925=LINE('',#143536,#31727);
#27926=LINE('',#143542,#31728);
#27927=LINE('',#143547,#31729);
#27928=LINE('',#143551,#31730);
#27929=LINE('',#143575,#31731);
#27930=LINE('',#143595,#31732);
#27931=LINE('',#143598,#31733);
#27932=LINE('',#143618,#31734);
#27933=LINE('',#143623,#31735);
#27934=LINE('',#143628,#31736);
#27935=LINE('',#143633,#31737);
#27936=LINE('',#143638,#31738);
#27937=LINE('',#143643,#31739);
#27938=LINE('',#143648,#31740);
#27939=LINE('',#143661,#31741);
#27940=LINE('',#143663,#31742);
#27941=LINE('',#143667,#31743);
#27942=LINE('',#143668,#31744);
#27943=LINE('',#143674,#31745);
#27944=LINE('',#143676,#31746);
#27945=LINE('',#143680,#31747);
#27946=LINE('',#143681,#31748);
#27947=LINE('',#143684,#31749);
#27948=LINE('',#143686,#31750);
#27949=LINE('',#143687,#31751);
#27950=LINE('',#143693,#31752);
#27951=LINE('',#143696,#31753);
#27952=LINE('',#143697,#31754);
#27953=LINE('',#143700,#31755);
#27954=LINE('',#143702,#31756);
#27955=LINE('',#143703,#31757);
#27956=LINE('',#143709,#31758);
#27957=LINE('',#143712,#31759);
#27958=LINE('',#143713,#31760);
#27959=LINE('',#143733,#31761);
#27960=LINE('',#143735,#31762);
#27961=LINE('',#143736,#31763);
#27962=LINE('',#143742,#31764);
#27963=LINE('',#143749,#31765);
#27964=LINE('',#143750,#31766);
#27965=LINE('',#143765,#31767);
#27966=LINE('',#143767,#31768);
#27967=LINE('',#143768,#31769);
#27968=LINE('',#143774,#31770);
#27969=LINE('',#143781,#31771);
#27970=LINE('',#143782,#31772);
#27971=LINE('',#143792,#31773);
#27972=LINE('',#143794,#31774);
#27973=LINE('',#143795,#31775);
#27974=LINE('',#143797,#31776);
#27975=LINE('',#143798,#31777);
#27976=LINE('',#143811,#31778);
#27977=LINE('',#143827,#31779);
#27978=LINE('',#143831,#31780);
#27979=LINE('',#143833,#31781);
#27980=LINE('',#143834,#31782);
#27981=LINE('',#143840,#31783);
#27982=LINE('',#143856,#31784);
#27983=LINE('',#143860,#31785);
#27984=LINE('',#143862,#31786);
#27985=LINE('',#143865,#31787);
#27986=LINE('',#143868,#31788);
#27987=LINE('',#143870,#31789);
#27988=LINE('',#143871,#31790);
#27989=LINE('',#143885,#31791);
#27990=LINE('',#143905,#31792);
#27991=LINE('',#143936,#31793);
#27992=LINE('',#143937,#31794);
#27993=LINE('',#143940,#31795);
#27994=LINE('',#143944,#31796);
#27995=LINE('',#143945,#31797);
#27996=LINE('',#143950,#31798);
#27997=LINE('',#143980,#31799);
#27998=LINE('',#143991,#31800);
#27999=LINE('',#144004,#31801);
#28000=LINE('',#144008,#31802);
#28001=LINE('',#144009,#31803);
#28002=LINE('',#144010,#31804);
#28003=LINE('',#144023,#31805);
#28004=LINE('',#144035,#31806);
#28005=LINE('',#144036,#31807);
#28006=LINE('',#144037,#31808);
#28007=LINE('',#144055,#31809);
#28008=LINE('',#144056,#31810);
#28009=LINE('',#144072,#31811);
#28010=LINE('',#144086,#31812);
#28011=LINE('',#144103,#31813);
#28012=LINE('',#144105,#31814);
#28013=LINE('',#144107,#31815);
#28014=LINE('',#144109,#31816);
#28015=LINE('',#144111,#31817);
#28016=LINE('',#144112,#31818);
#28017=LINE('',#144113,#31819);
#28018=LINE('',#144114,#31820);
#28019=LINE('',#144132,#31821);
#28020=LINE('',#144135,#31822);
#28021=LINE('',#144151,#31823);
#28022=LINE('',#144204,#31824);
#28023=LINE('',#144228,#31825);
#28024=LINE('',#144232,#31826);
#28025=LINE('',#144266,#31827);
#28026=LINE('',#144269,#31828);
#28027=LINE('',#144274,#31829);
#28028=LINE('',#144324,#31830);
#28029=LINE('',#144349,#31831);
#28030=LINE('',#144356,#31832);
#28031=LINE('',#144360,#31833);
#28032=LINE('',#144366,#31834);
#28033=LINE('',#144383,#31835);
#28034=LINE('',#144387,#31836);
#28035=LINE('',#144405,#31837);
#28036=LINE('',#144409,#31838);
#28037=LINE('',#144416,#31839);
#28038=LINE('',#144419,#31840);
#28039=LINE('',#144423,#31841);
#28040=LINE('',#144427,#31842);
#28041=LINE('',#144432,#31843);
#28042=LINE('',#144437,#31844);
#28043=LINE('',#144441,#31845);
#28044=LINE('',#144442,#31846);
#28045=LINE('',#144446,#31847);
#28046=LINE('',#144449,#31848);
#28047=LINE('',#144453,#31849);
#28048=LINE('',#144470,#31850);
#28049=LINE('',#144475,#31851);
#28050=LINE('',#144479,#31852);
#28051=LINE('',#144480,#31853);
#28052=LINE('',#144495,#31854);
#28053=LINE('',#144500,#31855);
#28054=LINE('',#144502,#31856);
#28055=LINE('',#144506,#31857);
#28056=LINE('',#144525,#31858);
#28057=LINE('',#144529,#31859);
#28058=LINE('',#144547,#31860);
#28059=LINE('',#144550,#31861);
#28060=LINE('',#144560,#31862);
#28061=LINE('',#144615,#31863);
#28062=LINE('',#144645,#31864);
#28063=LINE('',#144647,#31865);
#28064=LINE('',#144688,#31866);
#28065=LINE('',#144690,#31867);
#28066=LINE('',#144692,#31868);
#28067=LINE('',#144693,#31869);
#28068=LINE('',#144697,#31870);
#28069=LINE('',#144699,#31871);
#28070=LINE('',#144701,#31872);
#28071=LINE('',#144724,#31873);
#28072=LINE('',#144737,#31874);
#28073=LINE('',#144781,#31875);
#28074=LINE('',#144811,#31876);
#28075=LINE('',#144821,#31877);
#28076=LINE('',#144917,#31878);
#28077=LINE('',#144919,#31879);
#28078=LINE('',#144920,#31880);
#28079=LINE('',#144925,#31881);
#28080=LINE('',#144931,#31882);
#28081=LINE('',#144933,#31883);
#28082=LINE('',#144935,#31884);
#28083=LINE('',#144936,#31885);
#28084=LINE('',#144941,#31886);
#28085=LINE('',#144948,#31887);
#28086=LINE('',#144951,#31888);
#28087=LINE('',#144954,#31889);
#28088=LINE('',#144956,#31890);
#28089=LINE('',#144957,#31891);
#28090=LINE('',#144962,#31892);
#28091=LINE('',#144982,#31893);
#28092=LINE('',#144986,#31894);
#28093=LINE('',#144992,#31895);
#28094=LINE('',#144993,#31896);
#28095=LINE('',#144999,#31897);
#28096=LINE('',#145001,#31898);
#28097=LINE('',#145003,#31899);
#28098=LINE('',#145004,#31900);
#28099=LINE('',#145011,#31901);
#28100=LINE('',#145013,#31902);
#28101=LINE('',#145015,#31903);
#28102=LINE('',#145016,#31904);
#28103=LINE('',#145018,#31905);
#28104=LINE('',#145020,#31906);
#28105=LINE('',#145021,#31907);
#28106=LINE('',#145025,#31908);
#28107=LINE('',#145028,#31909);
#28108=LINE('',#145029,#31910);
#28109=LINE('',#145036,#31911);
#28110=LINE('',#145038,#31912);
#28111=LINE('',#145039,#31913);
#28112=LINE('',#145042,#31914);
#28113=LINE('',#145043,#31915);
#28114=LINE('',#145047,#31916);
#28115=LINE('',#145050,#31917);
#28116=LINE('',#145055,#31918);
#28117=LINE('',#145062,#31919);
#28118=LINE('',#145067,#31920);
#28119=LINE('',#145082,#31921);
#28120=LINE('',#145092,#31922);
#28121=LINE('',#145098,#31923);
#28122=LINE('',#145101,#31924);
#28123=LINE('',#145103,#31925);
#28124=LINE('',#145104,#31926);
#28125=LINE('',#145109,#31927);
#28126=LINE('',#145114,#31928);
#28127=LINE('',#145117,#31929);
#28128=LINE('',#145122,#31930);
#28129=LINE('',#145127,#31931);
#28130=LINE('',#145131,#31932);
#28131=LINE('',#145142,#31933);
#28132=LINE('',#145149,#31934);
#28133=LINE('',#145154,#31935);
#28134=LINE('',#145156,#31936);
#28135=LINE('',#145158,#31937);
#28136=LINE('',#145159,#31938);
#28137=LINE('',#145163,#31939);
#28138=LINE('',#145165,#31940);
#28139=LINE('',#145167,#31941);
#28140=LINE('',#145168,#31942);
#28141=LINE('',#145174,#31943);
#28142=LINE('',#145175,#31944);
#28143=LINE('',#145194,#31945);
#28144=LINE('',#145196,#31946);
#28145=LINE('',#145197,#31947);
#28146=LINE('',#145320,#31948);
#28147=LINE('',#145322,#31949);
#28148=LINE('',#145324,#31950);
#28149=LINE('',#145325,#31951);
#28150=LINE('',#145331,#31952);
#28151=LINE('',#145334,#31953);
#28152=LINE('',#145337,#31954);
#28153=LINE('',#145343,#31955);
#28154=LINE('',#145349,#31956);
#28155=LINE('',#145351,#31957);
#28156=LINE('',#145353,#31958);
#28157=LINE('',#145357,#31959);
#28158=LINE('',#145360,#31960);
#28159=LINE('',#145362,#31961);
#28160=LINE('',#145364,#31962);
#28161=LINE('',#145372,#31963);
#28162=LINE('',#145374,#31964);
#28163=LINE('',#145375,#31965);
#28164=LINE('',#145380,#31966);
#28165=LINE('',#145383,#31967);
#28166=LINE('',#145384,#31968);
#28167=LINE('',#145388,#31969);
#28168=LINE('',#145395,#31970);
#31142=VECTOR('',#106748,10.);
#31143=VECTOR('',#106751,10.);
#31144=VECTOR('',#106804,10.);
#31145=VECTOR('',#106805,10.);
#31146=VECTOR('',#106812,10.);
#31147=VECTOR('',#106815,10.);
#31148=VECTOR('',#106818,10.);
#31149=VECTOR('',#106819,12.);
#31150=VECTOR('',#106822,10.);
#31151=VECTOR('',#106825,10.);
#31152=VECTOR('',#106830,10.);
#31153=VECTOR('',#106831,10.);
#31154=VECTOR('',#106834,10.);
#31155=VECTOR('',#106839,10.);
#31156=VECTOR('',#106840,10.);
#31157=VECTOR('',#106847,10.);
#31158=VECTOR('',#106850,10.);
#31159=VECTOR('',#106875,10.);
#31160=VECTOR('',#106876,10.);
#31161=VECTOR('',#106887,10.);
#31162=VECTOR('',#106888,10.);
#31163=VECTOR('',#106901,10.);
#31164=VECTOR('',#106902,10.);
#31165=VECTOR('',#106939,10.);
#31166=VECTOR('',#106940,10.);
#31167=VECTOR('',#106941,10.);
#31168=VECTOR('',#106944,10.);
#31169=VECTOR('',#106949,10.);
#31170=VECTOR('',#106954,10.);
#31171=VECTOR('',#106961,3.15);
#31172=VECTOR('',#106962,10.);
#31173=VECTOR('',#106965,10.);
#31174=VECTOR('',#106968,10.);
#31175=VECTOR('',#106971,10.);
#31176=VECTOR('',#106974,10.);
#31177=VECTOR('',#106979,10.);
#31178=VECTOR('',#106984,10.);
#31179=VECTOR('',#106985,10.);
#31180=VECTOR('',#107008,10.);
#31181=VECTOR('',#107009,10.);
#31182=VECTOR('',#107020,10.);
#31183=VECTOR('',#107021,10.);
#31184=VECTOR('',#107046,10.);
#31185=VECTOR('',#107047,10.);
#31186=VECTOR('',#107066,10.);
#31187=VECTOR('',#107069,10.);
#31188=VECTOR('',#107072,3.2);
#31189=VECTOR('',#107075,10.);
#31190=VECTOR('',#107076,10.);
#31191=VECTOR('',#107083,10.);
#31192=VECTOR('',#107088,10.);
#31193=VECTOR('',#107097,10.);
#31194=VECTOR('',#107100,10.);
#31195=VECTOR('',#107141,10.);
#31196=VECTOR('',#107142,10.);
#31197=VECTOR('',#107161,10.);
#31198=VECTOR('',#107162,10.);
#31199=VECTOR('',#107169,5.80000000000001);
#31200=VECTOR('',#107170,10.);
#31201=VECTOR('',#107171,10.);
#31202=VECTOR('',#107172,10.);
#31203=VECTOR('',#107173,3.2);
#31204=VECTOR('',#107176,5.80000000000001);
#31205=VECTOR('',#107181,10.);
#31206=VECTOR('',#107186,10.);
#31207=VECTOR('',#107187,10.);
#31208=VECTOR('',#107190,10.);
#31209=VECTOR('',#107195,10.);
#31210=VECTOR('',#107196,10.);
#31211=VECTOR('',#107197,10.);
#31212=VECTOR('',#107198,10.);
#31213=VECTOR('',#107243,10.);
#31214=VECTOR('',#107244,10.);
#31215=VECTOR('',#107257,10.);
#31216=VECTOR('',#107258,10.);
#31217=VECTOR('',#107269,10.);
#31218=VECTOR('',#107270,10.);
#31219=VECTOR('',#107293,10.);
#31220=VECTOR('',#107294,10.);
#31221=VECTOR('',#107297,10.);
#31222=VECTOR('',#107300,10.);
#31223=VECTOR('',#107303,10.);
#31224=VECTOR('',#107304,10.);
#31225=VECTOR('',#107307,10.);
#31226=VECTOR('',#107312,0.800000000000001);
#31227=VECTOR('',#107317,0.800000000000001);
#31228=VECTOR('',#107322,10.);
#31229=VECTOR('',#107323,10.);
#31230=VECTOR('',#107326,10.);
#31231=VECTOR('',#107387,10.);
#31232=VECTOR('',#107388,10.);
#31233=VECTOR('',#107395,17.3949617393671);
#31234=VECTOR('',#107398,10.);
#31235=VECTOR('',#107401,10.);
#31236=VECTOR('',#107406,10.);
#31237=VECTOR('',#107407,10.);
#31238=VECTOR('',#107410,10.);
#31239=VECTOR('',#107415,9.3949617393671);
#31240=VECTOR('',#107470,10.);
#31241=VECTOR('',#107471,10.);
#31242=VECTOR('',#107482,10.);
#31243=VECTOR('',#107483,10.);
#31244=VECTOR('',#107494,10.);
#31245=VECTOR('',#107495,10.);
#31246=VECTOR('',#107530,10.);
#31247=VECTOR('',#107533,10.);
#31248=VECTOR('',#107536,10.);
#31249=VECTOR('',#107537,10.);
#31250=VECTOR('',#107540,10.);
#31251=VECTOR('',#107545,10.);
#31252=VECTOR('',#107550,10.);
#31253=VECTOR('',#107555,9.45);
#31254=VECTOR('',#107560,10.);
#31255=VECTOR('',#107565,10.);
#31256=VECTOR('',#107568,10.);
#31257=VECTOR('',#107601,10.);
#31258=VECTOR('',#107602,10.);
#31259=VECTOR('',#107637,10.);
#31260=VECTOR('',#107640,10.);
#31261=VECTOR('',#107643,10.);
#31262=VECTOR('',#107646,10.);
#31263=VECTOR('',#107649,10.);
#31264=VECTOR('',#107654,10.);
#31265=VECTOR('',#107659,10.);
#31266=VECTOR('',#107664,0.8);
#31267=VECTOR('',#107673,10.);
#31268=VECTOR('',#107676,10.);
#31269=VECTOR('',#107687,10.);
#31270=VECTOR('',#107688,10.);
#31271=VECTOR('',#107723,10.);
#31272=VECTOR('',#107726,3.6);
#31273=VECTOR('',#107729,10.);
#31274=VECTOR('',#107734,10.);
#31275=VECTOR('',#107739,10.);
#31276=VECTOR('',#107740,10.);
#31277=VECTOR('',#107749,10.);
#31278=VECTOR('',#107754,10.);
#31279=VECTOR('',#107757,10.);
#31280=VECTOR('',#107764,10.);
#31281=VECTOR('',#107767,10.);
#31282=VECTOR('',#107770,8.45);
#31283=VECTOR('',#107783,10.);
#31284=VECTOR('',#107786,10.);
#31285=VECTOR('',#107789,10.);
#31286=VECTOR('',#107790,10.);
#31287=VECTOR('',#107791,10.);
#31288=VECTOR('',#107798,10.);
#31289=VECTOR('',#107799,10.);
#31290=VECTOR('',#107800,10.);
#31291=VECTOR('',#107801,10.);
#31292=VECTOR('',#107806,10.);
#31293=VECTOR('',#107809,10.);
#31294=VECTOR('',#107814,10.);
#31295=VECTOR('',#107817,10.);
#31296=VECTOR('',#107820,10.);
#31297=VECTOR('',#107823,10.);
#31298=VECTOR('',#107838,10.);
#31299=VECTOR('',#107841,10.);
#31300=VECTOR('',#107842,10.);
#31301=VECTOR('',#107843,10.);
#31302=VECTOR('',#107846,10.);
#31303=VECTOR('',#107849,10.);
#31304=VECTOR('',#107856,10.);
#31305=VECTOR('',#107859,10.);
#31306=VECTOR('',#107862,10.);
#31307=VECTOR('',#107865,10.);
#31308=VECTOR('',#107868,10.);
#31309=VECTOR('',#107885,10.);
#31310=VECTOR('',#107888,10.);
#31311=VECTOR('',#107891,10.);
#31312=VECTOR('',#107900,10.);
#31313=VECTOR('',#107905,10.);
#31314=VECTOR('',#107906,10.);
#31315=VECTOR('',#107907,10.);
#31316=VECTOR('',#107910,10.);
#31317=VECTOR('',#107913,10.);
#31318=VECTOR('',#107916,10.);
#31319=VECTOR('',#107917,10.);
#31320=VECTOR('',#107920,10.);
#31321=VECTOR('',#107925,10.);
#31322=VECTOR('',#107928,10.);
#31323=VECTOR('',#107933,10.);
#31324=VECTOR('',#107936,10.);
#31325=VECTOR('',#107941,10.);
#31326=VECTOR('',#107946,10.);
#31327=VECTOR('',#107949,10.);
#31328=VECTOR('',#107952,10.);
#31329=VECTOR('',#107955,10.);
#31330=VECTOR('',#107958,10.);
#31331=VECTOR('',#107969,10.);
#31332=VECTOR('',#107972,10.);
#31333=VECTOR('',#107973,10.);
#31334=VECTOR('',#107978,10.);
#31335=VECTOR('',#107981,10.);
#31336=VECTOR('',#107984,10.);
#31337=VECTOR('',#107987,10.);
#31338=VECTOR('',#107988,10.);
#31339=VECTOR('',#107991,10.);
#31340=VECTOR('',#107994,10.);
#31341=VECTOR('',#107997,10.);
#31342=VECTOR('',#107998,10.);
#31343=VECTOR('',#108003,10.);
#31344=VECTOR('',#108006,10.);
#31345=VECTOR('',#108015,10.);
#31346=VECTOR('',#108018,10.);
#31347=VECTOR('',#108021,10.);
#31348=VECTOR('',#108022,10.);
#31349=VECTOR('',#108045,10.);
#31350=VECTOR('',#108050,10.);
#31351=VECTOR('',#108055,10.);
#31352=VECTOR('',#108058,10.);
#31353=VECTOR('',#108059,10.);
#31354=VECTOR('',#108062,10.);
#31355=VECTOR('',#108065,10.);
#31356=VECTOR('',#108068,7.69496173936711);
#31357=VECTOR('',#108069,10.);
#31358=VECTOR('',#108072,7.6949617393671);
#31359=VECTOR('',#108075,10.);
#31360=VECTOR('',#108078,10.);
#31361=VECTOR('',#108081,10.);
#31362=VECTOR('',#108086,10.);
#31363=VECTOR('',#108089,10.);
#31364=VECTOR('',#108092,9.45);
#31365=VECTOR('',#108101,23.7449617393671);
#31366=VECTOR('',#108104,10.);
#31367=VECTOR('',#108107,0.4);
#31368=VECTOR('',#108112,0.8);
#31369=VECTOR('',#108113,10.);
#31370=VECTOR('',#108118,0.8);
#31371=VECTOR('',#108121,10.);
#31372=VECTOR('',#108124,10.);
#31373=VECTOR('',#108135,3.2);
#31374=VECTOR('',#108136,10.);
#31375=VECTOR('',#108139,10.);
#31376=VECTOR('',#108142,10.);
#31377=VECTOR('',#108145,10.);
#31378=VECTOR('',#108148,10.);
#31379=VECTOR('',#108153,10.);
#31380=VECTOR('',#108154,4.65);
#31381=VECTOR('',#108157,10.0999999997296);
#31382=VECTOR('',#108162,10.);
#31383=VECTOR('',#108167,10.);
#31384=VECTOR('',#108174,10.);
#31385=VECTOR('',#108177,10.);
#31386=VECTOR('',#108178,10.);
#31387=VECTOR('',#108179,10.);
#31388=VECTOR('',#108190,10.);
#31389=VECTOR('',#108193,10.);
#31390=VECTOR('',#108204,10.);
#31391=VECTOR('',#108207,10.);
#31392=VECTOR('',#108222,10.);
#31393=VECTOR('',#108229,10.);
#31394=VECTOR('',#108230,10.);
#31395=VECTOR('',#108231,10.);
#31396=VECTOR('',#108234,10.);
#31397=VECTOR('',#108243,10.);
#31398=VECTOR('',#108244,10.);
#31399=VECTOR('',#108247,4.1);
#31400=VECTOR('',#108252,10.);
#31401=VECTOR('',#108253,10.);
#31402=VECTOR('',#108256,10.);
#31403=VECTOR('',#108259,10.);
#31404=VECTOR('',#108262,10.);
#31405=VECTOR('',#108267,0.8);
#31406=VECTOR('',#108270,13.4);
#31407=VECTOR('',#108273,10.);
#31408=VECTOR('',#108284,10.);
#31409=VECTOR('',#108293,10.);
#31410=VECTOR('',#108294,10.);
#31411=VECTOR('',#108297,10.);
#31412=VECTOR('',#108300,10.);
#31413=VECTOR('',#108313,10.);
#31414=VECTOR('',#108320,10.);
#31415=VECTOR('',#108323,10.);
#31416=VECTOR('',#108338,1.6);
#31417=VECTOR('',#108345,1.6);
#31418=VECTOR('',#108348,10.);
#31419=VECTOR('',#108351,10.);
#31420=VECTOR('',#108354,10.);
#31421=VECTOR('',#108355,10.);
#31422=VECTOR('',#108358,10.);
#31423=VECTOR('',#108365,10.);
#31424=VECTOR('',#108366,10.);
#31425=VECTOR('',#108369,10.);
#31426=VECTOR('',#108370,10.);
#31427=VECTOR('',#108375,10.);
#31428=VECTOR('',#108378,10.);
#31429=VECTOR('',#108385,3.05);
#31430=VECTOR('',#108390,2.);
#31431=VECTOR('',#108395,10.);
#31432=VECTOR('',#108400,10.);
#31433=VECTOR('',#108401,10.);
#31434=VECTOR('',#108404,10.);
#31435=VECTOR('',#108405,10.);
#31436=VECTOR('',#108420,10.);
#31437=VECTOR('',#108421,10.);
#31438=VECTOR('',#108424,10.);
#31439=VECTOR('',#108429,1.6);
#31440=VECTOR('',#108432,1.55);
#31441=VECTOR('',#108435,2.15);
#31442=VECTOR('',#108438,10.);
#31443=VECTOR('',#108441,10.);
#31444=VECTOR('',#108444,10.);
#31445=VECTOR('',#108447,10.);
#31446=VECTOR('',#108450,10.);
#31447=VECTOR('',#108453,10.);
#31448=VECTOR('',#108458,10.);
#31449=VECTOR('',#108461,10.);
#31450=VECTOR('',#108462,10.);
#31451=VECTOR('',#108463,10.);
#31452=VECTOR('',#108472,10.);
#31453=VECTOR('',#108479,10.);
#31454=VECTOR('',#108482,10.);
#31455=VECTOR('',#108489,10.);
#31456=VECTOR('',#108492,10.);
#31457=VECTOR('',#108499,10.);
#31458=VECTOR('',#108502,10.);
#31459=VECTOR('',#108505,10.);
#31460=VECTOR('',#108508,10.);
#31461=VECTOR('',#108511,10.);
#31462=VECTOR('',#108514,10.);
#31463=VECTOR('',#108519,10.);
#31464=VECTOR('',#108524,10.);
#31465=VECTOR('',#108527,10.);
#31466=VECTOR('',#108528,10.);
#31467=VECTOR('',#108529,10.);
#31468=VECTOR('',#108530,10.);
#31469=VECTOR('',#108551,10.);
#31470=VECTOR('',#108562,10.);
#31471=VECTOR('',#108563,10.);
#31472=VECTOR('',#108584,10.);
#31473=VECTOR('',#108587,10.);
#31474=VECTOR('',#108590,10.);
#31475=VECTOR('',#108595,10.);
#31476=VECTOR('',#108600,10.);
#31477=VECTOR('',#108603,10.);
#31478=VECTOR('',#108628,10.);
#31479=VECTOR('',#108629,10.);
#31480=VECTOR('',#108658,10.);
#31481=VECTOR('',#108659,10.);
#31482=VECTOR('',#108662,10.);
#31483=VECTOR('',#108665,10.);
#31484=VECTOR('',#108668,10.);
#31485=VECTOR('',#108673,10.);
#31486=VECTOR('',#108674,10.);
#31487=VECTOR('',#108677,10.);
#31488=VECTOR('',#108706,0.599999999999999);
#31489=VECTOR('',#108707,10.);
#31490=VECTOR('',#108708,0.599999999999999);
#31491=VECTOR('',#108711,10.);
#31492=VECTOR('',#108712,10.);
#31493=VECTOR('',#108715,0.599999999999999);
#31494=VECTOR('',#108718,10.);
#31495=VECTOR('',#108725,10.);
#31496=VECTOR('',#108728,10.);
#31497=VECTOR('',#108731,10.);
#31498=VECTOR('',#108732,10.);
#31499=VECTOR('',#108739,10.);
#31500=VECTOR('',#108740,10.);
#31501=VECTOR('',#108741,10.);
#31502=VECTOR('',#108750,10.);
#31503=VECTOR('',#108753,10.);
#31504=VECTOR('',#108758,10.);
#31505=VECTOR('',#108763,10.);
#31506=VECTOR('',#108768,0.75);
#31507=VECTOR('',#108769,10.);
#31508=VECTOR('',#108770,10.);
#31509=VECTOR('',#108771,10.);
#31510=VECTOR('',#108772,10.);
#31511=VECTOR('',#108773,10.);
#31512=VECTOR('',#108774,10.);
#31513=VECTOR('',#108775,10.);
#31514=VECTOR('',#108776,10.);
#31515=VECTOR('',#108777,10.);
#31516=VECTOR('',#108780,10.);
#31517=VECTOR('',#108783,10.);
#31518=VECTOR('',#108788,10.);
#31519=VECTOR('',#108789,10.);
#31520=VECTOR('',#108792,10.);
#31521=VECTOR('',#108795,10.);
#31522=VECTOR('',#108796,10.);
#31523=VECTOR('',#108827,10.);
#31524=VECTOR('',#108828,10.);
#31525=VECTOR('',#108833,10.);
#31526=VECTOR('',#108834,10.);
#31527=VECTOR('',#108837,10.);
#31528=VECTOR('',#108840,10.);
#31529=VECTOR('',#108841,10.);
#31530=VECTOR('',#108842,10.);
#31531=VECTOR('',#108845,10.);
#31532=VECTOR('',#108846,10.);
#31533=VECTOR('',#108847,10.);
#31534=VECTOR('',#108850,10.);
#31535=VECTOR('',#108885,10.);
#31536=VECTOR('',#108888,10.);
#31537=VECTOR('',#108891,10.);
#31538=VECTOR('',#108896,10.);
#31539=VECTOR('',#108905,10.);
#31540=VECTOR('',#108914,10.);
#31541=VECTOR('',#108925,0.600000000000001);
#31542=VECTOR('',#108928,0.600000000000001);
#31543=VECTOR('',#108931,3.2);
#31544=VECTOR('',#108936,10.);
#31545=VECTOR('',#108941,10.);
#31546=VECTOR('',#108942,10.);
#31547=VECTOR('',#108945,10.);
#31548=VECTOR('',#108950,10.);
#31549=VECTOR('',#108951,10.);
#31550=VECTOR('',#108954,10.);
#31551=VECTOR('',#108959,10.);
#31552=VECTOR('',#108960,10.);
#31553=VECTOR('',#108963,10.);
#31554=VECTOR('',#108970,9.3);
#31555=VECTOR('',#108973,10.);
#31556=VECTOR('',#108976,10.);
#31557=VECTOR('',#109001,10.);
#31558=VECTOR('',#109002,10.);
#31559=VECTOR('',#109015,10.);
#31560=VECTOR('',#109016,10.);
#31561=VECTOR('',#109051,10.);
#31562=VECTOR('',#109052,10.);
#31563=VECTOR('',#109065,10.);
#31564=VECTOR('',#109066,10.);
#31565=VECTOR('',#109067,0.800000000000001);
#31566=VECTOR('',#109070,10.);
#31567=VECTOR('',#109075,10.);
#31568=VECTOR('',#109076,10.);
#31569=VECTOR('',#109079,10.);
#31570=VECTOR('',#109084,10.);
#31571=VECTOR('',#109089,5.7);
#31572=VECTOR('',#109098,10.);
#31573=VECTOR('',#109101,10.);
#31574=VECTOR('',#109112,10.);
#31575=VECTOR('',#109113,10.);
#31576=VECTOR('',#109132,10.);
#31577=VECTOR('',#109133,10.);
#31578=VECTOR('',#109166,10.);
#31579=VECTOR('',#109167,10.);
#31580=VECTOR('',#109174,10.);
#31581=VECTOR('',#109177,10.);
#31582=VECTOR('',#109180,19.0949617393671);
#31583=VECTOR('',#109185,10.);
#31584=VECTOR('',#109190,10.);
#31585=VECTOR('',#109191,10.);
#31586=VECTOR('',#109194,10.);
#31587=VECTOR('',#109199,10.);
#31588=VECTOR('',#109200,10.);
#31589=VECTOR('',#109207,10.);
#31590=VECTOR('',#109210,10.);
#31591=VECTOR('',#109221,10.);
#31592=VECTOR('',#109222,10.);
#31593=VECTOR('',#109233,10.);
#31594=VECTOR('',#109234,10.);
#31595=VECTOR('',#109279,6.2);
#31596=VECTOR('',#109282,4.1);
#31597=VECTOR('',#109285,10.);
#31598=VECTOR('',#109290,10.);
#31599=VECTOR('',#109293,10.);
#31600=VECTOR('',#109298,10.);
#31601=VECTOR('',#109301,10.);
#31602=VECTOR('',#109304,10.);
#31603=VECTOR('',#109309,10.);
#31604=VECTOR('',#109314,10.);
#31605=VECTOR('',#109315,10.);
#31606=VECTOR('',#109348,10.);
#31607=VECTOR('',#109349,10.);
#31608=VECTOR('',#109354,10.);
#31609=VECTOR('',#109355,10.);
#31610=VECTOR('',#109360,10.);
#31611=VECTOR('',#109363,10.);
#31612=VECTOR('',#109368,10.);
#31613=VECTOR('',#109371,10.);
#31614=VECTOR('',#109372,10.);
#31615=VECTOR('',#109375,10.);
#31616=VECTOR('',#109378,10.);
#31617=VECTOR('',#109383,12.05);
#31618=VECTOR('',#109386,10.);
#31619=VECTOR('',#109387,10.);
#31620=VECTOR('',#109390,12.05);
#31621=VECTOR('',#109391,10.);
#31622=VECTOR('',#109396,10.);
#31623=VECTOR('',#109399,10.);
#31624=VECTOR('',#109412,10.);
#31625=VECTOR('',#109413,10.);
#31626=VECTOR('',#109438,10.);
#31627=VECTOR('',#109439,10.);
#31628=VECTOR('',#109466,10.);
#31629=VECTOR('',#109467,10.);
#31630=VECTOR('',#109474,10.);
#31631=VECTOR('',#109477,10.);
#31632=VECTOR('',#109482,3.5);
#31633=VECTOR('',#109483,10.);
#31634=VECTOR('',#109486,10.);
#31635=VECTOR('',#109489,10.);
#31636=VECTOR('',#109492,10.);
#31637=VECTOR('',#109495,10.);
#31638=VECTOR('',#109500,10.);
#31639=VECTOR('',#109505,0.8);
#31640=VECTOR('',#109506,10.);
#31641=VECTOR('',#109509,0.8);
#31642=VECTOR('',#109514,0.8);
#31643=VECTOR('',#109515,10.);
#31644=VECTOR('',#109536,10.);
#31645=VECTOR('',#109537,10.);
#31646=VECTOR('',#109548,10.);
#31647=VECTOR('',#109549,10.);
#31648=VECTOR('',#109572,10.);
#31649=VECTOR('',#109573,10.);
#31650=VECTOR('',#109594,10.);
#31651=VECTOR('',#109595,10.);
#31652=VECTOR('',#109596,10.);
#31653=VECTOR('',#109599,10.);
#31654=VECTOR('',#109606,10.);
#31655=VECTOR('',#109609,10.);
#31656=VECTOR('',#109612,10.);
#31657=VECTOR('',#109619,10.);
#31658=VECTOR('',#109622,10.);
#31659=VECTOR('',#109625,10.);
#31660=VECTOR('',#109648,10.);
#31661=VECTOR('',#109649,10.);
#31662=VECTOR('',#109672,10.);
#31663=VECTOR('',#109673,10.);
#31664=VECTOR('',#109684,10.);
#31665=VECTOR('',#109685,10.);
#31666=VECTOR('',#109692,10.);
#31667=VECTOR('',#109693,10.);
#31668=VECTOR('',#109694,10.);
#31669=VECTOR('',#109697,10.);
#31670=VECTOR('',#109702,10.);
#31671=VECTOR('',#109703,10.);
#31672=VECTOR('',#109706,10.);
#31673=VECTOR('',#109711,10.);
#31674=VECTOR('',#109714,10.);
#31675=VECTOR('',#109717,10.);
#31676=VECTOR('',#109722,10.);
#31677=VECTOR('',#109729,10.);
#31678=VECTOR('',#109734,10.);
#31679=VECTOR('',#109735,10.);
#31680=VECTOR('',#109742,10.);
#31681=VECTOR('',#109753,0.4);
#31682=VECTOR('',#109756,0.4);
#31683=VECTOR('',#109759,10.);
#31684=VECTOR('',#109760,10.);
#31685=VECTOR('',#109761,10.);
#31686=VECTOR('',#109762,10.);
#31687=VECTOR('',#109763,10.);
#31688=VECTOR('',#109764,10.);
#31689=VECTOR('',#109765,10.);
#31690=VECTOR('',#109768,10.);
#31691=VECTOR('',#109769,10.);
#31692=VECTOR('',#109770,10.);
#31693=VECTOR('',#109779,10.);
#31694=VECTOR('',#109786,10.);
#31695=VECTOR('',#109793,10.);
#31696=VECTOR('',#109800,10.);
#31697=VECTOR('',#109805,10.);
#31698=VECTOR('',#109806,10.);
#31699=VECTOR('',#109807,10.);
#31700=VECTOR('',#109814,10.);
#31701=VECTOR('',#109825,1.6);
#31702=VECTOR('',#109830,2.6);
#31703=VECTOR('',#109833,10.);
#31704=VECTOR('',#109834,10.);
#31705=VECTOR('',#109835,10.);
#31706=VECTOR('',#109836,10.);
#31707=VECTOR('',#109837,10.);
#31708=VECTOR('',#109838,10.);
#31709=VECTOR('',#109839,10.);
#31710=VECTOR('',#109840,10.);
#31711=VECTOR('',#109841,10.);
#31712=VECTOR('',#109844,10.);
#31713=VECTOR('',#109849,4.2);
#31714=VECTOR('',#109860,10.);
#31715=VECTOR('',#109867,10.);
#31716=VECTOR('',#109870,10.);
#31717=VECTOR('',#109873,10.);
#31718=VECTOR('',#109874,10.);
#31719=VECTOR('',#109875,10.);
#31720=VECTOR('',#109878,10.);
#31721=VECTOR('',#109883,10.);
#31722=VECTOR('',#109884,10.);
#31723=VECTOR('',#109885,10.);
#31724=VECTOR('',#109890,10.);
#31725=VECTOR('',#109897,10.);
#31726=VECTOR('',#109900,10.);
#31727=VECTOR('',#109911,1.6);
#31728=VECTOR('',#109918,10.);
#31729=VECTOR('',#109923,10.);
#31730=VECTOR('',#109926,10.);
#31731=VECTOR('',#109931,10.);
#31732=VECTOR('',#109932,10.);
#31733=VECTOR('',#109935,10.);
#31734=VECTOR('',#109936,10.);
#31735=VECTOR('',#109941,1.3);
#31736=VECTOR('',#109946,10.);
#31737=VECTOR('',#109953,1.70000000000355);
#31738=VECTOR('',#109958,1.3);
#31739=VECTOR('',#109963,10.);
#31740=VECTOR('',#109970,1.70000000000355);
#31741=VECTOR('',#109977,10.);
#31742=VECTOR('',#109978,10.);
#31743=VECTOR('',#109981,10.);
#31744=VECTOR('',#109982,10.);
#31745=VECTOR('',#109987,10.);
#31746=VECTOR('',#109988,10.);
#31747=VECTOR('',#109991,10.);
#31748=VECTOR('',#109992,10.);
#31749=VECTOR('',#109995,10.);
#31750=VECTOR('',#109996,10.);
#31751=VECTOR('',#109997,10.);
#31752=VECTOR('',#110004,10.);
#31753=VECTOR('',#110007,10.);
#31754=VECTOR('',#110008,10.);
#31755=VECTOR('',#110011,10.);
#31756=VECTOR('',#110012,10.);
#31757=VECTOR('',#110013,10.);
#31758=VECTOR('',#110020,10.);
#31759=VECTOR('',#110023,10.);
#31760=VECTOR('',#110024,10.);
#31761=VECTOR('',#110047,10.);
#31762=VECTOR('',#110048,10.);
#31763=VECTOR('',#110049,10.);
#31764=VECTOR('',#110056,10.);
#31765=VECTOR('',#110059,10.);
#31766=VECTOR('',#110060,10.);
#31767=VECTOR('',#110065,10.);
#31768=VECTOR('',#110066,10.);
#31769=VECTOR('',#110067,10.);
#31770=VECTOR('',#110074,10.);
#31771=VECTOR('',#110077,10.);
#31772=VECTOR('',#110078,10.);
#31773=VECTOR('',#110083,10.);
#31774=VECTOR('',#110084,10.);
#31775=VECTOR('',#110085,10.);
#31776=VECTOR('',#110088,10.);
#31777=VECTOR('',#110089,10.);
#31778=VECTOR('',#110092,10.);
#31779=VECTOR('',#110093,10.);
#31780=VECTOR('',#110098,10.);
#31781=VECTOR('',#110099,10.);
#31782=VECTOR('',#110100,10.);
#31783=VECTOR('',#110105,11.95);
#31784=VECTOR('',#110106,10.);
#31785=VECTOR('',#110109,10.);
#31786=VECTOR('',#110110,10.);
#31787=VECTOR('',#110113,10.);
#31788=VECTOR('',#110116,10.);
#31789=VECTOR('',#110117,10.);
#31790=VECTOR('',#110118,10.);
#31791=VECTOR('',#110121,10.);
#31792=VECTOR('',#110134,2.);
#31793=VECTOR('',#110141,10.);
#31794=VECTOR('',#110142,10.);
#31795=VECTOR('',#110145,10.);
#31796=VECTOR('',#110150,10.);
#31797=VECTOR('',#110151,10.);
#31798=VECTOR('',#110156,10.);
#31799=VECTOR('',#110161,10.);
#31800=VECTOR('',#110178,5.79999999999998);
#31801=VECTOR('',#110183,10.);
#31802=VECTOR('',#110186,10.);
#31803=VECTOR('',#110187,10.);
#31804=VECTOR('',#110188,10.);
#31805=VECTOR('',#110191,10.);
#31806=VECTOR('',#110194,10.);
#31807=VECTOR('',#110195,10.);
#31808=VECTOR('',#110196,10.);
#31809=VECTOR('',#110207,10.);
#31810=VECTOR('',#110208,10.);
#31811=VECTOR('',#110215,10.);
#31812=VECTOR('',#110220,10.);
#31813=VECTOR('',#110231,10.);
#31814=VECTOR('',#110234,10.);
#31815=VECTOR('',#110237,10.);
#31816=VECTOR('',#110240,10.);
#31817=VECTOR('',#110243,10.);
#31818=VECTOR('',#110244,10.);
#31819=VECTOR('',#110245,10.);
#31820=VECTOR('',#110246,10.);
#31821=VECTOR('',#110249,10.);
#31822=VECTOR('',#110252,10.);
#31823=VECTOR('',#110255,0.599999999999999);
#31824=VECTOR('',#110266,10.);
#31825=VECTOR('',#110279,10.);
#31826=VECTOR('',#110282,10.);
#31827=VECTOR('',#110285,10.);
#31828=VECTOR('',#110288,10.);
#31829=VECTOR('',#110293,0.800000000000001);
#31830=VECTOR('',#110298,10.);
#31831=VECTOR('',#110307,3.95);
#31832=VECTOR('',#110316,4.15);
#31833=VECTOR('',#110321,2.25);
#31834=VECTOR('',#110328,2.6);
#31835=VECTOR('',#110337,1.6);
#31836=VECTOR('',#110342,10.);
#31837=VECTOR('',#110347,2.14999999999987);
#31838=VECTOR('',#110352,2.);
#31839=VECTOR('',#110359,10.);
#31840=VECTOR('',#110362,10.);
#31841=VECTOR('',#110365,10.);
#31842=VECTOR('',#110368,10.);
#31843=VECTOR('',#110373,10.);
#31844=VECTOR('',#110380,10.);
#31845=VECTOR('',#110385,10.);
#31846=VECTOR('',#110386,10.);
#31847=VECTOR('',#110391,10.);
#31848=VECTOR('',#110394,10.);
#31849=VECTOR('',#110397,10.);
#31850=VECTOR('',#110398,10.);
#31851=VECTOR('',#110403,3.1);
#31852=VECTOR('',#110408,10.);
#31853=VECTOR('',#110409,10.);
#31854=VECTOR('',#110412,10.);
#31855=VECTOR('',#110419,10.);
#31856=VECTOR('',#110422,10.);
#31857=VECTOR('',#110427,10.);
#31858=VECTOR('',#110446,1.55);
#31859=VECTOR('',#110451,1.5);
#31860=VECTOR('',#110474,1.65);
#31861=VECTOR('',#110479,3.625);
#31862=VECTOR('',#110490,1.1);
#31863=VECTOR('',#110507,2.1);
#31864=VECTOR('',#110534,0.75);
#31865=VECTOR('',#110537,10.);
#31866=VECTOR('',#110544,10.);
#31867=VECTOR('',#110545,10.);
#31868=VECTOR('',#110546,10.);
#31869=VECTOR('',#110547,10.);
#31870=VECTOR('',#110550,10.);
#31871=VECTOR('',#110551,10.);
#31872=VECTOR('',#110552,10.);
#31873=VECTOR('',#110569,10.);
#31874=VECTOR('',#110570,10.);
#31875=VECTOR('',#110605,10.);
#31876=VECTOR('',#110612,0.6);
#31877=VECTOR('',#110615,10.);
#31878=VECTOR('',#110630,10.);
#31879=VECTOR('',#110631,10.);
#31880=VECTOR('',#110632,10.);
#31881=VECTOR('',#110639,4.1);
#31882=VECTOR('',#110648,10.);
#31883=VECTOR('',#110649,10.);
#31884=VECTOR('',#110650,10.);
#31885=VECTOR('',#110651,10.);
#31886=VECTOR('',#110656,10.);
#31887=VECTOR('',#110663,10.);
#31888=VECTOR('',#110666,10.);
#31889=VECTOR('',#110669,10.);
#31890=VECTOR('',#110670,10.);
#31891=VECTOR('',#110671,10.);
#31892=VECTOR('',#110676,10.);
#31893=VECTOR('',#110689,10.);
#31894=VECTOR('',#110694,10.);
#31895=VECTOR('',#110703,10.);
#31896=VECTOR('',#110704,10.);
#31897=VECTOR('',#110711,10.);
#31898=VECTOR('',#110712,10.);
#31899=VECTOR('',#110713,10.);
#31900=VECTOR('',#110714,10.);
#31901=VECTOR('',#110723,10.);
#31902=VECTOR('',#110724,10.);
#31903=VECTOR('',#110725,10.);
#31904=VECTOR('',#110726,10.);
#31905=VECTOR('',#110727,10.);
#31906=VECTOR('',#110728,10.);
#31907=VECTOR('',#110729,10.);
#31908=VECTOR('',#110734,10.);
#31909=VECTOR('',#110737,10.);
#31910=VECTOR('',#110738,10.);
#31911=VECTOR('',#110747,10.);
#31912=VECTOR('',#110750,10.);
#31913=VECTOR('',#110751,10.);
#31914=VECTOR('',#110754,10.);
#31915=VECTOR('',#110755,10.);
#31916=VECTOR('',#110760,10.);
#31917=VECTOR('',#110763,10.);
#31918=VECTOR('',#110768,10.);
#31919=VECTOR('',#110777,10.);
#31920=VECTOR('',#110784,10.);
#31921=VECTOR('',#110793,10.);
#31922=VECTOR('',#110808,3.05);
#31923=VECTOR('',#110817,3.15);
#31924=VECTOR('',#110820,10.);
#31925=VECTOR('',#110821,10.);
#31926=VECTOR('',#110822,10.);
#31927=VECTOR('',#110827,10.);
#31928=VECTOR('',#110832,10.);
#31929=VECTOR('',#110835,10.);
#31930=VECTOR('',#110840,10.);
#31931=VECTOR('',#110845,10.);
#31932=VECTOR('',#110848,10.);
#31933=VECTOR('',#110867,1.);
#31934=VECTOR('',#110874,10.);
#31935=VECTOR('',#110879,10.);
#31936=VECTOR('',#110880,10.);
#31937=VECTOR('',#110881,10.);
#31938=VECTOR('',#110882,10.);
#31939=VECTOR('',#110885,10.);
#31940=VECTOR('',#110886,10.);
#31941=VECTOR('',#110887,10.);
#31942=VECTOR('',#110888,10.);
#31943=VECTOR('',#110899,10.);
#31944=VECTOR('',#110900,10.);
#31945=VECTOR('',#110927,10.);
#31946=VECTOR('',#110928,10.);
#31947=VECTOR('',#110929,10.);
#31948=VECTOR('',#110956,10.);
#31949=VECTOR('',#110959,10.);
#31950=VECTOR('',#110962,10.);
#31951=VECTOR('',#110963,10.);
#31952=VECTOR('',#110972,10.);
#31953=VECTOR('',#110975,10.);
#31954=VECTOR('',#110978,10.);
#31955=VECTOR('',#110989,10.);
#31956=VECTOR('',#111000,10.);
#31957=VECTOR('',#111003,10.);
#31958=VECTOR('',#111006,10.);
#31959=VECTOR('',#111013,4.1);
#31960=VECTOR('',#111018,10.);
#31961=VECTOR('',#111021,10.);
#31962=VECTOR('',#111024,10.);
#31963=VECTOR('',#111037,10.);
#31964=VECTOR('',#111038,10.);
#31965=VECTOR('',#111039,10.);
#31966=VECTOR('',#111044,10.);
#31967=VECTOR('',#111049,10.);
#31968=VECTOR('',#111050,10.);
#31969=VECTOR('',#111057,1.);
#31970=VECTOR('',#111070,10.);
#35074=VERTEX_POINT('',#138717);
#35075=VERTEX_POINT('',#138718);
#35076=VERTEX_POINT('',#138720);
#35077=VERTEX_POINT('',#138722);
#35078=VERTEX_POINT('',#138740);
#35079=VERTEX_POINT('',#138741);
#35080=VERTEX_POINT('',#138746);
#35081=VERTEX_POINT('',#138747);
#35082=VERTEX_POINT('',#138766);
#35083=VERTEX_POINT('',#138767);
#35084=VERTEX_POINT('',#138772);
#35085=VERTEX_POINT('',#138773);
#35086=VERTEX_POINT('',#138792);
#35087=VERTEX_POINT('',#138793);
#35088=VERTEX_POINT('',#138798);
#35089=VERTEX_POINT('',#138799);
#35090=VERTEX_POINT('',#138812);
#35091=VERTEX_POINT('',#138813);
#35092=VERTEX_POINT('',#138818);
#35093=VERTEX_POINT('',#138819);
#35094=VERTEX_POINT('',#138835);
#35095=VERTEX_POINT('',#138837);
#35096=VERTEX_POINT('',#138839);
#35097=VERTEX_POINT('',#138841);
#35098=VERTEX_POINT('',#138843);
#35099=VERTEX_POINT('',#138845);
#35100=VERTEX_POINT('',#138853);
#35101=VERTEX_POINT('',#138855);
#35102=VERTEX_POINT('',#138859);
#35103=VERTEX_POINT('',#138863);
#35104=VERTEX_POINT('',#138867);
#35105=VERTEX_POINT('',#138871);
#35106=VERTEX_POINT('',#138876);
#35107=VERTEX_POINT('',#138877);
#35108=VERTEX_POINT('',#138879);
#35109=VERTEX_POINT('',#138881);
#35110=VERTEX_POINT('',#138893);
#35111=VERTEX_POINT('',#138894);
#35112=VERTEX_POINT('',#138899);
#35113=VERTEX_POINT('',#138900);
#35114=VERTEX_POINT('',#138919);
#35115=VERTEX_POINT('',#138920);
#35116=VERTEX_POINT('',#138925);
#35117=VERTEX_POINT('',#138926);
#35118=VERTEX_POINT('',#138939);
#35119=VERTEX_POINT('',#138940);
#35120=VERTEX_POINT('',#138945);
#35121=VERTEX_POINT('',#138946);
#35122=VERTEX_POINT('',#138951);
#35123=VERTEX_POINT('',#138952);
#35124=VERTEX_POINT('',#138957);
#35125=VERTEX_POINT('',#138958);
#35126=VERTEX_POINT('',#138977);
#35127=VERTEX_POINT('',#138978);
#35128=VERTEX_POINT('',#138983);
#35129=VERTEX_POINT('',#138984);
#35130=VERTEX_POINT('',#138997);
#35131=VERTEX_POINT('',#138998);
#35132=VERTEX_POINT('',#139003);
#35133=VERTEX_POINT('',#139004);
#35134=VERTEX_POINT('',#139006);
#35135=VERTEX_POINT('',#139022);
#35136=VERTEX_POINT('',#139024);
#35137=VERTEX_POINT('',#139028);
#35138=VERTEX_POINT('',#139032);
#35139=VERTEX_POINT('',#139036);
#35140=VERTEX_POINT('',#139040);
#35141=VERTEX_POINT('',#139043);
#35142=VERTEX_POINT('',#139045);
#35143=VERTEX_POINT('',#139047);
#35144=VERTEX_POINT('',#139049);
#35145=VERTEX_POINT('',#139051);
#35146=VERTEX_POINT('',#139053);
#35147=VERTEX_POINT('',#139055);
#35148=VERTEX_POINT('',#139057);
#35149=VERTEX_POINT('',#139059);
#35150=VERTEX_POINT('',#139063);
#35151=VERTEX_POINT('',#139067);
#35152=VERTEX_POINT('',#139072);
#35153=VERTEX_POINT('',#139073);
#35154=VERTEX_POINT('',#139075);
#35155=VERTEX_POINT('',#139077);
#35156=VERTEX_POINT('',#139089);
#35157=VERTEX_POINT('',#139090);
#35158=VERTEX_POINT('',#139095);
#35159=VERTEX_POINT('',#139096);
#35160=VERTEX_POINT('',#139115);
#35161=VERTEX_POINT('',#139116);
#35162=VERTEX_POINT('',#139121);
#35163=VERTEX_POINT('',#139122);
#35164=VERTEX_POINT('',#139141);
#35165=VERTEX_POINT('',#139142);
#35166=VERTEX_POINT('',#139147);
#35167=VERTEX_POINT('',#139148);
#35168=VERTEX_POINT('',#139161);
#35169=VERTEX_POINT('',#139162);
#35170=VERTEX_POINT('',#139167);
#35171=VERTEX_POINT('',#139168);
#35172=VERTEX_POINT('',#139181);
#35173=VERTEX_POINT('',#139186);
#35174=VERTEX_POINT('',#139201);
#35175=VERTEX_POINT('',#139203);
#35176=VERTEX_POINT('',#139205);
#35177=VERTEX_POINT('',#139207);
#35178=VERTEX_POINT('',#139211);
#35179=VERTEX_POINT('',#139217);
#35180=VERTEX_POINT('',#139221);
#35181=VERTEX_POINT('',#139226);
#35182=VERTEX_POINT('',#139227);
#35183=VERTEX_POINT('',#139229);
#35184=VERTEX_POINT('',#139231);
#35185=VERTEX_POINT('',#139243);
#35186=VERTEX_POINT('',#139244);
#35187=VERTEX_POINT('',#139249);
#35188=VERTEX_POINT('',#139250);
#35189=VERTEX_POINT('',#139263);
#35190=VERTEX_POINT('',#139264);
#35191=VERTEX_POINT('',#139269);
#35192=VERTEX_POINT('',#139270);
#35193=VERTEX_POINT('',#139275);
#35194=VERTEX_POINT('',#139276);
#35195=VERTEX_POINT('',#139281);
#35196=VERTEX_POINT('',#139282);
#35197=VERTEX_POINT('',#139287);
#35198=VERTEX_POINT('',#139288);
#35199=VERTEX_POINT('',#139307);
#35200=VERTEX_POINT('',#139308);
#35201=VERTEX_POINT('',#139313);
#35202=VERTEX_POINT('',#139314);
#35203=VERTEX_POINT('',#139330);
#35204=VERTEX_POINT('',#139332);
#35205=VERTEX_POINT('',#139334);
#35206=VERTEX_POINT('',#139336);
#35207=VERTEX_POINT('',#139340);
#35208=VERTEX_POINT('',#139344);
#35209=VERTEX_POINT('',#139348);
#35210=VERTEX_POINT('',#139352);
#35211=VERTEX_POINT('',#139356);
#35212=VERTEX_POINT('',#139358);
#35213=VERTEX_POINT('',#139360);
#35214=VERTEX_POINT('',#139365);
#35215=VERTEX_POINT('',#139366);
#35216=VERTEX_POINT('',#139368);
#35217=VERTEX_POINT('',#139370);
#35218=VERTEX_POINT('',#139388);
#35219=VERTEX_POINT('',#139389);
#35220=VERTEX_POINT('',#139394);
#35221=VERTEX_POINT('',#139395);
#35222=VERTEX_POINT('',#139400);
#35223=VERTEX_POINT('',#139401);
#35224=VERTEX_POINT('',#139420);
#35225=VERTEX_POINT('',#139421);
#35226=VERTEX_POINT('',#139426);
#35227=VERTEX_POINT('',#139427);
#35228=VERTEX_POINT('',#139432);
#35229=VERTEX_POINT('',#139433);
#35230=VERTEX_POINT('',#139438);
#35231=VERTEX_POINT('',#139439);
#35232=VERTEX_POINT('',#139452);
#35233=VERTEX_POINT('',#139453);
#35234=VERTEX_POINT('',#139458);
#35235=VERTEX_POINT('',#139459);
#35236=VERTEX_POINT('',#139478);
#35237=VERTEX_POINT('',#139479);
#35238=VERTEX_POINT('',#139484);
#35239=VERTEX_POINT('',#139485);
#35240=VERTEX_POINT('',#139504);
#35241=VERTEX_POINT('',#139505);
#35242=VERTEX_POINT('',#139513);
#35243=VERTEX_POINT('',#139515);
#35244=VERTEX_POINT('',#139519);
#35245=VERTEX_POINT('',#139523);
#35246=VERTEX_POINT('',#139527);
#35247=VERTEX_POINT('',#139531);
#35248=VERTEX_POINT('',#139535);
#35249=VERTEX_POINT('',#139539);
#35250=VERTEX_POINT('',#139544);
#35251=VERTEX_POINT('',#139545);
#35252=VERTEX_POINT('',#139547);
#35253=VERTEX_POINT('',#139549);
#35254=VERTEX_POINT('',#139553);
#35255=VERTEX_POINT('',#139554);
#35256=VERTEX_POINT('',#139573);
#35257=VERTEX_POINT('',#139574);
#35258=VERTEX_POINT('',#139579);
#35259=VERTEX_POINT('',#139580);
#35260=VERTEX_POINT('',#139593);
#35261=VERTEX_POINT('',#139594);
#35262=VERTEX_POINT('',#139599);
#35263=VERTEX_POINT('',#139600);
#35264=VERTEX_POINT('',#139619);
#35265=VERTEX_POINT('',#139620);
#35266=VERTEX_POINT('',#139625);
#35267=VERTEX_POINT('',#139626);
#35268=VERTEX_POINT('',#139642);
#35269=VERTEX_POINT('',#139644);
#35270=VERTEX_POINT('',#139648);
#35271=VERTEX_POINT('',#139652);
#35272=VERTEX_POINT('',#139656);
#35273=VERTEX_POINT('',#139660);
#35274=VERTEX_POINT('',#139665);
#35275=VERTEX_POINT('',#139666);
#35276=VERTEX_POINT('',#139668);
#35277=VERTEX_POINT('',#139670);
#35278=VERTEX_POINT('',#139682);
#35279=VERTEX_POINT('',#139683);
#35280=VERTEX_POINT('',#139688);
#35281=VERTEX_POINT('',#139689);
#35282=VERTEX_POINT('',#139694);
#35283=VERTEX_POINT('',#139695);
#35284=VERTEX_POINT('',#139700);
#35285=VERTEX_POINT('',#139701);
#35286=VERTEX_POINT('',#139714);
#35287=VERTEX_POINT('',#139715);
#35288=VERTEX_POINT('',#139720);
#35289=VERTEX_POINT('',#139721);
#35290=VERTEX_POINT('',#139740);
#35291=VERTEX_POINT('',#139741);
#35292=VERTEX_POINT('',#139746);
#35293=VERTEX_POINT('',#139747);
#35294=VERTEX_POINT('',#139760);
#35295=VERTEX_POINT('',#139761);
#35296=VERTEX_POINT('',#139766);
#35297=VERTEX_POINT('',#139767);
#35298=VERTEX_POINT('',#139780);
#35299=VERTEX_POINT('',#139781);
#35300=VERTEX_POINT('',#139786);
#35301=VERTEX_POINT('',#139787);
#35302=VERTEX_POINT('',#139800);
#35303=VERTEX_POINT('',#139801);
#35304=VERTEX_POINT('',#139806);
#35305=VERTEX_POINT('',#139807);
#35306=VERTEX_POINT('',#139829);
#35307=VERTEX_POINT('',#139831);
#35308=VERTEX_POINT('',#139835);
#35309=VERTEX_POINT('',#139839);
#35310=VERTEX_POINT('',#139843);
#35311=VERTEX_POINT('',#139847);
#35312=VERTEX_POINT('',#139851);
#35313=VERTEX_POINT('',#139855);
#35314=VERTEX_POINT('',#139859);
#35315=VERTEX_POINT('',#139861);
#35316=VERTEX_POINT('',#139863);
#35317=VERTEX_POINT('',#139868);
#35318=VERTEX_POINT('',#139869);
#35319=VERTEX_POINT('',#139871);
#35320=VERTEX_POINT('',#139873);
#35321=VERTEX_POINT('',#139891);
#35322=VERTEX_POINT('',#139892);
#35323=VERTEX_POINT('',#139897);
#35324=VERTEX_POINT('',#139898);
#35325=VERTEX_POINT('',#139903);
#35326=VERTEX_POINT('',#139904);
#35327=VERTEX_POINT('',#139917);
#35328=VERTEX_POINT('',#139918);
#35329=VERTEX_POINT('',#139923);
#35330=VERTEX_POINT('',#139924);
#35331=VERTEX_POINT('',#139943);
#35332=VERTEX_POINT('',#139944);
#35333=VERTEX_POINT('',#139949);
#35334=VERTEX_POINT('',#139950);
#35335=VERTEX_POINT('',#139972);
#35336=VERTEX_POINT('',#139974);
#35337=VERTEX_POINT('',#139976);
#35338=VERTEX_POINT('',#139978);
#35339=VERTEX_POINT('',#139980);
#35340=VERTEX_POINT('',#139982);
#35341=VERTEX_POINT('',#139986);
#35342=VERTEX_POINT('',#139990);
#35343=VERTEX_POINT('',#139994);
#35344=VERTEX_POINT('',#139998);
#35345=VERTEX_POINT('',#140003);
#35346=VERTEX_POINT('',#140004);
#35347=VERTEX_POINT('',#140006);
#35348=VERTEX_POINT('',#140008);
#35349=VERTEX_POINT('',#140020);
#35350=VERTEX_POINT('',#140021);
#35351=VERTEX_POINT('',#140026);
#35352=VERTEX_POINT('',#140027);
#35353=VERTEX_POINT('',#140046);
#35354=VERTEX_POINT('',#140047);
#35355=VERTEX_POINT('',#140052);
#35356=VERTEX_POINT('',#140053);
#35357=VERTEX_POINT('',#140072);
#35358=VERTEX_POINT('',#140073);
#35359=VERTEX_POINT('',#140078);
#35360=VERTEX_POINT('',#140079);
#35361=VERTEX_POINT('',#140101);
#35362=VERTEX_POINT('',#140103);
#35363=VERTEX_POINT('',#140107);
#35364=VERTEX_POINT('',#140111);
#35365=VERTEX_POINT('',#140115);
#35366=VERTEX_POINT('',#140164);
#35367=VERTEX_POINT('',#140165);
#35368=VERTEX_POINT('',#140197);
#35369=VERTEX_POINT('',#140207);
#35370=VERTEX_POINT('',#140242);
#35371=VERTEX_POINT('',#140291);
#35372=VERTEX_POINT('',#140328);
#35373=VERTEX_POINT('',#140332);
#35374=VERTEX_POINT('',#140334);
#35375=VERTEX_POINT('',#140336);
#35376=VERTEX_POINT('',#140338);
#35377=VERTEX_POINT('',#140340);
#35378=VERTEX_POINT('',#140347);
#35379=VERTEX_POINT('',#140349);
#35380=VERTEX_POINT('',#140357);
#35381=VERTEX_POINT('',#140359);
#35382=VERTEX_POINT('',#140361);
#35383=VERTEX_POINT('',#140363);
#35384=VERTEX_POINT('',#140365);
#35385=VERTEX_POINT('',#140367);
#35386=VERTEX_POINT('',#140385);
#35387=VERTEX_POINT('',#140387);
#35388=VERTEX_POINT('',#140391);
#35389=VERTEX_POINT('',#140393);
#35390=VERTEX_POINT('',#140395);
#35391=VERTEX_POINT('',#140397);
#35392=VERTEX_POINT('',#140399);
#35393=VERTEX_POINT('',#140404);
#35394=VERTEX_POINT('',#140406);
#35395=VERTEX_POINT('',#140408);
#35396=VERTEX_POINT('',#140412);
#35397=VERTEX_POINT('',#140413);
#35398=VERTEX_POINT('',#140415);
#35399=VERTEX_POINT('',#140417);
#35400=VERTEX_POINT('',#140421);
#35401=VERTEX_POINT('',#140423);
#35402=VERTEX_POINT('',#140425);
#35403=VERTEX_POINT('',#140428);
#35404=VERTEX_POINT('',#140430);
#35405=VERTEX_POINT('',#140432);
#35406=VERTEX_POINT('',#140434);
#35407=VERTEX_POINT('',#140436);
#35408=VERTEX_POINT('',#140439);
#35409=VERTEX_POINT('',#140441);
#35410=VERTEX_POINT('',#140443);
#35411=VERTEX_POINT('',#140445);
#35412=VERTEX_POINT('',#140447);
#35413=VERTEX_POINT('',#140449);
#35414=VERTEX_POINT('',#140451);
#35415=VERTEX_POINT('',#140453);
#35416=VERTEX_POINT('',#140455);
#35417=VERTEX_POINT('',#140457);
#35418=VERTEX_POINT('',#140459);
#35419=VERTEX_POINT('',#140461);
#35420=VERTEX_POINT('',#140463);
#35421=VERTEX_POINT('',#140466);
#35422=VERTEX_POINT('',#140469);
#35423=VERTEX_POINT('',#140473);
#35424=VERTEX_POINT('',#140475);
#35425=VERTEX_POINT('',#140477);
#35426=VERTEX_POINT('',#140479);
#35427=VERTEX_POINT('',#140481);
#35428=VERTEX_POINT('',#140483);
#35429=VERTEX_POINT('',#140485);
#35430=VERTEX_POINT('',#140487);
#35431=VERTEX_POINT('',#140491);
#35432=VERTEX_POINT('',#140493);
#35433=VERTEX_POINT('',#140495);
#35434=VERTEX_POINT('',#140497);
#35435=VERTEX_POINT('',#140500);
#35436=VERTEX_POINT('',#140502);
#35437=VERTEX_POINT('',#140505);
#35438=VERTEX_POINT('',#140506);
#35439=VERTEX_POINT('',#140509);
#35440=VERTEX_POINT('',#140511);
#35441=VERTEX_POINT('',#140513);
#35442=VERTEX_POINT('',#140515);
#35443=VERTEX_POINT('',#140518);
#35444=VERTEX_POINT('',#140521);
#35445=VERTEX_POINT('',#140523);
#35446=VERTEX_POINT('',#140527);
#35447=VERTEX_POINT('',#140529);
#35448=VERTEX_POINT('',#140533);
#35449=VERTEX_POINT('',#140537);
#35450=VERTEX_POINT('',#140540);
#35451=VERTEX_POINT('',#140542);
#35452=VERTEX_POINT('',#140544);
#35453=VERTEX_POINT('',#140546);
#35454=VERTEX_POINT('',#140549);
#35455=VERTEX_POINT('',#140551);
#35456=VERTEX_POINT('',#140553);
#35457=VERTEX_POINT('',#140555);
#35458=VERTEX_POINT('',#140557);
#35459=VERTEX_POINT('',#140559);
#35460=VERTEX_POINT('',#140561);
#35461=VERTEX_POINT('',#140563);
#35462=VERTEX_POINT('',#140565);
#35463=VERTEX_POINT('',#140567);
#35464=VERTEX_POINT('',#140569);
#35465=VERTEX_POINT('',#140571);
#35466=VERTEX_POINT('',#140573);
#35467=VERTEX_POINT('',#140575);
#35468=VERTEX_POINT('',#140578);
#35469=VERTEX_POINT('',#140579);
#35470=VERTEX_POINT('',#140581);
#35471=VERTEX_POINT('',#140583);
#35472=VERTEX_POINT('',#140586);
#35473=VERTEX_POINT('',#140588);
#35474=VERTEX_POINT('',#140590);
#35475=VERTEX_POINT('',#140595);
#35476=VERTEX_POINT('',#140597);
#35477=VERTEX_POINT('',#140603);
#35478=VERTEX_POINT('',#140607);
#35479=VERTEX_POINT('',#140609);
#35480=VERTEX_POINT('',#140613);
#35481=VERTEX_POINT('',#140615);
#35482=VERTEX_POINT('',#140621);
#35483=VERTEX_POINT('',#140623);
#35484=VERTEX_POINT('',#140625);
#35485=VERTEX_POINT('',#140627);
#35486=VERTEX_POINT('',#140629);
#35487=VERTEX_POINT('',#140631);
#35488=VERTEX_POINT('',#140633);
#35489=VERTEX_POINT('',#140635);
#35490=VERTEX_POINT('',#140637);
#35491=VERTEX_POINT('',#140639);
#35492=VERTEX_POINT('',#140642);
#35493=VERTEX_POINT('',#140647);
#35494=VERTEX_POINT('',#140649);
#35495=VERTEX_POINT('',#140653);
#35496=VERTEX_POINT('',#140659);
#35497=VERTEX_POINT('',#140661);
#35498=VERTEX_POINT('',#140663);
#35499=VERTEX_POINT('',#140665);
#35500=VERTEX_POINT('',#140669);
#35501=VERTEX_POINT('',#140671);
#35502=VERTEX_POINT('',#140673);
#35503=VERTEX_POINT('',#140676);
#35504=VERTEX_POINT('',#140679);
#35505=VERTEX_POINT('',#140703);
#35506=VERTEX_POINT('',#140705);
#35507=VERTEX_POINT('',#140709);
#35508=VERTEX_POINT('',#140715);
#35509=VERTEX_POINT('',#140717);
#35510=VERTEX_POINT('',#140721);
#35511=VERTEX_POINT('',#140726);
#35512=VERTEX_POINT('',#140767);
#35513=VERTEX_POINT('',#140769);
#35514=VERTEX_POINT('',#140774);
#35515=VERTEX_POINT('',#140777);
#35516=VERTEX_POINT('',#140785);
#35517=VERTEX_POINT('',#140788);
#35518=VERTEX_POINT('',#140790);
#35519=VERTEX_POINT('',#140799);
#35520=VERTEX_POINT('',#140805);
#35521=VERTEX_POINT('',#140807);
#35522=VERTEX_POINT('',#140811);
#35523=VERTEX_POINT('',#140848);
#35524=VERTEX_POINT('',#140850);
#35525=VERTEX_POINT('',#140852);
#35526=VERTEX_POINT('',#140854);
#35527=VERTEX_POINT('',#140856);
#35528=VERTEX_POINT('',#140858);
#35529=VERTEX_POINT('',#140862);
#35530=VERTEX_POINT('',#140878);
#35531=VERTEX_POINT('',#140881);
#35532=VERTEX_POINT('',#140885);
#35533=VERTEX_POINT('',#140890);
#35534=VERTEX_POINT('',#140892);
#35535=VERTEX_POINT('',#140896);
#35536=VERTEX_POINT('',#140900);
#35537=VERTEX_POINT('',#140904);
#35538=VERTEX_POINT('',#140905);
#35539=VERTEX_POINT('',#140910);
#35540=VERTEX_POINT('',#140914);
#35541=VERTEX_POINT('',#140920);
#35542=VERTEX_POINT('',#140925);
#35543=VERTEX_POINT('',#140929);
#35544=VERTEX_POINT('',#140933);
#35545=VERTEX_POINT('',#140934);
#35546=VERTEX_POINT('',#140939);
#35547=VERTEX_POINT('',#140948);
#35548=VERTEX_POINT('',#140949);
#35549=VERTEX_POINT('',#140952);
#35550=VERTEX_POINT('',#140954);
#35551=VERTEX_POINT('',#140978);
#35552=VERTEX_POINT('',#140979);
#35553=VERTEX_POINT('',#140990);
#35554=VERTEX_POINT('',#141001);
#35555=VERTEX_POINT('',#141003);
#35556=VERTEX_POINT('',#141007);
#35557=VERTEX_POINT('',#141014);
#35558=VERTEX_POINT('',#141015);
#35559=VERTEX_POINT('',#141017);
#35560=VERTEX_POINT('',#141019);
#35561=VERTEX_POINT('',#141023);
#35562=VERTEX_POINT('',#141025);
#35563=VERTEX_POINT('',#141027);
#35564=VERTEX_POINT('',#141029);
#35565=VERTEX_POINT('',#141031);
#35566=VERTEX_POINT('',#141033);
#35567=VERTEX_POINT('',#141035);
#35568=VERTEX_POINT('',#141037);
#35569=VERTEX_POINT('',#141039);
#35570=VERTEX_POINT('',#141041);
#35571=VERTEX_POINT('',#141043);
#35572=VERTEX_POINT('',#141045);
#35573=VERTEX_POINT('',#141047);
#35574=VERTEX_POINT('',#141049);
#35575=VERTEX_POINT('',#141051);
#35576=VERTEX_POINT('',#141053);
#35577=VERTEX_POINT('',#141055);
#35578=VERTEX_POINT('',#141057);
#35579=VERTEX_POINT('',#141061);
#35580=VERTEX_POINT('',#141065);
#35581=VERTEX_POINT('',#141069);
#35582=VERTEX_POINT('',#141071);
#35583=VERTEX_POINT('',#141073);
#35584=VERTEX_POINT('',#141077);
#35585=VERTEX_POINT('',#141078);
#35586=VERTEX_POINT('',#141080);
#35587=VERTEX_POINT('',#141082);
#35588=VERTEX_POINT('',#141100);
#35589=VERTEX_POINT('',#141105);
#35590=VERTEX_POINT('',#141117);
#35591=VERTEX_POINT('',#141118);
#35592=VERTEX_POINT('',#141123);
#35593=VERTEX_POINT('',#141124);
#35594=VERTEX_POINT('',#141143);
#35595=VERTEX_POINT('',#141144);
#35596=VERTEX_POINT('',#141149);
#35597=VERTEX_POINT('',#141150);
#35598=VERTEX_POINT('',#141172);
#35599=VERTEX_POINT('',#141174);
#35600=VERTEX_POINT('',#141178);
#35601=VERTEX_POINT('',#141182);
#35602=VERTEX_POINT('',#141186);
#35603=VERTEX_POINT('',#141188);
#35604=VERTEX_POINT('',#141190);
#35605=VERTEX_POINT('',#141195);
#35606=VERTEX_POINT('',#141196);
#35607=VERTEX_POINT('',#141198);
#35608=VERTEX_POINT('',#141200);
#35609=VERTEX_POINT('',#141217);
#35610=VERTEX_POINT('',#141218);
#35611=VERTEX_POINT('',#141220);
#35612=VERTEX_POINT('',#141222);
#35613=VERTEX_POINT('',#141239);
#35614=VERTEX_POINT('',#141240);
#35615=VERTEX_POINT('',#141248);
#35616=VERTEX_POINT('',#141249);
#35617=VERTEX_POINT('',#141251);
#35618=VERTEX_POINT('',#141253);
#35619=VERTEX_POINT('',#141273);
#35620=VERTEX_POINT('',#141275);
#35621=VERTEX_POINT('',#141297);
#35622=VERTEX_POINT('',#141299);
#35623=VERTEX_POINT('',#141303);
#35624=VERTEX_POINT('',#141307);
#35625=VERTEX_POINT('',#141311);
#35626=VERTEX_POINT('',#141316);
#35627=VERTEX_POINT('',#141317);
#35628=VERTEX_POINT('',#141330);
#35629=VERTEX_POINT('',#141332);
#35630=VERTEX_POINT('',#141334);
#35631=VERTEX_POINT('',#141359);
#35632=VERTEX_POINT('',#141360);
#35633=VERTEX_POINT('',#141365);
#35634=VERTEX_POINT('',#141366);
#35635=VERTEX_POINT('',#141373);
#35636=VERTEX_POINT('',#141375);
#35637=VERTEX_POINT('',#141391);
#35638=VERTEX_POINT('',#141400);
#35639=VERTEX_POINT('',#141402);
#35640=VERTEX_POINT('',#141407);
#35641=VERTEX_POINT('',#141409);
#35642=VERTEX_POINT('',#141414);
#35643=VERTEX_POINT('',#141416);
#35644=VERTEX_POINT('',#141418);
#35645=VERTEX_POINT('',#141420);
#35646=VERTEX_POINT('',#141427);
#35647=VERTEX_POINT('',#141434);
#35648=VERTEX_POINT('',#141449);
#35649=VERTEX_POINT('',#141456);
#35650=VERTEX_POINT('',#141471);
#35651=VERTEX_POINT('',#141473);
#35652=VERTEX_POINT('',#141475);
#35653=VERTEX_POINT('',#141491);
#35654=VERTEX_POINT('',#141509);
#35655=VERTEX_POINT('',#141511);
#35656=VERTEX_POINT('',#141515);
#35657=VERTEX_POINT('',#141517);
#35658=VERTEX_POINT('',#141521);
#35659=VERTEX_POINT('',#141523);
#35660=VERTEX_POINT('',#141525);
#35661=VERTEX_POINT('',#141529);
#35662=VERTEX_POINT('',#141531);
#35663=VERTEX_POINT('',#141535);
#35664=VERTEX_POINT('',#141544);
#35665=VERTEX_POINT('',#141556);
#35666=VERTEX_POINT('',#141562);
#35667=VERTEX_POINT('',#141564);
#35668=VERTEX_POINT('',#141566);
#35669=VERTEX_POINT('',#141568);
#35670=VERTEX_POINT('',#141573);
#35671=VERTEX_POINT('',#141576);
#35672=VERTEX_POINT('',#141593);
#35673=VERTEX_POINT('',#141595);
#35674=VERTEX_POINT('',#141597);
#35675=VERTEX_POINT('',#141599);
#35676=VERTEX_POINT('',#141601);
#35677=VERTEX_POINT('',#141604);
#35678=VERTEX_POINT('',#141606);
#35679=VERTEX_POINT('',#141608);
#35680=VERTEX_POINT('',#141610);
#35681=VERTEX_POINT('',#141612);
#35682=VERTEX_POINT('',#141618);
#35683=VERTEX_POINT('',#141620);
#35684=VERTEX_POINT('',#141624);
#35685=VERTEX_POINT('',#141629);
#35686=VERTEX_POINT('',#141635);
#35687=VERTEX_POINT('',#141639);
#35688=VERTEX_POINT('',#141640);
#35689=VERTEX_POINT('',#141642);
#35690=VERTEX_POINT('',#141644);
#35691=VERTEX_POINT('',#141677);
#35692=VERTEX_POINT('',#141678);
#35693=VERTEX_POINT('',#141683);
#35694=VERTEX_POINT('',#141684);
#35695=VERTEX_POINT('',#141697);
#35696=VERTEX_POINT('',#141698);
#35697=VERTEX_POINT('',#141703);
#35698=VERTEX_POINT('',#141705);
#35699=VERTEX_POINT('',#141712);
#35700=VERTEX_POINT('',#141714);
#35701=VERTEX_POINT('',#141716);
#35702=VERTEX_POINT('',#141718);
#35703=VERTEX_POINT('',#141722);
#35704=VERTEX_POINT('',#141724);
#35705=VERTEX_POINT('',#141729);
#35706=VERTEX_POINT('',#141731);
#35707=VERTEX_POINT('',#141744);
#35708=VERTEX_POINT('',#141749);
#35709=VERTEX_POINT('',#141750);
#35710=VERTEX_POINT('',#141755);
#35711=VERTEX_POINT('',#141757);
#35712=VERTEX_POINT('',#141762);
#35713=VERTEX_POINT('',#141777);
#35714=VERTEX_POINT('',#141779);
#35715=VERTEX_POINT('',#141788);
#35716=VERTEX_POINT('',#141820);
#35717=VERTEX_POINT('',#141824);
#35718=VERTEX_POINT('',#141828);
#35719=VERTEX_POINT('',#141830);
#35720=VERTEX_POINT('',#141834);
#35721=VERTEX_POINT('',#141836);
#35722=VERTEX_POINT('',#141838);
#35723=VERTEX_POINT('',#141840);
#35724=VERTEX_POINT('',#141842);
#35725=VERTEX_POINT('',#141844);
#35726=VERTEX_POINT('',#141848);
#35727=VERTEX_POINT('',#141860);
#35728=VERTEX_POINT('',#141864);
#35729=VERTEX_POINT('',#141876);
#35730=VERTEX_POINT('',#141880);
#35731=VERTEX_POINT('',#141892);
#35732=VERTEX_POINT('',#141898);
#35733=VERTEX_POINT('',#141900);
#35734=VERTEX_POINT('',#141902);
#35735=VERTEX_POINT('',#141914);
#35736=VERTEX_POINT('',#141918);
#35737=VERTEX_POINT('',#141922);
#35738=VERTEX_POINT('',#141926);
#35739=VERTEX_POINT('',#141930);
#35740=VERTEX_POINT('',#141934);
#35741=VERTEX_POINT('',#141938);
#35742=VERTEX_POINT('',#141942);
#35743=VERTEX_POINT('',#141971);
#35744=VERTEX_POINT('',#141973);
#35745=VERTEX_POINT('',#141975);
#35746=VERTEX_POINT('',#141977);
#35747=VERTEX_POINT('',#141979);
#35748=VERTEX_POINT('',#141981);
#35749=VERTEX_POINT('',#141988);
#35750=VERTEX_POINT('',#142013);
#35751=VERTEX_POINT('',#142027);
#35752=VERTEX_POINT('',#142032);
#35753=VERTEX_POINT('',#142033);
#35754=VERTEX_POINT('',#142035);
#35755=VERTEX_POINT('',#142037);
#35756=VERTEX_POINT('',#142055);
#35757=VERTEX_POINT('',#142056);
#35758=VERTEX_POINT('',#142061);
#35759=VERTEX_POINT('',#142062);
#35760=VERTEX_POINT('',#142067);
#35761=VERTEX_POINT('',#142068);
#35762=VERTEX_POINT('',#142073);
#35763=VERTEX_POINT('',#142074);
#35764=VERTEX_POINT('',#142093);
#35765=VERTEX_POINT('',#142094);
#35766=VERTEX_POINT('',#142099);
#35767=VERTEX_POINT('',#142100);
#35768=VERTEX_POINT('',#142102);
#35769=VERTEX_POINT('',#142104);
#35770=VERTEX_POINT('',#142122);
#35771=VERTEX_POINT('',#142123);
#35772=VERTEX_POINT('',#142128);
#35773=VERTEX_POINT('',#142129);
#35774=VERTEX_POINT('',#142134);
#35775=VERTEX_POINT('',#142144);
#35776=VERTEX_POINT('',#142146);
#35777=VERTEX_POINT('',#142150);
#35778=VERTEX_POINT('',#142154);
#35779=VERTEX_POINT('',#142158);
#35780=VERTEX_POINT('',#142162);
#35781=VERTEX_POINT('',#142166);
#35782=VERTEX_POINT('',#142171);
#35783=VERTEX_POINT('',#142172);
#35784=VERTEX_POINT('',#142174);
#35785=VERTEX_POINT('',#142176);
#35786=VERTEX_POINT('',#142188);
#35787=VERTEX_POINT('',#142189);
#35788=VERTEX_POINT('',#142194);
#35789=VERTEX_POINT('',#142195);
#35790=VERTEX_POINT('',#142200);
#35791=VERTEX_POINT('',#142201);
#35792=VERTEX_POINT('',#142220);
#35793=VERTEX_POINT('',#142221);
#35794=VERTEX_POINT('',#142226);
#35795=VERTEX_POINT('',#142227);
#35796=VERTEX_POINT('',#142232);
#35797=VERTEX_POINT('',#142233);
#35798=VERTEX_POINT('',#142252);
#35799=VERTEX_POINT('',#142253);
#35800=VERTEX_POINT('',#142258);
#35801=VERTEX_POINT('',#142259);
#35802=VERTEX_POINT('',#142272);
#35803=VERTEX_POINT('',#142273);
#35804=VERTEX_POINT('',#142278);
#35805=VERTEX_POINT('',#142279);
#35806=VERTEX_POINT('',#142295);
#35807=VERTEX_POINT('',#142297);
#35808=VERTEX_POINT('',#142301);
#35809=VERTEX_POINT('',#142305);
#35810=VERTEX_POINT('',#142309);
#35811=VERTEX_POINT('',#142313);
#35812=VERTEX_POINT('',#142317);
#35813=VERTEX_POINT('',#142322);
#35814=VERTEX_POINT('',#142323);
#35815=VERTEX_POINT('',#142325);
#35816=VERTEX_POINT('',#142327);
#35817=VERTEX_POINT('',#142339);
#35818=VERTEX_POINT('',#142340);
#35819=VERTEX_POINT('',#142345);
#35820=VERTEX_POINT('',#142346);
#35821=VERTEX_POINT('',#142359);
#35822=VERTEX_POINT('',#142360);
#35823=VERTEX_POINT('',#142365);
#35824=VERTEX_POINT('',#142366);
#35825=VERTEX_POINT('',#142371);
#35826=VERTEX_POINT('',#142372);
#35827=VERTEX_POINT('',#142377);
#35828=VERTEX_POINT('',#142378);
#35829=VERTEX_POINT('',#142397);
#35830=VERTEX_POINT('',#142398);
#35831=VERTEX_POINT('',#142403);
#35832=VERTEX_POINT('',#142404);
#35833=VERTEX_POINT('',#142409);
#35834=VERTEX_POINT('',#142410);
#35835=VERTEX_POINT('',#142426);
#35836=VERTEX_POINT('',#142428);
#35837=VERTEX_POINT('',#142432);
#35838=VERTEX_POINT('',#142436);
#35839=VERTEX_POINT('',#142438);
#35840=VERTEX_POINT('',#142440);
#35841=VERTEX_POINT('',#142444);
#35842=VERTEX_POINT('',#142446);
#35843=VERTEX_POINT('',#142448);
#35844=VERTEX_POINT('',#142450);
#35845=VERTEX_POINT('',#142464);
#35846=VERTEX_POINT('',#142493);
#35847=VERTEX_POINT('',#142519);
#35848=VERTEX_POINT('',#142521);
#35849=VERTEX_POINT('',#142525);
#35850=VERTEX_POINT('',#142529);
#35851=VERTEX_POINT('',#142534);
#35852=VERTEX_POINT('',#142535);
#35853=VERTEX_POINT('',#142537);
#35854=VERTEX_POINT('',#142539);
#35855=VERTEX_POINT('',#142570);
#35856=VERTEX_POINT('',#142571);
#35857=VERTEX_POINT('',#142576);
#35858=VERTEX_POINT('',#142577);
#35859=VERTEX_POINT('',#142596);
#35860=VERTEX_POINT('',#142597);
#35861=VERTEX_POINT('',#142602);
#35862=VERTEX_POINT('',#142604);
#35863=VERTEX_POINT('',#142609);
#35864=VERTEX_POINT('',#142614);
#35865=VERTEX_POINT('',#142618);
#35866=VERTEX_POINT('',#142620);
#35867=VERTEX_POINT('',#142624);
#35868=VERTEX_POINT('',#142626);
#35869=VERTEX_POINT('',#142628);
#35870=VERTEX_POINT('',#142630);
#35871=VERTEX_POINT('',#142632);
#35872=VERTEX_POINT('',#142634);
#35873=VERTEX_POINT('',#142638);
#35874=VERTEX_POINT('',#142659);
#35875=VERTEX_POINT('',#142661);
#35876=VERTEX_POINT('',#142663);
#35877=VERTEX_POINT('',#142674);
#35878=VERTEX_POINT('',#142676);
#35879=VERTEX_POINT('',#142695);
#35880=VERTEX_POINT('',#142697);
#35881=VERTEX_POINT('',#142708);
#35882=VERTEX_POINT('',#142710);
#35883=VERTEX_POINT('',#142712);
#35884=VERTEX_POINT('',#142727);
#35885=VERTEX_POINT('',#142728);
#35886=VERTEX_POINT('',#142730);
#35887=VERTEX_POINT('',#142732);
#35888=VERTEX_POINT('',#142736);
#35889=VERTEX_POINT('',#142737);
#35890=VERTEX_POINT('',#142742);
#35891=VERTEX_POINT('',#142743);
#35892=VERTEX_POINT('',#142762);
#35893=VERTEX_POINT('',#142763);
#35894=VERTEX_POINT('',#142768);
#35895=VERTEX_POINT('',#142769);
#35896=VERTEX_POINT('',#142788);
#35897=VERTEX_POINT('',#142789);
#35898=VERTEX_POINT('',#142794);
#35899=VERTEX_POINT('',#142795);
#35900=VERTEX_POINT('',#142808);
#35901=VERTEX_POINT('',#142809);
#35902=VERTEX_POINT('',#142814);
#35903=VERTEX_POINT('',#142815);
#35904=VERTEX_POINT('',#142817);
#35905=VERTEX_POINT('',#142830);
#35906=VERTEX_POINT('',#142831);
#35907=VERTEX_POINT('',#142836);
#35908=VERTEX_POINT('',#142837);
#35909=VERTEX_POINT('',#142859);
#35910=VERTEX_POINT('',#142861);
#35911=VERTEX_POINT('',#142865);
#35912=VERTEX_POINT('',#142868);
#35913=VERTEX_POINT('',#142870);
#35914=VERTEX_POINT('',#142872);
#35915=VERTEX_POINT('',#142874);
#35916=VERTEX_POINT('',#142876);
#35917=VERTEX_POINT('',#142878);
#35918=VERTEX_POINT('',#142880);
#35919=VERTEX_POINT('',#142882);
#35920=VERTEX_POINT('',#142884);
#35921=VERTEX_POINT('',#142888);
#35922=VERTEX_POINT('',#142892);
#35923=VERTEX_POINT('',#142896);
#35924=VERTEX_POINT('',#142900);
#35925=VERTEX_POINT('',#142905);
#35926=VERTEX_POINT('',#142906);
#35927=VERTEX_POINT('',#142908);
#35928=VERTEX_POINT('',#142910);
#35929=VERTEX_POINT('',#142935);
#35930=VERTEX_POINT('',#142936);
#35931=VERTEX_POINT('',#142941);
#35932=VERTEX_POINT('',#142942);
#35933=VERTEX_POINT('',#142955);
#35934=VERTEX_POINT('',#142956);
#35935=VERTEX_POINT('',#142961);
#35936=VERTEX_POINT('',#142962);
#35937=VERTEX_POINT('',#142975);
#35938=VERTEX_POINT('',#142980);
#35939=VERTEX_POINT('',#142992);
#35940=VERTEX_POINT('',#142993);
#35941=VERTEX_POINT('',#142998);
#35942=VERTEX_POINT('',#142999);
#35943=VERTEX_POINT('',#143018);
#35944=VERTEX_POINT('',#143019);
#35945=VERTEX_POINT('',#143024);
#35946=VERTEX_POINT('',#143026);
#35947=VERTEX_POINT('',#143043);
#35948=VERTEX_POINT('',#143044);
#35949=VERTEX_POINT('',#143058);
#35950=VERTEX_POINT('',#143060);
#35951=VERTEX_POINT('',#143064);
#35952=VERTEX_POINT('',#143097);
#35953=VERTEX_POINT('',#143100);
#35954=VERTEX_POINT('',#143102);
#35955=VERTEX_POINT('',#143104);
#35956=VERTEX_POINT('',#143106);
#35957=VERTEX_POINT('',#143108);
#35958=VERTEX_POINT('',#143128);
#35959=VERTEX_POINT('',#143143);
#35960=VERTEX_POINT('',#143156);
#35961=VERTEX_POINT('',#143164);
#35962=VERTEX_POINT('',#143166);
#35963=VERTEX_POINT('',#143168);
#35964=VERTEX_POINT('',#143170);
#35965=VERTEX_POINT('',#143172);
#35966=VERTEX_POINT('',#143174);
#35967=VERTEX_POINT('',#143179);
#35968=VERTEX_POINT('',#143180);
#35969=VERTEX_POINT('',#143182);
#35970=VERTEX_POINT('',#143184);
#35971=VERTEX_POINT('',#143202);
#35972=VERTEX_POINT('',#143203);
#35973=VERTEX_POINT('',#143208);
#35974=VERTEX_POINT('',#143209);
#35975=VERTEX_POINT('',#143222);
#35976=VERTEX_POINT('',#143227);
#35977=VERTEX_POINT('',#143239);
#35978=VERTEX_POINT('',#143240);
#35979=VERTEX_POINT('',#143245);
#35980=VERTEX_POINT('',#143246);
#35981=VERTEX_POINT('',#143259);
#35982=VERTEX_POINT('',#143260);
#35983=VERTEX_POINT('',#143265);
#35984=VERTEX_POINT('',#143266);
#35985=VERTEX_POINT('',#143282);
#35986=VERTEX_POINT('',#143284);
#35987=VERTEX_POINT('',#143288);
#35988=VERTEX_POINT('',#143292);
#35989=VERTEX_POINT('',#143296);
#35990=VERTEX_POINT('',#143300);
#35991=VERTEX_POINT('',#143302);
#35992=VERTEX_POINT('',#143304);
#35993=VERTEX_POINT('',#143306);
#35994=VERTEX_POINT('',#143308);
#35995=VERTEX_POINT('',#143310);
#35996=VERTEX_POINT('',#143312);
#35997=VERTEX_POINT('',#143319);
#35998=VERTEX_POINT('',#143332);
#35999=VERTEX_POINT('',#143347);
#36000=VERTEX_POINT('',#143354);
#36001=VERTEX_POINT('',#143356);
#36002=VERTEX_POINT('',#143361);
#36003=VERTEX_POINT('',#143365);
#36004=VERTEX_POINT('',#143371);
#36005=VERTEX_POINT('',#143377);
#36006=VERTEX_POINT('',#143378);
#36007=VERTEX_POINT('',#143380);
#36008=VERTEX_POINT('',#143382);
#36009=VERTEX_POINT('',#143386);
#36010=VERTEX_POINT('',#143388);
#36011=VERTEX_POINT('',#143390);
#36012=VERTEX_POINT('',#143392);
#36013=VERTEX_POINT('',#143394);
#36014=VERTEX_POINT('',#143396);
#36015=VERTEX_POINT('',#143400);
#36016=VERTEX_POINT('',#143402);
#36017=VERTEX_POINT('',#143409);
#36018=VERTEX_POINT('',#143413);
#36019=VERTEX_POINT('',#143415);
#36020=VERTEX_POINT('',#143419);
#36021=VERTEX_POINT('',#143421);
#36022=VERTEX_POINT('',#143425);
#36023=VERTEX_POINT('',#143427);
#36024=VERTEX_POINT('',#143431);
#36025=VERTEX_POINT('',#143433);
#36026=VERTEX_POINT('',#143437);
#36027=VERTEX_POINT('',#143439);
#36028=VERTEX_POINT('',#143443);
#36029=VERTEX_POINT('',#143445);
#36030=VERTEX_POINT('',#143448);
#36031=VERTEX_POINT('',#143452);
#36032=VERTEX_POINT('',#143456);
#36033=VERTEX_POINT('',#143458);
#36034=VERTEX_POINT('',#143460);
#36035=VERTEX_POINT('',#143462);
#36036=VERTEX_POINT('',#143464);
#36037=VERTEX_POINT('',#143466);
#36038=VERTEX_POINT('',#143468);
#36039=VERTEX_POINT('',#143470);
#36040=VERTEX_POINT('',#143474);
#36041=VERTEX_POINT('',#143478);
#36042=VERTEX_POINT('',#143484);
#36043=VERTEX_POINT('',#143486);
#36044=VERTEX_POINT('',#143490);
#36045=VERTEX_POINT('',#143491);
#36046=VERTEX_POINT('',#143493);
#36047=VERTEX_POINT('',#143495);
#36048=VERTEX_POINT('',#143499);
#36049=VERTEX_POINT('',#143501);
#36050=VERTEX_POINT('',#143505);
#36051=VERTEX_POINT('',#143509);
#36052=VERTEX_POINT('',#143511);
#36053=VERTEX_POINT('',#143515);
#36054=VERTEX_POINT('',#143517);
#36055=VERTEX_POINT('',#143521);
#36056=VERTEX_POINT('',#143522);
#36057=VERTEX_POINT('',#143524);
#36058=VERTEX_POINT('',#143526);
#36059=VERTEX_POINT('',#143533);
#36060=VERTEX_POINT('',#143535);
#36061=VERTEX_POINT('',#143539);
#36062=VERTEX_POINT('',#143541);
#36063=VERTEX_POINT('',#143545);
#36064=VERTEX_POINT('',#143546);
#36065=VERTEX_POINT('',#143548);
#36066=VERTEX_POINT('',#143550);
#36067=VERTEX_POINT('',#143554);
#36068=VERTEX_POINT('',#143555);
#36069=VERTEX_POINT('',#143574);
#36070=VERTEX_POINT('',#143576);
#36071=VERTEX_POINT('',#143597);
#36072=VERTEX_POINT('',#143599);
#36073=VERTEX_POINT('',#143620);
#36074=VERTEX_POINT('',#143622);
#36075=VERTEX_POINT('',#143626);
#36076=VERTEX_POINT('',#143627);
#36077=VERTEX_POINT('',#143630);
#36078=VERTEX_POINT('',#143635);
#36079=VERTEX_POINT('',#143637);
#36080=VERTEX_POINT('',#143641);
#36081=VERTEX_POINT('',#143642);
#36082=VERTEX_POINT('',#143645);
#36083=VERTEX_POINT('',#143657);
#36084=VERTEX_POINT('',#143658);
#36085=VERTEX_POINT('',#143660);
#36086=VERTEX_POINT('',#143662);
#36087=VERTEX_POINT('',#143664);
#36088=VERTEX_POINT('',#143666);
#36089=VERTEX_POINT('',#143670);
#36090=VERTEX_POINT('',#143671);
#36091=VERTEX_POINT('',#143673);
#36092=VERTEX_POINT('',#143675);
#36093=VERTEX_POINT('',#143677);
#36094=VERTEX_POINT('',#143679);
#36095=VERTEX_POINT('',#143683);
#36096=VERTEX_POINT('',#143685);
#36097=VERTEX_POINT('',#143689);
#36098=VERTEX_POINT('',#143691);
#36099=VERTEX_POINT('',#143695);
#36100=VERTEX_POINT('',#143699);
#36101=VERTEX_POINT('',#143701);
#36102=VERTEX_POINT('',#143705);
#36103=VERTEX_POINT('',#143707);
#36104=VERTEX_POINT('',#143711);
#36105=VERTEX_POINT('',#143716);
#36106=VERTEX_POINT('',#143722);
#36107=VERTEX_POINT('',#143727);
#36108=VERTEX_POINT('',#143728);
#36109=VERTEX_POINT('',#143732);
#36110=VERTEX_POINT('',#143734);
#36111=VERTEX_POINT('',#143738);
#36112=VERTEX_POINT('',#143740);
#36113=VERTEX_POINT('',#143744);
#36114=VERTEX_POINT('',#143748);
#36115=VERTEX_POINT('',#143759);
#36116=VERTEX_POINT('',#143760);
#36117=VERTEX_POINT('',#143764);
#36118=VERTEX_POINT('',#143766);
#36119=VERTEX_POINT('',#143770);
#36120=VERTEX_POINT('',#143772);
#36121=VERTEX_POINT('',#143776);
#36122=VERTEX_POINT('',#143780);
#36123=VERTEX_POINT('',#143791);
#36124=VERTEX_POINT('',#143793);
#36125=VERTEX_POINT('',#143800);
#36126=VERTEX_POINT('',#143812);
#36127=VERTEX_POINT('',#143830);
#36128=VERTEX_POINT('',#143832);
#36129=VERTEX_POINT('',#143836);
#36130=VERTEX_POINT('',#143837);
#36131=VERTEX_POINT('',#143839);
#36132=VERTEX_POINT('',#143841);
#36133=VERTEX_POINT('',#143858);
#36134=VERTEX_POINT('',#143859);
#36135=VERTEX_POINT('',#143861);
#36136=VERTEX_POINT('',#143863);
#36137=VERTEX_POINT('',#143867);
#36138=VERTEX_POINT('',#143869);
#36139=VERTEX_POINT('',#143873);
#36140=VERTEX_POINT('',#143874);
#36141=VERTEX_POINT('',#143898);
#36142=VERTEX_POINT('',#143900);
#36143=VERTEX_POINT('',#143903);
#36144=VERTEX_POINT('',#143907);
#36145=VERTEX_POINT('',#143908);
#36146=VERTEX_POINT('',#143929);
#36147=VERTEX_POINT('',#143935);
#36148=VERTEX_POINT('',#143939);
#36149=VERTEX_POINT('',#143943);
#36150=VERTEX_POINT('',#143948);
#36151=VERTEX_POINT('',#143949);
#36152=VERTEX_POINT('',#143957);
#36153=VERTEX_POINT('',#143977);
#36154=VERTEX_POINT('',#143979);
#36155=VERTEX_POINT('',#143983);
#36156=VERTEX_POINT('',#143989);
#36157=VERTEX_POINT('',#143993);
#36158=VERTEX_POINT('',#143994);
#36159=VERTEX_POINT('',#144006);
#36160=VERTEX_POINT('',#144007);
#36161=VERTEX_POINT('',#144012);
#36162=VERTEX_POINT('',#144033);
#36163=VERTEX_POINT('',#144034);
#36164=VERTEX_POINT('',#144039);
#36165=VERTEX_POINT('',#144054);
#36166=VERTEX_POINT('',#144059);
#36167=VERTEX_POINT('',#144071);
#36168=VERTEX_POINT('',#144073);
#36169=VERTEX_POINT('',#144088);
#36170=VERTEX_POINT('',#144116);
#36171=VERTEX_POINT('',#144117);
#36172=VERTEX_POINT('',#144131);
#36173=VERTEX_POINT('',#144133);
#36174=VERTEX_POINT('',#144137);
#36175=VERTEX_POINT('',#144150);
#36176=VERTEX_POINT('',#144154);
#36177=VERTEX_POINT('',#144155);
#36178=VERTEX_POINT('',#144162);
#36179=VERTEX_POINT('',#144167);
#36180=VERTEX_POINT('',#144184);
#36181=VERTEX_POINT('',#144202);
#36182=VERTEX_POINT('',#144203);
#36183=VERTEX_POINT('',#144205);
#36184=VERTEX_POINT('',#144230);
#36185=VERTEX_POINT('',#144231);
#36186=VERTEX_POINT('',#144233);
#36187=VERTEX_POINT('',#144247);
#36188=VERTEX_POINT('',#144248);
#36189=VERTEX_POINT('',#144265);
#36190=VERTEX_POINT('',#144267);
#36191=VERTEX_POINT('',#144271);
#36192=VERTEX_POINT('',#144273);
#36193=VERTEX_POINT('',#144275);
#36194=VERTEX_POINT('',#144282);
#36195=VERTEX_POINT('',#144289);
#36196=VERTEX_POINT('',#144307);
#36197=VERTEX_POINT('',#144322);
#36198=VERTEX_POINT('',#144326);
#36199=VERTEX_POINT('',#144331);
#36200=VERTEX_POINT('',#144346);
#36201=VERTEX_POINT('',#144348);
#36202=VERTEX_POINT('',#144352);
#36203=VERTEX_POINT('',#144355);
#36204=VERTEX_POINT('',#144359);
#36205=VERTEX_POINT('',#144363);
#36206=VERTEX_POINT('',#144365);
#36207=VERTEX_POINT('',#144380);
#36208=VERTEX_POINT('',#144382);
#36209=VERTEX_POINT('',#144386);
#36210=VERTEX_POINT('',#144402);
#36211=VERTEX_POINT('',#144404);
#36212=VERTEX_POINT('',#144408);
#36213=VERTEX_POINT('',#144412);
#36214=VERTEX_POINT('',#144413);
#36215=VERTEX_POINT('',#144415);
#36216=VERTEX_POINT('',#144417);
#36217=VERTEX_POINT('',#144421);
#36218=VERTEX_POINT('',#144422);
#36219=VERTEX_POINT('',#144424);
#36220=VERTEX_POINT('',#144426);
#36221=VERTEX_POINT('',#144430);
#36222=VERTEX_POINT('',#144431);
#36223=VERTEX_POINT('',#144436);
#36224=VERTEX_POINT('',#144440);
#36225=VERTEX_POINT('',#144444);
#36226=VERTEX_POINT('',#144448);
#36227=VERTEX_POINT('',#144450);
#36228=VERTEX_POINT('',#144452);
#36229=VERTEX_POINT('',#144454);
#36230=VERTEX_POINT('',#144461);
#36231=VERTEX_POINT('',#144472);
#36232=VERTEX_POINT('',#144474);
#36233=VERTEX_POINT('',#144478);
#36234=VERTEX_POINT('',#144482);
#36235=VERTEX_POINT('',#144494);
#36236=VERTEX_POINT('',#144498);
#36237=VERTEX_POINT('',#144505);
#36238=VERTEX_POINT('',#144507);
#36239=VERTEX_POINT('',#144516);
#36240=VERTEX_POINT('',#144519);
#36241=VERTEX_POINT('',#144521);
#36242=VERTEX_POINT('',#144524);
#36243=VERTEX_POINT('',#144528);
#36244=VERTEX_POINT('',#144534);
#36245=VERTEX_POINT('',#144535);
#36246=VERTEX_POINT('',#144545);
#36247=VERTEX_POINT('',#144552);
#36248=VERTEX_POINT('',#144554);
#36249=VERTEX_POINT('',#144557);
#36250=VERTEX_POINT('',#144558);
#36251=VERTEX_POINT('',#144563);
#36252=VERTEX_POINT('',#144572);
#36253=VERTEX_POINT('',#144586);
#36254=VERTEX_POINT('',#144595);
#36255=VERTEX_POINT('',#144617);
#36256=VERTEX_POINT('',#144643);
#36257=VERTEX_POINT('',#144644);
#36258=VERTEX_POINT('',#144649);
#36259=VERTEX_POINT('',#144686);
#36260=VERTEX_POINT('',#144687);
#36261=VERTEX_POINT('',#144689);
#36262=VERTEX_POINT('',#144691);
#36263=VERTEX_POINT('',#144695);
#36264=VERTEX_POINT('',#144696);
#36265=VERTEX_POINT('',#144698);
#36266=VERTEX_POINT('',#144700);
#36267=VERTEX_POINT('',#144711);
#36268=VERTEX_POINT('',#144715);
#36269=VERTEX_POINT('',#144716);
#36270=VERTEX_POINT('',#144718);
#36271=VERTEX_POINT('',#144780);
#36272=VERTEX_POINT('',#144810);
#36273=VERTEX_POINT('',#144813);
#36274=VERTEX_POINT('',#144902);
#36275=VERTEX_POINT('',#144910);
#36276=VERTEX_POINT('',#144916);
#36277=VERTEX_POINT('',#144918);
#36278=VERTEX_POINT('',#144924);
#36279=VERTEX_POINT('',#144930);
#36280=VERTEX_POINT('',#144932);
#36281=VERTEX_POINT('',#144934);
#36282=VERTEX_POINT('',#144938);
#36283=VERTEX_POINT('',#144940);
#36284=VERTEX_POINT('',#144944);
#36285=VERTEX_POINT('',#144945);
#36286=VERTEX_POINT('',#144947);
#36287=VERTEX_POINT('',#144949);
#36288=VERTEX_POINT('',#144953);
#36289=VERTEX_POINT('',#144955);
#36290=VERTEX_POINT('',#144959);
#36291=VERTEX_POINT('',#144961);
#36292=VERTEX_POINT('',#144965);
#36293=VERTEX_POINT('',#144966);
#36294=VERTEX_POINT('',#144971);
#36295=VERTEX_POINT('',#144981);
#36296=VERTEX_POINT('',#144985);
#36297=VERTEX_POINT('',#144991);
#36298=VERTEX_POINT('',#144997);
#36299=VERTEX_POINT('',#144998);
#36300=VERTEX_POINT('',#145000);
#36301=VERTEX_POINT('',#145002);
#36302=VERTEX_POINT('',#145009);
#36303=VERTEX_POINT('',#145010);
#36304=VERTEX_POINT('',#145012);
#36305=VERTEX_POINT('',#145014);
#36306=VERTEX_POINT('',#145017);
#36307=VERTEX_POINT('',#145019);
#36308=VERTEX_POINT('',#145023);
#36309=VERTEX_POINT('',#145027);
#36310=VERTEX_POINT('',#145033);
#36311=VERTEX_POINT('',#145034);
#36312=VERTEX_POINT('',#145041);
#36313=VERTEX_POINT('',#145045);
#36314=VERTEX_POINT('',#145049);
#36315=VERTEX_POINT('',#145053);
#36316=VERTEX_POINT('',#145054);
#36317=VERTEX_POINT('',#145059);
#36318=VERTEX_POINT('',#145061);
#36319=VERTEX_POINT('',#145066);
#36320=VERTEX_POINT('',#145070);
#36321=VERTEX_POINT('',#145071);
#36322=VERTEX_POINT('',#145079);
#36323=VERTEX_POINT('',#145081);
#36324=VERTEX_POINT('',#145088);
#36325=VERTEX_POINT('',#145089);
#36326=VERTEX_POINT('',#145094);
#36327=VERTEX_POINT('',#145100);
#36328=VERTEX_POINT('',#145102);
#36329=VERTEX_POINT('',#145106);
#36330=VERTEX_POINT('',#145108);
#36331=VERTEX_POINT('',#145111);
#36332=VERTEX_POINT('',#145113);
#36333=VERTEX_POINT('',#145115);
#36334=VERTEX_POINT('',#145119);
#36335=VERTEX_POINT('',#145121);
#36336=VERTEX_POINT('',#145124);
#36337=VERTEX_POINT('',#145126);
#36338=VERTEX_POINT('',#145128);
#36339=VERTEX_POINT('',#145130);
#36340=VERTEX_POINT('',#145133);
#36341=VERTEX_POINT('',#145144);
#36342=VERTEX_POINT('',#145146);
#36343=VERTEX_POINT('',#145148);
#36344=VERTEX_POINT('',#145152);
#36345=VERTEX_POINT('',#145153);
#36346=VERTEX_POINT('',#145155);
#36347=VERTEX_POINT('',#145157);
#36348=VERTEX_POINT('',#145161);
#36349=VERTEX_POINT('',#145162);
#36350=VERTEX_POINT('',#145164);
#36351=VERTEX_POINT('',#145166);
#36352=VERTEX_POINT('',#145193);
#36353=VERTEX_POINT('',#145195);
#36354=VERTEX_POINT('',#145201);
#36355=VERTEX_POINT('',#145266);
#36356=VERTEX_POINT('',#145318);
#36357=VERTEX_POINT('',#145330);
#36358=VERTEX_POINT('',#145332);
#36359=VERTEX_POINT('',#145336);
#36360=VERTEX_POINT('',#145371);
#36361=VERTEX_POINT('',#145373);
#36362=VERTEX_POINT('',#145377);
#36363=VERTEX_POINT('',#145379);
#44160=EDGE_CURVE('',#35074,#35075,#18355,.T.);
#44161=EDGE_CURVE('',#35075,#35076,#27340,.T.);
#44162=EDGE_CURVE('',#35076,#35077,#18356,.T.);
#44163=EDGE_CURVE('',#35077,#35074,#27341,.T.);
#44164=EDGE_CURVE('',#35078,#35079,#18357,.T.);
#44165=EDGE_CURVE('',#35079,#35077,#18358,.T.);
#44166=EDGE_CURVE('',#35076,#35078,#18359,.T.);
#44167=EDGE_CURVE('',#35080,#35081,#18360,.T.);
#44168=EDGE_CURVE('',#35081,#35079,#18361,.T.);
#44169=EDGE_CURVE('',#35078,#35080,#18362,.T.);
#44170=EDGE_CURVE('',#35082,#35083,#18363,.T.);
#44171=EDGE_CURVE('',#35083,#35081,#18364,.T.);
#44172=EDGE_CURVE('',#35080,#35082,#18365,.T.);
#44173=EDGE_CURVE('',#35084,#35085,#18366,.T.);
#44174=EDGE_CURVE('',#35085,#35083,#18367,.T.);
#44175=EDGE_CURVE('',#35082,#35084,#18368,.T.);
#44176=EDGE_CURVE('',#35086,#35087,#18369,.T.);
#44177=EDGE_CURVE('',#35087,#35085,#18370,.T.);
#44178=EDGE_CURVE('',#35084,#35086,#18371,.T.);
#44179=EDGE_CURVE('',#35088,#35089,#18372,.T.);
#44180=EDGE_CURVE('',#35089,#35087,#18373,.T.);
#44181=EDGE_CURVE('',#35086,#35088,#18374,.T.);
#44182=EDGE_CURVE('',#35090,#35091,#18375,.T.);
#44183=EDGE_CURVE('',#35091,#35089,#18376,.T.);
#44184=EDGE_CURVE('',#35088,#35090,#18377,.T.);
#44185=EDGE_CURVE('',#35092,#35093,#18378,.T.);
#44186=EDGE_CURVE('',#35093,#35091,#27342,.T.);
#44187=EDGE_CURVE('',#35090,#35092,#27343,.T.);
#44188=EDGE_CURVE('',#35074,#35093,#18379,.T.);
#44189=EDGE_CURVE('',#35092,#35075,#18380,.T.);
#44190=EDGE_CURVE('',#35094,#35089,#27344,.T.);
#44191=EDGE_CURVE('',#35094,#35095,#18381,.T.);
#44192=EDGE_CURVE('',#35096,#35095,#27345,.T.);
#44193=EDGE_CURVE('',#35096,#35097,#18382,.T.);
#44194=EDGE_CURVE('',#35098,#35097,#27346,.T.);
#44195=EDGE_CURVE('',#35099,#35098,#23610,.T.);
#44196=EDGE_CURVE('',#35100,#35099,#27347,.T.);
#44197=EDGE_CURVE('',#35101,#35100,#18383,.T.);
#44198=EDGE_CURVE('',#35087,#35101,#27348,.T.);
#44199=EDGE_CURVE('',#35091,#35102,#27349,.T.);
#44200=EDGE_CURVE('',#35102,#35094,#18384,.T.);
#44201=EDGE_CURVE('',#35103,#35093,#27350,.T.);
#44202=EDGE_CURVE('',#35102,#35103,#27351,.T.);
#44203=EDGE_CURVE('',#35074,#35104,#27352,.T.);
#44204=EDGE_CURVE('',#35104,#35103,#18385,.T.);
#44205=EDGE_CURVE('',#35105,#35077,#27353,.T.);
#44206=EDGE_CURVE('',#35104,#35105,#27354,.T.);
#44207=EDGE_CURVE('',#35106,#35107,#18386,.T.);
#44208=EDGE_CURVE('',#35107,#35108,#27355,.T.);
#44209=EDGE_CURVE('',#35108,#35109,#18387,.T.);
#44210=EDGE_CURVE('',#35109,#35106,#27356,.T.);
#44211=EDGE_CURVE('',#35110,#35111,#18388,.T.);
#44212=EDGE_CURVE('',#35111,#35109,#18389,.T.);
#44213=EDGE_CURVE('',#35108,#35110,#18390,.T.);
#44214=EDGE_CURVE('',#35112,#35113,#18391,.T.);
#44215=EDGE_CURVE('',#35113,#35111,#18392,.T.);
#44216=EDGE_CURVE('',#35110,#35112,#18393,.T.);
#44217=EDGE_CURVE('',#35114,#35115,#18394,.T.);
#44218=EDGE_CURVE('',#35115,#35113,#18395,.T.);
#44219=EDGE_CURVE('',#35112,#35114,#18396,.T.);
#44220=EDGE_CURVE('',#35116,#35117,#18397,.T.);
#44221=EDGE_CURVE('',#35117,#35115,#27357,.T.);
#44222=EDGE_CURVE('',#35114,#35116,#27358,.T.);
#44223=EDGE_CURVE('',#35118,#35119,#18398,.T.);
#44224=EDGE_CURVE('',#35119,#35117,#18399,.T.);
#44225=EDGE_CURVE('',#35116,#35118,#18400,.T.);
#44226=EDGE_CURVE('',#35120,#35121,#18401,.T.);
#44227=EDGE_CURVE('',#35121,#35119,#27359,.T.);
#44228=EDGE_CURVE('',#35118,#35120,#27360,.T.);
#44229=EDGE_CURVE('',#35122,#35123,#18402,.T.);
#44230=EDGE_CURVE('',#35123,#35121,#18403,.T.);
#44231=EDGE_CURVE('',#35120,#35122,#18404,.T.);
#44232=EDGE_CURVE('',#35124,#35125,#18405,.T.);
#44233=EDGE_CURVE('',#35125,#35123,#27361,.T.);
#44234=EDGE_CURVE('',#35122,#35124,#27362,.T.);
#44235=EDGE_CURVE('',#35126,#35127,#18406,.T.);
#44236=EDGE_CURVE('',#35127,#35125,#18407,.T.);
#44237=EDGE_CURVE('',#35124,#35126,#18408,.T.);
#44238=EDGE_CURVE('',#35128,#35129,#18409,.T.);
#44239=EDGE_CURVE('',#35129,#35127,#18410,.T.);
#44240=EDGE_CURVE('',#35126,#35128,#18411,.T.);
#44241=EDGE_CURVE('',#35130,#35131,#18412,.T.);
#44242=EDGE_CURVE('',#35131,#35129,#18413,.T.);
#44243=EDGE_CURVE('',#35128,#35130,#18414,.T.);
#44244=EDGE_CURVE('',#35132,#35133,#18415,.T.);
#44245=EDGE_CURVE('',#35133,#35134,#18416,.T.);
#44246=EDGE_CURVE('',#35134,#35131,#18417,.T.);
#44247=EDGE_CURVE('',#35130,#35132,#18418,.T.);
#44248=EDGE_CURVE('',#35106,#35133,#18419,.T.);
#44249=EDGE_CURVE('',#35132,#35107,#18420,.T.);
#44250=EDGE_CURVE('',#35135,#35125,#27363,.T.);
#44251=EDGE_CURVE('',#35135,#35136,#27364,.T.);
#44252=EDGE_CURVE('',#35123,#35136,#27365,.T.);
#44253=EDGE_CURVE('',#35127,#35137,#27366,.T.);
#44254=EDGE_CURVE('',#35135,#35137,#18421,.F.);
#44255=EDGE_CURVE('',#35138,#35129,#27367,.T.);
#44256=EDGE_CURVE('',#35138,#35137,#18422,.T.);
#44257=EDGE_CURVE('',#35131,#35139,#27368,.T.);
#44258=EDGE_CURVE('',#35139,#35138,#18423,.T.);
#44259=EDGE_CURVE('',#35140,#35140,#18424,.F.);
#44260=EDGE_CURVE('',#35140,#35134,#27369,.T.);
#44261=EDGE_CURVE('',#35141,#35133,#27370,.T.);
#44262=EDGE_CURVE('',#35141,#35142,#18425,.T.);
#44263=EDGE_CURVE('',#35143,#35142,#27371,.T.);
#44264=EDGE_CURVE('',#35144,#35143,#18426,.T.);
#44265=EDGE_CURVE('',#35145,#35144,#27372,.T.);
#44266=EDGE_CURVE('',#35145,#35146,#18427,.T.);
#44267=EDGE_CURVE('',#35147,#35146,#27373,.T.);
#44268=EDGE_CURVE('',#35148,#35147,#18428,.T.);
#44269=EDGE_CURVE('',#35149,#35148,#27374,.T.);
#44270=EDGE_CURVE('',#35149,#35139,#18429,.T.);
#44271=EDGE_CURVE('',#35106,#35150,#27375,.T.);
#44272=EDGE_CURVE('',#35150,#35141,#18430,.T.);
#44273=EDGE_CURVE('',#35151,#35109,#27376,.T.);
#44274=EDGE_CURVE('',#35151,#35150,#27377,.T.);
#44275=EDGE_CURVE('',#35152,#35153,#18431,.T.);
#44276=EDGE_CURVE('',#35153,#35154,#18432,.T.);
#44277=EDGE_CURVE('',#35154,#35155,#18433,.T.);
#44278=EDGE_CURVE('',#35155,#35152,#18434,.T.);
#44279=EDGE_CURVE('',#35156,#35157,#18435,.T.);
#44280=EDGE_CURVE('',#35157,#35155,#18436,.T.);
#44281=EDGE_CURVE('',#35154,#35156,#18437,.T.);
#44282=EDGE_CURVE('',#35158,#35159,#18438,.T.);
#44283=EDGE_CURVE('',#35159,#35157,#27378,.T.);
#44284=EDGE_CURVE('',#35156,#35158,#27379,.T.);
#44285=EDGE_CURVE('',#35160,#35161,#18439,.T.);
#44286=EDGE_CURVE('',#35161,#35159,#18440,.T.);
#44287=EDGE_CURVE('',#35158,#35160,#18441,.T.);
#44288=EDGE_CURVE('',#35162,#35163,#18442,.T.);
#44289=EDGE_CURVE('',#35163,#35161,#27380,.T.);
#44290=EDGE_CURVE('',#35160,#35162,#27381,.T.);
#44291=EDGE_CURVE('',#35164,#35165,#18443,.T.);
#44292=EDGE_CURVE('',#35165,#35163,#18444,.T.);
#44293=EDGE_CURVE('',#35162,#35164,#18445,.T.);
#44294=EDGE_CURVE('',#35166,#35167,#18446,.T.);
#44295=EDGE_CURVE('',#35167,#35165,#18447,.T.);
#44296=EDGE_CURVE('',#35164,#35166,#18448,.T.);
#44297=EDGE_CURVE('',#35168,#35169,#18449,.T.);
#44298=EDGE_CURVE('',#35169,#35167,#18450,.T.);
#44299=EDGE_CURVE('',#35166,#35168,#18451,.T.);
#44300=EDGE_CURVE('',#35170,#35171,#18452,.T.);
#44301=EDGE_CURVE('',#35171,#35169,#27382,.T.);
#44302=EDGE_CURVE('',#35168,#35170,#27383,.T.);
#44303=EDGE_CURVE('',#35172,#35143,#18453,.T.);
#44304=EDGE_CURVE('',#35143,#35171,#18454,.T.);
#44305=EDGE_CURVE('',#35170,#35172,#18455,.T.);
#44306=EDGE_CURVE('',#35173,#35144,#18456,.T.);
#44307=EDGE_CURVE('',#35172,#35173,#18457,.T.);
#44308=EDGE_CURVE('',#35152,#35144,#18458,.T.);
#44309=EDGE_CURVE('',#35173,#35153,#18459,.T.);
#44310=EDGE_CURVE('',#35169,#35174,#27384,.T.);
#44311=EDGE_CURVE('',#35174,#35175,#18460,.T.);
#44312=EDGE_CURVE('',#35175,#35176,#27385,.T.);
#44313=EDGE_CURVE('',#35176,#35177,#18461,.T.);
#44314=EDGE_CURVE('',#35177,#35167,#27386,.T.);
#44315=EDGE_CURVE('',#35178,#35171,#27387,.T.);
#44316=EDGE_CURVE('',#35178,#35174,#27388,.T.);
#44317=EDGE_CURVE('',#35142,#35178,#18462,.T.);
#44318=EDGE_CURVE('',#35152,#35179,#27389,.T.);
#44319=EDGE_CURVE('',#35179,#35145,#18463,.T.);
#44320=EDGE_CURVE('',#35180,#35155,#27390,.T.);
#44321=EDGE_CURVE('',#35180,#35179,#18464,.T.);
#44322=EDGE_CURVE('',#35181,#35182,#18465,.T.);
#44323=EDGE_CURVE('',#35182,#35183,#27391,.T.);
#44324=EDGE_CURVE('',#35183,#35184,#18466,.T.);
#44325=EDGE_CURVE('',#35184,#35181,#27392,.T.);
#44326=EDGE_CURVE('',#35185,#35186,#18467,.T.);
#44327=EDGE_CURVE('',#35186,#35184,#18468,.T.);
#44328=EDGE_CURVE('',#35183,#35185,#18469,.T.);
#44329=EDGE_CURVE('',#35187,#35188,#18470,.T.);
#44330=EDGE_CURVE('',#35188,#35186,#18471,.T.);
#44331=EDGE_CURVE('',#35185,#35187,#18472,.T.);
#44332=EDGE_CURVE('',#35189,#35190,#18473,.T.);
#44333=EDGE_CURVE('',#35190,#35188,#18474,.T.);
#44334=EDGE_CURVE('',#35187,#35189,#18475,.T.);
#44335=EDGE_CURVE('',#35191,#35192,#18476,.T.);
#44336=EDGE_CURVE('',#35192,#35190,#18477,.T.);
#44337=EDGE_CURVE('',#35189,#35191,#18478,.T.);
#44338=EDGE_CURVE('',#35193,#35194,#18479,.T.);
#44339=EDGE_CURVE('',#35194,#35192,#18480,.T.);
#44340=EDGE_CURVE('',#35191,#35193,#18481,.T.);
#44341=EDGE_CURVE('',#35195,#35196,#18482,.T.);
#44342=EDGE_CURVE('',#35196,#35194,#27393,.T.);
#44343=EDGE_CURVE('',#35193,#35195,#27394,.T.);
#44344=EDGE_CURVE('',#35197,#35198,#18483,.T.);
#44345=EDGE_CURVE('',#35198,#35196,#18484,.T.);
#44346=EDGE_CURVE('',#35195,#35197,#18485,.T.);
#44347=EDGE_CURVE('',#35199,#35200,#18486,.T.);
#44348=EDGE_CURVE('',#35200,#35198,#18487,.T.);
#44349=EDGE_CURVE('',#35197,#35199,#18488,.T.);
#44350=EDGE_CURVE('',#35201,#35202,#18489,.T.);
#44351=EDGE_CURVE('',#35202,#35200,#27395,.T.);
#44352=EDGE_CURVE('',#35199,#35201,#27396,.T.);
#44353=EDGE_CURVE('',#35181,#35202,#18490,.T.);
#44354=EDGE_CURVE('',#35201,#35182,#18491,.T.);
#44355=EDGE_CURVE('',#35203,#35196,#27397,.T.);
#44356=EDGE_CURVE('',#35204,#35203,#27398,.T.);
#44357=EDGE_CURVE('',#35204,#35205,#27399,.T.);
#44358=EDGE_CURVE('',#35205,#35206,#27400,.F.);
#44359=EDGE_CURVE('',#35206,#35194,#27401,.T.);
#44360=EDGE_CURVE('',#35207,#35198,#27402,.T.);
#44361=EDGE_CURVE('',#35203,#35207,#18492,.T.);
#44362=EDGE_CURVE('',#35200,#35208,#27403,.T.);
#44363=EDGE_CURVE('',#35208,#35207,#18493,.T.);
#44364=EDGE_CURVE('',#35209,#35202,#27404,.T.);
#44365=EDGE_CURVE('',#35208,#35209,#27405,.T.);
#44366=EDGE_CURVE('',#35181,#35210,#27406,.T.);
#44367=EDGE_CURVE('',#35210,#35209,#18494,.T.);
#44368=EDGE_CURVE('',#35211,#35184,#27407,.T.);
#44369=EDGE_CURVE('',#35211,#35212,#27408,.T.);
#44370=EDGE_CURVE('',#35213,#35212,#27409,.T.);
#44371=EDGE_CURVE('',#35210,#35213,#27410,.T.);
#44372=EDGE_CURVE('',#35214,#35215,#18495,.T.);
#44373=EDGE_CURVE('',#35215,#35216,#18496,.T.);
#44374=EDGE_CURVE('',#35216,#35217,#18497,.T.);
#44375=EDGE_CURVE('',#35217,#35214,#18498,.T.);
#44376=EDGE_CURVE('',#35218,#35219,#18499,.T.);
#44377=EDGE_CURVE('',#35219,#35217,#18500,.T.);
#44378=EDGE_CURVE('',#35216,#35218,#18501,.T.);
#44379=EDGE_CURVE('',#35220,#35221,#18502,.T.);
#44380=EDGE_CURVE('',#35221,#35219,#18503,.T.);
#44381=EDGE_CURVE('',#35218,#35220,#18504,.T.);
#44382=EDGE_CURVE('',#35222,#35223,#18505,.T.);
#44383=EDGE_CURVE('',#35223,#35221,#18506,.T.);
#44384=EDGE_CURVE('',#35220,#35222,#18507,.T.);
#44385=EDGE_CURVE('',#35224,#35225,#18508,.T.);
#44386=EDGE_CURVE('',#35225,#35223,#18509,.T.);
#44387=EDGE_CURVE('',#35222,#35224,#18510,.T.);
#44388=EDGE_CURVE('',#35226,#35227,#18511,.T.);
#44389=EDGE_CURVE('',#35227,#35225,#27411,.T.);
#44390=EDGE_CURVE('',#35224,#35226,#27412,.T.);
#44391=EDGE_CURVE('',#35228,#35229,#18512,.T.);
#44392=EDGE_CURVE('',#35229,#35227,#18513,.T.);
#44393=EDGE_CURVE('',#35226,#35228,#18514,.T.);
#44394=EDGE_CURVE('',#35230,#35231,#18515,.T.);
#44395=EDGE_CURVE('',#35231,#35229,#27413,.T.);
#44396=EDGE_CURVE('',#35228,#35230,#27414,.T.);
#44397=EDGE_CURVE('',#35232,#35233,#18516,.T.);
#44398=EDGE_CURVE('',#35233,#35231,#18517,.T.);
#44399=EDGE_CURVE('',#35230,#35232,#18518,.T.);
#44400=EDGE_CURVE('',#35234,#35235,#18519,.T.);
#44401=EDGE_CURVE('',#35235,#35233,#27415,.T.);
#44402=EDGE_CURVE('',#35232,#35234,#27416,.T.);
#44403=EDGE_CURVE('',#35236,#35237,#18520,.T.);
#44404=EDGE_CURVE('',#35237,#35235,#18521,.T.);
#44405=EDGE_CURVE('',#35234,#35236,#18522,.T.);
#44406=EDGE_CURVE('',#35238,#35239,#18523,.T.);
#44407=EDGE_CURVE('',#35239,#35237,#18524,.T.);
#44408=EDGE_CURVE('',#35236,#35238,#18525,.T.);
#44409=EDGE_CURVE('',#35240,#35241,#18526,.T.);
#44410=EDGE_CURVE('',#35241,#35239,#18527,.T.);
#44411=EDGE_CURVE('',#35238,#35240,#18528,.T.);
#44412=EDGE_CURVE('',#35214,#35241,#27417,.T.);
#44413=EDGE_CURVE('',#35240,#35215,#27418,.T.);
#44414=EDGE_CURVE('',#35233,#35242,#27419,.T.);
#44415=EDGE_CURVE('',#35242,#35243,#18529,.T.);
#44416=EDGE_CURVE('',#35243,#35231,#27420,.T.);
#44417=EDGE_CURVE('',#35244,#35235,#27421,.T.);
#44418=EDGE_CURVE('',#35242,#35244,#27422,.T.);
#44419=EDGE_CURVE('',#35237,#35245,#27423,.T.);
#44420=EDGE_CURVE('',#35245,#35244,#18530,.T.);
#44421=EDGE_CURVE('',#35246,#35239,#27424,.T.);
#44422=EDGE_CURVE('',#35245,#35246,#18531,.T.);
#44423=EDGE_CURVE('',#35241,#35247,#27425,.T.);
#44424=EDGE_CURVE('',#35247,#35246,#18532,.T.);
#44425=EDGE_CURVE('',#35248,#35214,#27426,.T.);
#44426=EDGE_CURVE('',#35248,#35247,#27427,.T.);
#44427=EDGE_CURVE('',#35249,#35217,#27428,.T.);
#44428=EDGE_CURVE('',#35249,#35248,#18533,.T.);
#44429=EDGE_CURVE('',#35250,#35251,#18534,.T.);
#44430=EDGE_CURVE('',#35251,#35252,#18535,.T.);
#44431=EDGE_CURVE('',#35252,#35253,#18536,.T.);
#44432=EDGE_CURVE('',#35253,#35250,#18537,.T.);
#44433=EDGE_CURVE('',#35254,#35255,#18538,.T.);
#44434=EDGE_CURVE('',#35255,#35253,#18539,.T.);
#44435=EDGE_CURVE('',#35252,#35254,#18540,.T.);
#44436=EDGE_CURVE('',#35256,#35257,#18541,.T.);
#44437=EDGE_CURVE('',#35257,#35255,#18542,.T.);
#44438=EDGE_CURVE('',#35254,#35256,#18543,.T.);
#44439=EDGE_CURVE('',#35258,#35259,#18544,.T.);
#44440=EDGE_CURVE('',#35259,#35257,#18545,.T.);
#44441=EDGE_CURVE('',#35256,#35258,#18546,.T.);
#44442=EDGE_CURVE('',#35260,#35261,#18547,.T.);
#44443=EDGE_CURVE('',#35261,#35259,#18548,.T.);
#44444=EDGE_CURVE('',#35258,#35260,#18549,.T.);
#44445=EDGE_CURVE('',#35262,#35263,#18550,.T.);
#44446=EDGE_CURVE('',#35263,#35261,#18551,.T.);
#44447=EDGE_CURVE('',#35260,#35262,#18552,.T.);
#44448=EDGE_CURVE('',#35264,#35265,#18553,.T.);
#44449=EDGE_CURVE('',#35265,#35263,#18554,.T.);
#44450=EDGE_CURVE('',#35262,#35264,#18555,.T.);
#44451=EDGE_CURVE('',#35266,#35267,#18556,.T.);
#44452=EDGE_CURVE('',#35267,#35265,#27429,.T.);
#44453=EDGE_CURVE('',#35264,#35266,#27430,.T.);
#44454=EDGE_CURVE('',#35250,#35267,#18557,.T.);
#44455=EDGE_CURVE('',#35266,#35251,#18558,.T.);
#44456=EDGE_CURVE('',#35268,#35263,#27431,.T.);
#44457=EDGE_CURVE('',#35268,#35269,#18559,.T.);
#44458=EDGE_CURVE('',#35261,#35269,#27432,.T.);
#44459=EDGE_CURVE('',#35265,#35270,#27433,.T.);
#44460=EDGE_CURVE('',#35270,#35268,#18560,.T.);
#44461=EDGE_CURVE('',#35271,#35267,#27434,.T.);
#44462=EDGE_CURVE('',#35270,#35271,#27435,.T.);
#44463=EDGE_CURVE('',#35250,#35272,#27436,.T.);
#44464=EDGE_CURVE('',#35271,#35272,#18561,.F.);
#44465=EDGE_CURVE('',#35273,#35253,#27437,.T.);
#44466=EDGE_CURVE('',#35272,#35273,#18562,.T.);
#44467=EDGE_CURVE('',#35274,#35275,#18563,.T.);
#44468=EDGE_CURVE('',#35275,#35276,#18564,.T.);
#44469=EDGE_CURVE('',#35276,#35277,#18565,.T.);
#44470=EDGE_CURVE('',#35277,#35274,#18566,.T.);
#44471=EDGE_CURVE('',#35278,#35279,#18567,.T.);
#44472=EDGE_CURVE('',#35279,#35277,#18568,.T.);
#44473=EDGE_CURVE('',#35276,#35278,#18569,.T.);
#44474=EDGE_CURVE('',#35280,#35281,#18570,.T.);
#44475=EDGE_CURVE('',#35281,#35279,#18571,.T.);
#44476=EDGE_CURVE('',#35278,#35280,#18572,.T.);
#44477=EDGE_CURVE('',#35282,#35283,#18573,.T.);
#44478=EDGE_CURVE('',#35283,#35281,#18574,.T.);
#44479=EDGE_CURVE('',#35280,#35282,#18575,.T.);
#44480=EDGE_CURVE('',#35284,#35285,#18576,.T.);
#44481=EDGE_CURVE('',#35285,#35283,#18577,.T.);
#44482=EDGE_CURVE('',#35282,#35284,#18578,.T.);
#44483=EDGE_CURVE('',#35286,#35287,#18579,.T.);
#44484=EDGE_CURVE('',#35287,#35285,#18580,.T.);
#44485=EDGE_CURVE('',#35284,#35286,#18581,.T.);
#44486=EDGE_CURVE('',#35288,#35289,#18582,.T.);
#44487=EDGE_CURVE('',#35289,#35287,#27438,.T.);
#44488=EDGE_CURVE('',#35286,#35288,#27439,.T.);
#44489=EDGE_CURVE('',#35290,#35291,#18583,.T.);
#44490=EDGE_CURVE('',#35291,#35289,#18584,.T.);
#44491=EDGE_CURVE('',#35288,#35290,#18585,.T.);
#44492=EDGE_CURVE('',#35292,#35293,#18586,.T.);
#44493=EDGE_CURVE('',#35293,#35291,#27440,.T.);
#44494=EDGE_CURVE('',#35290,#35292,#27441,.T.);
#44495=EDGE_CURVE('',#35294,#35295,#18587,.T.);
#44496=EDGE_CURVE('',#35295,#35293,#18588,.T.);
#44497=EDGE_CURVE('',#35292,#35294,#18589,.T.);
#44498=EDGE_CURVE('',#35296,#35297,#18590,.T.);
#44499=EDGE_CURVE('',#35297,#35295,#27442,.T.);
#44500=EDGE_CURVE('',#35294,#35296,#27443,.T.);
#44501=EDGE_CURVE('',#35298,#35299,#18591,.T.);
#44502=EDGE_CURVE('',#35299,#35297,#18592,.T.);
#44503=EDGE_CURVE('',#35296,#35298,#18593,.T.);
#44504=EDGE_CURVE('',#35300,#35301,#18594,.T.);
#44505=EDGE_CURVE('',#35301,#35299,#18595,.T.);
#44506=EDGE_CURVE('',#35298,#35300,#18596,.T.);
#44507=EDGE_CURVE('',#35302,#35303,#18597,.T.);
#44508=EDGE_CURVE('',#35303,#35301,#18598,.T.);
#44509=EDGE_CURVE('',#35300,#35302,#18599,.T.);
#44510=EDGE_CURVE('',#35304,#35305,#18600,.T.);
#44511=EDGE_CURVE('',#35305,#35303,#18601,.T.);
#44512=EDGE_CURVE('',#35302,#35304,#18602,.T.);
#44513=EDGE_CURVE('',#35274,#35305,#18603,.T.);
#44514=EDGE_CURVE('',#35304,#35275,#18604,.T.);
#44515=EDGE_CURVE('',#35295,#35306,#27444,.T.);
#44516=EDGE_CURVE('',#35306,#35307,#18605,.T.);
#44517=EDGE_CURVE('',#35307,#35293,#27445,.T.);
#44518=EDGE_CURVE('',#35308,#35297,#27446,.T.);
#44519=EDGE_CURVE('',#35306,#35308,#27447,.T.);
#44520=EDGE_CURVE('',#35299,#35309,#27448,.T.);
#44521=EDGE_CURVE('',#35309,#35308,#18606,.T.);
#44522=EDGE_CURVE('',#35310,#35301,#27449,.T.);
#44523=EDGE_CURVE('',#35309,#35310,#18607,.T.);
#44524=EDGE_CURVE('',#35303,#35311,#27450,.T.);
#44525=EDGE_CURVE('',#35311,#35310,#18608,.T.);
#44526=EDGE_CURVE('',#35312,#35305,#27451,.T.);
#44527=EDGE_CURVE('',#35312,#35311,#18609,.F.);
#44528=EDGE_CURVE('',#35274,#35313,#27452,.T.);
#44529=EDGE_CURVE('',#35313,#35312,#18610,.T.);
#44530=EDGE_CURVE('',#35314,#35277,#27453,.T.);
#44531=EDGE_CURVE('',#35315,#35314,#18611,.T.);
#44532=EDGE_CURVE('',#35316,#35315,#27454,.T.);
#44533=EDGE_CURVE('',#35316,#35313,#18612,.T.);
#44534=EDGE_CURVE('',#35317,#35318,#18613,.T.);
#44535=EDGE_CURVE('',#35318,#35319,#18614,.T.);
#44536=EDGE_CURVE('',#35319,#35320,#18615,.T.);
#44537=EDGE_CURVE('',#35320,#35317,#18616,.T.);
#44538=EDGE_CURVE('',#35321,#35322,#18617,.T.);
#44539=EDGE_CURVE('',#35322,#35320,#18618,.T.);
#44540=EDGE_CURVE('',#35319,#35321,#18619,.T.);
#44541=EDGE_CURVE('',#35323,#35324,#18620,.T.);
#44542=EDGE_CURVE('',#35324,#35322,#18621,.T.);
#44543=EDGE_CURVE('',#35321,#35323,#18622,.T.);
#44544=EDGE_CURVE('',#35325,#35326,#18623,.T.);
#44545=EDGE_CURVE('',#35326,#35324,#27455,.T.);
#44546=EDGE_CURVE('',#35323,#35325,#27456,.T.);
#44547=EDGE_CURVE('',#35327,#35328,#18624,.T.);
#44548=EDGE_CURVE('',#35328,#35326,#18625,.T.);
#44549=EDGE_CURVE('',#35325,#35327,#18626,.T.);
#44550=EDGE_CURVE('',#35329,#35330,#18627,.T.);
#44551=EDGE_CURVE('',#35330,#35328,#18628,.T.);
#44552=EDGE_CURVE('',#35327,#35329,#18629,.T.);
#44553=EDGE_CURVE('',#35331,#35332,#18630,.T.);
#44554=EDGE_CURVE('',#35332,#35330,#18631,.T.);
#44555=EDGE_CURVE('',#35329,#35331,#18632,.T.);
#44556=EDGE_CURVE('',#35333,#35334,#18633,.T.);
#44557=EDGE_CURVE('',#35334,#35332,#18634,.T.);
#44558=EDGE_CURVE('',#35331,#35333,#18635,.T.);
#44559=EDGE_CURVE('',#35317,#35334,#18636,.T.);
#44560=EDGE_CURVE('',#35333,#35318,#18637,.T.);
#44561=EDGE_CURVE('',#35335,#35330,#27457,.T.);
#44562=EDGE_CURVE('',#35336,#35335,#18638,.T.);
#44563=EDGE_CURVE('',#35337,#35336,#27458,.T.);
#44564=EDGE_CURVE('',#35338,#35337,#18639,.T.);
#44565=EDGE_CURVE('',#35339,#35338,#27459,.T.);
#44566=EDGE_CURVE('',#35340,#35339,#18640,.T.);
#44567=EDGE_CURVE('',#35328,#35340,#27460,.T.);
#44568=EDGE_CURVE('',#35332,#35341,#27461,.T.);
#44569=EDGE_CURVE('',#35341,#35335,#18641,.T.);
#44570=EDGE_CURVE('',#35342,#35334,#27462,.T.);
#44571=EDGE_CURVE('',#35341,#35342,#18642,.T.);
#44572=EDGE_CURVE('',#35317,#35343,#27463,.T.);
#44573=EDGE_CURVE('',#35343,#35342,#18643,.T.);
#44574=EDGE_CURVE('',#35344,#35320,#27464,.T.);
#44575=EDGE_CURVE('',#35343,#35344,#18644,.T.);
#44576=EDGE_CURVE('',#35345,#35346,#18645,.T.);
#44577=EDGE_CURVE('',#35346,#35347,#27465,.T.);
#44578=EDGE_CURVE('',#35347,#35348,#18646,.T.);
#44579=EDGE_CURVE('',#35348,#35345,#27466,.T.);
#44580=EDGE_CURVE('',#35349,#35350,#18647,.T.);
#44581=EDGE_CURVE('',#35350,#35348,#18648,.T.);
#44582=EDGE_CURVE('',#35347,#35349,#18649,.T.);
#44583=EDGE_CURVE('',#35351,#35352,#18650,.T.);
#44584=EDGE_CURVE('',#35352,#35350,#27467,.T.);
#44585=EDGE_CURVE('',#35349,#35351,#27468,.T.);
#44586=EDGE_CURVE('',#35353,#35354,#18651,.T.);
#44587=EDGE_CURVE('',#35354,#35352,#18652,.T.);
#44588=EDGE_CURVE('',#35351,#35353,#18653,.T.);
#44589=EDGE_CURVE('',#35355,#35356,#18654,.T.);
#44590=EDGE_CURVE('',#35356,#35354,#18655,.T.);
#44591=EDGE_CURVE('',#35353,#35355,#18656,.T.);
#44592=EDGE_CURVE('',#35357,#35358,#18657,.T.);
#44593=EDGE_CURVE('',#35358,#35356,#18658,.T.);
#44594=EDGE_CURVE('',#35355,#35357,#18659,.T.);
#44595=EDGE_CURVE('',#35359,#35360,#18660,.T.);
#44596=EDGE_CURVE('',#35360,#35358,#18661,.T.);
#44597=EDGE_CURVE('',#35357,#35359,#18662,.T.);
#44598=EDGE_CURVE('',#35345,#35360,#18663,.T.);
#44599=EDGE_CURVE('',#35359,#35346,#18664,.T.);
#44600=EDGE_CURVE('',#35358,#35361,#27469,.T.);
#44601=EDGE_CURVE('',#35361,#35362,#18665,.T.);
#44602=EDGE_CURVE('',#35362,#35356,#27470,.T.);
#44603=EDGE_CURVE('',#35363,#35360,#27471,.T.);
#44604=EDGE_CURVE('',#35361,#35363,#18666,.T.);
#44605=EDGE_CURVE('',#35345,#35364,#27472,.T.);
#44606=EDGE_CURVE('',#35364,#35363,#18667,.T.);
#44607=EDGE_CURVE('',#35365,#35348,#27473,.T.);
#44608=EDGE_CURVE('',#35364,#35365,#27474,.T.);
#44609=EDGE_CURVE('',#35366,#35367,#23611,.T.);
#44610=EDGE_CURVE('',#35367,#35368,#23612,.T.);
#44611=EDGE_CURVE('',#35368,#35369,#18668,.T.);
#44612=EDGE_CURVE('',#35369,#35366,#23613,.T.);
#44613=EDGE_CURVE('',#35099,#35370,#18669,.T.);
#44614=EDGE_CURVE('',#35370,#35369,#23614,.T.);
#44615=EDGE_CURVE('',#35368,#35099,#23615,.T.);
#44616=EDGE_CURVE('',#35098,#35371,#23616,.T.);
#44617=EDGE_CURVE('',#35371,#35370,#23617,.T.);
#44618=EDGE_CURVE('',#35368,#35372,#27475,.T.);
#44619=EDGE_CURVE('',#35372,#35100,#18670,.F.);
#44620=EDGE_CURVE('',#35373,#35367,#27476,.T.);
#44621=EDGE_CURVE('',#35373,#35374,#18671,.T.);
#44622=EDGE_CURVE('',#35375,#35374,#27477,.T.);
#44623=EDGE_CURVE('',#35375,#35376,#18672,.T.);
#44624=EDGE_CURVE('',#35376,#35377,#23618,.T.);
#44625=EDGE_CURVE('',#35378,#35377,#18673,.T.);
#44626=EDGE_CURVE('',#35379,#35378,#23619,.T.);
#44627=EDGE_CURVE('',#35380,#35379,#18674,.T.);
#44628=EDGE_CURVE('',#35381,#35380,#27478,.T.);
#44629=EDGE_CURVE('',#35382,#35381,#18675,.T.);
#44630=EDGE_CURVE('',#35383,#35382,#27479,.T.);
#44631=EDGE_CURVE('',#35384,#35383,#18676,.F.);
#44632=EDGE_CURVE('',#35384,#35385,#27480,.T.);
#44633=EDGE_CURVE('',#35385,#35385,#18677,.F.);
#44634=EDGE_CURVE('',#35372,#35384,#18678,.F.);
#44635=EDGE_CURVE('',#35371,#35148,#23620,.F.);
#44636=EDGE_CURVE('',#35366,#35147,#23621,.T.);
#44637=EDGE_CURVE('',#35386,#35096,#18679,.T.);
#44638=EDGE_CURVE('',#35095,#35387,#18680,.F.);
#44639=EDGE_CURVE('',#35387,#35386,#27481,.T.);
#44640=EDGE_CURVE('',#35386,#35388,#27482,.T.);
#44641=EDGE_CURVE('',#35389,#35388,#18681,.T.);
#44642=EDGE_CURVE('',#35390,#35389,#27483,.T.);
#44643=EDGE_CURVE('',#35391,#35390,#27484,.T.);
#44644=EDGE_CURVE('',#35392,#35391,#27485,.T.);
#44645=EDGE_CURVE('',#35136,#35392,#18682,.T.);
#44646=EDGE_CURVE('',#35097,#35149,#18683,.T.);
#44647=EDGE_CURVE('',#35393,#35387,#27486,.T.);
#44648=EDGE_CURVE('',#35394,#35393,#27487,.T.);
#44649=EDGE_CURVE('',#35395,#35394,#27488,.T.);
#44650=EDGE_CURVE('',#35388,#35395,#27489,.T.);
#44651=EDGE_CURVE('',#35396,#35397,#18684,.T.);
#44652=EDGE_CURVE('',#35397,#35398,#27490,.T.);
#44653=EDGE_CURVE('',#35398,#35399,#18685,.F.);
#44654=EDGE_CURVE('',#35399,#35396,#27491,.T.);
#44655=EDGE_CURVE('',#35396,#35400,#18686,.T.);
#44656=EDGE_CURVE('',#35400,#35401,#27492,.T.);
#44657=EDGE_CURVE('',#35401,#35402,#18687,.T.);
#44658=EDGE_CURVE('',#35402,#35204,#27493,.T.);
#44659=EDGE_CURVE('',#35213,#35403,#18688,.T.);
#44660=EDGE_CURVE('',#35403,#35404,#27494,.T.);
#44661=EDGE_CURVE('',#35405,#35404,#18689,.T.);
#44662=EDGE_CURVE('',#35405,#35406,#27495,.T.);
#44663=EDGE_CURVE('',#35407,#35406,#18690,.T.);
#44664=EDGE_CURVE('',#35407,#35177,#18691,.T.);
#44665=EDGE_CURVE('',#35176,#35408,#18692,.T.);
#44666=EDGE_CURVE('',#35408,#35409,#18693,.T.);
#44667=EDGE_CURVE('',#35410,#35409,#18694,.T.);
#44668=EDGE_CURVE('',#35410,#35411,#18695,.T.);
#44669=EDGE_CURVE('',#35412,#35411,#18696,.T.);
#44670=EDGE_CURVE('',#35412,#35413,#27496,.T.);
#44671=EDGE_CURVE('',#35414,#35413,#18697,.T.);
#44672=EDGE_CURVE('',#35414,#35415,#27497,.T.);
#44673=EDGE_CURVE('',#35415,#35416,#27498,.T.);
#44674=EDGE_CURVE('',#35416,#35417,#27499,.T.);
#44675=EDGE_CURVE('',#35418,#35417,#18698,.T.);
#44676=EDGE_CURVE('',#35418,#35419,#27500,.T.);
#44677=EDGE_CURVE('',#35419,#35420,#18699,.T.);
#44678=EDGE_CURVE('',#35420,#35397,#27501,.T.);
#44679=EDGE_CURVE('',#35421,#35421,#18700,.T.);
#44680=EDGE_CURVE('',#35399,#35422,#18701,.T.);
#44681=EDGE_CURVE('',#35400,#35422,#27502,.T.);
#44682=EDGE_CURVE('',#35423,#35398,#27503,.T.);
#44683=EDGE_CURVE('',#35424,#35423,#18702,.T.);
#44684=EDGE_CURVE('',#35425,#35424,#27504,.T.);
#44685=EDGE_CURVE('',#35426,#35425,#18703,.T.);
#44686=EDGE_CURVE('',#35426,#35427,#27505,.T.);
#44687=EDGE_CURVE('',#35428,#35427,#18704,.T.);
#44688=EDGE_CURVE('',#35428,#35429,#27506,.T.);
#44689=EDGE_CURVE('',#35430,#35429,#18705,.T.);
#44690=EDGE_CURVE('',#35376,#35430,#18706,.T.);
#44691=EDGE_CURVE('',#35212,#35375,#18707,.F.);
#44692=EDGE_CURVE('',#35431,#35211,#18708,.T.);
#44693=EDGE_CURVE('',#35432,#35431,#18709,.T.);
#44694=EDGE_CURVE('',#35433,#35432,#18710,.T.);
#44695=EDGE_CURVE('',#35434,#35433,#18711,.F.);
#44696=EDGE_CURVE('',#35206,#35434,#18712,.F.);
#44697=EDGE_CURVE('',#35435,#35205,#27507,.T.);
#44698=EDGE_CURVE('',#35436,#35435,#18713,.T.);
#44699=EDGE_CURVE('',#35422,#35436,#27508,.T.);
#44700=EDGE_CURVE('',#35437,#35438,#18714,.T.);
#44701=EDGE_CURVE('',#35437,#35243,#27509,.T.);
#44702=EDGE_CURVE('',#35439,#35249,#18715,.T.);
#44703=EDGE_CURVE('',#35439,#35440,#18716,.T.);
#44704=EDGE_CURVE('',#35440,#35441,#18717,.T.);
#44705=EDGE_CURVE('',#35442,#35441,#18718,.T.);
#44706=EDGE_CURVE('',#35442,#35438,#27510,.T.);
#44707=EDGE_CURVE('',#35443,#35443,#18719,.T.);
#44708=EDGE_CURVE('',#35444,#35420,#27511,.T.);
#44709=EDGE_CURVE('',#35444,#35445,#27512,.T.);
#44710=EDGE_CURVE('',#35423,#35445,#27513,.T.);
#44711=EDGE_CURVE('',#35425,#35446,#27514,.T.);
#44712=EDGE_CURVE('',#35446,#35447,#18720,.T.);
#44713=EDGE_CURVE('',#35447,#35426,#27515,.T.);
#44714=EDGE_CURVE('',#35448,#35447,#27516,.T.);
#44715=EDGE_CURVE('',#35427,#35448,#27517,.T.);
#44716=EDGE_CURVE('',#35449,#35446,#27518,.T.);
#44717=EDGE_CURVE('',#35445,#35449,#18721,.T.);
#44718=EDGE_CURVE('',#35450,#35444,#18722,.T.);
#44719=EDGE_CURVE('',#35450,#35451,#27519,.T.);
#44720=EDGE_CURVE('',#35452,#35451,#18723,.T.);
#44721=EDGE_CURVE('',#35452,#35453,#27520,.T.);
#44722=EDGE_CURVE('',#35395,#35453,#18724,.T.);
#44723=EDGE_CURVE('',#35454,#35394,#18725,.T.);
#44724=EDGE_CURVE('',#35454,#35455,#27521,.T.);
#44725=EDGE_CURVE('',#35456,#35455,#18726,.T.);
#44726=EDGE_CURVE('',#35457,#35456,#27522,.T.);
#44727=EDGE_CURVE('',#35458,#35457,#18727,.T.);
#44728=EDGE_CURVE('',#35458,#35459,#18728,.T.);
#44729=EDGE_CURVE('',#35459,#35460,#27523,.T.);
#44730=EDGE_CURVE('',#35460,#35461,#18729,.T.);
#44731=EDGE_CURVE('',#35462,#35461,#18730,.T.);
#44732=EDGE_CURVE('',#35463,#35462,#27524,.T.);
#44733=EDGE_CURVE('',#35464,#35463,#18731,.T.);
#44734=EDGE_CURVE('',#35464,#35465,#27525,.T.);
#44735=EDGE_CURVE('',#35466,#35465,#18732,.T.);
#44736=EDGE_CURVE('',#35466,#35467,#27526,.T.);
#44737=EDGE_CURVE('',#35448,#35467,#18733,.T.);
#44738=EDGE_CURVE('',#35468,#35469,#27527,.T.);
#44739=EDGE_CURVE('',#35469,#35470,#18734,.T.);
#44740=EDGE_CURVE('',#35470,#35471,#27528,.T.);
#44741=EDGE_CURVE('',#35471,#35468,#18735,.T.);
#44742=EDGE_CURVE('',#35472,#35472,#18736,.T.);
#44743=EDGE_CURVE('',#35473,#35473,#18737,.F.);
#44744=EDGE_CURVE('',#35474,#35474,#18738,.T.);
#44745=EDGE_CURVE('',#35467,#35428,#27529,.T.);
#44746=EDGE_CURVE('',#35475,#35466,#27530,.T.);
#44747=EDGE_CURVE('',#35476,#35475,#27531,.T.);
#44748=EDGE_CURVE('',#35429,#35476,#4089,.T.);
#44749=EDGE_CURVE('',#35477,#35475,#18739,.T.);
#44750=EDGE_CURVE('',#35465,#35477,#27532,.T.);
#44751=EDGE_CURVE('',#35463,#35478,#27533,.T.);
#44752=EDGE_CURVE('',#35478,#35479,#18740,.T.);
#44753=EDGE_CURVE('',#35479,#35464,#27534,.T.);
#44754=EDGE_CURVE('',#35480,#35479,#27535,.T.);
#44755=EDGE_CURVE('',#35481,#35480,#4090,.T.);
#44756=EDGE_CURVE('',#35477,#35481,#27536,.T.);
#44757=EDGE_CURVE('',#35482,#35478,#27537,.T.);
#44758=EDGE_CURVE('',#35483,#35482,#18741,.T.);
#44759=EDGE_CURVE('',#35483,#35484,#27538,.T.);
#44760=EDGE_CURVE('',#35485,#35484,#18742,.T.);
#44761=EDGE_CURVE('',#35485,#35486,#27539,.F.);
#44762=EDGE_CURVE('',#35486,#35487,#27540,.F.);
#44763=EDGE_CURVE('',#35488,#35487,#18743,.T.);
#44764=EDGE_CURVE('',#35488,#35489,#18744,.F.);
#44765=EDGE_CURVE('',#35489,#35490,#27541,.T.);
#44766=EDGE_CURVE('',#35491,#35490,#18745,.T.);
#44767=EDGE_CURVE('',#35491,#35307,#27542,.T.);
#44768=EDGE_CURVE('',#35316,#35492,#18746,.T.);
#44769=EDGE_CURVE('',#35380,#35492,#18747,.F.);
#44770=EDGE_CURVE('',#35480,#35379,#18748,.T.);
#44771=EDGE_CURVE('',#35455,#35493,#27543,.T.);
#44772=EDGE_CURVE('',#35493,#35494,#18749,.T.);
#44773=EDGE_CURVE('',#35494,#35456,#27544,.T.);
#44774=EDGE_CURVE('',#35495,#35454,#27545,.T.);
#44775=EDGE_CURVE('',#35493,#35495,#27546,.T.);
#44776=EDGE_CURVE('',#35393,#35495,#18750,.T.);
#44777=EDGE_CURVE('',#35496,#35105,#18751,.T.);
#44778=EDGE_CURVE('',#35496,#35497,#18752,.T.);
#44779=EDGE_CURVE('',#35498,#35497,#18753,.T.);
#44780=EDGE_CURVE('',#35498,#35499,#18754,.T.);
#44781=EDGE_CURVE('',#35101,#35499,#18755,.T.);
#44782=EDGE_CURVE('',#35336,#35383,#18756,.F.);
#44783=EDGE_CURVE('',#35344,#35500,#18757,.F.);
#44784=EDGE_CURVE('',#35500,#35501,#18758,.T.);
#44785=EDGE_CURVE('',#35501,#35502,#27547,.T.);
#44786=EDGE_CURVE('',#35340,#35502,#18759,.T.);
#44787=EDGE_CURVE('',#35503,#35339,#18760,.F.);
#44788=EDGE_CURVE('',#35503,#35494,#27548,.T.);
#44789=EDGE_CURVE('',#35504,#35504,#18761,.T.);
#44790=EDGE_CURVE('',#35453,#35389,#27549,.T.);
#44791=EDGE_CURVE('',#35451,#35418,#27550,.T.);
#44792=EDGE_CURVE('',#35417,#35452,#27551,.T.);
#44793=EDGE_CURVE('',#35416,#35390,#27552,.T.);
#44794=EDGE_CURVE('',#35391,#35415,#27553,.T.);
#44795=EDGE_CURVE('',#35440,#35221,#27554,.T.);
#44796=EDGE_CURVE('',#35219,#35439,#27555,.T.);
#44797=EDGE_CURVE('',#35441,#35223,#27556,.T.);
#44798=EDGE_CURVE('',#35225,#35442,#27557,.T.);
#44799=EDGE_CURVE('',#35438,#35227,#27558,.T.);
#44800=EDGE_CURVE('',#35229,#35437,#27559,.T.);
#44801=EDGE_CURVE('',#35257,#35505,#27560,.T.);
#44802=EDGE_CURVE('',#35505,#35506,#18762,.T.);
#44803=EDGE_CURVE('',#35506,#35255,#27561,.T.);
#44804=EDGE_CURVE('',#35507,#35259,#27562,.T.);
#44805=EDGE_CURVE('',#35505,#35507,#18763,.T.);
#44806=EDGE_CURVE('',#35269,#35507,#18764,.T.);
#44807=EDGE_CURVE('',#35508,#35281,#27563,.T.);
#44808=EDGE_CURVE('',#35509,#35508,#18765,.T.);
#44809=EDGE_CURVE('',#35279,#35509,#27564,.T.);
#44810=EDGE_CURVE('',#35510,#35283,#27565,.T.);
#44811=EDGE_CURVE('',#35508,#35510,#18766,.T.);
#44812=EDGE_CURVE('',#35488,#35285,#27566,.T.);
#44813=EDGE_CURVE('',#35487,#35511,#27567,.T.);
#44814=EDGE_CURVE('',#35511,#35510,#18767,.T.);
#44815=EDGE_CURVE('',#35287,#35489,#27568,.T.);
#44816=EDGE_CURVE('',#35490,#35289,#27569,.T.);
#44817=EDGE_CURVE('',#35291,#35491,#27570,.T.);
#44818=EDGE_CURVE('',#35481,#35268,#18768,.T.);
#44819=EDGE_CURVE('',#35476,#35272,#18769,.T.);
#44820=EDGE_CURVE('',#35411,#35113,#27571,.T.);
#44821=EDGE_CURVE('',#35111,#35410,#27572,.T.);
#44822=EDGE_CURVE('',#35115,#35412,#27573,.T.);
#44823=EDGE_CURVE('',#35413,#35117,#27574,.T.);
#44824=EDGE_CURVE('',#35119,#35414,#27575,.T.);
#44825=EDGE_CURVE('',#35392,#35121,#27576,.T.);
#44826=EDGE_CURVE('',#35083,#35498,#27577,.T.);
#44827=EDGE_CURVE('',#35497,#35081,#27578,.T.);
#44828=EDGE_CURVE('',#35499,#35085,#27579,.T.);
#44829=EDGE_CURVE('',#35079,#35496,#27580,.T.);
#44830=EDGE_CURVE('',#35450,#35419,#27581,.T.);
#44831=EDGE_CURVE('',#35378,#35269,#18770,.T.);
#44832=EDGE_CURVE('',#35449,#35424,#27582,.T.);
#44833=EDGE_CURVE('',#35512,#35462,#27583,.T.);
#44834=EDGE_CURVE('',#35512,#35513,#27584,.F.);
#44835=EDGE_CURVE('',#35482,#35513,#27585,.T.);
#44836=EDGE_CURVE('',#35374,#35514,#18771,.T.);
#44837=EDGE_CURVE('',#35146,#35373,#18772,.T.);
#44838=EDGE_CURVE('',#35515,#35180,#18773,.T.);
#44839=EDGE_CURVE('',#35514,#35515,#27586,.T.);
#44840=EDGE_CURVE('',#35157,#35515,#27587,.T.);
#44841=EDGE_CURVE('',#35516,#35516,#18774,.F.);
#44842=EDGE_CURVE('',#35408,#35517,#27588,.T.);
#44843=EDGE_CURVE('',#35517,#35518,#18775,.T.);
#44844=EDGE_CURVE('',#35409,#35518,#27589,.T.);
#44845=EDGE_CURVE('',#35175,#35517,#18776,.T.);
#44846=EDGE_CURVE('',#35518,#35151,#18777,.T.);
#44847=EDGE_CURVE('',#35315,#35519,#18778,.T.);
#44848=EDGE_CURVE('',#35519,#35492,#27590,.T.);
#44849=EDGE_CURVE('',#35519,#35381,#18779,.T.);
#44850=EDGE_CURVE('',#35520,#35352,#27591,.T.);
#44851=EDGE_CURVE('',#35521,#35520,#27592,.T.);
#44852=EDGE_CURVE('',#35350,#35521,#27593,.T.);
#44853=EDGE_CURVE('',#35354,#35522,#27594,.T.);
#44854=EDGE_CURVE('',#35522,#35520,#18780,.T.);
#44855=EDGE_CURVE('',#35522,#35362,#18781,.T.);
#44856=EDGE_CURVE('',#35190,#35433,#27595,.T.);
#44857=EDGE_CURVE('',#35432,#35188,#27596,.T.);
#44858=EDGE_CURVE('',#35434,#35192,#27597,.T.);
#44859=EDGE_CURVE('',#35404,#35159,#27598,.T.);
#44860=EDGE_CURVE('',#35403,#35514,#27599,.T.);
#44861=EDGE_CURVE('',#35161,#35405,#27600,.T.);
#44862=EDGE_CURVE('',#35406,#35163,#27601,.T.);
#44863=EDGE_CURVE('',#35165,#35407,#27602,.T.);
#44864=EDGE_CURVE('',#35322,#35500,#27603,.T.);
#44865=EDGE_CURVE('',#35501,#35324,#27604,.T.);
#44866=EDGE_CURVE('',#35502,#35326,#27605,.T.);
#44867=EDGE_CURVE('',#35521,#35365,#18782,.T.);
#44868=EDGE_CURVE('',#35186,#35431,#27606,.T.);
#44869=EDGE_CURVE('',#35509,#35314,#18783,.T.);
#44870=EDGE_CURVE('',#35511,#35523,#27607,.T.);
#44871=EDGE_CURVE('',#35523,#35524,#27608,.T.);
#44872=EDGE_CURVE('',#35525,#35524,#18784,.T.);
#44873=EDGE_CURVE('',#35525,#35526,#27609,.T.);
#44874=EDGE_CURVE('',#35527,#35526,#18785,.T.);
#44875=EDGE_CURVE('',#35527,#35528,#27610,.T.);
#44876=EDGE_CURVE('',#35338,#35528,#18786,.T.);
#44877=EDGE_CURVE('',#35382,#35337,#18787,.T.);
#44878=EDGE_CURVE('',#35529,#35529,#18788,.T.);
#44879=EDGE_CURVE('',#35273,#35506,#18789,.T.);
#44880=EDGE_CURVE('',#35506,#35377,#18790,.T.);
#44881=EDGE_CURVE('',#35273,#35430,#27611,.T.);
#44882=EDGE_CURVE('',#35402,#35435,#27612,.T.);
#44883=EDGE_CURVE('',#35436,#35401,#27613,.T.);
#44884=EDGE_CURVE('',#35530,#35530,#18791,.F.);
#44885=EDGE_CURVE('',#35531,#35531,#18792,.T.);
#44886=EDGE_CURVE('',#35531,#35530,#27614,.T.);
#44887=EDGE_CURVE('',#35532,#35532,#18793,.T.);
#44888=EDGE_CURVE('',#35443,#35473,#27615,.T.);
#44889=EDGE_CURVE('',#35533,#35458,#27616,.T.);
#44890=EDGE_CURVE('',#35534,#35533,#18794,.T.);
#44891=EDGE_CURVE('',#35534,#35459,#27617,.T.);
#44892=EDGE_CURVE('',#35535,#35460,#27618,.T.);
#44893=EDGE_CURVE('',#35535,#35534,#27619,.T.);
#44894=EDGE_CURVE('',#35461,#35536,#27620,.T.);
#44895=EDGE_CURVE('',#35536,#35535,#18795,.T.);
#44896=EDGE_CURVE('',#35537,#35538,#18796,.F.);
#44897=EDGE_CURVE('',#35537,#35470,#27621,.T.);
#44898=EDGE_CURVE('',#35538,#35469,#27622,.T.);
#44899=EDGE_CURVE('',#35539,#35537,#27623,.F.);
#44900=EDGE_CURVE('',#35539,#35471,#27624,.T.);
#44901=EDGE_CURVE('',#35540,#35539,#18797,.F.);
#44902=EDGE_CURVE('',#35540,#35468,#27625,.T.);
#44903=EDGE_CURVE('',#35538,#35540,#27626,.F.);
#44904=EDGE_CURVE('',#35541,#35541,#18798,.T.);
#44905=EDGE_CURVE('',#35504,#35474,#27627,.T.);
#44906=EDGE_CURVE('',#35542,#35542,#18799,.T.);
#44907=EDGE_CURVE('',#35542,#35532,#27628,.T.);
#44908=EDGE_CURVE('',#35533,#35543,#18800,.T.);
#44909=EDGE_CURVE('',#35457,#35543,#27629,.T.);
#44910=EDGE_CURVE('',#35544,#35545,#18801,.F.);
#44911=EDGE_CURVE('',#35544,#35485,#27630,.T.);
#44912=EDGE_CURVE('',#35484,#35545,#27631,.T.);
#44913=EDGE_CURVE('',#35546,#35483,#27632,.T.);
#44914=EDGE_CURVE('',#35546,#35545,#27633,.F.);
#44915=EDGE_CURVE('',#35536,#35512,#18802,.F.);
#44916=EDGE_CURVE('',#35513,#35546,#18803,.T.);
#44917=EDGE_CURVE('',#35547,#35548,#18804,.F.);
#44918=EDGE_CURVE('',#35548,#35544,#27634,.T.);
#44919=EDGE_CURVE('',#35543,#35549,#27635,.T.);
#44920=EDGE_CURVE('',#35549,#35550,#18805,.F.);
#44921=EDGE_CURVE('',#35550,#35547,#27636,.T.);
#44922=EDGE_CURVE('',#35421,#35472,#27637,.T.);
#44923=EDGE_CURVE('',#35516,#35541,#27638,.T.);
#44924=EDGE_CURVE('',#35529,#35542,#27639,.T.);
#44925=EDGE_CURVE('',#35528,#35503,#27640,.T.);
#44926=EDGE_CURVE('',#35549,#35527,#27641,.T.);
#44927=EDGE_CURVE('',#35526,#35550,#27642,.T.);
#44928=EDGE_CURVE('',#35547,#35525,#27643,.T.);
#44929=EDGE_CURVE('',#35524,#35548,#27644,.T.);
#44930=EDGE_CURVE('',#35486,#35523,#27645,.F.);
#44931=EDGE_CURVE('',#35551,#35552,#23622,.T.);
#44932=EDGE_CURVE('',#35553,#35551,#23623,.T.);
#44933=EDGE_CURVE('',#35553,#35552,#27646,.T.);
#44934=EDGE_CURVE('',#35552,#35554,#27647,.T.);
#44935=EDGE_CURVE('',#35555,#35553,#27648,.T.);
#44936=EDGE_CURVE('',#35554,#35555,#27649,.T.);
#44937=EDGE_CURVE('',#35556,#35555,#18806,.T.);
#44938=EDGE_CURVE('',#35554,#35556,#18807,.T.);
#44939=EDGE_CURVE('',#35556,#35551,#27650,.T.);
#44940=EDGE_CURVE('',#35557,#35558,#18808,.T.);
#44941=EDGE_CURVE('',#35558,#35559,#27651,.T.);
#44942=EDGE_CURVE('',#35559,#35560,#18809,.F.);
#44943=EDGE_CURVE('',#35560,#35557,#27652,.T.);
#44944=EDGE_CURVE('',#35557,#35561,#18810,.F.);
#44945=EDGE_CURVE('',#35562,#35561,#18811,.T.);
#44946=EDGE_CURVE('',#35562,#35563,#27653,.T.);
#44947=EDGE_CURVE('',#35564,#35563,#18812,.F.);
#44948=EDGE_CURVE('',#35564,#35565,#27654,.T.);
#44949=EDGE_CURVE('',#35566,#35565,#18813,.F.);
#44950=EDGE_CURVE('',#35566,#35567,#18814,.T.);
#44951=EDGE_CURVE('',#35568,#35567,#18815,.F.);
#44952=EDGE_CURVE('',#35568,#35569,#27655,.F.);
#44953=EDGE_CURVE('',#35570,#35569,#18816,.F.);
#44954=EDGE_CURVE('',#35570,#35571,#27656,.F.);
#44955=EDGE_CURVE('',#35572,#35571,#18817,.F.);
#44956=EDGE_CURVE('',#35572,#35573,#27657,.T.);
#44957=EDGE_CURVE('',#35573,#35574,#18818,.T.);
#44958=EDGE_CURVE('',#35574,#35575,#27658,.T.);
#44959=EDGE_CURVE('',#35576,#35575,#18819,.F.);
#44960=EDGE_CURVE('',#35576,#35577,#27659,.F.);
#44961=EDGE_CURVE('',#35578,#35577,#18820,.F.);
#44962=EDGE_CURVE('',#35578,#35558,#27660,.T.);
#44963=EDGE_CURVE('',#35579,#35560,#18821,.T.);
#44964=EDGE_CURVE('',#35561,#35579,#27661,.T.);
#44965=EDGE_CURVE('',#35579,#35580,#18822,.F.);
#44966=EDGE_CURVE('',#35580,#35562,#27662,.T.);
#44967=EDGE_CURVE('',#35581,#35580,#27663,.T.);
#44968=EDGE_CURVE('',#35582,#35581,#27664,.T.);
#44969=EDGE_CURVE('',#35583,#35582,#27665,.T.);
#44970=EDGE_CURVE('',#35563,#35583,#27666,.T.);
#44971=EDGE_CURVE('',#35584,#35585,#18823,.T.);
#44972=EDGE_CURVE('',#35585,#35586,#18824,.T.);
#44973=EDGE_CURVE('',#35586,#35587,#18825,.T.);
#44974=EDGE_CURVE('',#35587,#35584,#18826,.T.);
#44975=EDGE_CURVE('',#35588,#35582,#18827,.T.);
#44976=EDGE_CURVE('',#35582,#35587,#18828,.T.);
#44977=EDGE_CURVE('',#35586,#35588,#18829,.T.);
#44978=EDGE_CURVE('',#35589,#35583,#18830,.T.);
#44979=EDGE_CURVE('',#35588,#35589,#27667,.T.);
#44980=EDGE_CURVE('',#35590,#35591,#18831,.T.);
#44981=EDGE_CURVE('',#35591,#35583,#18832,.T.);
#44982=EDGE_CURVE('',#35589,#35590,#18833,.T.);
#44983=EDGE_CURVE('',#35592,#35593,#18834,.T.);
#44984=EDGE_CURVE('',#35593,#35591,#27668,.T.);
#44985=EDGE_CURVE('',#35590,#35592,#27669,.T.);
#44986=EDGE_CURVE('',#35594,#35595,#18835,.T.);
#44987=EDGE_CURVE('',#35595,#35593,#18836,.T.);
#44988=EDGE_CURVE('',#35592,#35594,#18837,.T.);
#44989=EDGE_CURVE('',#35596,#35597,#18838,.T.);
#44990=EDGE_CURVE('',#35597,#35595,#18839,.T.);
#44991=EDGE_CURVE('',#35594,#35596,#18840,.T.);
#44992=EDGE_CURVE('',#35584,#35597,#18841,.T.);
#44993=EDGE_CURVE('',#35596,#35585,#18842,.T.);
#44994=EDGE_CURVE('',#35595,#35598,#27670,.T.);
#44995=EDGE_CURVE('',#35599,#35598,#18843,.F.);
#44996=EDGE_CURVE('',#35599,#35593,#27671,.T.);
#44997=EDGE_CURVE('',#35600,#35597,#27672,.T.);
#44998=EDGE_CURVE('',#35598,#35600,#18844,.T.);
#44999=EDGE_CURVE('',#35584,#35601,#27673,.T.);
#45000=EDGE_CURVE('',#35601,#35600,#18845,.T.);
#45001=EDGE_CURVE('',#35602,#35587,#27674,.T.);
#45002=EDGE_CURVE('',#35603,#35602,#18846,.T.);
#45003=EDGE_CURVE('',#35604,#35603,#27675,.T.);
#45004=EDGE_CURVE('',#35604,#35601,#18847,.T.);
#45005=EDGE_CURVE('',#35605,#35606,#18848,.T.);
#45006=EDGE_CURVE('',#35606,#35607,#18849,.T.);
#45007=EDGE_CURVE('',#35607,#35608,#18850,.T.);
#45008=EDGE_CURVE('',#35608,#35605,#23624,.T.);
#45009=EDGE_CURVE('',#35609,#35610,#18851,.T.);
#45010=EDGE_CURVE('',#35610,#35611,#18852,.T.);
#45011=EDGE_CURVE('',#35611,#35612,#18853,.T.);
#45012=EDGE_CURVE('',#35612,#35609,#23625,.T.);
#45013=EDGE_CURVE('',#35613,#35614,#18854,.T.);
#45014=EDGE_CURVE('',#35614,#35611,#27676,.T.);
#45015=EDGE_CURVE('',#35610,#35613,#27677,.T.);
#45016=EDGE_CURVE('',#35608,#35614,#18855,.T.);
#45017=EDGE_CURVE('',#35613,#35605,#18856,.T.);
#45018=EDGE_CURVE('',#35615,#35616,#18857,.T.);
#45019=EDGE_CURVE('',#35616,#35617,#18858,.T.);
#45020=EDGE_CURVE('',#35617,#35618,#18859,.T.);
#45021=EDGE_CURVE('',#35618,#35615,#23626,.T.);
#45022=EDGE_CURVE('',#35612,#35617,#18860,.T.);
#45023=EDGE_CURVE('',#35616,#35609,#18861,.T.);
#45024=EDGE_CURVE('',#35619,#35607,#18862,.T.);
#45025=EDGE_CURVE('',#35606,#35620,#18863,.T.);
#45026=EDGE_CURVE('',#35620,#35619,#23627,.T.);
#45027=EDGE_CURVE('',#35618,#35619,#27678,.T.);
#45028=EDGE_CURVE('',#35620,#35615,#27679,.T.);
#45029=EDGE_CURVE('',#35621,#35607,#27680,.T.);
#45030=EDGE_CURVE('',#35622,#35621,#18864,.T.);
#45031=EDGE_CURVE('',#35608,#35622,#27681,.T.);
#45032=EDGE_CURVE('',#35619,#35623,#27682,.T.);
#45033=EDGE_CURVE('',#35621,#35623,#18865,.T.);
#45034=EDGE_CURVE('',#35624,#35618,#27683,.T.);
#45035=EDGE_CURVE('',#35623,#35624,#27684,.T.);
#45036=EDGE_CURVE('',#35625,#35617,#27685,.T.);
#45037=EDGE_CURVE('',#35624,#35625,#18866,.T.);
#45038=EDGE_CURVE('',#35626,#35627,#23628,.T.);
#45039=EDGE_CURVE('',#35626,#35628,#18867,.T.);
#45040=EDGE_CURVE('',#35628,#35629,#18868,.T.);
#45041=EDGE_CURVE('',#35629,#35630,#18869,.T.);
#45042=EDGE_CURVE('',#35627,#35630,#23629,.T.);
#45043=EDGE_CURVE('',#35631,#35632,#18870,.T.);
#45044=EDGE_CURVE('',#35632,#35629,#18871,.T.);
#45045=EDGE_CURVE('',#35628,#35631,#18872,.T.);
#45046=EDGE_CURVE('',#35633,#35634,#23630,.T.);
#45047=EDGE_CURVE('',#35633,#35635,#18873,.T.);
#45048=EDGE_CURVE('',#35636,#35635,#23631,.T.);
#45049=EDGE_CURVE('',#35636,#35632,#18874,.T.);
#45050=EDGE_CURVE('',#35631,#35637,#18875,.T.);
#45051=EDGE_CURVE('',#35634,#35637,#23632,.T.);
#45052=EDGE_CURVE('',#35638,#35629,#27686,.T.);
#45053=EDGE_CURVE('',#35639,#35638,#23633,.F.);
#45054=EDGE_CURVE('',#35640,#35639,#27687,.T.);
#45055=EDGE_CURVE('',#35641,#35640,#23634,.T.);
#45056=EDGE_CURVE('',#35642,#35641,#27688,.T.);
#45057=EDGE_CURVE('',#35643,#35642,#18876,.T.);
#45058=EDGE_CURVE('',#35644,#35643,#27689,.T.);
#45059=EDGE_CURVE('',#35644,#35645,#23635,.T.);
#45060=EDGE_CURVE('',#35645,#35646,#23636,.T.);
#45061=EDGE_CURVE('',#35646,#35647,#23637,.T.);
#45062=EDGE_CURVE('',#35647,#35648,#23638,.T.);
#45063=EDGE_CURVE('',#35648,#35630,#27690,.T.);
#45064=EDGE_CURVE('',#35632,#35649,#27691,.T.);
#45065=EDGE_CURVE('',#35638,#35649,#23639,.F.);
#45066=EDGE_CURVE('',#35636,#35650,#27692,.T.);
#45067=EDGE_CURVE('',#35651,#35650,#18877,.T.);
#45068=EDGE_CURVE('',#35651,#35652,#23640,.T.);
#45069=EDGE_CURVE('',#35652,#35653,#23641,.T.);
#45070=EDGE_CURVE('',#35649,#35653,#18878,.T.);
#45071=EDGE_CURVE('',#35635,#35654,#27693,.T.);
#45072=EDGE_CURVE('',#35654,#35655,#18879,.T.);
#45073=EDGE_CURVE('',#35655,#35636,#27694,.T.);
#45074=EDGE_CURVE('',#35656,#35633,#27695,.T.);
#45075=EDGE_CURVE('',#35657,#35656,#27696,.T.);
#45076=EDGE_CURVE('',#35654,#35657,#18880,.T.);
#45077=EDGE_CURVE('',#35658,#35634,#156,.T.);
#45078=EDGE_CURVE('',#35658,#35659,#27697,.T.);
#45079=EDGE_CURVE('',#35660,#35659,#4091,.T.);
#45080=EDGE_CURVE('',#35660,#35661,#27698,.T.);
#45081=EDGE_CURVE('',#35661,#35662,#4092,.F.);
#45082=EDGE_CURVE('',#35662,#35663,#23642,.T.);
#45083=EDGE_CURVE('',#35664,#35663,#27699,.T.);
#45084=EDGE_CURVE('',#35664,#35656,#18881,.T.);
#45085=EDGE_CURVE('',#35657,#35665,#18882,.T.);
#45086=EDGE_CURVE('',#35665,#35655,#18883,.T.);
#45087=EDGE_CURVE('',#35664,#35665,#27700,.T.);
#45088=EDGE_CURVE('',#35666,#35655,#27701,.T.);
#45089=EDGE_CURVE('',#35666,#35667,#18884,.F.);
#45090=EDGE_CURVE('',#35668,#35667,#18885,.F.);
#45091=EDGE_CURVE('',#35669,#35668,#27702,.T.);
#45092=EDGE_CURVE('',#35650,#35669,#4093,.T.);
#45093=EDGE_CURVE('',#35670,#35670,#18886,.T.);
#45094=EDGE_CURVE('',#35665,#35671,#27703,.T.);
#45095=EDGE_CURVE('',#35671,#35666,#23643,.F.);
#45096=EDGE_CURVE('',#35672,#35663,#18887,.T.);
#45097=EDGE_CURVE('',#35673,#35672,#27704,.T.);
#45098=EDGE_CURVE('',#35673,#35674,#27705,.T.);
#45099=EDGE_CURVE('',#35675,#35674,#27706,.T.);
#45100=EDGE_CURVE('',#35676,#35675,#27707,.T.);
#45101=EDGE_CURVE('',#35577,#35676,#27708,.T.);
#45102=EDGE_CURVE('',#35677,#35576,#27709,.T.);
#45103=EDGE_CURVE('',#35678,#35677,#27710,.T.);
#45104=EDGE_CURVE('',#35679,#35678,#27711,.T.);
#45105=EDGE_CURVE('',#35680,#35679,#27712,.T.);
#45106=EDGE_CURVE('',#35680,#35681,#4094,.T.);
#45107=EDGE_CURVE('',#35671,#35681,#27713,.T.);
#45108=EDGE_CURVE('',#35637,#35682,#27714,.T.);
#45109=EDGE_CURVE('',#35682,#35683,#157,.T.);
#45110=EDGE_CURVE('',#35683,#35658,#27715,.T.);
#45111=EDGE_CURVE('',#35627,#35684,#158,.T.);
#45112=EDGE_CURVE('',#35684,#35683,#27716,.T.);
#45113=EDGE_CURVE('',#35682,#35626,#27717,.T.);
#45114=EDGE_CURVE('',#35683,#35685,#27718,.T.);
#45115=EDGE_CURVE('',#35659,#35685,#4095,.T.);
#45116=EDGE_CURVE('',#35684,#35686,#27719,.T.);
#45117=EDGE_CURVE('',#35685,#35686,#27720,.T.);
#45118=EDGE_CURVE('',#35687,#35688,#18888,.T.);
#45119=EDGE_CURVE('',#35688,#35689,#18889,.T.);
#45120=EDGE_CURVE('',#35689,#35690,#18890,.T.);
#45121=EDGE_CURVE('',#35687,#35690,#23644,.T.);
#45122=EDGE_CURVE('',#35691,#35692,#18891,.T.);
#45123=EDGE_CURVE('',#35692,#35689,#18892,.T.);
#45124=EDGE_CURVE('',#35688,#35691,#18893,.T.);
#45125=EDGE_CURVE('',#35693,#35694,#18894,.T.);
#45126=EDGE_CURVE('',#35694,#35692,#18895,.T.);
#45127=EDGE_CURVE('',#35691,#35693,#18896,.T.);
#45128=EDGE_CURVE('',#35695,#35696,#18897,.T.);
#45129=EDGE_CURVE('',#35696,#35694,#18898,.T.);
#45130=EDGE_CURVE('',#35693,#35695,#18899,.T.);
#45131=EDGE_CURVE('',#35697,#35696,#27721,.T.);
#45132=EDGE_CURVE('',#35695,#35698,#27722,.T.);
#45133=EDGE_CURVE('',#35698,#35697,#159,.T.);
#45134=EDGE_CURVE('',#35690,#35697,#27723,.T.);
#45135=EDGE_CURVE('',#35698,#35687,#27724,.T.);
#45136=EDGE_CURVE('',#35697,#35699,#27725,.T.);
#45137=EDGE_CURVE('',#35700,#35699,#18900,.T.);
#45138=EDGE_CURVE('',#35701,#35700,#27726,.T.);
#45139=EDGE_CURVE('',#35702,#35701,#27727,.T.);
#45140=EDGE_CURVE('',#35696,#35702,#27728,.T.);
#45141=EDGE_CURVE('',#35690,#35703,#27729,.T.);
#45142=EDGE_CURVE('',#35704,#35703,#4096,.F.);
#45143=EDGE_CURVE('',#35705,#35704,#27730,.T.);
#45144=EDGE_CURVE('',#35706,#35705,#27731,.T.);
#45145=EDGE_CURVE('',#35706,#35699,#23645,.T.);
#45146=EDGE_CURVE('',#35707,#35689,#27732,.T.);
#45147=EDGE_CURVE('',#35703,#35707,#18901,.T.);
#45148=EDGE_CURVE('',#35708,#35709,#23646,.T.);
#45149=EDGE_CURVE('',#35708,#35710,#18902,.T.);
#45150=EDGE_CURVE('',#35711,#35710,#23647,.T.);
#45151=EDGE_CURVE('',#35712,#35711,#23648,.T.);
#45152=EDGE_CURVE('',#35712,#35713,#18903,.T.);
#45153=EDGE_CURVE('',#35714,#35713,#23649,.T.);
#45154=EDGE_CURVE('',#35715,#35714,#23650,.T.);
#45155=EDGE_CURVE('',#35709,#35715,#23651,.T.);
#45156=EDGE_CURVE('',#35715,#35716,#18904,.T.);
#45157=EDGE_CURVE('',#35716,#35709,#18905,.T.);
#45158=EDGE_CURVE('',#35714,#35717,#18906,.T.);
#45159=EDGE_CURVE('',#35717,#35716,#18907,.T.);
#45160=EDGE_CURVE('',#35713,#35718,#18908,.T.);
#45161=EDGE_CURVE('',#35718,#35719,#18909,.T.);
#45162=EDGE_CURVE('',#35719,#35717,#18910,.T.);
#45163=EDGE_CURVE('',#35720,#35712,#18911,.T.);
#45164=EDGE_CURVE('',#35721,#35720,#18912,.T.);
#45165=EDGE_CURVE('',#35722,#35721,#27733,.T.);
#45166=EDGE_CURVE('',#35723,#35722,#18913,.T.);
#45167=EDGE_CURVE('',#35724,#35723,#27734,.T.);
#45168=EDGE_CURVE('',#35725,#35724,#18914,.T.);
#45169=EDGE_CURVE('',#35718,#35725,#27735,.T.);
#45170=EDGE_CURVE('',#35725,#35726,#18915,.T.);
#45171=EDGE_CURVE('',#35726,#35719,#27736,.T.);
#45172=EDGE_CURVE('',#35724,#35727,#18916,.T.);
#45173=EDGE_CURVE('',#35727,#35726,#18917,.T.);
#45174=EDGE_CURVE('',#35723,#35728,#18918,.T.);
#45175=EDGE_CURVE('',#35728,#35727,#27737,.T.);
#45176=EDGE_CURVE('',#35722,#35729,#18919,.T.);
#45177=EDGE_CURVE('',#35729,#35728,#18920,.T.);
#45178=EDGE_CURVE('',#35721,#35730,#18921,.T.);
#45179=EDGE_CURVE('',#35730,#35729,#27738,.T.);
#45180=EDGE_CURVE('',#35720,#35731,#18922,.T.);
#45181=EDGE_CURVE('',#35731,#35730,#18923,.T.);
#45182=EDGE_CURVE('',#35711,#35731,#18924,.T.);
#45183=EDGE_CURVE('',#35716,#35732,#27739,.T.);
#45184=EDGE_CURVE('',#35733,#35732,#18925,.F.);
#45185=EDGE_CURVE('',#35733,#35734,#27740,.T.);
#45186=EDGE_CURVE('',#35708,#35734,#23652,.F.);
#45187=EDGE_CURVE('',#35735,#35717,#27741,.T.);
#45188=EDGE_CURVE('',#35732,#35735,#18926,.F.);
#45189=EDGE_CURVE('',#35736,#35719,#27742,.T.);
#45190=EDGE_CURVE('',#35735,#35736,#18927,.F.);
#45191=EDGE_CURVE('',#35737,#35726,#27743,.T.);
#45192=EDGE_CURVE('',#35736,#35737,#27744,.F.);
#45193=EDGE_CURVE('',#35727,#35738,#27745,.T.);
#45194=EDGE_CURVE('',#35738,#35737,#18928,.F.);
#45195=EDGE_CURVE('',#35739,#35728,#27746,.T.);
#45196=EDGE_CURVE('',#35738,#35739,#27747,.F.);
#45197=EDGE_CURVE('',#35729,#35740,#27748,.T.);
#45198=EDGE_CURVE('',#35740,#35739,#18929,.T.);
#45199=EDGE_CURVE('',#35741,#35730,#27749,.T.);
#45200=EDGE_CURVE('',#35740,#35741,#27750,.T.);
#45201=EDGE_CURVE('',#35731,#35742,#27751,.T.);
#45202=EDGE_CURVE('',#35742,#35741,#18930,.T.);
#45203=EDGE_CURVE('',#35710,#35734,#23653,.F.);
#45204=EDGE_CURVE('',#35733,#35743,#18931,.T.);
#45205=EDGE_CURVE('',#35743,#35744,#27752,.T.);
#45206=EDGE_CURVE('',#35745,#35744,#18932,.F.);
#45207=EDGE_CURVE('',#35746,#35745,#27753,.T.);
#45208=EDGE_CURVE('',#35746,#35747,#160,.T.);
#45209=EDGE_CURVE('',#35748,#35747,#23654,.T.);
#45210=EDGE_CURVE('',#35748,#35749,#23655,.F.);
#45211=EDGE_CURVE('',#35750,#35749,#23656,.T.);
#45212=EDGE_CURVE('',#35751,#35750,#27754,.T.);
#45213=EDGE_CURVE('',#35751,#35742,#18933,.T.);
#45214=EDGE_CURVE('',#35752,#35753,#18934,.T.);
#45215=EDGE_CURVE('',#35753,#35754,#18935,.T.);
#45216=EDGE_CURVE('',#35754,#35755,#18936,.T.);
#45217=EDGE_CURVE('',#35755,#35752,#18937,.T.);
#45218=EDGE_CURVE('',#35756,#35757,#18938,.T.);
#45219=EDGE_CURVE('',#35757,#35755,#18939,.T.);
#45220=EDGE_CURVE('',#35754,#35756,#18940,.T.);
#45221=EDGE_CURVE('',#35758,#35759,#18941,.T.);
#45222=EDGE_CURVE('',#35759,#35757,#27755,.T.);
#45223=EDGE_CURVE('',#35756,#35758,#27756,.T.);
#45224=EDGE_CURVE('',#35760,#35761,#18942,.T.);
#45225=EDGE_CURVE('',#35761,#35759,#18943,.T.);
#45226=EDGE_CURVE('',#35758,#35760,#18944,.T.);
#45227=EDGE_CURVE('',#35762,#35763,#18945,.T.);
#45228=EDGE_CURVE('',#35763,#35761,#27757,.T.);
#45229=EDGE_CURVE('',#35760,#35762,#27758,.T.);
#45230=EDGE_CURVE('',#35764,#35765,#18946,.T.);
#45231=EDGE_CURVE('',#35765,#35763,#18947,.T.);
#45232=EDGE_CURVE('',#35762,#35764,#18948,.T.);
#45233=EDGE_CURVE('',#35766,#35767,#18949,.T.);
#45234=EDGE_CURVE('',#35767,#35768,#18950,.T.);
#45235=EDGE_CURVE('',#35768,#35769,#18951,.T.);
#45236=EDGE_CURVE('',#35769,#35766,#18952,.T.);
#45237=EDGE_CURVE('',#35770,#35771,#18953,.T.);
#45238=EDGE_CURVE('',#35771,#35769,#18954,.T.);
#45239=EDGE_CURVE('',#35768,#35770,#18955,.T.);
#45240=EDGE_CURVE('',#35772,#35773,#18956,.T.);
#45241=EDGE_CURVE('',#35773,#35771,#18957,.T.);
#45242=EDGE_CURVE('',#35770,#35772,#18958,.T.);
#45243=EDGE_CURVE('',#35753,#35774,#18959,.T.);
#45244=EDGE_CURVE('',#35774,#35773,#27759,.T.);
#45245=EDGE_CURVE('',#35772,#35753,#27760,.T.);
#45246=EDGE_CURVE('',#35766,#35765,#18960,.T.);
#45247=EDGE_CURVE('',#35764,#35767,#18961,.T.);
#45248=EDGE_CURVE('',#35752,#35774,#18962,.T.);
#45249=EDGE_CURVE('',#35775,#35759,#27761,.T.);
#45250=EDGE_CURVE('',#35776,#35775,#27762,.T.);
#45251=EDGE_CURVE('',#35757,#35776,#27763,.T.);
#45252=EDGE_CURVE('',#35761,#35777,#27764,.T.);
#45253=EDGE_CURVE('',#35777,#35775,#18963,.T.);
#45254=EDGE_CURVE('',#35778,#35763,#27765,.T.);
#45255=EDGE_CURVE('',#35777,#35778,#27766,.T.);
#45256=EDGE_CURVE('',#35765,#35779,#27767,.T.);
#45257=EDGE_CURVE('',#35779,#35778,#18964,.T.);
#45258=EDGE_CURVE('',#35780,#35766,#27768,.T.);
#45259=EDGE_CURVE('',#35779,#35780,#18965,.T.);
#45260=EDGE_CURVE('',#35781,#35769,#27769,.T.);
#45261=EDGE_CURVE('',#35780,#35781,#18966,.T.);
#45262=EDGE_CURVE('',#35782,#35783,#18967,.T.);
#45263=EDGE_CURVE('',#35783,#35784,#27770,.T.);
#45264=EDGE_CURVE('',#35784,#35785,#18968,.T.);
#45265=EDGE_CURVE('',#35785,#35782,#27771,.T.);
#45266=EDGE_CURVE('',#35786,#35787,#18969,.T.);
#45267=EDGE_CURVE('',#35787,#35785,#18970,.T.);
#45268=EDGE_CURVE('',#35784,#35786,#18971,.T.);
#45269=EDGE_CURVE('',#35788,#35789,#18972,.T.);
#45270=EDGE_CURVE('',#35789,#35787,#27772,.T.);
#45271=EDGE_CURVE('',#35786,#35788,#27773,.T.);
#45272=EDGE_CURVE('',#35790,#35791,#18973,.T.);
#45273=EDGE_CURVE('',#35791,#35789,#18974,.T.);
#45274=EDGE_CURVE('',#35788,#35790,#18975,.T.);
#45275=EDGE_CURVE('',#35792,#35793,#18976,.T.);
#45276=EDGE_CURVE('',#35793,#35791,#18977,.T.);
#45277=EDGE_CURVE('',#35790,#35792,#18978,.T.);
#45278=EDGE_CURVE('',#35794,#35795,#18979,.T.);
#45279=EDGE_CURVE('',#35795,#35793,#27774,.T.);
#45280=EDGE_CURVE('',#35792,#35794,#27775,.T.);
#45281=EDGE_CURVE('',#35796,#35797,#18980,.T.);
#45282=EDGE_CURVE('',#35797,#35795,#18981,.T.);
#45283=EDGE_CURVE('',#35794,#35796,#18982,.T.);
#45284=EDGE_CURVE('',#35798,#35799,#18983,.T.);
#45285=EDGE_CURVE('',#35799,#35797,#18984,.T.);
#45286=EDGE_CURVE('',#35796,#35798,#18985,.T.);
#45287=EDGE_CURVE('',#35800,#35801,#18986,.T.);
#45288=EDGE_CURVE('',#35801,#35799,#18987,.T.);
#45289=EDGE_CURVE('',#35798,#35800,#18988,.T.);
#45290=EDGE_CURVE('',#35802,#35803,#18989,.T.);
#45291=EDGE_CURVE('',#35803,#35801,#18990,.T.);
#45292=EDGE_CURVE('',#35800,#35802,#18991,.T.);
#45293=EDGE_CURVE('',#35804,#35805,#18992,.T.);
#45294=EDGE_CURVE('',#35805,#35803,#27776,.T.);
#45295=EDGE_CURVE('',#35802,#35804,#27777,.T.);
#45296=EDGE_CURVE('',#35782,#35805,#18993,.T.);
#45297=EDGE_CURVE('',#35804,#35783,#18994,.T.);
#45298=EDGE_CURVE('',#35799,#35806,#27778,.T.);
#45299=EDGE_CURVE('',#35806,#35807,#18995,.T.);
#45300=EDGE_CURVE('',#35807,#35797,#27779,.T.);
#45301=EDGE_CURVE('',#35808,#35801,#27780,.T.);
#45302=EDGE_CURVE('',#35806,#35808,#18996,.T.);
#45303=EDGE_CURVE('',#35803,#35809,#27781,.T.);
#45304=EDGE_CURVE('',#35809,#35808,#18997,.T.);
#45305=EDGE_CURVE('',#35810,#35805,#27782,.T.);
#45306=EDGE_CURVE('',#35809,#35810,#27783,.T.);
#45307=EDGE_CURVE('',#35782,#35811,#27784,.T.);
#45308=EDGE_CURVE('',#35811,#35810,#18998,.T.);
#45309=EDGE_CURVE('',#35812,#35785,#27785,.T.);
#45310=EDGE_CURVE('',#35811,#35812,#27786,.T.);
#45311=EDGE_CURVE('',#35813,#35814,#18999,.T.);
#45312=EDGE_CURVE('',#35814,#35815,#27787,.T.);
#45313=EDGE_CURVE('',#35815,#35816,#19000,.T.);
#45314=EDGE_CURVE('',#35816,#35813,#27788,.T.);
#45315=EDGE_CURVE('',#35817,#35818,#19001,.T.);
#45316=EDGE_CURVE('',#35818,#35816,#19002,.T.);
#45317=EDGE_CURVE('',#35815,#35817,#19003,.T.);
#45318=EDGE_CURVE('',#35819,#35820,#19004,.T.);
#45319=EDGE_CURVE('',#35820,#35818,#27789,.T.);
#45320=EDGE_CURVE('',#35817,#35819,#27790,.T.);
#45321=EDGE_CURVE('',#35821,#35822,#19005,.T.);
#45322=EDGE_CURVE('',#35822,#35820,#19006,.T.);
#45323=EDGE_CURVE('',#35819,#35821,#19007,.T.);
#45324=EDGE_CURVE('',#35823,#35824,#19008,.T.);
#45325=EDGE_CURVE('',#35824,#35822,#27791,.T.);
#45326=EDGE_CURVE('',#35821,#35823,#27792,.T.);
#45327=EDGE_CURVE('',#35825,#35826,#19009,.T.);
#45328=EDGE_CURVE('',#35826,#35824,#19010,.T.);
#45329=EDGE_CURVE('',#35823,#35825,#19011,.T.);
#45330=EDGE_CURVE('',#35827,#35828,#19012,.T.);
#45331=EDGE_CURVE('',#35828,#35826,#19013,.T.);
#45332=EDGE_CURVE('',#35825,#35827,#19014,.T.);
#45333=EDGE_CURVE('',#35829,#35830,#19015,.T.);
#45334=EDGE_CURVE('',#35830,#35828,#19016,.T.);
#45335=EDGE_CURVE('',#35827,#35829,#19017,.T.);
#45336=EDGE_CURVE('',#35831,#35832,#19018,.T.);
#45337=EDGE_CURVE('',#35832,#35830,#19019,.T.);
#45338=EDGE_CURVE('',#35829,#35831,#19020,.T.);
#45339=EDGE_CURVE('',#35833,#35834,#19021,.T.);
#45340=EDGE_CURVE('',#35834,#35832,#19022,.T.);
#45341=EDGE_CURVE('',#35831,#35833,#19023,.T.);
#45342=EDGE_CURVE('',#35813,#35834,#19024,.T.);
#45343=EDGE_CURVE('',#35833,#35814,#19025,.T.);
#45344=EDGE_CURVE('',#35835,#35828,#27793,.T.);
#45345=EDGE_CURVE('',#35836,#35835,#19026,.F.);
#45346=EDGE_CURVE('',#35836,#35826,#27794,.T.);
#45347=EDGE_CURVE('',#35830,#35837,#27795,.T.);
#45348=EDGE_CURVE('',#35837,#35835,#19027,.T.);
#45349=EDGE_CURVE('',#35832,#35838,#27796,.T.);
#45350=EDGE_CURVE('',#35839,#35838,#19028,.T.);
#45351=EDGE_CURVE('',#35840,#35839,#27797,.T.);
#45352=EDGE_CURVE('',#35840,#35837,#19029,.T.);
#45353=EDGE_CURVE('',#35841,#35834,#27798,.T.);
#45354=EDGE_CURVE('',#35841,#35842,#19030,.F.);
#45355=EDGE_CURVE('',#35843,#35842,#27799,.T.);
#45356=EDGE_CURVE('',#35844,#35843,#23657,.T.);
#45357=EDGE_CURVE('',#35844,#35845,#23658,.F.);
#45358=EDGE_CURVE('',#35846,#35845,#23659,.T.);
#45359=EDGE_CURVE('',#35846,#35847,#161,.T.);
#45360=EDGE_CURVE('',#35848,#35847,#27800,.T.);
#45361=EDGE_CURVE('',#35838,#35848,#19031,.F.);
#45362=EDGE_CURVE('',#35813,#35849,#27801,.T.);
#45363=EDGE_CURVE('',#35849,#35841,#19032,.T.);
#45364=EDGE_CURVE('',#35850,#35816,#27802,.T.);
#45365=EDGE_CURVE('',#35849,#35850,#27803,.T.);
#45366=EDGE_CURVE('',#35851,#35852,#19033,.T.);
#45367=EDGE_CURVE('',#35852,#35853,#19034,.T.);
#45368=EDGE_CURVE('',#35853,#35854,#19035,.T.);
#45369=EDGE_CURVE('',#35854,#35851,#23660,.T.);
#45370=EDGE_CURVE('',#35855,#35856,#19036,.T.);
#45371=EDGE_CURVE('',#35856,#35853,#19037,.T.);
#45372=EDGE_CURVE('',#35852,#35855,#19038,.T.);
#45373=EDGE_CURVE('',#35857,#35858,#19039,.T.);
#45374=EDGE_CURVE('',#35858,#35856,#19040,.T.);
#45375=EDGE_CURVE('',#35855,#35857,#19041,.T.);
#45376=EDGE_CURVE('',#35859,#35860,#19042,.T.);
#45377=EDGE_CURVE('',#35860,#35858,#19043,.T.);
#45378=EDGE_CURVE('',#35857,#35859,#19044,.T.);
#45379=EDGE_CURVE('',#35861,#35860,#27804,.T.);
#45380=EDGE_CURVE('',#35859,#35862,#27805,.T.);
#45381=EDGE_CURVE('',#35861,#35862,#162,.T.);
#45382=EDGE_CURVE('',#35862,#35851,#27806,.T.);
#45383=EDGE_CURVE('',#35863,#35854,#23661,.T.);
#45384=EDGE_CURVE('',#35863,#35864,#27807,.T.);
#45385=EDGE_CURVE('',#35861,#35864,#19045,.T.);
#45386=EDGE_CURVE('',#35860,#35865,#27808,.T.);
#45387=EDGE_CURVE('',#35865,#35866,#19046,.T.);
#45388=EDGE_CURVE('',#35866,#35858,#27809,.T.);
#45389=EDGE_CURVE('',#35864,#35867,#19047,.T.);
#45390=EDGE_CURVE('',#35867,#35868,#27810,.T.);
#45391=EDGE_CURVE('',#35868,#35869,#19048,.F.);
#45392=EDGE_CURVE('',#35870,#35869,#27811,.T.);
#45393=EDGE_CURVE('',#35871,#35870,#27812,.T.);
#45394=EDGE_CURVE('',#35872,#35871,#19049,.T.);
#45395=EDGE_CURVE('',#35865,#35872,#27813,.T.);
#45396=EDGE_CURVE('',#35873,#35863,#23662,.F.);
#45397=EDGE_CURVE('',#35867,#35873,#27814,.T.);
#45398=EDGE_CURVE('',#35874,#35853,#27815,.T.);
#45399=EDGE_CURVE('',#35875,#35874,#19050,.T.);
#45400=EDGE_CURVE('',#35876,#35875,#23663,.T.);
#45401=EDGE_CURVE('',#35876,#35877,#27816,.T.);
#45402=EDGE_CURVE('',#35877,#35878,#23664,.T.);
#45403=EDGE_CURVE('',#35878,#35879,#27817,.T.);
#45404=EDGE_CURVE('',#35880,#35879,#23665,.T.);
#45405=EDGE_CURVE('',#35881,#35880,#19051,.T.);
#45406=EDGE_CURVE('',#35881,#35882,#27818,.T.);
#45407=EDGE_CURVE('',#35883,#35882,#23666,.T.);
#45408=EDGE_CURVE('',#35873,#35883,#27819,.F.);
#45409=EDGE_CURVE('',#35884,#35885,#19052,.T.);
#45410=EDGE_CURVE('',#35885,#35886,#27820,.T.);
#45411=EDGE_CURVE('',#35886,#35887,#19053,.T.);
#45412=EDGE_CURVE('',#35887,#35884,#27821,.T.);
#45413=EDGE_CURVE('',#35888,#35889,#19054,.T.);
#45414=EDGE_CURVE('',#35889,#35887,#19055,.T.);
#45415=EDGE_CURVE('',#35886,#35888,#19056,.T.);
#45416=EDGE_CURVE('',#35890,#35891,#19057,.T.);
#45417=EDGE_CURVE('',#35891,#35889,#27822,.T.);
#45418=EDGE_CURVE('',#35888,#35890,#27823,.T.);
#45419=EDGE_CURVE('',#35892,#35893,#19058,.T.);
#45420=EDGE_CURVE('',#35893,#35891,#19059,.T.);
#45421=EDGE_CURVE('',#35890,#35892,#19060,.T.);
#45422=EDGE_CURVE('',#35894,#35895,#19061,.T.);
#45423=EDGE_CURVE('',#35895,#35893,#19062,.T.);
#45424=EDGE_CURVE('',#35892,#35894,#19063,.T.);
#45425=EDGE_CURVE('',#35896,#35897,#19064,.T.);
#45426=EDGE_CURVE('',#35897,#35895,#19065,.T.);
#45427=EDGE_CURVE('',#35894,#35896,#19066,.T.);
#45428=EDGE_CURVE('',#35898,#35899,#19067,.T.);
#45429=EDGE_CURVE('',#35899,#35897,#27824,.T.);
#45430=EDGE_CURVE('',#35896,#35898,#27825,.T.);
#45431=EDGE_CURVE('',#35900,#35901,#19068,.T.);
#45432=EDGE_CURVE('',#35901,#35899,#19069,.T.);
#45433=EDGE_CURVE('',#35898,#35900,#19070,.T.);
#45434=EDGE_CURVE('',#35902,#35903,#19071,.T.);
#45435=EDGE_CURVE('',#35903,#35904,#19072,.T.);
#45436=EDGE_CURVE('',#35904,#35901,#19073,.T.);
#45437=EDGE_CURVE('',#35900,#35902,#19074,.T.);
#45438=EDGE_CURVE('',#35905,#35906,#19075,.T.);
#45439=EDGE_CURVE('',#35906,#35903,#19076,.T.);
#45440=EDGE_CURVE('',#35902,#35905,#19077,.T.);
#45441=EDGE_CURVE('',#35907,#35908,#19078,.T.);
#45442=EDGE_CURVE('',#35908,#35906,#27826,.T.);
#45443=EDGE_CURVE('',#35905,#35907,#27827,.T.);
#45444=EDGE_CURVE('',#35884,#35908,#19079,.T.);
#45445=EDGE_CURVE('',#35907,#35885,#19080,.T.);
#45446=EDGE_CURVE('',#35901,#35909,#27828,.T.);
#45447=EDGE_CURVE('',#35909,#35910,#19081,.F.);
#45448=EDGE_CURVE('',#35910,#35899,#27829,.T.);
#45449=EDGE_CURVE('',#35911,#35911,#19082,.T.);
#45450=EDGE_CURVE('',#35911,#35904,#27830,.T.);
#45451=EDGE_CURVE('',#35912,#35903,#27831,.T.);
#45452=EDGE_CURVE('',#35913,#35912,#19083,.F.);
#45453=EDGE_CURVE('',#35914,#35913,#27832,.T.);
#45454=EDGE_CURVE('',#35915,#35914,#19084,.T.);
#45455=EDGE_CURVE('',#35916,#35915,#27833,.T.);
#45456=EDGE_CURVE('',#35917,#35916,#19085,.F.);
#45457=EDGE_CURVE('',#35918,#35917,#27834,.T.);
#45458=EDGE_CURVE('',#35919,#35918,#19086,.T.);
#45459=EDGE_CURVE('',#35920,#35919,#27835,.T.);
#45460=EDGE_CURVE('',#35909,#35920,#19087,.F.);
#45461=EDGE_CURVE('',#35906,#35921,#27836,.T.);
#45462=EDGE_CURVE('',#35921,#35912,#19088,.F.);
#45463=EDGE_CURVE('',#35922,#35908,#27837,.T.);
#45464=EDGE_CURVE('',#35921,#35922,#27838,.F.);
#45465=EDGE_CURVE('',#35884,#35923,#27839,.T.);
#45466=EDGE_CURVE('',#35923,#35922,#19089,.F.);
#45467=EDGE_CURVE('',#35887,#35924,#27840,.T.);
#45468=EDGE_CURVE('',#35923,#35924,#27841,.T.);
#45469=EDGE_CURVE('',#35925,#35926,#19090,.T.);
#45470=EDGE_CURVE('',#35926,#35927,#19091,.T.);
#45471=EDGE_CURVE('',#35927,#35928,#19092,.T.);
#45472=EDGE_CURVE('',#35925,#35928,#23667,.T.);
#45473=EDGE_CURVE('',#35929,#35930,#19093,.T.);
#45474=EDGE_CURVE('',#35930,#35927,#19094,.T.);
#45475=EDGE_CURVE('',#35926,#35929,#19095,.T.);
#45476=EDGE_CURVE('',#35931,#35932,#19096,.T.);
#45477=EDGE_CURVE('',#35932,#35930,#27842,.T.);
#45478=EDGE_CURVE('',#35929,#35931,#27843,.T.);
#45479=EDGE_CURVE('',#35933,#35934,#19097,.T.);
#45480=EDGE_CURVE('',#35934,#35932,#19098,.T.);
#45481=EDGE_CURVE('',#35931,#35933,#19099,.T.);
#45482=EDGE_CURVE('',#35935,#35936,#19100,.T.);
#45483=EDGE_CURVE('',#35936,#35934,#27844,.T.);
#45484=EDGE_CURVE('',#35933,#35935,#27845,.T.);
#45485=EDGE_CURVE('',#35937,#35918,#19101,.T.);
#45486=EDGE_CURVE('',#35918,#35936,#19102,.T.);
#45487=EDGE_CURVE('',#35935,#35937,#19103,.T.);
#45488=EDGE_CURVE('',#35938,#35919,#19104,.T.);
#45489=EDGE_CURVE('',#35937,#35938,#19105,.T.);
#45490=EDGE_CURVE('',#35939,#35940,#19106,.T.);
#45491=EDGE_CURVE('',#35940,#35919,#19107,.T.);
#45492=EDGE_CURVE('',#35938,#35939,#19108,.T.);
#45493=EDGE_CURVE('',#35941,#35942,#19109,.T.);
#45494=EDGE_CURVE('',#35942,#35940,#27846,.T.);
#45495=EDGE_CURVE('',#35939,#35941,#27847,.T.);
#45496=EDGE_CURVE('',#35943,#35944,#19110,.T.);
#45497=EDGE_CURVE('',#35944,#35942,#19111,.T.);
#45498=EDGE_CURVE('',#35941,#35943,#19112,.T.);
#45499=EDGE_CURVE('',#35945,#35944,#19113,.T.);
#45500=EDGE_CURVE('',#35943,#35946,#19114,.T.);
#45501=EDGE_CURVE('',#35946,#35945,#23668,.T.);
#45502=EDGE_CURVE('',#35947,#35948,#19115,.T.);
#45503=EDGE_CURVE('',#35945,#35948,#23669,.T.);
#45504=EDGE_CURVE('',#35946,#35925,#19116,.T.);
#45505=EDGE_CURVE('',#35947,#35928,#23670,.T.);
#45506=EDGE_CURVE('',#35949,#35942,#27848,.T.);
#45507=EDGE_CURVE('',#35950,#35949,#27849,.F.);
#45508=EDGE_CURVE('',#35940,#35950,#27850,.T.);
#45509=EDGE_CURVE('',#35944,#35951,#27851,.T.);
#45510=EDGE_CURVE('',#35951,#35949,#19117,.T.);
#45511=EDGE_CURVE('',#35948,#35947,#23671,.F.);
#45512=EDGE_CURVE('',#35952,#35895,#27852,.T.);
#45513=EDGE_CURVE('',#35951,#35952,#19118,.T.);
#45514=EDGE_CURVE('',#35953,#35927,#27853,.T.);
#45515=EDGE_CURVE('',#35953,#35954,#19119,.T.);
#45516=EDGE_CURVE('',#35955,#35954,#27854,.T.);
#45517=EDGE_CURVE('',#35955,#35956,#163,.T.);
#45518=EDGE_CURVE('',#35957,#35956,#23672,.T.);
#45519=EDGE_CURVE('',#35958,#35957,#23673,.F.);
#45520=EDGE_CURVE('',#35959,#35958,#23674,.F.);
#45521=EDGE_CURVE('',#35960,#35959,#23675,.T.);
#45522=EDGE_CURVE('',#35960,#35961,#164,.T.);
#45523=EDGE_CURVE('',#35961,#35962,#165,.T.);
#45524=EDGE_CURVE('',#35963,#35962,#27855,.T.);
#45525=EDGE_CURVE('',#35963,#35964,#19120,.F.);
#45526=EDGE_CURVE('',#35965,#35964,#27856,.T.);
#45527=EDGE_CURVE('',#35965,#35966,#19121,.T.);
#45528=EDGE_CURVE('',#35893,#35966,#27857,.T.);
#45529=EDGE_CURVE('',#35967,#35968,#19122,.T.);
#45530=EDGE_CURVE('',#35968,#35969,#19123,.T.);
#45531=EDGE_CURVE('',#35969,#35970,#19124,.T.);
#45532=EDGE_CURVE('',#35970,#35967,#19125,.T.);
#45533=EDGE_CURVE('',#35971,#35972,#19126,.T.);
#45534=EDGE_CURVE('',#35972,#35970,#19127,.T.);
#45535=EDGE_CURVE('',#35969,#35971,#19128,.T.);
#45536=EDGE_CURVE('',#35973,#35974,#19129,.T.);
#45537=EDGE_CURVE('',#35974,#35972,#27858,.T.);
#45538=EDGE_CURVE('',#35971,#35973,#27859,.T.);
#45539=EDGE_CURVE('',#35975,#35914,#19130,.T.);
#45540=EDGE_CURVE('',#35914,#35974,#19131,.T.);
#45541=EDGE_CURVE('',#35973,#35975,#19132,.T.);
#45542=EDGE_CURVE('',#35976,#35915,#19133,.T.);
#45543=EDGE_CURVE('',#35975,#35976,#19134,.T.);
#45544=EDGE_CURVE('',#35977,#35978,#19135,.T.);
#45545=EDGE_CURVE('',#35978,#35915,#19136,.T.);
#45546=EDGE_CURVE('',#35976,#35977,#19137,.T.);
#45547=EDGE_CURVE('',#35979,#35980,#19138,.T.);
#45548=EDGE_CURVE('',#35980,#35978,#27860,.T.);
#45549=EDGE_CURVE('',#35977,#35979,#27861,.T.);
#45550=EDGE_CURVE('',#35981,#35982,#19139,.T.);
#45551=EDGE_CURVE('',#35982,#35980,#19140,.T.);
#45552=EDGE_CURVE('',#35979,#35981,#19141,.T.);
#45553=EDGE_CURVE('',#35983,#35984,#19142,.T.);
#45554=EDGE_CURVE('',#35984,#35982,#27862,.T.);
#45555=EDGE_CURVE('',#35981,#35983,#27863,.T.);
#45556=EDGE_CURVE('',#35967,#35984,#19143,.T.);
#45557=EDGE_CURVE('',#35983,#35968,#19144,.T.);
#45558=EDGE_CURVE('',#35985,#35980,#27864,.T.);
#45559=EDGE_CURVE('',#35986,#35985,#27865,.F.);
#45560=EDGE_CURVE('',#35978,#35986,#27866,.T.);
#45561=EDGE_CURVE('',#35982,#35987,#27867,.T.);
#45562=EDGE_CURVE('',#35987,#35985,#19145,.T.);
#45563=EDGE_CURVE('',#35988,#35984,#27868,.T.);
#45564=EDGE_CURVE('',#35988,#35987,#27869,.F.);
#45565=EDGE_CURVE('',#35967,#35989,#27870,.T.);
#45566=EDGE_CURVE('',#35989,#35988,#19146,.T.);
#45567=EDGE_CURVE('',#35990,#35970,#27871,.T.);
#45568=EDGE_CURVE('',#35991,#35990,#19147,.F.);
#45569=EDGE_CURVE('',#35992,#35991,#27872,.T.);
#45570=EDGE_CURVE('',#35992,#35993,#19148,.F.);
#45571=EDGE_CURVE('',#35994,#35993,#27873,.T.);
#45572=EDGE_CURVE('',#35994,#35995,#166,.T.);
#45573=EDGE_CURVE('',#35996,#35995,#23676,.T.);
#45574=EDGE_CURVE('',#35997,#35996,#23677,.F.);
#45575=EDGE_CURVE('',#35998,#35997,#23678,.F.);
#45576=EDGE_CURVE('',#35999,#35998,#23679,.T.);
#45577=EDGE_CURVE('',#35999,#36000,#167,.T.);
#45578=EDGE_CURVE('',#36001,#36000,#27874,.T.);
#45579=EDGE_CURVE('',#36001,#35989,#19149,.T.);
#45580=EDGE_CURVE('',#35889,#36002,#27875,.T.);
#45581=EDGE_CURVE('',#36002,#35924,#19150,.F.);
#45582=EDGE_CURVE('',#36003,#35891,#27876,.T.);
#45583=EDGE_CURVE('',#36002,#36003,#27877,.T.);
#45584=EDGE_CURVE('',#35966,#36003,#19151,.T.);
#45585=EDGE_CURVE('',#35856,#36004,#27878,.T.);
#45586=EDGE_CURVE('',#36004,#35874,#19152,.T.);
#45587=EDGE_CURVE('',#36004,#35866,#19153,.T.);
#45588=EDGE_CURVE('',#36005,#36006,#19154,.F.);
#45589=EDGE_CURVE('',#36006,#36007,#27879,.T.);
#45590=EDGE_CURVE('',#36007,#36008,#19155,.T.);
#45591=EDGE_CURVE('',#36008,#36005,#27880,.T.);
#45592=EDGE_CURVE('',#36005,#36009,#27881,.T.);
#45593=EDGE_CURVE('',#36010,#36008,#27882,.T.);
#45594=EDGE_CURVE('',#36011,#36010,#27883,.T.);
#45595=EDGE_CURVE('',#36012,#36011,#27884,.F.);
#45596=EDGE_CURVE('',#36013,#36012,#27885,.T.);
#45597=EDGE_CURVE('',#36014,#36013,#27886,.T.);
#45598=EDGE_CURVE('',#36009,#36014,#27887,.T.);
#45599=EDGE_CURVE('',#36015,#36006,#27888,.T.);
#45600=EDGE_CURVE('',#36016,#36015,#27889,.T.);
#45601=EDGE_CURVE('',#36007,#36016,#27890,.T.);
#45602=EDGE_CURVE('',#35964,#36009,#19156,.T.);
#45603=EDGE_CURVE('',#36014,#35965,#19157,.F.);
#45604=EDGE_CURVE('',#35897,#36017,#27891,.T.);
#45605=EDGE_CURVE('',#36017,#35952,#19158,.T.);
#45606=EDGE_CURVE('',#36010,#36018,#19159,.T.);
#45607=EDGE_CURVE('',#36018,#36019,#27892,.T.);
#45608=EDGE_CURVE('',#36019,#36011,#19160,.F.);
#45609=EDGE_CURVE('',#36020,#36015,#19161,.T.);
#45610=EDGE_CURVE('',#36020,#36021,#27893,.T.);
#45611=EDGE_CURVE('',#36021,#36016,#19162,.T.);
#45612=EDGE_CURVE('',#36020,#36022,#19163,.T.);
#45613=EDGE_CURVE('',#36023,#36022,#27894,.T.);
#45614=EDGE_CURVE('',#36021,#36023,#19164,.T.);
#45615=EDGE_CURVE('',#36024,#36018,#27895,.T.);
#45616=EDGE_CURVE('',#36025,#36024,#27896,.T.);
#45617=EDGE_CURVE('',#36019,#36025,#27897,.F.);
#45618=EDGE_CURVE('',#36025,#36026,#19165,.T.);
#45619=EDGE_CURVE('',#36027,#36024,#19166,.T.);
#45620=EDGE_CURVE('',#36026,#36027,#27898,.T.);
#45621=EDGE_CURVE('',#36028,#36028,#19167,.F.);
#45622=EDGE_CURVE('',#36029,#36029,#19168,.F.);
#45623=EDGE_CURVE('',#36030,#36030,#19169,.T.);
#45624=EDGE_CURVE('',#36030,#36029,#27899,.T.);
#45625=EDGE_CURVE('',#36031,#36031,#19170,.F.);
#45626=EDGE_CURVE('',#36031,#36028,#27900,.T.);
#45627=EDGE_CURVE('',#36032,#35774,#27901,.T.);
#45628=EDGE_CURVE('',#36032,#36033,#27902,.T.);
#45629=EDGE_CURVE('',#36033,#36034,#27903,.T.);
#45630=EDGE_CURVE('',#36035,#36034,#27904,.T.);
#45631=EDGE_CURVE('',#36036,#36035,#27905,.T.);
#45632=EDGE_CURVE('',#36037,#36036,#27906,.T.);
#45633=EDGE_CURVE('',#36038,#36037,#27907,.T.);
#45634=EDGE_CURVE('',#36038,#36039,#27908,.T.);
#45635=EDGE_CURVE('',#35773,#36039,#27909,.T.);
#45636=EDGE_CURVE('',#35752,#36040,#27910,.T.);
#45637=EDGE_CURVE('',#36032,#36040,#19171,.F.);
#45638=EDGE_CURVE('',#36041,#35755,#27911,.T.);
#45639=EDGE_CURVE('',#36040,#36041,#19172,.T.);
#45640=EDGE_CURVE('',#35776,#36041,#19173,.T.);
#45641=EDGE_CURVE('',#36037,#36042,#19174,.T.);
#45642=EDGE_CURVE('',#36042,#36043,#27912,.T.);
#45643=EDGE_CURVE('',#36043,#36038,#19175,.F.);
#45644=EDGE_CURVE('',#36044,#36045,#19176,.F.);
#45645=EDGE_CURVE('',#36045,#36046,#27913,.T.);
#45646=EDGE_CURVE('',#36046,#36047,#19177,.T.);
#45647=EDGE_CURVE('',#36047,#36044,#27914,.T.);
#45648=EDGE_CURVE('',#36048,#36047,#27915,.T.);
#45649=EDGE_CURVE('',#36049,#36048,#27916,.T.);
#45650=EDGE_CURVE('',#36044,#36049,#27917,.F.);
#45651=EDGE_CURVE('',#35771,#36050,#27918,.T.);
#45652=EDGE_CURVE('',#36050,#35781,#19178,.T.);
#45653=EDGE_CURVE('',#36051,#36045,#27919,.T.);
#45654=EDGE_CURVE('',#36052,#36051,#27920,.T.);
#45655=EDGE_CURVE('',#36046,#36052,#27921,.T.);
#45656=EDGE_CURVE('',#36053,#36051,#19179,.T.);
#45657=EDGE_CURVE('',#36053,#36054,#27922,.T.);
#45658=EDGE_CURVE('',#36054,#36052,#19180,.T.);
#45659=EDGE_CURVE('',#36055,#36056,#19181,.T.);
#45660=EDGE_CURVE('',#36056,#36057,#27923,.T.);
#45661=EDGE_CURVE('',#36057,#36058,#19182,.F.);
#45662=EDGE_CURVE('',#36058,#36055,#27924,.T.);
#45663=EDGE_CURVE('',#36034,#36056,#19183,.T.);
#45664=EDGE_CURVE('',#36057,#36033,#19184,.T.);
#45665=EDGE_CURVE('',#36059,#36059,#19185,.T.);
#45666=EDGE_CURVE('',#36059,#36060,#27925,.T.);
#45667=EDGE_CURVE('',#36060,#36060,#19186,.F.);
#45668=EDGE_CURVE('',#36035,#36061,#19187,.T.);
#45669=EDGE_CURVE('',#36061,#36062,#27926,.T.);
#45670=EDGE_CURVE('',#36062,#36036,#19188,.F.);
#45671=EDGE_CURVE('',#36063,#36064,#27927,.T.);
#45672=EDGE_CURVE('',#36064,#36065,#19189,.T.);
#45673=EDGE_CURVE('',#36065,#36066,#27928,.T.);
#45674=EDGE_CURVE('',#36066,#36063,#19190,.T.);
#45675=EDGE_CURVE('',#36067,#36068,#23680,.T.);
#45676=EDGE_CURVE('',#36067,#36069,#27929,.T.);
#45677=EDGE_CURVE('',#36070,#36069,#23681,.T.);
#45678=EDGE_CURVE('',#36068,#36070,#27930,.T.);
#45679=EDGE_CURVE('',#35877,#36071,#27931,.T.);
#45680=EDGE_CURVE('',#36072,#36071,#23682,.T.);
#45681=EDGE_CURVE('',#35878,#36072,#27932,.T.);
#45682=EDGE_CURVE('',#36073,#36073,#19191,.T.);
#45683=EDGE_CURVE('',#36073,#36074,#27933,.T.);
#45684=EDGE_CURVE('',#36074,#36074,#19192,.T.);
#45685=EDGE_CURVE('',#36075,#36076,#27934,.T.);
#45686=EDGE_CURVE('',#36076,#36075,#19193,.T.);
#45687=EDGE_CURVE('',#36077,#36077,#19194,.T.);
#45688=EDGE_CURVE('',#36077,#36074,#27935,.T.);
#45689=EDGE_CURVE('',#36078,#36078,#19195,.T.);
#45690=EDGE_CURVE('',#36078,#36079,#27936,.T.);
#45691=EDGE_CURVE('',#36079,#36079,#19196,.T.);
#45692=EDGE_CURVE('',#36080,#36081,#27937,.T.);
#45693=EDGE_CURVE('',#36081,#36080,#19197,.T.);
#45694=EDGE_CURVE('',#36082,#36082,#19198,.T.);
#45695=EDGE_CURVE('',#36082,#36079,#27938,.T.);
#45696=EDGE_CURVE('',#35871,#36075,#4097,.T.);
#45697=EDGE_CURVE('',#36076,#35872,#4098,.T.);
#45698=EDGE_CURVE('',#36083,#36084,#19199,.T.);
#45699=EDGE_CURVE('',#36085,#36084,#27939,.T.);
#45700=EDGE_CURVE('',#36086,#36085,#27940,.T.);
#45701=EDGE_CURVE('',#36086,#36087,#19200,.T.);
#45702=EDGE_CURVE('',#36088,#36087,#27941,.T.);
#45703=EDGE_CURVE('',#36083,#36088,#27942,.T.);
#45704=EDGE_CURVE('',#36089,#36090,#19201,.T.);
#45705=EDGE_CURVE('',#36091,#36090,#27943,.T.);
#45706=EDGE_CURVE('',#36092,#36091,#27944,.T.);
#45707=EDGE_CURVE('',#36092,#36093,#19202,.T.);
#45708=EDGE_CURVE('',#36094,#36093,#27945,.T.);
#45709=EDGE_CURVE('',#36089,#36094,#27946,.T.);
#45710=EDGE_CURVE('',#36095,#36085,#27947,.T.);
#45711=EDGE_CURVE('',#36095,#36096,#27948,.T.);
#45712=EDGE_CURVE('',#36086,#36096,#27949,.T.);
#45713=EDGE_CURVE('',#36096,#36097,#19203,.T.);
#45714=EDGE_CURVE('',#36097,#36098,#19204,.T.);
#45715=EDGE_CURVE('',#36087,#36098,#27950,.T.);
#45716=EDGE_CURVE('',#36098,#36099,#27951,.T.);
#45717=EDGE_CURVE('',#36088,#36099,#27952,.T.);
#45718=EDGE_CURVE('',#36100,#36091,#27953,.T.);
#45719=EDGE_CURVE('',#36100,#36101,#27954,.T.);
#45720=EDGE_CURVE('',#36092,#36101,#27955,.T.);
#45721=EDGE_CURVE('',#36101,#36102,#19205,.T.);
#45722=EDGE_CURVE('',#36102,#36103,#19206,.T.);
#45723=EDGE_CURVE('',#36093,#36103,#27956,.T.);
#45724=EDGE_CURVE('',#36103,#36104,#27957,.T.);
#45725=EDGE_CURVE('',#36094,#36104,#27958,.T.);
#45726=EDGE_CURVE('',#36101,#36103,#19207,.T.);
#45727=EDGE_CURVE('',#36102,#36105,#19208,.T.);
#45728=EDGE_CURVE('',#36104,#36100,#19209,.T.);
#45729=EDGE_CURVE('',#36096,#36098,#19210,.T.);
#45730=EDGE_CURVE('',#36097,#36106,#19211,.T.);
#45731=EDGE_CURVE('',#36099,#36095,#19212,.T.);
#45732=EDGE_CURVE('',#36107,#36108,#4099,.T.);
#45733=EDGE_CURVE('',#36109,#36108,#27959,.T.);
#45734=EDGE_CURVE('',#36110,#36109,#27960,.T.);
#45735=EDGE_CURVE('',#36110,#36107,#27961,.T.);
#45736=EDGE_CURVE('',#36111,#36107,#19213,.T.);
#45737=EDGE_CURVE('',#36112,#36110,#19214,.T.);
#45738=EDGE_CURVE('',#36112,#36111,#27962,.T.);
#45739=EDGE_CURVE('',#36113,#36111,#4100,.T.);
#45740=EDGE_CURVE('',#36114,#36112,#27963,.T.);
#45741=EDGE_CURVE('',#36113,#36114,#27964,.T.);
#45742=EDGE_CURVE('',#36090,#36113,#4101,.T.);
#45743=EDGE_CURVE('',#36108,#36089,#4102,.T.);
#45744=EDGE_CURVE('',#36115,#36116,#4103,.T.);
#45745=EDGE_CURVE('',#36117,#36116,#27965,.T.);
#45746=EDGE_CURVE('',#36118,#36117,#27966,.T.);
#45747=EDGE_CURVE('',#36118,#36115,#27967,.T.);
#45748=EDGE_CURVE('',#36119,#36115,#19215,.T.);
#45749=EDGE_CURVE('',#36120,#36118,#19216,.T.);
#45750=EDGE_CURVE('',#36120,#36119,#27968,.T.);
#45751=EDGE_CURVE('',#36121,#36119,#4104,.T.);
#45752=EDGE_CURVE('',#36122,#36120,#27969,.T.);
#45753=EDGE_CURVE('',#36121,#36122,#27970,.T.);
#45754=EDGE_CURVE('',#36084,#36121,#4105,.T.);
#45755=EDGE_CURVE('',#36116,#36083,#4106,.T.);
#45756=EDGE_CURVE('',#36123,#36061,#27971,.T.);
#45757=EDGE_CURVE('',#36123,#36124,#27972,.T.);
#45758=EDGE_CURVE('',#36124,#36062,#27973,.F.);
#45759=EDGE_CURVE('',#35744,#36042,#27974,.T.);
#45760=EDGE_CURVE('',#35743,#36043,#27975,.T.);
#45761=EDGE_CURVE('',#36125,#35869,#23683,.T.);
#45762=EDGE_CURVE('',#35883,#35868,#27976,.T.);
#45763=EDGE_CURVE('',#35882,#36126,#23684,.F.);
#45764=EDGE_CURVE('',#36125,#36126,#27977,.F.);
#45765=EDGE_CURVE('',#36125,#36127,#27978,.T.);
#45766=EDGE_CURVE('',#36128,#36126,#27979,.T.);
#45767=EDGE_CURVE('',#36127,#36128,#27980,.T.);
#45768=EDGE_CURVE('',#36129,#36130,#19217,.T.);
#45769=EDGE_CURVE('',#36130,#36131,#27981,.T.);
#45770=EDGE_CURVE('',#36132,#36131,#23685,.F.);
#45771=EDGE_CURVE('',#36132,#36129,#27982,.T.);
#45772=EDGE_CURVE('',#36133,#36134,#27983,.T.);
#45773=EDGE_CURVE('',#36133,#36135,#27984,.T.);
#45774=EDGE_CURVE('',#36135,#36136,#19218,.T.);
#45775=EDGE_CURVE('',#36134,#36136,#27985,.F.);
#45776=EDGE_CURVE('',#36134,#36137,#27986,.T.);
#45777=EDGE_CURVE('',#36136,#36138,#27987,.F.);
#45778=EDGE_CURVE('',#36138,#36137,#27988,.T.);
#45779=EDGE_CURVE('',#36139,#36140,#23686,.T.);
#45780=EDGE_CURVE('',#36132,#36140,#27989,.F.);
#45781=EDGE_CURVE('',#36131,#36135,#23687,.T.);
#45782=EDGE_CURVE('',#36139,#36133,#19219,.F.);
#45783=EDGE_CURVE('',#36141,#36141,#19220,.T.);
#45784=EDGE_CURVE('',#36142,#36142,#19221,.T.);
#45785=EDGE_CURVE('',#36143,#36143,#19222,.T.);
#45786=EDGE_CURVE('',#36143,#36141,#27990,.T.);
#45787=EDGE_CURVE('',#36144,#36145,#23688,.T.);
#45788=EDGE_CURVE('',#36080,#36145,#4107,.F.);
#45789=EDGE_CURVE('',#36081,#36146,#4108,.T.);
#45790=EDGE_CURVE('',#36146,#36144,#19223,.T.);
#45791=EDGE_CURVE('',#36147,#36140,#27991,.T.);
#45792=EDGE_CURVE('',#36129,#36147,#27992,.T.);
#45793=EDGE_CURVE('',#36139,#36148,#27993,.T.);
#45794=EDGE_CURVE('',#36148,#36147,#19224,.T.);
#45795=EDGE_CURVE('',#36144,#36149,#27994,.T.);
#45796=EDGE_CURVE('',#36148,#36146,#27995,.T.);
#45797=EDGE_CURVE('',#36137,#36149,#19225,.T.);
#45798=EDGE_CURVE('',#36150,#36151,#27996,.F.);
#45799=EDGE_CURVE('',#36150,#36149,#23689,.T.);
#45800=EDGE_CURVE('',#36152,#36138,#23690,.F.);
#45801=EDGE_CURVE('',#36151,#36152,#23691,.T.);
#45802=EDGE_CURVE('',#36153,#36150,#19226,.F.);
#45803=EDGE_CURVE('',#36153,#36154,#27997,.T.);
#45804=EDGE_CURVE('',#36154,#36145,#19227,.T.);
#45805=EDGE_CURVE('',#36151,#36155,#19228,.T.);
#45806=EDGE_CURVE('',#36153,#36155,#19229,.F.);
#45807=EDGE_CURVE('',#36127,#35870,#19230,.T.);
#45808=EDGE_CURVE('',#36154,#36156,#19231,.T.);
#45809=EDGE_CURVE('',#36156,#36155,#27998,.T.);
#45810=EDGE_CURVE('',#36157,#36158,#23692,.T.);
#45811=EDGE_CURVE('',#36156,#36157,#19232,.T.);
#45812=EDGE_CURVE('',#36152,#36158,#27999,.T.);
#45813=EDGE_CURVE('',#36159,#36160,#28000,.T.);
#45814=EDGE_CURVE('',#36068,#36159,#28001,.T.);
#45815=EDGE_CURVE('',#36160,#36070,#28002,.T.);
#45816=EDGE_CURVE('',#36160,#36161,#23693,.T.);
#45817=EDGE_CURVE('',#36161,#36157,#28003,.T.);
#45818=EDGE_CURVE('',#36158,#36159,#23694,.T.);
#45819=EDGE_CURVE('',#36162,#36163,#28004,.T.);
#45820=EDGE_CURVE('',#36069,#36162,#28005,.T.);
#45821=EDGE_CURVE('',#36163,#36067,#28006,.T.);
#45822=EDGE_CURVE('',#36163,#36164,#23695,.T.);
#45823=EDGE_CURVE('',#36130,#36164,#19233,.T.);
#45824=EDGE_CURVE('',#35881,#36128,#19234,.T.);
#45825=EDGE_CURVE('',#35879,#36165,#28007,.T.);
#45826=EDGE_CURVE('',#36165,#36072,#28008,.T.);
#45827=EDGE_CURVE('',#36022,#36066,#19235,.F.);
#45828=EDGE_CURVE('',#36166,#36065,#19236,.T.);
#45829=EDGE_CURVE('',#36165,#36166,#23696,.T.);
#45830=EDGE_CURVE('',#36071,#36167,#28009,.T.);
#45831=EDGE_CURVE('',#36168,#36167,#23697,.T.);
#45832=EDGE_CURVE('',#36023,#36168,#19237,.T.);
#45833=EDGE_CURVE('',#36167,#35876,#28010,.T.);
#45834=EDGE_CURVE('',#36169,#36162,#23698,.T.);
#45835=EDGE_CURVE('',#36064,#36169,#19238,.F.);
#45836=EDGE_CURVE('',#36124,#36063,#19239,.F.);
#45837=EDGE_CURVE('',#36161,#36123,#19240,.T.);
#45838=EDGE_CURVE('',#36164,#36169,#28011,.T.);
#45839=EDGE_CURVE('',#36166,#35880,#28012,.T.);
#45840=EDGE_CURVE('',#35875,#36168,#28013,.T.);
#45841=EDGE_CURVE('',#36055,#36027,#28014,.T.);
#45842=EDGE_CURVE('',#36053,#36114,#28015,.F.);
#45843=EDGE_CURVE('',#36109,#36122,#28016,.F.);
#45844=EDGE_CURVE('',#36026,#36117,#28017,.T.);
#45845=EDGE_CURVE('',#36054,#36058,#28018,.T.);
#45846=EDGE_CURVE('',#36170,#36171,#23699,.T.);
#45847=EDGE_CURVE('',#36171,#36172,#28019,.T.);
#45848=EDGE_CURVE('',#36172,#36173,#19241,.T.);
#45849=EDGE_CURVE('',#36173,#36170,#28020,.T.);
#45850=EDGE_CURVE('',#35641,#36174,#23700,.T.);
#45851=EDGE_CURVE('',#36174,#36175,#28021,.T.);
#45852=EDGE_CURVE('',#36175,#35642,#19242,.T.);
#45853=EDGE_CURVE('',#36176,#36177,#23701,.T.);
#45854=EDGE_CURVE('',#36177,#36178,#23702,.T.);
#45855=EDGE_CURVE('',#36179,#36178,#19243,.F.);
#45856=EDGE_CURVE('',#36179,#35681,#23703,.T.);
#45857=EDGE_CURVE('',#36180,#35680,#23704,.T.);
#45858=EDGE_CURVE('',#36180,#36176,#19244,.T.);
#45859=EDGE_CURVE('',#36181,#36182,#28022,.T.);
#45860=EDGE_CURVE('',#36183,#36181,#19245,.T.);
#45861=EDGE_CURVE('',#35705,#36183,#23705,.T.);
#45862=EDGE_CURVE('',#36182,#35704,#19246,.F.);
#45863=EDGE_CURVE('',#36175,#36173,#19247,.T.);
#45864=EDGE_CURVE('',#36170,#36174,#19248,.T.);
#45865=EDGE_CURVE('',#36179,#35667,#28023,.T.);
#45866=EDGE_CURVE('',#36184,#36185,#28024,.T.);
#45867=EDGE_CURVE('',#36186,#36184,#23706,.T.);
#45868=EDGE_CURVE('',#35640,#36186,#23707,.T.);
#45869=EDGE_CURVE('',#36185,#35639,#23708,.F.);
#45870=EDGE_CURVE('',#36187,#36188,#23709,.T.);
#45871=EDGE_CURVE('',#36187,#36189,#28025,.T.);
#45872=EDGE_CURVE('',#36189,#36190,#19249,.T.);
#45873=EDGE_CURVE('',#36190,#36188,#28026,.T.);
#45874=EDGE_CURVE('',#36191,#36190,#19250,.T.);
#45875=EDGE_CURVE('',#36192,#36191,#28027,.T.);
#45876=EDGE_CURVE('',#36192,#36193,#23710,.T.);
#45877=EDGE_CURVE('',#36193,#36194,#23711,.T.);
#45878=EDGE_CURVE('',#36194,#36195,#23712,.T.);
#45879=EDGE_CURVE('',#36195,#36188,#23713,.T.);
#45880=EDGE_CURVE('',#35644,#36196,#23714,.T.);
#45881=EDGE_CURVE('',#35643,#36197,#19251,.T.);
#45882=EDGE_CURVE('',#36197,#36196,#28028,.T.);
#45883=EDGE_CURVE('',#36187,#36198,#23715,.T.);
#45884=EDGE_CURVE('',#36198,#36199,#23716,.T.);
#45885=EDGE_CURVE('',#36199,#36196,#23717,.T.);
#45886=EDGE_CURVE('',#36189,#36197,#19252,.T.);
#45887=EDGE_CURVE('',#36200,#36200,#19253,.T.);
#45888=EDGE_CURVE('',#36200,#36201,#28029,.T.);
#45889=EDGE_CURVE('',#36201,#36201,#19254,.T.);
#45890=EDGE_CURVE('',#36202,#36202,#19255,.T.);
#45891=EDGE_CURVE('',#36200,#36203,#28030,.T.);
#45892=EDGE_CURVE('',#36203,#36203,#19256,.T.);
#45893=EDGE_CURVE('',#36202,#36204,#28031,.T.);
#45894=EDGE_CURVE('',#36204,#36204,#19257,.T.);
#45895=EDGE_CURVE('',#36205,#36205,#19258,.F.);
#45896=EDGE_CURVE('',#36205,#36206,#28032,.T.);
#45897=EDGE_CURVE('',#36206,#36206,#19259,.F.);
#45898=EDGE_CURVE('',#36178,#35668,#23718,.T.);
#45899=EDGE_CURVE('',#36207,#36207,#19260,.T.);
#45900=EDGE_CURVE('',#36207,#36208,#28033,.T.);
#45901=EDGE_CURVE('',#36208,#36208,#19261,.T.);
#45902=EDGE_CURVE('',#35692,#36209,#28034,.T.);
#45903=EDGE_CURVE('',#36209,#35707,#23719,.T.);
#45904=EDGE_CURVE('',#36210,#36210,#19262,.T.);
#45905=EDGE_CURVE('',#36210,#36211,#28035,.T.);
#45906=EDGE_CURVE('',#36211,#36211,#19263,.T.);
#45907=EDGE_CURVE('',#36211,#36212,#28036,.T.);
#45908=EDGE_CURVE('',#36212,#36212,#19264,.T.);
#45909=EDGE_CURVE('',#36213,#36214,#19265,.T.);
#45910=EDGE_CURVE('',#36214,#36215,#28037,.T.);
#45911=EDGE_CURVE('',#36215,#36216,#19266,.F.);
#45912=EDGE_CURVE('',#36216,#36213,#28038,.T.);
#45913=EDGE_CURVE('',#36217,#36218,#28039,.T.);
#45914=EDGE_CURVE('',#36219,#36217,#19267,.F.);
#45915=EDGE_CURVE('',#36220,#36219,#28040,.T.);
#45916=EDGE_CURVE('',#36218,#36220,#19268,.F.);
#45917=EDGE_CURVE('',#36221,#36222,#28041,.T.);
#45918=EDGE_CURVE('',#36222,#36217,#19269,.T.);
#45919=EDGE_CURVE('',#36218,#36221,#19270,.T.);
#45920=EDGE_CURVE('',#35575,#36223,#28042,.T.);
#45921=EDGE_CURVE('',#36223,#35677,#19271,.F.);
#45922=EDGE_CURVE('',#36224,#35574,#28043,.T.);
#45923=EDGE_CURVE('',#36223,#36224,#28044,.T.);
#45924=EDGE_CURVE('',#36224,#36225,#19272,.T.);
#45925=EDGE_CURVE('',#36225,#35573,#28045,.T.);
#45926=EDGE_CURVE('',#36226,#35611,#28046,.T.);
#45927=EDGE_CURVE('',#36226,#36227,#19273,.F.);
#45928=EDGE_CURVE('',#36227,#36228,#28047,.T.);
#45929=EDGE_CURVE('',#36229,#36228,#23720,.T.);
#45930=EDGE_CURVE('',#36230,#36229,#23721,.T.);
#45931=EDGE_CURVE('',#36230,#35612,#28048,.T.);
#45932=EDGE_CURVE('',#36231,#36231,#19274,.T.);
#45933=EDGE_CURVE('',#36231,#36232,#28049,.T.);
#45934=EDGE_CURVE('',#36232,#36232,#19275,.T.);
#45935=EDGE_CURVE('',#36233,#35614,#28050,.T.);
#45936=EDGE_CURVE('',#36226,#36233,#28051,.T.);
#45937=EDGE_CURVE('',#36234,#35622,#23722,.T.);
#45938=EDGE_CURVE('',#36234,#36235,#28052,.T.);
#45939=EDGE_CURVE('',#36235,#36233,#19276,.F.);
#45940=EDGE_CURVE('',#35917,#36236,#19277,.F.);
#45941=EDGE_CURVE('',#36236,#35936,#28053,.T.);
#45942=EDGE_CURVE('',#35625,#36229,#28054,.T.);
#45943=EDGE_CURVE('',#35625,#36230,#19278,.T.);
#45944=EDGE_CURVE('',#35621,#36237,#28055,.T.);
#45945=EDGE_CURVE('',#36237,#36238,#19279,.T.);
#45946=EDGE_CURVE('',#36234,#36238,#23723,.F.);
#45947=EDGE_CURVE('',#35950,#35920,#19280,.F.);
#45948=EDGE_CURVE('',#36239,#36239,#19281,.T.);
#45949=EDGE_CURVE('',#36240,#36240,#19282,.T.);
#45950=EDGE_CURVE('',#36241,#36241,#19283,.T.);
#45951=EDGE_CURVE('',#36239,#36242,#28056,.T.);
#45952=EDGE_CURVE('',#36242,#36242,#19284,.F.);
#45953=EDGE_CURVE('',#36241,#36243,#28057,.T.);
#45954=EDGE_CURVE('',#36243,#36243,#19285,.F.);
#45955=EDGE_CURVE('',#36244,#36245,#4109,.T.);
#45956=EDGE_CURVE('',#36245,#36237,#19286,.T.);
#45957=EDGE_CURVE('',#35623,#36244,#19287,.T.);
#45958=EDGE_CURVE('',#36213,#36219,#19288,.T.);
#45959=EDGE_CURVE('',#36216,#36220,#19289,.F.);
#45960=EDGE_CURVE('',#36246,#36246,#19290,.T.);
#45961=EDGE_CURVE('',#36246,#35670,#28058,.T.);
#45962=EDGE_CURVE('',#36232,#36203,#28059,.T.);
#45963=EDGE_CURVE('',#36247,#36247,#19291,.T.);
#45964=EDGE_CURVE('',#36248,#36248,#19292,.T.);
#45965=EDGE_CURVE('',#36249,#36250,#19293,.T.);
#45966=EDGE_CURVE('',#36250,#36248,#28060,.T.);
#45967=EDGE_CURVE('',#36250,#36249,#19294,.T.);
#45968=EDGE_CURVE('',#35669,#36251,#19295,.F.);
#45969=EDGE_CURVE('',#36251,#35651,#23724,.F.);
#45970=EDGE_CURVE('',#36252,#36185,#23725,.T.);
#45971=EDGE_CURVE('',#35653,#36253,#23726,.F.);
#45972=EDGE_CURVE('',#36253,#36252,#19296,.F.);
#45973=EDGE_CURVE('',#36254,#36182,#23727,.T.);
#45974=EDGE_CURVE('',#36209,#36254,#23728,.F.);
#45975=EDGE_CURVE('',#36204,#36247,#28061,.T.);
#45976=EDGE_CURVE('',#36255,#36251,#23729,.T.);
#45977=EDGE_CURVE('',#36194,#36255,#19297,.F.);
#45978=EDGE_CURVE('',#35661,#36193,#19298,.F.);
#45979=EDGE_CURVE('',#35652,#35660,#19299,.F.);
#45980=EDGE_CURVE('',#35685,#36195,#19300,.T.);
#45981=EDGE_CURVE('',#35647,#35686,#19301,.F.);
#45982=EDGE_CURVE('',#36198,#35646,#19302,.F.);
#45983=EDGE_CURVE('',#35686,#35648,#4110,.T.);
#45984=EDGE_CURVE('',#35645,#36199,#19303,.T.);
#45985=EDGE_CURVE('',#36256,#36257,#28062,.T.);
#45986=EDGE_CURVE('',#36256,#36192,#168,.T.);
#45987=EDGE_CURVE('',#36257,#36191,#28063,.T.);
#45988=EDGE_CURVE('',#36258,#35672,#23730,.T.);
#45989=EDGE_CURVE('',#36256,#36258,#23731,.T.);
#45990=EDGE_CURVE('',#35673,#36257,#19304,.F.);
#45991=EDGE_CURVE('',#36259,#36260,#28064,.T.);
#45992=EDGE_CURVE('',#36261,#36259,#28065,.T.);
#45993=EDGE_CURVE('',#36261,#36262,#28066,.T.);
#45994=EDGE_CURVE('',#36260,#36262,#28067,.T.);
#45995=EDGE_CURVE('',#36263,#36264,#28068,.T.);
#45996=EDGE_CURVE('',#36263,#36265,#28069,.T.);
#45997=EDGE_CURVE('',#36266,#36265,#28070,.T.);
#45998=EDGE_CURVE('',#36264,#36266,#19305,.T.);
#45999=EDGE_CURVE('',#36266,#36259,#23732,.T.);
#46000=EDGE_CURVE('',#36265,#36261,#19306,.T.);
#46001=EDGE_CURVE('',#35700,#36267,#19307,.T.);
#46002=EDGE_CURVE('',#35706,#36267,#19308,.T.);
#46003=EDGE_CURVE('',#36268,#36269,#19309,.T.);
#46004=EDGE_CURVE('',#36270,#36268,#23733,.T.);
#46005=EDGE_CURVE('',#36267,#36270,#28071,.T.);
#46006=EDGE_CURVE('',#36183,#36176,#23734,.T.);
#46007=EDGE_CURVE('',#36269,#36180,#28072,.T.);
#46008=EDGE_CURVE('',#36269,#35679,#19310,.T.);
#46009=EDGE_CURVE('',#35700,#36260,#19311,.T.);
#46010=EDGE_CURVE('',#36260,#36267,#19312,.T.);
#46011=EDGE_CURVE('',#36262,#35701,#19313,.T.);
#46012=EDGE_CURVE('',#36269,#36264,#19314,.T.);
#46013=EDGE_CURVE('',#36264,#35679,#19315,.T.);
#46014=EDGE_CURVE('',#36259,#36270,#19316,.T.);
#46015=EDGE_CURVE('',#36266,#36268,#19317,.T.);
#46016=EDGE_CURVE('',#35678,#36263,#19318,.T.);
#46017=EDGE_CURVE('',#36252,#36271,#28073,.T.);
#46018=EDGE_CURVE('',#36253,#36255,#23735,.T.);
#46019=EDGE_CURVE('',#36271,#36177,#19319,.T.);
#46020=EDGE_CURVE('',#36184,#36271,#23736,.T.);
#46021=EDGE_CURVE('',#36272,#35694,#28074,.T.);
#46022=EDGE_CURVE('',#36172,#36272,#19320,.T.);
#46023=EDGE_CURVE('',#36273,#36171,#23737,.T.);
#46024=EDGE_CURVE('',#36254,#36273,#28075,.T.);
#46025=EDGE_CURVE('',#36181,#36273,#23738,.T.);
#46026=EDGE_CURVE('',#36258,#36274,#23739,.T.);
#46027=EDGE_CURVE('',#36275,#35672,#19321,.T.);
#46028=EDGE_CURVE('',#36275,#36274,#19322,.T.);
#46029=EDGE_CURVE('',#35662,#36275,#19323,.T.);
#46030=EDGE_CURVE('',#36276,#35789,#28076,.T.);
#46031=EDGE_CURVE('',#36277,#36276,#28077,.T.);
#46032=EDGE_CURVE('',#35787,#36277,#28078,.T.);
#46033=EDGE_CURVE('',#36277,#35812,#19324,.T.);
#46034=EDGE_CURVE('',#36278,#35791,#28079,.T.);
#46035=EDGE_CURVE('',#36276,#36278,#19325,.T.);
#46036=EDGE_CURVE('',#35702,#36272,#19326,.T.);
#46037=EDGE_CURVE('',#36279,#35572,#28080,.T.);
#46038=EDGE_CURVE('',#36280,#36279,#28081,.T.);
#46039=EDGE_CURVE('',#36281,#36280,#28082,.T.);
#46040=EDGE_CURVE('',#36281,#36225,#28083,.T.);
#46041=EDGE_CURVE('',#36282,#36280,#19327,.T.);
#46042=EDGE_CURVE('',#36282,#36283,#28084,.T.);
#46043=EDGE_CURVE('',#36283,#36281,#19328,.T.);
#46044=EDGE_CURVE('',#36284,#36285,#19329,.T.);
#46045=EDGE_CURVE('',#36284,#36286,#28085,.T.);
#46046=EDGE_CURVE('',#36286,#36287,#19330,.T.);
#46047=EDGE_CURVE('',#36287,#36285,#28086,.T.);
#46048=EDGE_CURVE('',#36288,#36284,#28087,.F.);
#46049=EDGE_CURVE('',#36289,#36288,#28088,.T.);
#46050=EDGE_CURVE('',#36286,#36289,#28089,.T.);
#46051=EDGE_CURVE('',#36290,#36288,#19331,.T.);
#46052=EDGE_CURVE('',#36290,#36291,#28090,.T.);
#46053=EDGE_CURVE('',#36291,#36289,#19332,.T.);
#46054=EDGE_CURVE('',#36292,#36293,#4111,.T.);
#46055=EDGE_CURVE('',#36293,#35624,#19333,.T.);
#46056=EDGE_CURVE('',#36294,#36228,#23740,.F.);
#46057=EDGE_CURVE('',#36294,#36292,#19334,.T.);
#46058=EDGE_CURVE('',#36238,#36050,#19335,.T.);
#46059=EDGE_CURVE('',#36245,#36295,#28091,.T.);
#46060=EDGE_CURVE('',#36048,#36295,#19336,.T.);
#46061=EDGE_CURVE('',#35793,#36296,#28092,.T.);
#46062=EDGE_CURVE('',#36296,#36278,#19337,.T.);
#46063=EDGE_CURVE('',#35602,#35581,#19338,.T.);
#46064=EDGE_CURVE('',#36297,#35578,#28093,.T.);
#46065=EDGE_CURVE('',#35559,#36297,#28094,.T.);
#46066=EDGE_CURVE('',#36297,#35676,#19339,.T.);
#46067=EDGE_CURVE('',#36298,#36299,#28095,.T.);
#46068=EDGE_CURVE('',#36300,#36298,#28096,.T.);
#46069=EDGE_CURVE('',#36301,#36300,#28097,.T.);
#46070=EDGE_CURVE('',#36301,#36299,#28098,.T.);
#46071=EDGE_CURVE('',#35675,#36298,#19340,.T.);
#46072=EDGE_CURVE('',#35674,#36300,#19341,.T.);
#46073=EDGE_CURVE('',#36302,#36303,#28099,.T.);
#46074=EDGE_CURVE('',#36304,#36302,#28100,.T.);
#46075=EDGE_CURVE('',#36305,#36304,#28101,.F.);
#46076=EDGE_CURVE('',#35569,#36305,#28102,.T.);
#46077=EDGE_CURVE('',#36306,#35568,#28103,.T.);
#46078=EDGE_CURVE('',#36307,#36306,#28104,.T.);
#46079=EDGE_CURVE('',#36303,#36307,#28105,.T.);
#46080=EDGE_CURVE('',#36305,#36308,#19342,.F.);
#46081=EDGE_CURVE('',#36308,#35570,#28106,.T.);
#46082=EDGE_CURVE('',#35571,#36309,#28107,.T.);
#46083=EDGE_CURVE('',#36309,#36308,#28108,.F.);
#46084=EDGE_CURVE('',#36309,#36279,#19343,.F.);
#46085=EDGE_CURVE('',#36310,#36311,#19344,.T.);
#46086=EDGE_CURVE('',#36310,#36292,#28109,.T.);
#46087=EDGE_CURVE('',#35807,#36294,#19345,.F.);
#46088=EDGE_CURVE('',#36296,#36287,#28110,.T.);
#46089=EDGE_CURVE('',#36291,#36311,#28111,.T.);
#46090=EDGE_CURVE('',#36311,#36312,#28112,.T.);
#46091=EDGE_CURVE('',#36312,#36290,#28113,.T.);
#46092=EDGE_CURVE('',#36312,#36313,#19346,.F.);
#46093=EDGE_CURVE('',#36313,#36310,#28114,.T.);
#46094=EDGE_CURVE('',#36295,#36314,#28115,.T.);
#46095=EDGE_CURVE('',#36314,#36049,#19347,.F.);
#46096=EDGE_CURVE('',#36315,#36316,#28116,.T.);
#46097=EDGE_CURVE('',#36299,#36315,#19348,.T.);
#46098=EDGE_CURVE('',#36316,#36301,#19349,.T.);
#46099=EDGE_CURVE('',#36316,#36317,#19350,.T.);
#46100=EDGE_CURVE('',#36283,#36318,#28117,.T.);
#46101=EDGE_CURVE('',#36214,#36318,#19351,.T.);
#46102=EDGE_CURVE('',#36222,#36317,#19352,.T.);
#46103=EDGE_CURVE('',#36317,#36319,#28118,.T.);
#46104=EDGE_CURVE('',#36319,#36315,#19353,.F.);
#46105=EDGE_CURVE('',#36320,#36321,#23741,.T.);
#46106=EDGE_CURVE('',#36319,#36321,#19354,.T.);
#46107=EDGE_CURVE('',#36221,#36322,#19355,.F.);
#46108=EDGE_CURVE('',#36323,#36322,#28119,.T.);
#46109=EDGE_CURVE('',#36320,#36323,#19356,.T.);
#46110=EDGE_CURVE('',#35603,#36323,#19357,.T.);
#46111=EDGE_CURVE('',#36322,#35604,#19358,.F.);
#46112=EDGE_CURVE('',#36324,#36325,#19359,.T.);
#46113=EDGE_CURVE('',#36325,#36324,#19360,.T.);
#46114=EDGE_CURVE('',#36325,#36240,#28120,.T.);
#46115=EDGE_CURVE('',#36326,#36321,#19361,.T.);
#46116=EDGE_CURVE('',#36320,#36326,#19362,.T.);
#46117=EDGE_CURVE('',#36326,#36324,#28121,.T.);
#46118=EDGE_CURVE('',#36327,#35974,#28122,.T.);
#46119=EDGE_CURVE('',#36328,#36327,#28123,.F.);
#46120=EDGE_CURVE('',#35972,#36328,#28124,.T.);
#46121=EDGE_CURVE('',#36329,#35751,#19363,.F.);
#46122=EDGE_CURVE('',#36330,#36329,#28125,.T.);
#46123=EDGE_CURVE('',#35954,#36330,#19364,.F.);
#46124=EDGE_CURVE('',#36331,#35953,#19365,.T.);
#46125=EDGE_CURVE('',#36332,#36331,#28126,.F.);
#46126=EDGE_CURVE('',#36333,#36332,#19366,.T.);
#46127=EDGE_CURVE('',#36333,#36236,#28127,.F.);
#46128=EDGE_CURVE('',#35986,#35916,#19367,.F.);
#46129=EDGE_CURVE('',#36334,#36001,#19368,.F.);
#46130=EDGE_CURVE('',#36335,#36334,#28128,.T.);
#46131=EDGE_CURVE('',#35842,#36335,#19369,.F.);
#46132=EDGE_CURVE('',#36336,#35850,#19370,.T.);
#46133=EDGE_CURVE('',#36336,#36337,#28129,.F.);
#46134=EDGE_CURVE('',#36338,#36337,#19371,.F.);
#46135=EDGE_CURVE('',#36338,#36339,#28130,.F.);
#46136=EDGE_CURVE('',#36339,#35836,#19372,.F.);
#46137=EDGE_CURVE('',#36340,#35840,#19373,.F.);
#46138=EDGE_CURVE('',#36227,#36340,#19374,.T.);
#46139=EDGE_CURVE('',#36039,#36235,#19375,.F.);
#46140=EDGE_CURVE('',#36328,#35990,#19376,.T.);
#46141=EDGE_CURVE('',#35845,#35996,#169,.T.);
#46142=EDGE_CURVE('',#35998,#35844,#170,.T.);
#46143=EDGE_CURVE('',#35997,#36249,#28131,.T.);
#46144=EDGE_CURVE('',#35956,#36341,#171,.T.);
#46145=EDGE_CURVE('',#36342,#35955,#172,.T.);
#46146=EDGE_CURVE('',#36343,#36342,#28132,.T.);
#46147=EDGE_CURVE('',#36341,#36343,#173,.T.);
#46148=EDGE_CURVE('',#36344,#36345,#28133,.T.);
#46149=EDGE_CURVE('',#36346,#36344,#28134,.T.);
#46150=EDGE_CURVE('',#36347,#36346,#28135,.T.);
#46151=EDGE_CURVE('',#36347,#36345,#28136,.T.);
#46152=EDGE_CURVE('',#36348,#36349,#28137,.T.);
#46153=EDGE_CURVE('',#36350,#36348,#28138,.T.);
#46154=EDGE_CURVE('',#36351,#36350,#28139,.T.);
#46155=EDGE_CURVE('',#36349,#36351,#28140,.T.);
#46156=EDGE_CURVE('',#35747,#35961,#174,.T.);
#46157=EDGE_CURVE('',#36350,#35746,#175,.T.);
#46158=EDGE_CURVE('',#35962,#36348,#176,.T.);
#46159=EDGE_CURVE('',#36343,#36329,#28141,.T.);
#46160=EDGE_CURVE('',#36330,#36342,#28142,.T.);
#46161=EDGE_CURVE('',#36341,#35750,#23742,.T.);
#46162=EDGE_CURVE('',#35745,#36351,#19377,.T.);
#46163=EDGE_CURVE('',#36349,#35963,#19378,.T.);
#46164=EDGE_CURVE('',#36346,#35848,#19379,.T.);
#46165=EDGE_CURVE('',#35847,#36347,#177,.T.);
#46166=EDGE_CURVE('',#35993,#36344,#19380,.T.);
#46167=EDGE_CURVE('',#36345,#35994,#178,.T.);
#46168=EDGE_CURVE('',#36352,#36334,#28143,.T.);
#46169=EDGE_CURVE('',#36353,#36352,#28144,.T.);
#46170=EDGE_CURVE('',#36335,#36353,#28145,.T.);
#46171=EDGE_CURVE('',#36000,#36352,#179,.T.);
#46172=EDGE_CURVE('',#35843,#36354,#23743,.T.);
#46173=EDGE_CURVE('',#36353,#36354,#180,.T.);
#46174=EDGE_CURVE('',#36354,#35999,#181,.T.);
#46175=EDGE_CURVE('',#35749,#35957,#182,.T.);
#46176=EDGE_CURVE('',#35959,#36355,#23744,.T.);
#46177=EDGE_CURVE('',#35961,#36355,#19381,.T.);
#46178=EDGE_CURVE('',#36355,#35748,#183,.T.);
#46179=EDGE_CURVE('',#35995,#35846,#184,.T.);
#46180=EDGE_CURVE('',#35839,#36356,#19382,.T.);
#46181=EDGE_CURVE('',#36356,#36340,#28146,.T.);
#46182=EDGE_CURVE('',#35818,#36336,#28147,.T.);
#46183=EDGE_CURVE('',#35822,#36338,#28148,.T.);
#46184=EDGE_CURVE('',#36337,#35820,#28149,.T.);
#46185=EDGE_CURVE('',#35913,#36327,#19383,.F.);
#46186=EDGE_CURVE('',#35565,#36357,#28150,.T.);
#46187=EDGE_CURVE('',#36357,#36358,#19384,.F.);
#46188=EDGE_CURVE('',#36358,#35566,#28151,.T.);
#46189=EDGE_CURVE('',#35567,#36359,#28152,.T.);
#46190=EDGE_CURVE('',#36359,#36358,#19385,.T.);
#46191=EDGE_CURVE('',#36359,#36306,#19386,.F.);
#46192=EDGE_CURVE('',#36307,#35992,#19387,.T.);
#46193=EDGE_CURVE('',#35599,#36357,#28153,.T.);
#46194=EDGE_CURVE('',#36356,#36215,#19388,.F.);
#46195=EDGE_CURVE('',#35991,#36303,#19389,.F.);
#46196=EDGE_CURVE('',#35934,#36333,#28154,.T.);
#46197=EDGE_CURVE('',#36332,#35932,#28155,.T.);
#46198=EDGE_CURVE('',#35930,#36331,#28156,.T.);
#46199=EDGE_CURVE('',#36339,#35824,#28157,.T.);
#46200=EDGE_CURVE('',#36318,#35795,#28158,.T.);
#46201=EDGE_CURVE('',#36285,#36282,#28159,.T.);
#46202=EDGE_CURVE('',#35591,#35564,#28160,.T.);
#46203=EDGE_CURVE('',#36360,#36313,#28161,.F.);
#46204=EDGE_CURVE('',#36361,#36360,#28162,.T.);
#46205=EDGE_CURVE('',#36293,#36361,#28163,.T.);
#46206=EDGE_CURVE('',#36360,#36362,#19390,.F.);
#46207=EDGE_CURVE('',#36362,#36363,#28164,.T.);
#46208=EDGE_CURVE('',#36361,#36363,#19391,.T.);
#46209=EDGE_CURVE('',#36314,#36362,#28165,.F.);
#46210=EDGE_CURVE('',#36363,#36244,#28166,.T.);
#46211=EDGE_CURVE('',#36142,#35958,#28167,.T.);
#46212=EDGE_CURVE('',#36012,#36304,#19392,.F.);
#46213=EDGE_CURVE('',#36302,#36013,#19393,.F.);
#46214=EDGE_CURVE('',#36017,#35910,#28168,.F.);
#59316=ORIENTED_EDGE('',*,*,#44160,.T.);
#59317=ORIENTED_EDGE('',*,*,#44161,.T.);
#59318=ORIENTED_EDGE('',*,*,#44162,.T.);
#59319=ORIENTED_EDGE('',*,*,#44163,.T.);
#59320=ORIENTED_EDGE('',*,*,#44164,.T.);
#59321=ORIENTED_EDGE('',*,*,#44165,.T.);
#59322=ORIENTED_EDGE('',*,*,#44162,.F.);
#59323=ORIENTED_EDGE('',*,*,#44166,.T.);
#59324=ORIENTED_EDGE('',*,*,#44167,.T.);
#59325=ORIENTED_EDGE('',*,*,#44168,.T.);
#59326=ORIENTED_EDGE('',*,*,#44164,.F.);
#59327=ORIENTED_EDGE('',*,*,#44169,.T.);
#59328=ORIENTED_EDGE('',*,*,#44170,.T.);
#59329=ORIENTED_EDGE('',*,*,#44171,.T.);
#59330=ORIENTED_EDGE('',*,*,#44167,.F.);
#59331=ORIENTED_EDGE('',*,*,#44172,.T.);
#59332=ORIENTED_EDGE('',*,*,#44173,.T.);
#59333=ORIENTED_EDGE('',*,*,#44174,.T.);
#59334=ORIENTED_EDGE('',*,*,#44170,.F.);
#59335=ORIENTED_EDGE('',*,*,#44175,.T.);
#59336=ORIENTED_EDGE('',*,*,#44176,.T.);
#59337=ORIENTED_EDGE('',*,*,#44177,.T.);
#59338=ORIENTED_EDGE('',*,*,#44173,.F.);
#59339=ORIENTED_EDGE('',*,*,#44178,.T.);
#59340=ORIENTED_EDGE('',*,*,#44179,.T.);
#59341=ORIENTED_EDGE('',*,*,#44180,.T.);
#59342=ORIENTED_EDGE('',*,*,#44176,.F.);
#59343=ORIENTED_EDGE('',*,*,#44181,.T.);
#59344=ORIENTED_EDGE('',*,*,#44182,.T.);
#59345=ORIENTED_EDGE('',*,*,#44183,.T.);
#59346=ORIENTED_EDGE('',*,*,#44179,.F.);
#59347=ORIENTED_EDGE('',*,*,#44184,.T.);
#59348=ORIENTED_EDGE('',*,*,#44185,.T.);
#59349=ORIENTED_EDGE('',*,*,#44186,.T.);
#59350=ORIENTED_EDGE('',*,*,#44182,.F.);
#59351=ORIENTED_EDGE('',*,*,#44187,.T.);
#59352=ORIENTED_EDGE('',*,*,#44160,.F.);
#59353=ORIENTED_EDGE('',*,*,#44188,.T.);
#59354=ORIENTED_EDGE('',*,*,#44185,.F.);
#59355=ORIENTED_EDGE('',*,*,#44189,.T.);
#59356=ORIENTED_EDGE('',*,*,#44180,.F.);
#59357=ORIENTED_EDGE('',*,*,#44190,.F.);
#59358=ORIENTED_EDGE('',*,*,#44191,.T.);
#59359=ORIENTED_EDGE('',*,*,#44192,.F.);
#59360=ORIENTED_EDGE('',*,*,#44193,.T.);
#59361=ORIENTED_EDGE('',*,*,#44194,.F.);
#59362=ORIENTED_EDGE('',*,*,#44195,.F.);
#59363=ORIENTED_EDGE('',*,*,#44196,.F.);
#59364=ORIENTED_EDGE('',*,*,#44197,.F.);
#59365=ORIENTED_EDGE('',*,*,#44198,.F.);
#59366=ORIENTED_EDGE('',*,*,#44183,.F.);
#59367=ORIENTED_EDGE('',*,*,#44199,.T.);
#59368=ORIENTED_EDGE('',*,*,#44200,.T.);
#59369=ORIENTED_EDGE('',*,*,#44190,.T.);
#59370=ORIENTED_EDGE('',*,*,#44186,.F.);
#59371=ORIENTED_EDGE('',*,*,#44201,.F.);
#59372=ORIENTED_EDGE('',*,*,#44202,.F.);
#59373=ORIENTED_EDGE('',*,*,#44199,.F.);
#59374=ORIENTED_EDGE('',*,*,#44188,.F.);
#59375=ORIENTED_EDGE('',*,*,#44203,.T.);
#59376=ORIENTED_EDGE('',*,*,#44204,.T.);
#59377=ORIENTED_EDGE('',*,*,#44201,.T.);
#59378=ORIENTED_EDGE('',*,*,#44163,.F.);
#59379=ORIENTED_EDGE('',*,*,#44205,.F.);
#59380=ORIENTED_EDGE('',*,*,#44206,.F.);
#59381=ORIENTED_EDGE('',*,*,#44203,.F.);
#59382=ORIENTED_EDGE('',*,*,#44161,.F.);
#59383=ORIENTED_EDGE('',*,*,#44189,.F.);
#59384=ORIENTED_EDGE('',*,*,#44187,.F.);
#59385=ORIENTED_EDGE('',*,*,#44184,.F.);
#59386=ORIENTED_EDGE('',*,*,#44181,.F.);
#59387=ORIENTED_EDGE('',*,*,#44178,.F.);
#59388=ORIENTED_EDGE('',*,*,#44175,.F.);
#59389=ORIENTED_EDGE('',*,*,#44172,.F.);
#59390=ORIENTED_EDGE('',*,*,#44169,.F.);
#59391=ORIENTED_EDGE('',*,*,#44166,.F.);
#59392=ORIENTED_EDGE('',*,*,#44207,.T.);
#59393=ORIENTED_EDGE('',*,*,#44208,.T.);
#59394=ORIENTED_EDGE('',*,*,#44209,.T.);
#59395=ORIENTED_EDGE('',*,*,#44210,.T.);
#59396=ORIENTED_EDGE('',*,*,#44211,.T.);
#59397=ORIENTED_EDGE('',*,*,#44212,.T.);
#59398=ORIENTED_EDGE('',*,*,#44209,.F.);
#59399=ORIENTED_EDGE('',*,*,#44213,.T.);
#59400=ORIENTED_EDGE('',*,*,#44214,.T.);
#59401=ORIENTED_EDGE('',*,*,#44215,.T.);
#59402=ORIENTED_EDGE('',*,*,#44211,.F.);
#59403=ORIENTED_EDGE('',*,*,#44216,.T.);
#59404=ORIENTED_EDGE('',*,*,#44217,.T.);
#59405=ORIENTED_EDGE('',*,*,#44218,.T.);
#59406=ORIENTED_EDGE('',*,*,#44214,.F.);
#59407=ORIENTED_EDGE('',*,*,#44219,.T.);
#59408=ORIENTED_EDGE('',*,*,#44220,.T.);
#59409=ORIENTED_EDGE('',*,*,#44221,.T.);
#59410=ORIENTED_EDGE('',*,*,#44217,.F.);
#59411=ORIENTED_EDGE('',*,*,#44222,.T.);
#59412=ORIENTED_EDGE('',*,*,#44223,.T.);
#59413=ORIENTED_EDGE('',*,*,#44224,.T.);
#59414=ORIENTED_EDGE('',*,*,#44220,.F.);
#59415=ORIENTED_EDGE('',*,*,#44225,.T.);
#59416=ORIENTED_EDGE('',*,*,#44226,.T.);
#59417=ORIENTED_EDGE('',*,*,#44227,.T.);
#59418=ORIENTED_EDGE('',*,*,#44223,.F.);
#59419=ORIENTED_EDGE('',*,*,#44228,.T.);
#59420=ORIENTED_EDGE('',*,*,#44229,.T.);
#59421=ORIENTED_EDGE('',*,*,#44230,.T.);
#59422=ORIENTED_EDGE('',*,*,#44226,.F.);
#59423=ORIENTED_EDGE('',*,*,#44231,.T.);
#59424=ORIENTED_EDGE('',*,*,#44232,.T.);
#59425=ORIENTED_EDGE('',*,*,#44233,.T.);
#59426=ORIENTED_EDGE('',*,*,#44229,.F.);
#59427=ORIENTED_EDGE('',*,*,#44234,.T.);
#59428=ORIENTED_EDGE('',*,*,#44235,.T.);
#59429=ORIENTED_EDGE('',*,*,#44236,.T.);
#59430=ORIENTED_EDGE('',*,*,#44232,.F.);
#59431=ORIENTED_EDGE('',*,*,#44237,.T.);
#59432=ORIENTED_EDGE('',*,*,#44238,.T.);
#59433=ORIENTED_EDGE('',*,*,#44239,.T.);
#59434=ORIENTED_EDGE('',*,*,#44235,.F.);
#59435=ORIENTED_EDGE('',*,*,#44240,.T.);
#59436=ORIENTED_EDGE('',*,*,#44241,.T.);
#59437=ORIENTED_EDGE('',*,*,#44242,.T.);
#59438=ORIENTED_EDGE('',*,*,#44238,.F.);
#59439=ORIENTED_EDGE('',*,*,#44243,.T.);
#59440=ORIENTED_EDGE('',*,*,#44244,.T.);
#59441=ORIENTED_EDGE('',*,*,#44245,.T.);
#59442=ORIENTED_EDGE('',*,*,#44246,.T.);
#59443=ORIENTED_EDGE('',*,*,#44241,.F.);
#59444=ORIENTED_EDGE('',*,*,#44247,.T.);
#59445=ORIENTED_EDGE('',*,*,#44207,.F.);
#59446=ORIENTED_EDGE('',*,*,#44248,.T.);
#59447=ORIENTED_EDGE('',*,*,#44244,.F.);
#59448=ORIENTED_EDGE('',*,*,#44249,.T.);
#59449=ORIENTED_EDGE('',*,*,#44233,.F.);
#59450=ORIENTED_EDGE('',*,*,#44250,.F.);
#59451=ORIENTED_EDGE('',*,*,#44251,.T.);
#59452=ORIENTED_EDGE('',*,*,#44252,.F.);
#59453=ORIENTED_EDGE('',*,*,#44236,.F.);
#59454=ORIENTED_EDGE('',*,*,#44253,.T.);
#59455=ORIENTED_EDGE('',*,*,#44254,.F.);
#59456=ORIENTED_EDGE('',*,*,#44250,.T.);
#59457=ORIENTED_EDGE('',*,*,#44239,.F.);
#59458=ORIENTED_EDGE('',*,*,#44255,.F.);
#59459=ORIENTED_EDGE('',*,*,#44256,.T.);
#59460=ORIENTED_EDGE('',*,*,#44253,.F.);
#59461=ORIENTED_EDGE('',*,*,#44242,.F.);
#59462=ORIENTED_EDGE('',*,*,#44257,.T.);
#59463=ORIENTED_EDGE('',*,*,#44258,.T.);
#59464=ORIENTED_EDGE('',*,*,#44255,.T.);
#59465=ORIENTED_EDGE('',*,*,#44259,.F.);
#59466=ORIENTED_EDGE('',*,*,#44260,.T.);
#59467=ORIENTED_EDGE('',*,*,#44245,.F.);
#59468=ORIENTED_EDGE('',*,*,#44261,.F.);
#59469=ORIENTED_EDGE('',*,*,#44262,.T.);
#59470=ORIENTED_EDGE('',*,*,#44263,.F.);
#59471=ORIENTED_EDGE('',*,*,#44264,.F.);
#59472=ORIENTED_EDGE('',*,*,#44265,.F.);
#59473=ORIENTED_EDGE('',*,*,#44266,.T.);
#59474=ORIENTED_EDGE('',*,*,#44267,.F.);
#59475=ORIENTED_EDGE('',*,*,#44268,.F.);
#59476=ORIENTED_EDGE('',*,*,#44269,.F.);
#59477=ORIENTED_EDGE('',*,*,#44270,.T.);
#59478=ORIENTED_EDGE('',*,*,#44257,.F.);
#59479=ORIENTED_EDGE('',*,*,#44246,.F.);
#59480=ORIENTED_EDGE('',*,*,#44260,.F.);
#59481=ORIENTED_EDGE('',*,*,#44248,.F.);
#59482=ORIENTED_EDGE('',*,*,#44271,.T.);
#59483=ORIENTED_EDGE('',*,*,#44272,.T.);
#59484=ORIENTED_EDGE('',*,*,#44261,.T.);
#59485=ORIENTED_EDGE('',*,*,#44210,.F.);
#59486=ORIENTED_EDGE('',*,*,#44273,.F.);
#59487=ORIENTED_EDGE('',*,*,#44274,.T.);
#59488=ORIENTED_EDGE('',*,*,#44271,.F.);
#59489=ORIENTED_EDGE('',*,*,#44208,.F.);
#59490=ORIENTED_EDGE('',*,*,#44249,.F.);
#59491=ORIENTED_EDGE('',*,*,#44247,.F.);
#59492=ORIENTED_EDGE('',*,*,#44243,.F.);
#59493=ORIENTED_EDGE('',*,*,#44240,.F.);
#59494=ORIENTED_EDGE('',*,*,#44237,.F.);
#59495=ORIENTED_EDGE('',*,*,#44234,.F.);
#59496=ORIENTED_EDGE('',*,*,#44231,.F.);
#59497=ORIENTED_EDGE('',*,*,#44228,.F.);
#59498=ORIENTED_EDGE('',*,*,#44225,.F.);
#59499=ORIENTED_EDGE('',*,*,#44222,.F.);
#59500=ORIENTED_EDGE('',*,*,#44219,.F.);
#59501=ORIENTED_EDGE('',*,*,#44216,.F.);
#59502=ORIENTED_EDGE('',*,*,#44213,.F.);
#59503=ORIENTED_EDGE('',*,*,#44275,.T.);
#59504=ORIENTED_EDGE('',*,*,#44276,.T.);
#59505=ORIENTED_EDGE('',*,*,#44277,.T.);
#59506=ORIENTED_EDGE('',*,*,#44278,.T.);
#59507=ORIENTED_EDGE('',*,*,#44279,.T.);
#59508=ORIENTED_EDGE('',*,*,#44280,.T.);
#59509=ORIENTED_EDGE('',*,*,#44277,.F.);
#59510=ORIENTED_EDGE('',*,*,#44281,.T.);
#59511=ORIENTED_EDGE('',*,*,#44282,.T.);
#59512=ORIENTED_EDGE('',*,*,#44283,.T.);
#59513=ORIENTED_EDGE('',*,*,#44279,.F.);
#59514=ORIENTED_EDGE('',*,*,#44284,.T.);
#59515=ORIENTED_EDGE('',*,*,#44285,.T.);
#59516=ORIENTED_EDGE('',*,*,#44286,.T.);
#59517=ORIENTED_EDGE('',*,*,#44282,.F.);
#59518=ORIENTED_EDGE('',*,*,#44287,.T.);
#59519=ORIENTED_EDGE('',*,*,#44288,.T.);
#59520=ORIENTED_EDGE('',*,*,#44289,.T.);
#59521=ORIENTED_EDGE('',*,*,#44285,.F.);
#59522=ORIENTED_EDGE('',*,*,#44290,.T.);
#59523=ORIENTED_EDGE('',*,*,#44291,.T.);
#59524=ORIENTED_EDGE('',*,*,#44292,.T.);
#59525=ORIENTED_EDGE('',*,*,#44288,.F.);
#59526=ORIENTED_EDGE('',*,*,#44293,.T.);
#59527=ORIENTED_EDGE('',*,*,#44294,.T.);
#59528=ORIENTED_EDGE('',*,*,#44295,.T.);
#59529=ORIENTED_EDGE('',*,*,#44291,.F.);
#59530=ORIENTED_EDGE('',*,*,#44296,.T.);
#59531=ORIENTED_EDGE('',*,*,#44297,.T.);
#59532=ORIENTED_EDGE('',*,*,#44298,.T.);
#59533=ORIENTED_EDGE('',*,*,#44294,.F.);
#59534=ORIENTED_EDGE('',*,*,#44299,.T.);
#59535=ORIENTED_EDGE('',*,*,#44300,.T.);
#59536=ORIENTED_EDGE('',*,*,#44301,.T.);
#59537=ORIENTED_EDGE('',*,*,#44297,.F.);
#59538=ORIENTED_EDGE('',*,*,#44302,.T.);
#59539=ORIENTED_EDGE('',*,*,#44303,.T.);
#59540=ORIENTED_EDGE('',*,*,#44304,.T.);
#59541=ORIENTED_EDGE('',*,*,#44300,.F.);
#59542=ORIENTED_EDGE('',*,*,#44305,.T.);
#59543=ORIENTED_EDGE('',*,*,#44306,.T.);
#59544=ORIENTED_EDGE('',*,*,#44264,.T.);
#59545=ORIENTED_EDGE('',*,*,#44303,.F.);
#59546=ORIENTED_EDGE('',*,*,#44307,.T.);
#59547=ORIENTED_EDGE('',*,*,#44275,.F.);
#59548=ORIENTED_EDGE('',*,*,#44308,.T.);
#59549=ORIENTED_EDGE('',*,*,#44306,.F.);
#59550=ORIENTED_EDGE('',*,*,#44309,.T.);
#59551=ORIENTED_EDGE('',*,*,#44298,.F.);
#59552=ORIENTED_EDGE('',*,*,#44310,.T.);
#59553=ORIENTED_EDGE('',*,*,#44311,.T.);
#59554=ORIENTED_EDGE('',*,*,#44312,.T.);
#59555=ORIENTED_EDGE('',*,*,#44313,.T.);
#59556=ORIENTED_EDGE('',*,*,#44314,.T.);
#59557=ORIENTED_EDGE('',*,*,#44301,.F.);
#59558=ORIENTED_EDGE('',*,*,#44315,.F.);
#59559=ORIENTED_EDGE('',*,*,#44316,.T.);
#59560=ORIENTED_EDGE('',*,*,#44310,.F.);
#59561=ORIENTED_EDGE('',*,*,#44304,.F.);
#59562=ORIENTED_EDGE('',*,*,#44263,.T.);
#59563=ORIENTED_EDGE('',*,*,#44317,.T.);
#59564=ORIENTED_EDGE('',*,*,#44315,.T.);
#59565=ORIENTED_EDGE('',*,*,#44308,.F.);
#59566=ORIENTED_EDGE('',*,*,#44318,.T.);
#59567=ORIENTED_EDGE('',*,*,#44319,.T.);
#59568=ORIENTED_EDGE('',*,*,#44265,.T.);
#59569=ORIENTED_EDGE('',*,*,#44278,.F.);
#59570=ORIENTED_EDGE('',*,*,#44320,.F.);
#59571=ORIENTED_EDGE('',*,*,#44321,.T.);
#59572=ORIENTED_EDGE('',*,*,#44318,.F.);
#59573=ORIENTED_EDGE('',*,*,#44276,.F.);
#59574=ORIENTED_EDGE('',*,*,#44309,.F.);
#59575=ORIENTED_EDGE('',*,*,#44307,.F.);
#59576=ORIENTED_EDGE('',*,*,#44305,.F.);
#59577=ORIENTED_EDGE('',*,*,#44302,.F.);
#59578=ORIENTED_EDGE('',*,*,#44299,.F.);
#59579=ORIENTED_EDGE('',*,*,#44296,.F.);
#59580=ORIENTED_EDGE('',*,*,#44293,.F.);
#59581=ORIENTED_EDGE('',*,*,#44290,.F.);
#59582=ORIENTED_EDGE('',*,*,#44287,.F.);
#59583=ORIENTED_EDGE('',*,*,#44284,.F.);
#59584=ORIENTED_EDGE('',*,*,#44281,.F.);
#59585=ORIENTED_EDGE('',*,*,#44322,.T.);
#59586=ORIENTED_EDGE('',*,*,#44323,.T.);
#59587=ORIENTED_EDGE('',*,*,#44324,.T.);
#59588=ORIENTED_EDGE('',*,*,#44325,.T.);
#59589=ORIENTED_EDGE('',*,*,#44326,.T.);
#59590=ORIENTED_EDGE('',*,*,#44327,.T.);
#59591=ORIENTED_EDGE('',*,*,#44324,.F.);
#59592=ORIENTED_EDGE('',*,*,#44328,.T.);
#59593=ORIENTED_EDGE('',*,*,#44329,.T.);
#59594=ORIENTED_EDGE('',*,*,#44330,.T.);
#59595=ORIENTED_EDGE('',*,*,#44326,.F.);
#59596=ORIENTED_EDGE('',*,*,#44331,.T.);
#59597=ORIENTED_EDGE('',*,*,#44332,.T.);
#59598=ORIENTED_EDGE('',*,*,#44333,.T.);
#59599=ORIENTED_EDGE('',*,*,#44329,.F.);
#59600=ORIENTED_EDGE('',*,*,#44334,.T.);
#59601=ORIENTED_EDGE('',*,*,#44335,.T.);
#59602=ORIENTED_EDGE('',*,*,#44336,.T.);
#59603=ORIENTED_EDGE('',*,*,#44332,.F.);
#59604=ORIENTED_EDGE('',*,*,#44337,.T.);
#59605=ORIENTED_EDGE('',*,*,#44338,.T.);
#59606=ORIENTED_EDGE('',*,*,#44339,.T.);
#59607=ORIENTED_EDGE('',*,*,#44335,.F.);
#59608=ORIENTED_EDGE('',*,*,#44340,.T.);
#59609=ORIENTED_EDGE('',*,*,#44341,.T.);
#59610=ORIENTED_EDGE('',*,*,#44342,.T.);
#59611=ORIENTED_EDGE('',*,*,#44338,.F.);
#59612=ORIENTED_EDGE('',*,*,#44343,.T.);
#59613=ORIENTED_EDGE('',*,*,#44344,.T.);
#59614=ORIENTED_EDGE('',*,*,#44345,.T.);
#59615=ORIENTED_EDGE('',*,*,#44341,.F.);
#59616=ORIENTED_EDGE('',*,*,#44346,.T.);
#59617=ORIENTED_EDGE('',*,*,#44347,.T.);
#59618=ORIENTED_EDGE('',*,*,#44348,.T.);
#59619=ORIENTED_EDGE('',*,*,#44344,.F.);
#59620=ORIENTED_EDGE('',*,*,#44349,.T.);
#59621=ORIENTED_EDGE('',*,*,#44350,.T.);
#59622=ORIENTED_EDGE('',*,*,#44351,.T.);
#59623=ORIENTED_EDGE('',*,*,#44347,.F.);
#59624=ORIENTED_EDGE('',*,*,#44352,.T.);
#59625=ORIENTED_EDGE('',*,*,#44322,.F.);
#59626=ORIENTED_EDGE('',*,*,#44353,.T.);
#59627=ORIENTED_EDGE('',*,*,#44350,.F.);
#59628=ORIENTED_EDGE('',*,*,#44354,.T.);
#59629=ORIENTED_EDGE('',*,*,#44342,.F.);
#59630=ORIENTED_EDGE('',*,*,#44355,.F.);
#59631=ORIENTED_EDGE('',*,*,#44356,.F.);
#59632=ORIENTED_EDGE('',*,*,#44357,.T.);
#59633=ORIENTED_EDGE('',*,*,#44358,.T.);
#59634=ORIENTED_EDGE('',*,*,#44359,.T.);
#59635=ORIENTED_EDGE('',*,*,#44345,.F.);
#59636=ORIENTED_EDGE('',*,*,#44360,.F.);
#59637=ORIENTED_EDGE('',*,*,#44361,.F.);
#59638=ORIENTED_EDGE('',*,*,#44355,.T.);
#59639=ORIENTED_EDGE('',*,*,#44348,.F.);
#59640=ORIENTED_EDGE('',*,*,#44362,.T.);
#59641=ORIENTED_EDGE('',*,*,#44363,.T.);
#59642=ORIENTED_EDGE('',*,*,#44360,.T.);
#59643=ORIENTED_EDGE('',*,*,#44351,.F.);
#59644=ORIENTED_EDGE('',*,*,#44364,.F.);
#59645=ORIENTED_EDGE('',*,*,#44365,.F.);
#59646=ORIENTED_EDGE('',*,*,#44362,.F.);
#59647=ORIENTED_EDGE('',*,*,#44353,.F.);
#59648=ORIENTED_EDGE('',*,*,#44366,.T.);
#59649=ORIENTED_EDGE('',*,*,#44367,.T.);
#59650=ORIENTED_EDGE('',*,*,#44364,.T.);
#59651=ORIENTED_EDGE('',*,*,#44325,.F.);
#59652=ORIENTED_EDGE('',*,*,#44368,.F.);
#59653=ORIENTED_EDGE('',*,*,#44369,.T.);
#59654=ORIENTED_EDGE('',*,*,#44370,.F.);
#59655=ORIENTED_EDGE('',*,*,#44371,.F.);
#59656=ORIENTED_EDGE('',*,*,#44366,.F.);
#59657=ORIENTED_EDGE('',*,*,#44323,.F.);
#59658=ORIENTED_EDGE('',*,*,#44354,.F.);
#59659=ORIENTED_EDGE('',*,*,#44352,.F.);
#59660=ORIENTED_EDGE('',*,*,#44349,.F.);
#59661=ORIENTED_EDGE('',*,*,#44346,.F.);
#59662=ORIENTED_EDGE('',*,*,#44343,.F.);
#59663=ORIENTED_EDGE('',*,*,#44340,.F.);
#59664=ORIENTED_EDGE('',*,*,#44337,.F.);
#59665=ORIENTED_EDGE('',*,*,#44334,.F.);
#59666=ORIENTED_EDGE('',*,*,#44331,.F.);
#59667=ORIENTED_EDGE('',*,*,#44328,.F.);
#59668=ORIENTED_EDGE('',*,*,#44372,.T.);
#59669=ORIENTED_EDGE('',*,*,#44373,.T.);
#59670=ORIENTED_EDGE('',*,*,#44374,.T.);
#59671=ORIENTED_EDGE('',*,*,#44375,.T.);
#59672=ORIENTED_EDGE('',*,*,#44376,.T.);
#59673=ORIENTED_EDGE('',*,*,#44377,.T.);
#59674=ORIENTED_EDGE('',*,*,#44374,.F.);
#59675=ORIENTED_EDGE('',*,*,#44378,.T.);
#59676=ORIENTED_EDGE('',*,*,#44379,.T.);
#59677=ORIENTED_EDGE('',*,*,#44380,.T.);
#59678=ORIENTED_EDGE('',*,*,#44376,.F.);
#59679=ORIENTED_EDGE('',*,*,#44381,.T.);
#59680=ORIENTED_EDGE('',*,*,#44382,.T.);
#59681=ORIENTED_EDGE('',*,*,#44383,.T.);
#59682=ORIENTED_EDGE('',*,*,#44379,.F.);
#59683=ORIENTED_EDGE('',*,*,#44384,.T.);
#59684=ORIENTED_EDGE('',*,*,#44385,.T.);
#59685=ORIENTED_EDGE('',*,*,#44386,.T.);
#59686=ORIENTED_EDGE('',*,*,#44382,.F.);
#59687=ORIENTED_EDGE('',*,*,#44387,.T.);
#59688=ORIENTED_EDGE('',*,*,#44388,.T.);
#59689=ORIENTED_EDGE('',*,*,#44389,.T.);
#59690=ORIENTED_EDGE('',*,*,#44385,.F.);
#59691=ORIENTED_EDGE('',*,*,#44390,.T.);
#59692=ORIENTED_EDGE('',*,*,#44391,.T.);
#59693=ORIENTED_EDGE('',*,*,#44392,.T.);
#59694=ORIENTED_EDGE('',*,*,#44388,.F.);
#59695=ORIENTED_EDGE('',*,*,#44393,.T.);
#59696=ORIENTED_EDGE('',*,*,#44394,.T.);
#59697=ORIENTED_EDGE('',*,*,#44395,.T.);
#59698=ORIENTED_EDGE('',*,*,#44391,.F.);
#59699=ORIENTED_EDGE('',*,*,#44396,.T.);
#59700=ORIENTED_EDGE('',*,*,#44397,.T.);
#59701=ORIENTED_EDGE('',*,*,#44398,.T.);
#59702=ORIENTED_EDGE('',*,*,#44394,.F.);
#59703=ORIENTED_EDGE('',*,*,#44399,.T.);
#59704=ORIENTED_EDGE('',*,*,#44400,.T.);
#59705=ORIENTED_EDGE('',*,*,#44401,.T.);
#59706=ORIENTED_EDGE('',*,*,#44397,.F.);
#59707=ORIENTED_EDGE('',*,*,#44402,.T.);
#59708=ORIENTED_EDGE('',*,*,#44403,.T.);
#59709=ORIENTED_EDGE('',*,*,#44404,.T.);
#59710=ORIENTED_EDGE('',*,*,#44400,.F.);
#59711=ORIENTED_EDGE('',*,*,#44405,.T.);
#59712=ORIENTED_EDGE('',*,*,#44406,.T.);
#59713=ORIENTED_EDGE('',*,*,#44407,.T.);
#59714=ORIENTED_EDGE('',*,*,#44403,.F.);
#59715=ORIENTED_EDGE('',*,*,#44408,.T.);
#59716=ORIENTED_EDGE('',*,*,#44409,.T.);
#59717=ORIENTED_EDGE('',*,*,#44410,.T.);
#59718=ORIENTED_EDGE('',*,*,#44406,.F.);
#59719=ORIENTED_EDGE('',*,*,#44411,.T.);
#59720=ORIENTED_EDGE('',*,*,#44372,.F.);
#59721=ORIENTED_EDGE('',*,*,#44412,.T.);
#59722=ORIENTED_EDGE('',*,*,#44409,.F.);
#59723=ORIENTED_EDGE('',*,*,#44413,.T.);
#59724=ORIENTED_EDGE('',*,*,#44398,.F.);
#59725=ORIENTED_EDGE('',*,*,#44414,.T.);
#59726=ORIENTED_EDGE('',*,*,#44415,.T.);
#59727=ORIENTED_EDGE('',*,*,#44416,.T.);
#59728=ORIENTED_EDGE('',*,*,#44401,.F.);
#59729=ORIENTED_EDGE('',*,*,#44417,.F.);
#59730=ORIENTED_EDGE('',*,*,#44418,.F.);
#59731=ORIENTED_EDGE('',*,*,#44414,.F.);
#59732=ORIENTED_EDGE('',*,*,#44404,.F.);
#59733=ORIENTED_EDGE('',*,*,#44419,.T.);
#59734=ORIENTED_EDGE('',*,*,#44420,.T.);
#59735=ORIENTED_EDGE('',*,*,#44417,.T.);
#59736=ORIENTED_EDGE('',*,*,#44407,.F.);
#59737=ORIENTED_EDGE('',*,*,#44421,.F.);
#59738=ORIENTED_EDGE('',*,*,#44422,.F.);
#59739=ORIENTED_EDGE('',*,*,#44419,.F.);
#59740=ORIENTED_EDGE('',*,*,#44410,.F.);
#59741=ORIENTED_EDGE('',*,*,#44423,.T.);
#59742=ORIENTED_EDGE('',*,*,#44424,.T.);
#59743=ORIENTED_EDGE('',*,*,#44421,.T.);
#59744=ORIENTED_EDGE('',*,*,#44412,.F.);
#59745=ORIENTED_EDGE('',*,*,#44425,.F.);
#59746=ORIENTED_EDGE('',*,*,#44426,.T.);
#59747=ORIENTED_EDGE('',*,*,#44423,.F.);
#59748=ORIENTED_EDGE('',*,*,#44375,.F.);
#59749=ORIENTED_EDGE('',*,*,#44427,.F.);
#59750=ORIENTED_EDGE('',*,*,#44428,.T.);
#59751=ORIENTED_EDGE('',*,*,#44425,.T.);
#59752=ORIENTED_EDGE('',*,*,#44373,.F.);
#59753=ORIENTED_EDGE('',*,*,#44413,.F.);
#59754=ORIENTED_EDGE('',*,*,#44411,.F.);
#59755=ORIENTED_EDGE('',*,*,#44408,.F.);
#59756=ORIENTED_EDGE('',*,*,#44405,.F.);
#59757=ORIENTED_EDGE('',*,*,#44402,.F.);
#59758=ORIENTED_EDGE('',*,*,#44399,.F.);
#59759=ORIENTED_EDGE('',*,*,#44396,.F.);
#59760=ORIENTED_EDGE('',*,*,#44393,.F.);
#59761=ORIENTED_EDGE('',*,*,#44390,.F.);
#59762=ORIENTED_EDGE('',*,*,#44387,.F.);
#59763=ORIENTED_EDGE('',*,*,#44384,.F.);
#59764=ORIENTED_EDGE('',*,*,#44381,.F.);
#59765=ORIENTED_EDGE('',*,*,#44378,.F.);
#59766=ORIENTED_EDGE('',*,*,#44429,.T.);
#59767=ORIENTED_EDGE('',*,*,#44430,.T.);
#59768=ORIENTED_EDGE('',*,*,#44431,.T.);
#59769=ORIENTED_EDGE('',*,*,#44432,.T.);
#59770=ORIENTED_EDGE('',*,*,#44433,.T.);
#59771=ORIENTED_EDGE('',*,*,#44434,.T.);
#59772=ORIENTED_EDGE('',*,*,#44431,.F.);
#59773=ORIENTED_EDGE('',*,*,#44435,.T.);
#59774=ORIENTED_EDGE('',*,*,#44436,.T.);
#59775=ORIENTED_EDGE('',*,*,#44437,.T.);
#59776=ORIENTED_EDGE('',*,*,#44433,.F.);
#59777=ORIENTED_EDGE('',*,*,#44438,.T.);
#59778=ORIENTED_EDGE('',*,*,#44439,.T.);
#59779=ORIENTED_EDGE('',*,*,#44440,.T.);
#59780=ORIENTED_EDGE('',*,*,#44436,.F.);
#59781=ORIENTED_EDGE('',*,*,#44441,.T.);
#59782=ORIENTED_EDGE('',*,*,#44442,.T.);
#59783=ORIENTED_EDGE('',*,*,#44443,.T.);
#59784=ORIENTED_EDGE('',*,*,#44439,.F.);
#59785=ORIENTED_EDGE('',*,*,#44444,.T.);
#59786=ORIENTED_EDGE('',*,*,#44445,.T.);
#59787=ORIENTED_EDGE('',*,*,#44446,.T.);
#59788=ORIENTED_EDGE('',*,*,#44442,.F.);
#59789=ORIENTED_EDGE('',*,*,#44447,.T.);
#59790=ORIENTED_EDGE('',*,*,#44448,.T.);
#59791=ORIENTED_EDGE('',*,*,#44449,.T.);
#59792=ORIENTED_EDGE('',*,*,#44445,.F.);
#59793=ORIENTED_EDGE('',*,*,#44450,.T.);
#59794=ORIENTED_EDGE('',*,*,#44451,.T.);
#59795=ORIENTED_EDGE('',*,*,#44452,.T.);
#59796=ORIENTED_EDGE('',*,*,#44448,.F.);
#59797=ORIENTED_EDGE('',*,*,#44453,.T.);
#59798=ORIENTED_EDGE('',*,*,#44429,.F.);
#59799=ORIENTED_EDGE('',*,*,#44454,.T.);
#59800=ORIENTED_EDGE('',*,*,#44451,.F.);
#59801=ORIENTED_EDGE('',*,*,#44455,.T.);
#59802=ORIENTED_EDGE('',*,*,#44446,.F.);
#59803=ORIENTED_EDGE('',*,*,#44456,.F.);
#59804=ORIENTED_EDGE('',*,*,#44457,.T.);
#59805=ORIENTED_EDGE('',*,*,#44458,.F.);
#59806=ORIENTED_EDGE('',*,*,#44449,.F.);
#59807=ORIENTED_EDGE('',*,*,#44459,.T.);
#59808=ORIENTED_EDGE('',*,*,#44460,.T.);
#59809=ORIENTED_EDGE('',*,*,#44456,.T.);
#59810=ORIENTED_EDGE('',*,*,#44452,.F.);
#59811=ORIENTED_EDGE('',*,*,#44461,.F.);
#59812=ORIENTED_EDGE('',*,*,#44462,.F.);
#59813=ORIENTED_EDGE('',*,*,#44459,.F.);
#59814=ORIENTED_EDGE('',*,*,#44454,.F.);
#59815=ORIENTED_EDGE('',*,*,#44463,.T.);
#59816=ORIENTED_EDGE('',*,*,#44464,.F.);
#59817=ORIENTED_EDGE('',*,*,#44461,.T.);
#59818=ORIENTED_EDGE('',*,*,#44432,.F.);
#59819=ORIENTED_EDGE('',*,*,#44465,.F.);
#59820=ORIENTED_EDGE('',*,*,#44466,.F.);
#59821=ORIENTED_EDGE('',*,*,#44463,.F.);
#59822=ORIENTED_EDGE('',*,*,#44430,.F.);
#59823=ORIENTED_EDGE('',*,*,#44455,.F.);
#59824=ORIENTED_EDGE('',*,*,#44453,.F.);
#59825=ORIENTED_EDGE('',*,*,#44450,.F.);
#59826=ORIENTED_EDGE('',*,*,#44447,.F.);
#59827=ORIENTED_EDGE('',*,*,#44444,.F.);
#59828=ORIENTED_EDGE('',*,*,#44441,.F.);
#59829=ORIENTED_EDGE('',*,*,#44438,.F.);
#59830=ORIENTED_EDGE('',*,*,#44435,.F.);
#59831=ORIENTED_EDGE('',*,*,#44467,.T.);
#59832=ORIENTED_EDGE('',*,*,#44468,.T.);
#59833=ORIENTED_EDGE('',*,*,#44469,.T.);
#59834=ORIENTED_EDGE('',*,*,#44470,.T.);
#59835=ORIENTED_EDGE('',*,*,#44471,.T.);
#59836=ORIENTED_EDGE('',*,*,#44472,.T.);
#59837=ORIENTED_EDGE('',*,*,#44469,.F.);
#59838=ORIENTED_EDGE('',*,*,#44473,.T.);
#59839=ORIENTED_EDGE('',*,*,#44474,.T.);
#59840=ORIENTED_EDGE('',*,*,#44475,.T.);
#59841=ORIENTED_EDGE('',*,*,#44471,.F.);
#59842=ORIENTED_EDGE('',*,*,#44476,.T.);
#59843=ORIENTED_EDGE('',*,*,#44477,.T.);
#59844=ORIENTED_EDGE('',*,*,#44478,.T.);
#59845=ORIENTED_EDGE('',*,*,#44474,.F.);
#59846=ORIENTED_EDGE('',*,*,#44479,.T.);
#59847=ORIENTED_EDGE('',*,*,#44480,.T.);
#59848=ORIENTED_EDGE('',*,*,#44481,.T.);
#59849=ORIENTED_EDGE('',*,*,#44477,.F.);
#59850=ORIENTED_EDGE('',*,*,#44482,.T.);
#59851=ORIENTED_EDGE('',*,*,#44483,.T.);
#59852=ORIENTED_EDGE('',*,*,#44484,.T.);
#59853=ORIENTED_EDGE('',*,*,#44480,.F.);
#59854=ORIENTED_EDGE('',*,*,#44485,.T.);
#59855=ORIENTED_EDGE('',*,*,#44486,.T.);
#59856=ORIENTED_EDGE('',*,*,#44487,.T.);
#59857=ORIENTED_EDGE('',*,*,#44483,.F.);
#59858=ORIENTED_EDGE('',*,*,#44488,.T.);
#59859=ORIENTED_EDGE('',*,*,#44489,.T.);
#59860=ORIENTED_EDGE('',*,*,#44490,.T.);
#59861=ORIENTED_EDGE('',*,*,#44486,.F.);
#59862=ORIENTED_EDGE('',*,*,#44491,.T.);
#59863=ORIENTED_EDGE('',*,*,#44492,.T.);
#59864=ORIENTED_EDGE('',*,*,#44493,.T.);
#59865=ORIENTED_EDGE('',*,*,#44489,.F.);
#59866=ORIENTED_EDGE('',*,*,#44494,.T.);
#59867=ORIENTED_EDGE('',*,*,#44495,.T.);
#59868=ORIENTED_EDGE('',*,*,#44496,.T.);
#59869=ORIENTED_EDGE('',*,*,#44492,.F.);
#59870=ORIENTED_EDGE('',*,*,#44497,.T.);
#59871=ORIENTED_EDGE('',*,*,#44498,.T.);
#59872=ORIENTED_EDGE('',*,*,#44499,.T.);
#59873=ORIENTED_EDGE('',*,*,#44495,.F.);
#59874=ORIENTED_EDGE('',*,*,#44500,.T.);
#59875=ORIENTED_EDGE('',*,*,#44501,.T.);
#59876=ORIENTED_EDGE('',*,*,#44502,.T.);
#59877=ORIENTED_EDGE('',*,*,#44498,.F.);
#59878=ORIENTED_EDGE('',*,*,#44503,.T.);
#59879=ORIENTED_EDGE('',*,*,#44504,.T.);
#59880=ORIENTED_EDGE('',*,*,#44505,.T.);
#59881=ORIENTED_EDGE('',*,*,#44501,.F.);
#59882=ORIENTED_EDGE('',*,*,#44506,.T.);
#59883=ORIENTED_EDGE('',*,*,#44507,.T.);
#59884=ORIENTED_EDGE('',*,*,#44508,.T.);
#59885=ORIENTED_EDGE('',*,*,#44504,.F.);
#59886=ORIENTED_EDGE('',*,*,#44509,.T.);
#59887=ORIENTED_EDGE('',*,*,#44510,.T.);
#59888=ORIENTED_EDGE('',*,*,#44511,.T.);
#59889=ORIENTED_EDGE('',*,*,#44507,.F.);
#59890=ORIENTED_EDGE('',*,*,#44512,.T.);
#59891=ORIENTED_EDGE('',*,*,#44467,.F.);
#59892=ORIENTED_EDGE('',*,*,#44513,.T.);
#59893=ORIENTED_EDGE('',*,*,#44510,.F.);
#59894=ORIENTED_EDGE('',*,*,#44514,.T.);
#59895=ORIENTED_EDGE('',*,*,#44496,.F.);
#59896=ORIENTED_EDGE('',*,*,#44515,.T.);
#59897=ORIENTED_EDGE('',*,*,#44516,.T.);
#59898=ORIENTED_EDGE('',*,*,#44517,.T.);
#59899=ORIENTED_EDGE('',*,*,#44499,.F.);
#59900=ORIENTED_EDGE('',*,*,#44518,.F.);
#59901=ORIENTED_EDGE('',*,*,#44519,.F.);
#59902=ORIENTED_EDGE('',*,*,#44515,.F.);
#59903=ORIENTED_EDGE('',*,*,#44502,.F.);
#59904=ORIENTED_EDGE('',*,*,#44520,.T.);
#59905=ORIENTED_EDGE('',*,*,#44521,.T.);
#59906=ORIENTED_EDGE('',*,*,#44518,.T.);
#59907=ORIENTED_EDGE('',*,*,#44505,.F.);
#59908=ORIENTED_EDGE('',*,*,#44522,.F.);
#59909=ORIENTED_EDGE('',*,*,#44523,.F.);
#59910=ORIENTED_EDGE('',*,*,#44520,.F.);
#59911=ORIENTED_EDGE('',*,*,#44508,.F.);
#59912=ORIENTED_EDGE('',*,*,#44524,.T.);
#59913=ORIENTED_EDGE('',*,*,#44525,.T.);
#59914=ORIENTED_EDGE('',*,*,#44522,.T.);
#59915=ORIENTED_EDGE('',*,*,#44511,.F.);
#59916=ORIENTED_EDGE('',*,*,#44526,.F.);
#59917=ORIENTED_EDGE('',*,*,#44527,.T.);
#59918=ORIENTED_EDGE('',*,*,#44524,.F.);
#59919=ORIENTED_EDGE('',*,*,#44513,.F.);
#59920=ORIENTED_EDGE('',*,*,#44528,.T.);
#59921=ORIENTED_EDGE('',*,*,#44529,.T.);
#59922=ORIENTED_EDGE('',*,*,#44526,.T.);
#59923=ORIENTED_EDGE('',*,*,#44470,.F.);
#59924=ORIENTED_EDGE('',*,*,#44530,.F.);
#59925=ORIENTED_EDGE('',*,*,#44531,.F.);
#59926=ORIENTED_EDGE('',*,*,#44532,.F.);
#59927=ORIENTED_EDGE('',*,*,#44533,.T.);
#59928=ORIENTED_EDGE('',*,*,#44528,.F.);
#59929=ORIENTED_EDGE('',*,*,#44468,.F.);
#59930=ORIENTED_EDGE('',*,*,#44514,.F.);
#59931=ORIENTED_EDGE('',*,*,#44512,.F.);
#59932=ORIENTED_EDGE('',*,*,#44509,.F.);
#59933=ORIENTED_EDGE('',*,*,#44506,.F.);
#59934=ORIENTED_EDGE('',*,*,#44503,.F.);
#59935=ORIENTED_EDGE('',*,*,#44500,.F.);
#59936=ORIENTED_EDGE('',*,*,#44497,.F.);
#59937=ORIENTED_EDGE('',*,*,#44494,.F.);
#59938=ORIENTED_EDGE('',*,*,#44491,.F.);
#59939=ORIENTED_EDGE('',*,*,#44488,.F.);
#59940=ORIENTED_EDGE('',*,*,#44485,.F.);
#59941=ORIENTED_EDGE('',*,*,#44482,.F.);
#59942=ORIENTED_EDGE('',*,*,#44479,.F.);
#59943=ORIENTED_EDGE('',*,*,#44476,.F.);
#59944=ORIENTED_EDGE('',*,*,#44473,.F.);
#59945=ORIENTED_EDGE('',*,*,#44534,.T.);
#59946=ORIENTED_EDGE('',*,*,#44535,.T.);
#59947=ORIENTED_EDGE('',*,*,#44536,.T.);
#59948=ORIENTED_EDGE('',*,*,#44537,.T.);
#59949=ORIENTED_EDGE('',*,*,#44538,.T.);
#59950=ORIENTED_EDGE('',*,*,#44539,.T.);
#59951=ORIENTED_EDGE('',*,*,#44536,.F.);
#59952=ORIENTED_EDGE('',*,*,#44540,.T.);
#59953=ORIENTED_EDGE('',*,*,#44541,.T.);
#59954=ORIENTED_EDGE('',*,*,#44542,.T.);
#59955=ORIENTED_EDGE('',*,*,#44538,.F.);
#59956=ORIENTED_EDGE('',*,*,#44543,.T.);
#59957=ORIENTED_EDGE('',*,*,#44544,.T.);
#59958=ORIENTED_EDGE('',*,*,#44545,.T.);
#59959=ORIENTED_EDGE('',*,*,#44541,.F.);
#59960=ORIENTED_EDGE('',*,*,#44546,.T.);
#59961=ORIENTED_EDGE('',*,*,#44547,.T.);
#59962=ORIENTED_EDGE('',*,*,#44548,.T.);
#59963=ORIENTED_EDGE('',*,*,#44544,.F.);
#59964=ORIENTED_EDGE('',*,*,#44549,.T.);
#59965=ORIENTED_EDGE('',*,*,#44550,.T.);
#59966=ORIENTED_EDGE('',*,*,#44551,.T.);
#59967=ORIENTED_EDGE('',*,*,#44547,.F.);
#59968=ORIENTED_EDGE('',*,*,#44552,.T.);
#59969=ORIENTED_EDGE('',*,*,#44553,.T.);
#59970=ORIENTED_EDGE('',*,*,#44554,.T.);
#59971=ORIENTED_EDGE('',*,*,#44550,.F.);
#59972=ORIENTED_EDGE('',*,*,#44555,.T.);
#59973=ORIENTED_EDGE('',*,*,#44556,.T.);
#59974=ORIENTED_EDGE('',*,*,#44557,.T.);
#59975=ORIENTED_EDGE('',*,*,#44553,.F.);
#59976=ORIENTED_EDGE('',*,*,#44558,.T.);
#59977=ORIENTED_EDGE('',*,*,#44534,.F.);
#59978=ORIENTED_EDGE('',*,*,#44559,.T.);
#59979=ORIENTED_EDGE('',*,*,#44556,.F.);
#59980=ORIENTED_EDGE('',*,*,#44560,.T.);
#59981=ORIENTED_EDGE('',*,*,#44551,.F.);
#59982=ORIENTED_EDGE('',*,*,#44561,.F.);
#59983=ORIENTED_EDGE('',*,*,#44562,.F.);
#59984=ORIENTED_EDGE('',*,*,#44563,.F.);
#59985=ORIENTED_EDGE('',*,*,#44564,.F.);
#59986=ORIENTED_EDGE('',*,*,#44565,.F.);
#59987=ORIENTED_EDGE('',*,*,#44566,.F.);
#59988=ORIENTED_EDGE('',*,*,#44567,.F.);
#59989=ORIENTED_EDGE('',*,*,#44554,.F.);
#59990=ORIENTED_EDGE('',*,*,#44568,.T.);
#59991=ORIENTED_EDGE('',*,*,#44569,.T.);
#59992=ORIENTED_EDGE('',*,*,#44561,.T.);
#59993=ORIENTED_EDGE('',*,*,#44557,.F.);
#59994=ORIENTED_EDGE('',*,*,#44570,.F.);
#59995=ORIENTED_EDGE('',*,*,#44571,.F.);
#59996=ORIENTED_EDGE('',*,*,#44568,.F.);
#59997=ORIENTED_EDGE('',*,*,#44559,.F.);
#59998=ORIENTED_EDGE('',*,*,#44572,.T.);
#59999=ORIENTED_EDGE('',*,*,#44573,.T.);
#60000=ORIENTED_EDGE('',*,*,#44570,.T.);
#60001=ORIENTED_EDGE('',*,*,#44537,.F.);
#60002=ORIENTED_EDGE('',*,*,#44574,.F.);
#60003=ORIENTED_EDGE('',*,*,#44575,.F.);
#60004=ORIENTED_EDGE('',*,*,#44572,.F.);
#60005=ORIENTED_EDGE('',*,*,#44535,.F.);
#60006=ORIENTED_EDGE('',*,*,#44560,.F.);
#60007=ORIENTED_EDGE('',*,*,#44558,.F.);
#60008=ORIENTED_EDGE('',*,*,#44555,.F.);
#60009=ORIENTED_EDGE('',*,*,#44552,.F.);
#60010=ORIENTED_EDGE('',*,*,#44549,.F.);
#60011=ORIENTED_EDGE('',*,*,#44546,.F.);
#60012=ORIENTED_EDGE('',*,*,#44543,.F.);
#60013=ORIENTED_EDGE('',*,*,#44540,.F.);
#60014=ORIENTED_EDGE('',*,*,#44576,.T.);
#60015=ORIENTED_EDGE('',*,*,#44577,.T.);
#60016=ORIENTED_EDGE('',*,*,#44578,.T.);
#60017=ORIENTED_EDGE('',*,*,#44579,.T.);
#60018=ORIENTED_EDGE('',*,*,#44580,.T.);
#60019=ORIENTED_EDGE('',*,*,#44581,.T.);
#60020=ORIENTED_EDGE('',*,*,#44578,.F.);
#60021=ORIENTED_EDGE('',*,*,#44582,.T.);
#60022=ORIENTED_EDGE('',*,*,#44583,.T.);
#60023=ORIENTED_EDGE('',*,*,#44584,.T.);
#60024=ORIENTED_EDGE('',*,*,#44580,.F.);
#60025=ORIENTED_EDGE('',*,*,#44585,.T.);
#60026=ORIENTED_EDGE('',*,*,#44586,.T.);
#60027=ORIENTED_EDGE('',*,*,#44587,.T.);
#60028=ORIENTED_EDGE('',*,*,#44583,.F.);
#60029=ORIENTED_EDGE('',*,*,#44588,.T.);
#60030=ORIENTED_EDGE('',*,*,#44589,.T.);
#60031=ORIENTED_EDGE('',*,*,#44590,.T.);
#60032=ORIENTED_EDGE('',*,*,#44586,.F.);
#60033=ORIENTED_EDGE('',*,*,#44591,.T.);
#60034=ORIENTED_EDGE('',*,*,#44592,.T.);
#60035=ORIENTED_EDGE('',*,*,#44593,.T.);
#60036=ORIENTED_EDGE('',*,*,#44589,.F.);
#60037=ORIENTED_EDGE('',*,*,#44594,.T.);
#60038=ORIENTED_EDGE('',*,*,#44595,.T.);
#60039=ORIENTED_EDGE('',*,*,#44596,.T.);
#60040=ORIENTED_EDGE('',*,*,#44592,.F.);
#60041=ORIENTED_EDGE('',*,*,#44597,.T.);
#60042=ORIENTED_EDGE('',*,*,#44576,.F.);
#60043=ORIENTED_EDGE('',*,*,#44598,.T.);
#60044=ORIENTED_EDGE('',*,*,#44595,.F.);
#60045=ORIENTED_EDGE('',*,*,#44599,.T.);
#60046=ORIENTED_EDGE('',*,*,#44593,.F.);
#60047=ORIENTED_EDGE('',*,*,#44600,.T.);
#60048=ORIENTED_EDGE('',*,*,#44601,.T.);
#60049=ORIENTED_EDGE('',*,*,#44602,.T.);
#60050=ORIENTED_EDGE('',*,*,#44596,.F.);
#60051=ORIENTED_EDGE('',*,*,#44603,.F.);
#60052=ORIENTED_EDGE('',*,*,#44604,.F.);
#60053=ORIENTED_EDGE('',*,*,#44600,.F.);
#60054=ORIENTED_EDGE('',*,*,#44598,.F.);
#60055=ORIENTED_EDGE('',*,*,#44605,.T.);
#60056=ORIENTED_EDGE('',*,*,#44606,.T.);
#60057=ORIENTED_EDGE('',*,*,#44603,.T.);
#60058=ORIENTED_EDGE('',*,*,#44579,.F.);
#60059=ORIENTED_EDGE('',*,*,#44607,.F.);
#60060=ORIENTED_EDGE('',*,*,#44608,.F.);
#60061=ORIENTED_EDGE('',*,*,#44605,.F.);
#60062=ORIENTED_EDGE('',*,*,#44577,.F.);
#60063=ORIENTED_EDGE('',*,*,#44599,.F.);
#60064=ORIENTED_EDGE('',*,*,#44597,.F.);
#60065=ORIENTED_EDGE('',*,*,#44594,.F.);
#60066=ORIENTED_EDGE('',*,*,#44591,.F.);
#60067=ORIENTED_EDGE('',*,*,#44588,.F.);
#60068=ORIENTED_EDGE('',*,*,#44585,.F.);
#60069=ORIENTED_EDGE('',*,*,#44582,.F.);
#60070=ORIENTED_EDGE('',*,*,#44609,.T.);
#60071=ORIENTED_EDGE('',*,*,#44610,.T.);
#60072=ORIENTED_EDGE('',*,*,#44611,.T.);
#60073=ORIENTED_EDGE('',*,*,#44612,.T.);
#60074=ORIENTED_EDGE('',*,*,#44613,.T.);
#60075=ORIENTED_EDGE('',*,*,#44614,.T.);
#60076=ORIENTED_EDGE('',*,*,#44611,.F.);
#60077=ORIENTED_EDGE('',*,*,#44615,.T.);
#60078=ORIENTED_EDGE('',*,*,#44616,.T.);
#60079=ORIENTED_EDGE('',*,*,#44617,.T.);
#60080=ORIENTED_EDGE('',*,*,#44613,.F.);
#60081=ORIENTED_EDGE('',*,*,#44195,.T.);
#60082=ORIENTED_EDGE('',*,*,#44615,.F.);
#60083=ORIENTED_EDGE('',*,*,#44618,.T.);
#60084=ORIENTED_EDGE('',*,*,#44619,.T.);
#60085=ORIENTED_EDGE('',*,*,#44196,.T.);
#60086=ORIENTED_EDGE('',*,*,#44610,.F.);
#60087=ORIENTED_EDGE('',*,*,#44620,.F.);
#60088=ORIENTED_EDGE('',*,*,#44621,.T.);
#60089=ORIENTED_EDGE('',*,*,#44622,.F.);
#60090=ORIENTED_EDGE('',*,*,#44623,.T.);
#60091=ORIENTED_EDGE('',*,*,#44624,.T.);
#60092=ORIENTED_EDGE('',*,*,#44625,.F.);
#60093=ORIENTED_EDGE('',*,*,#44626,.F.);
#60094=ORIENTED_EDGE('',*,*,#44627,.F.);
#60095=ORIENTED_EDGE('',*,*,#44628,.F.);
#60096=ORIENTED_EDGE('',*,*,#44629,.F.);
#60097=ORIENTED_EDGE('',*,*,#44630,.F.);
#60098=ORIENTED_EDGE('',*,*,#44631,.F.);
#60099=ORIENTED_EDGE('',*,*,#44632,.T.);
#60100=ORIENTED_EDGE('',*,*,#44633,.T.);
#60101=ORIENTED_EDGE('',*,*,#44632,.F.);
#60102=ORIENTED_EDGE('',*,*,#44634,.F.);
#60103=ORIENTED_EDGE('',*,*,#44618,.F.);
#60104=ORIENTED_EDGE('',*,*,#44617,.F.);
#60105=ORIENTED_EDGE('',*,*,#44635,.T.);
#60106=ORIENTED_EDGE('',*,*,#44268,.T.);
#60107=ORIENTED_EDGE('',*,*,#44636,.F.);
#60108=ORIENTED_EDGE('',*,*,#44612,.F.);
#60109=ORIENTED_EDGE('',*,*,#44614,.F.);
#60110=ORIENTED_EDGE('',*,*,#44637,.T.);
#60111=ORIENTED_EDGE('',*,*,#44192,.T.);
#60112=ORIENTED_EDGE('',*,*,#44638,.T.);
#60113=ORIENTED_EDGE('',*,*,#44639,.T.);
#60114=ORIENTED_EDGE('',*,*,#44637,.F.);
#60115=ORIENTED_EDGE('',*,*,#44640,.T.);
#60116=ORIENTED_EDGE('',*,*,#44641,.F.);
#60117=ORIENTED_EDGE('',*,*,#44642,.F.);
#60118=ORIENTED_EDGE('',*,*,#44643,.F.);
#60119=ORIENTED_EDGE('',*,*,#44644,.F.);
#60120=ORIENTED_EDGE('',*,*,#44645,.F.);
#60121=ORIENTED_EDGE('',*,*,#44251,.F.);
#60122=ORIENTED_EDGE('',*,*,#44254,.T.);
#60123=ORIENTED_EDGE('',*,*,#44256,.F.);
#60124=ORIENTED_EDGE('',*,*,#44258,.F.);
#60125=ORIENTED_EDGE('',*,*,#44270,.F.);
#60126=ORIENTED_EDGE('',*,*,#44646,.F.);
#60127=ORIENTED_EDGE('',*,*,#44193,.F.);
#60128=ORIENTED_EDGE('',*,*,#44639,.F.);
#60129=ORIENTED_EDGE('',*,*,#44647,.F.);
#60130=ORIENTED_EDGE('',*,*,#44648,.F.);
#60131=ORIENTED_EDGE('',*,*,#44649,.F.);
#60132=ORIENTED_EDGE('',*,*,#44650,.F.);
#60133=ORIENTED_EDGE('',*,*,#44640,.F.);
#60134=ORIENTED_EDGE('',*,*,#44651,.T.);
#60135=ORIENTED_EDGE('',*,*,#44652,.T.);
#60136=ORIENTED_EDGE('',*,*,#44653,.T.);
#60137=ORIENTED_EDGE('',*,*,#44654,.T.);
#60138=ORIENTED_EDGE('',*,*,#44651,.F.);
#60139=ORIENTED_EDGE('',*,*,#44655,.T.);
#60140=ORIENTED_EDGE('',*,*,#44656,.T.);
#60141=ORIENTED_EDGE('',*,*,#44657,.T.);
#60142=ORIENTED_EDGE('',*,*,#44658,.T.);
#60143=ORIENTED_EDGE('',*,*,#44356,.T.);
#60144=ORIENTED_EDGE('',*,*,#44361,.T.);
#60145=ORIENTED_EDGE('',*,*,#44363,.F.);
#60146=ORIENTED_EDGE('',*,*,#44365,.T.);
#60147=ORIENTED_EDGE('',*,*,#44367,.F.);
#60148=ORIENTED_EDGE('',*,*,#44371,.T.);
#60149=ORIENTED_EDGE('',*,*,#44659,.T.);
#60150=ORIENTED_EDGE('',*,*,#44660,.T.);
#60151=ORIENTED_EDGE('',*,*,#44661,.F.);
#60152=ORIENTED_EDGE('',*,*,#44662,.T.);
#60153=ORIENTED_EDGE('',*,*,#44663,.F.);
#60154=ORIENTED_EDGE('',*,*,#44664,.T.);
#60155=ORIENTED_EDGE('',*,*,#44313,.F.);
#60156=ORIENTED_EDGE('',*,*,#44665,.T.);
#60157=ORIENTED_EDGE('',*,*,#44666,.T.);
#60158=ORIENTED_EDGE('',*,*,#44667,.F.);
#60159=ORIENTED_EDGE('',*,*,#44668,.T.);
#60160=ORIENTED_EDGE('',*,*,#44669,.F.);
#60161=ORIENTED_EDGE('',*,*,#44670,.T.);
#60162=ORIENTED_EDGE('',*,*,#44671,.F.);
#60163=ORIENTED_EDGE('',*,*,#44672,.T.);
#60164=ORIENTED_EDGE('',*,*,#44673,.T.);
#60165=ORIENTED_EDGE('',*,*,#44674,.T.);
#60166=ORIENTED_EDGE('',*,*,#44675,.F.);
#60167=ORIENTED_EDGE('',*,*,#44676,.T.);
#60168=ORIENTED_EDGE('',*,*,#44677,.T.);
#60169=ORIENTED_EDGE('',*,*,#44678,.T.);
#60170=ORIENTED_EDGE('',*,*,#44679,.T.);
#60171=ORIENTED_EDGE('',*,*,#44654,.F.);
#60172=ORIENTED_EDGE('',*,*,#44680,.T.);
#60173=ORIENTED_EDGE('',*,*,#44681,.F.);
#60174=ORIENTED_EDGE('',*,*,#44655,.F.);
#60175=ORIENTED_EDGE('',*,*,#44682,.F.);
#60176=ORIENTED_EDGE('',*,*,#44683,.F.);
#60177=ORIENTED_EDGE('',*,*,#44684,.F.);
#60178=ORIENTED_EDGE('',*,*,#44685,.F.);
#60179=ORIENTED_EDGE('',*,*,#44686,.T.);
#60180=ORIENTED_EDGE('',*,*,#44687,.F.);
#60181=ORIENTED_EDGE('',*,*,#44688,.T.);
#60182=ORIENTED_EDGE('',*,*,#44689,.F.);
#60183=ORIENTED_EDGE('',*,*,#44690,.F.);
#60184=ORIENTED_EDGE('',*,*,#44623,.F.);
#60185=ORIENTED_EDGE('',*,*,#44691,.F.);
#60186=ORIENTED_EDGE('',*,*,#44369,.F.);
#60187=ORIENTED_EDGE('',*,*,#44692,.F.);
#60188=ORIENTED_EDGE('',*,*,#44693,.F.);
#60189=ORIENTED_EDGE('',*,*,#44694,.F.);
#60190=ORIENTED_EDGE('',*,*,#44695,.F.);
#60191=ORIENTED_EDGE('',*,*,#44696,.F.);
#60192=ORIENTED_EDGE('',*,*,#44358,.F.);
#60193=ORIENTED_EDGE('',*,*,#44697,.F.);
#60194=ORIENTED_EDGE('',*,*,#44698,.F.);
#60195=ORIENTED_EDGE('',*,*,#44699,.F.);
#60196=ORIENTED_EDGE('',*,*,#44680,.F.);
#60197=ORIENTED_EDGE('',*,*,#44653,.F.);
#60198=ORIENTED_EDGE('',*,*,#44700,.F.);
#60199=ORIENTED_EDGE('',*,*,#44701,.T.);
#60200=ORIENTED_EDGE('',*,*,#44415,.F.);
#60201=ORIENTED_EDGE('',*,*,#44418,.T.);
#60202=ORIENTED_EDGE('',*,*,#44420,.F.);
#60203=ORIENTED_EDGE('',*,*,#44422,.T.);
#60204=ORIENTED_EDGE('',*,*,#44424,.F.);
#60205=ORIENTED_EDGE('',*,*,#44426,.F.);
#60206=ORIENTED_EDGE('',*,*,#44428,.F.);
#60207=ORIENTED_EDGE('',*,*,#44702,.F.);
#60208=ORIENTED_EDGE('',*,*,#44703,.T.);
#60209=ORIENTED_EDGE('',*,*,#44704,.T.);
#60210=ORIENTED_EDGE('',*,*,#44705,.F.);
#60211=ORIENTED_EDGE('',*,*,#44706,.T.);
#60212=ORIENTED_EDGE('',*,*,#44707,.F.);
#60213=ORIENTED_EDGE('',*,*,#44652,.F.);
#60214=ORIENTED_EDGE('',*,*,#44678,.F.);
#60215=ORIENTED_EDGE('',*,*,#44708,.F.);
#60216=ORIENTED_EDGE('',*,*,#44709,.T.);
#60217=ORIENTED_EDGE('',*,*,#44710,.F.);
#60218=ORIENTED_EDGE('',*,*,#44682,.T.);
#60219=ORIENTED_EDGE('',*,*,#44685,.T.);
#60220=ORIENTED_EDGE('',*,*,#44711,.T.);
#60221=ORIENTED_EDGE('',*,*,#44712,.T.);
#60222=ORIENTED_EDGE('',*,*,#44713,.T.);
#60223=ORIENTED_EDGE('',*,*,#44713,.F.);
#60224=ORIENTED_EDGE('',*,*,#44714,.F.);
#60225=ORIENTED_EDGE('',*,*,#44715,.F.);
#60226=ORIENTED_EDGE('',*,*,#44686,.F.);
#60227=ORIENTED_EDGE('',*,*,#44712,.F.);
#60228=ORIENTED_EDGE('',*,*,#44716,.F.);
#60229=ORIENTED_EDGE('',*,*,#44717,.F.);
#60230=ORIENTED_EDGE('',*,*,#44709,.F.);
#60231=ORIENTED_EDGE('',*,*,#44718,.F.);
#60232=ORIENTED_EDGE('',*,*,#44719,.T.);
#60233=ORIENTED_EDGE('',*,*,#44720,.F.);
#60234=ORIENTED_EDGE('',*,*,#44721,.T.);
#60235=ORIENTED_EDGE('',*,*,#44722,.F.);
#60236=ORIENTED_EDGE('',*,*,#44649,.T.);
#60237=ORIENTED_EDGE('',*,*,#44723,.F.);
#60238=ORIENTED_EDGE('',*,*,#44724,.T.);
#60239=ORIENTED_EDGE('',*,*,#44725,.F.);
#60240=ORIENTED_EDGE('',*,*,#44726,.F.);
#60241=ORIENTED_EDGE('',*,*,#44727,.F.);
#60242=ORIENTED_EDGE('',*,*,#44728,.T.);
#60243=ORIENTED_EDGE('',*,*,#44729,.T.);
#60244=ORIENTED_EDGE('',*,*,#44730,.T.);
#60245=ORIENTED_EDGE('',*,*,#44731,.F.);
#60246=ORIENTED_EDGE('',*,*,#44732,.F.);
#60247=ORIENTED_EDGE('',*,*,#44733,.F.);
#60248=ORIENTED_EDGE('',*,*,#44734,.T.);
#60249=ORIENTED_EDGE('',*,*,#44735,.F.);
#60250=ORIENTED_EDGE('',*,*,#44736,.T.);
#60251=ORIENTED_EDGE('',*,*,#44737,.F.);
#60252=ORIENTED_EDGE('',*,*,#44714,.T.);
#60253=ORIENTED_EDGE('',*,*,#44633,.F.);
#60254=ORIENTED_EDGE('',*,*,#44738,.T.);
#60255=ORIENTED_EDGE('',*,*,#44739,.T.);
#60256=ORIENTED_EDGE('',*,*,#44740,.T.);
#60257=ORIENTED_EDGE('',*,*,#44741,.T.);
#60258=ORIENTED_EDGE('',*,*,#44742,.F.);
#60259=ORIENTED_EDGE('',*,*,#44743,.F.);
#60260=ORIENTED_EDGE('',*,*,#44744,.F.);
#60261=ORIENTED_EDGE('',*,*,#44737,.T.);
#60262=ORIENTED_EDGE('',*,*,#44745,.T.);
#60263=ORIENTED_EDGE('',*,*,#44687,.T.);
#60264=ORIENTED_EDGE('',*,*,#44715,.T.);
#60265=ORIENTED_EDGE('',*,*,#44745,.F.);
#60266=ORIENTED_EDGE('',*,*,#44736,.F.);
#60267=ORIENTED_EDGE('',*,*,#44746,.F.);
#60268=ORIENTED_EDGE('',*,*,#44747,.F.);
#60269=ORIENTED_EDGE('',*,*,#44748,.F.);
#60270=ORIENTED_EDGE('',*,*,#44688,.F.);
#60271=ORIENTED_EDGE('',*,*,#44749,.T.);
#60272=ORIENTED_EDGE('',*,*,#44746,.T.);
#60273=ORIENTED_EDGE('',*,*,#44735,.T.);
#60274=ORIENTED_EDGE('',*,*,#44750,.T.);
#60275=ORIENTED_EDGE('',*,*,#44733,.T.);
#60276=ORIENTED_EDGE('',*,*,#44751,.T.);
#60277=ORIENTED_EDGE('',*,*,#44752,.T.);
#60278=ORIENTED_EDGE('',*,*,#44753,.T.);
#60279=ORIENTED_EDGE('',*,*,#44750,.F.);
#60280=ORIENTED_EDGE('',*,*,#44734,.F.);
#60281=ORIENTED_EDGE('',*,*,#44753,.F.);
#60282=ORIENTED_EDGE('',*,*,#44754,.F.);
#60283=ORIENTED_EDGE('',*,*,#44755,.F.);
#60284=ORIENTED_EDGE('',*,*,#44756,.F.);
#60285=ORIENTED_EDGE('',*,*,#44752,.F.);
#60286=ORIENTED_EDGE('',*,*,#44757,.F.);
#60287=ORIENTED_EDGE('',*,*,#44758,.F.);
#60288=ORIENTED_EDGE('',*,*,#44759,.T.);
#60289=ORIENTED_EDGE('',*,*,#44760,.F.);
#60290=ORIENTED_EDGE('',*,*,#44761,.T.);
#60291=ORIENTED_EDGE('',*,*,#44762,.T.);
#60292=ORIENTED_EDGE('',*,*,#44763,.F.);
#60293=ORIENTED_EDGE('',*,*,#44764,.T.);
#60294=ORIENTED_EDGE('',*,*,#44765,.T.);
#60295=ORIENTED_EDGE('',*,*,#44766,.F.);
#60296=ORIENTED_EDGE('',*,*,#44767,.T.);
#60297=ORIENTED_EDGE('',*,*,#44516,.F.);
#60298=ORIENTED_EDGE('',*,*,#44519,.T.);
#60299=ORIENTED_EDGE('',*,*,#44521,.F.);
#60300=ORIENTED_EDGE('',*,*,#44523,.T.);
#60301=ORIENTED_EDGE('',*,*,#44525,.F.);
#60302=ORIENTED_EDGE('',*,*,#44527,.F.);
#60303=ORIENTED_EDGE('',*,*,#44529,.F.);
#60304=ORIENTED_EDGE('',*,*,#44533,.F.);
#60305=ORIENTED_EDGE('',*,*,#44768,.T.);
#60306=ORIENTED_EDGE('',*,*,#44769,.F.);
#60307=ORIENTED_EDGE('',*,*,#44627,.T.);
#60308=ORIENTED_EDGE('',*,*,#44770,.F.);
#60309=ORIENTED_EDGE('',*,*,#44754,.T.);
#60310=ORIENTED_EDGE('',*,*,#44725,.T.);
#60311=ORIENTED_EDGE('',*,*,#44771,.T.);
#60312=ORIENTED_EDGE('',*,*,#44772,.T.);
#60313=ORIENTED_EDGE('',*,*,#44773,.T.);
#60314=ORIENTED_EDGE('',*,*,#44771,.F.);
#60315=ORIENTED_EDGE('',*,*,#44724,.F.);
#60316=ORIENTED_EDGE('',*,*,#44774,.F.);
#60317=ORIENTED_EDGE('',*,*,#44775,.F.);
#60318=ORIENTED_EDGE('',*,*,#44723,.T.);
#60319=ORIENTED_EDGE('',*,*,#44648,.T.);
#60320=ORIENTED_EDGE('',*,*,#44776,.T.);
#60321=ORIENTED_EDGE('',*,*,#44774,.T.);
#60322=ORIENTED_EDGE('',*,*,#44772,.F.);
#60323=ORIENTED_EDGE('',*,*,#44775,.T.);
#60324=ORIENTED_EDGE('',*,*,#44776,.F.);
#60325=ORIENTED_EDGE('',*,*,#44647,.T.);
#60326=ORIENTED_EDGE('',*,*,#44638,.F.);
#60327=ORIENTED_EDGE('',*,*,#44191,.F.);
#60328=ORIENTED_EDGE('',*,*,#44200,.F.);
#60329=ORIENTED_EDGE('',*,*,#44202,.T.);
#60330=ORIENTED_EDGE('',*,*,#44204,.F.);
#60331=ORIENTED_EDGE('',*,*,#44206,.T.);
#60332=ORIENTED_EDGE('',*,*,#44777,.F.);
#60333=ORIENTED_EDGE('',*,*,#44778,.T.);
#60334=ORIENTED_EDGE('',*,*,#44779,.F.);
#60335=ORIENTED_EDGE('',*,*,#44780,.T.);
#60336=ORIENTED_EDGE('',*,*,#44781,.F.);
#60337=ORIENTED_EDGE('',*,*,#44197,.T.);
#60338=ORIENTED_EDGE('',*,*,#44619,.F.);
#60339=ORIENTED_EDGE('',*,*,#44634,.T.);
#60340=ORIENTED_EDGE('',*,*,#44631,.T.);
#60341=ORIENTED_EDGE('',*,*,#44782,.F.);
#60342=ORIENTED_EDGE('',*,*,#44562,.T.);
#60343=ORIENTED_EDGE('',*,*,#44569,.F.);
#60344=ORIENTED_EDGE('',*,*,#44571,.T.);
#60345=ORIENTED_EDGE('',*,*,#44573,.F.);
#60346=ORIENTED_EDGE('',*,*,#44575,.T.);
#60347=ORIENTED_EDGE('',*,*,#44783,.T.);
#60348=ORIENTED_EDGE('',*,*,#44784,.T.);
#60349=ORIENTED_EDGE('',*,*,#44785,.T.);
#60350=ORIENTED_EDGE('',*,*,#44786,.F.);
#60351=ORIENTED_EDGE('',*,*,#44566,.T.);
#60352=ORIENTED_EDGE('',*,*,#44787,.F.);
#60353=ORIENTED_EDGE('',*,*,#44788,.T.);
#60354=ORIENTED_EDGE('',*,*,#44789,.T.);
#60355=ORIENTED_EDGE('',*,*,#44641,.T.);
#60356=ORIENTED_EDGE('',*,*,#44650,.T.);
#60357=ORIENTED_EDGE('',*,*,#44722,.T.);
#60358=ORIENTED_EDGE('',*,*,#44790,.T.);
#60359=ORIENTED_EDGE('',*,*,#44720,.T.);
#60360=ORIENTED_EDGE('',*,*,#44791,.T.);
#60361=ORIENTED_EDGE('',*,*,#44675,.T.);
#60362=ORIENTED_EDGE('',*,*,#44792,.T.);
#60363=ORIENTED_EDGE('',*,*,#44790,.F.);
#60364=ORIENTED_EDGE('',*,*,#44721,.F.);
#60365=ORIENTED_EDGE('',*,*,#44792,.F.);
#60366=ORIENTED_EDGE('',*,*,#44674,.F.);
#60367=ORIENTED_EDGE('',*,*,#44793,.T.);
#60368=ORIENTED_EDGE('',*,*,#44642,.T.);
#60369=ORIENTED_EDGE('',*,*,#44673,.F.);
#60370=ORIENTED_EDGE('',*,*,#44794,.F.);
#60371=ORIENTED_EDGE('',*,*,#44643,.T.);
#60372=ORIENTED_EDGE('',*,*,#44793,.F.);
#60373=ORIENTED_EDGE('',*,*,#44380,.F.);
#60374=ORIENTED_EDGE('',*,*,#44795,.F.);
#60375=ORIENTED_EDGE('',*,*,#44703,.F.);
#60376=ORIENTED_EDGE('',*,*,#44796,.F.);
#60377=ORIENTED_EDGE('',*,*,#44383,.F.);
#60378=ORIENTED_EDGE('',*,*,#44797,.F.);
#60379=ORIENTED_EDGE('',*,*,#44704,.F.);
#60380=ORIENTED_EDGE('',*,*,#44795,.T.);
#60381=ORIENTED_EDGE('',*,*,#44386,.F.);
#60382=ORIENTED_EDGE('',*,*,#44798,.T.);
#60383=ORIENTED_EDGE('',*,*,#44705,.T.);
#60384=ORIENTED_EDGE('',*,*,#44797,.T.);
#60385=ORIENTED_EDGE('',*,*,#44389,.F.);
#60386=ORIENTED_EDGE('',*,*,#44799,.F.);
#60387=ORIENTED_EDGE('',*,*,#44706,.F.);
#60388=ORIENTED_EDGE('',*,*,#44798,.F.);
#60389=ORIENTED_EDGE('',*,*,#44392,.F.);
#60390=ORIENTED_EDGE('',*,*,#44800,.T.);
#60391=ORIENTED_EDGE('',*,*,#44700,.T.);
#60392=ORIENTED_EDGE('',*,*,#44799,.T.);
#60393=ORIENTED_EDGE('',*,*,#44395,.F.);
#60394=ORIENTED_EDGE('',*,*,#44416,.F.);
#60395=ORIENTED_EDGE('',*,*,#44701,.F.);
#60396=ORIENTED_EDGE('',*,*,#44800,.F.);
#60397=ORIENTED_EDGE('',*,*,#44437,.F.);
#60398=ORIENTED_EDGE('',*,*,#44801,.T.);
#60399=ORIENTED_EDGE('',*,*,#44802,.T.);
#60400=ORIENTED_EDGE('',*,*,#44803,.T.);
#60401=ORIENTED_EDGE('',*,*,#44440,.F.);
#60402=ORIENTED_EDGE('',*,*,#44804,.F.);
#60403=ORIENTED_EDGE('',*,*,#44805,.F.);
#60404=ORIENTED_EDGE('',*,*,#44801,.F.);
#60405=ORIENTED_EDGE('',*,*,#44443,.F.);
#60406=ORIENTED_EDGE('',*,*,#44458,.T.);
#60407=ORIENTED_EDGE('',*,*,#44806,.T.);
#60408=ORIENTED_EDGE('',*,*,#44804,.T.);
#60409=ORIENTED_EDGE('',*,*,#44475,.F.);
#60410=ORIENTED_EDGE('',*,*,#44807,.F.);
#60411=ORIENTED_EDGE('',*,*,#44808,.F.);
#60412=ORIENTED_EDGE('',*,*,#44809,.F.);
#60413=ORIENTED_EDGE('',*,*,#44478,.F.);
#60414=ORIENTED_EDGE('',*,*,#44810,.F.);
#60415=ORIENTED_EDGE('',*,*,#44811,.F.);
#60416=ORIENTED_EDGE('',*,*,#44807,.T.);
#60417=ORIENTED_EDGE('',*,*,#44481,.F.);
#60418=ORIENTED_EDGE('',*,*,#44812,.F.);
#60419=ORIENTED_EDGE('',*,*,#44763,.T.);
#60420=ORIENTED_EDGE('',*,*,#44813,.T.);
#60421=ORIENTED_EDGE('',*,*,#44814,.T.);
#60422=ORIENTED_EDGE('',*,*,#44810,.T.);
#60423=ORIENTED_EDGE('',*,*,#44484,.F.);
#60424=ORIENTED_EDGE('',*,*,#44815,.T.);
#60425=ORIENTED_EDGE('',*,*,#44764,.F.);
#60426=ORIENTED_EDGE('',*,*,#44812,.T.);
#60427=ORIENTED_EDGE('',*,*,#44487,.F.);
#60428=ORIENTED_EDGE('',*,*,#44816,.F.);
#60429=ORIENTED_EDGE('',*,*,#44765,.F.);
#60430=ORIENTED_EDGE('',*,*,#44815,.F.);
#60431=ORIENTED_EDGE('',*,*,#44490,.F.);
#60432=ORIENTED_EDGE('',*,*,#44817,.T.);
#60433=ORIENTED_EDGE('',*,*,#44766,.T.);
#60434=ORIENTED_EDGE('',*,*,#44816,.T.);
#60435=ORIENTED_EDGE('',*,*,#44493,.F.);
#60436=ORIENTED_EDGE('',*,*,#44517,.F.);
#60437=ORIENTED_EDGE('',*,*,#44767,.F.);
#60438=ORIENTED_EDGE('',*,*,#44817,.F.);
#60439=ORIENTED_EDGE('',*,*,#44756,.T.);
#60440=ORIENTED_EDGE('',*,*,#44818,.T.);
#60441=ORIENTED_EDGE('',*,*,#44460,.F.);
#60442=ORIENTED_EDGE('',*,*,#44462,.T.);
#60443=ORIENTED_EDGE('',*,*,#44464,.T.);
#60444=ORIENTED_EDGE('',*,*,#44819,.F.);
#60445=ORIENTED_EDGE('',*,*,#44747,.T.);
#60446=ORIENTED_EDGE('',*,*,#44749,.F.);
#60447=ORIENTED_EDGE('',*,*,#44215,.F.);
#60448=ORIENTED_EDGE('',*,*,#44820,.F.);
#60449=ORIENTED_EDGE('',*,*,#44668,.F.);
#60450=ORIENTED_EDGE('',*,*,#44821,.F.);
#60451=ORIENTED_EDGE('',*,*,#44218,.F.);
#60452=ORIENTED_EDGE('',*,*,#44822,.T.);
#60453=ORIENTED_EDGE('',*,*,#44669,.T.);
#60454=ORIENTED_EDGE('',*,*,#44820,.T.);
#60455=ORIENTED_EDGE('',*,*,#44221,.F.);
#60456=ORIENTED_EDGE('',*,*,#44823,.F.);
#60457=ORIENTED_EDGE('',*,*,#44670,.F.);
#60458=ORIENTED_EDGE('',*,*,#44822,.F.);
#60459=ORIENTED_EDGE('',*,*,#44224,.F.);
#60460=ORIENTED_EDGE('',*,*,#44824,.T.);
#60461=ORIENTED_EDGE('',*,*,#44671,.T.);
#60462=ORIENTED_EDGE('',*,*,#44823,.T.);
#60463=ORIENTED_EDGE('',*,*,#44227,.F.);
#60464=ORIENTED_EDGE('',*,*,#44825,.F.);
#60465=ORIENTED_EDGE('',*,*,#44644,.T.);
#60466=ORIENTED_EDGE('',*,*,#44794,.T.);
#60467=ORIENTED_EDGE('',*,*,#44672,.F.);
#60468=ORIENTED_EDGE('',*,*,#44824,.F.);
#60469=ORIENTED_EDGE('',*,*,#44230,.F.);
#60470=ORIENTED_EDGE('',*,*,#44252,.T.);
#60471=ORIENTED_EDGE('',*,*,#44645,.T.);
#60472=ORIENTED_EDGE('',*,*,#44825,.T.);
#60473=ORIENTED_EDGE('',*,*,#44171,.F.);
#60474=ORIENTED_EDGE('',*,*,#44826,.T.);
#60475=ORIENTED_EDGE('',*,*,#44779,.T.);
#60476=ORIENTED_EDGE('',*,*,#44827,.T.);
#60477=ORIENTED_EDGE('',*,*,#44174,.F.);
#60478=ORIENTED_EDGE('',*,*,#44828,.F.);
#60479=ORIENTED_EDGE('',*,*,#44780,.F.);
#60480=ORIENTED_EDGE('',*,*,#44826,.F.);
#60481=ORIENTED_EDGE('',*,*,#44177,.F.);
#60482=ORIENTED_EDGE('',*,*,#44198,.T.);
#60483=ORIENTED_EDGE('',*,*,#44781,.T.);
#60484=ORIENTED_EDGE('',*,*,#44828,.T.);
#60485=ORIENTED_EDGE('',*,*,#44165,.F.);
#60486=ORIENTED_EDGE('',*,*,#44829,.T.);
#60487=ORIENTED_EDGE('',*,*,#44777,.T.);
#60488=ORIENTED_EDGE('',*,*,#44205,.T.);
#60489=ORIENTED_EDGE('',*,*,#44168,.F.);
#60490=ORIENTED_EDGE('',*,*,#44827,.F.);
#60491=ORIENTED_EDGE('',*,*,#44778,.F.);
#60492=ORIENTED_EDGE('',*,*,#44829,.F.);
#60493=ORIENTED_EDGE('',*,*,#44791,.F.);
#60494=ORIENTED_EDGE('',*,*,#44719,.F.);
#60495=ORIENTED_EDGE('',*,*,#44830,.T.);
#60496=ORIENTED_EDGE('',*,*,#44676,.F.);
#60497=ORIENTED_EDGE('',*,*,#44755,.T.);
#60498=ORIENTED_EDGE('',*,*,#44770,.T.);
#60499=ORIENTED_EDGE('',*,*,#44626,.T.);
#60500=ORIENTED_EDGE('',*,*,#44831,.T.);
#60501=ORIENTED_EDGE('',*,*,#44457,.F.);
#60502=ORIENTED_EDGE('',*,*,#44818,.F.);
#60503=ORIENTED_EDGE('',*,*,#44711,.F.);
#60504=ORIENTED_EDGE('',*,*,#44684,.T.);
#60505=ORIENTED_EDGE('',*,*,#44832,.F.);
#60506=ORIENTED_EDGE('',*,*,#44716,.T.);
#60507=ORIENTED_EDGE('',*,*,#44751,.F.);
#60508=ORIENTED_EDGE('',*,*,#44732,.T.);
#60509=ORIENTED_EDGE('',*,*,#44833,.F.);
#60510=ORIENTED_EDGE('',*,*,#44834,.T.);
#60511=ORIENTED_EDGE('',*,*,#44835,.F.);
#60512=ORIENTED_EDGE('',*,*,#44757,.T.);
#60513=ORIENTED_EDGE('',*,*,#44677,.F.);
#60514=ORIENTED_EDGE('',*,*,#44830,.F.);
#60515=ORIENTED_EDGE('',*,*,#44718,.T.);
#60516=ORIENTED_EDGE('',*,*,#44708,.T.);
#60517=ORIENTED_EDGE('',*,*,#44836,.F.);
#60518=ORIENTED_EDGE('',*,*,#44621,.F.);
#60519=ORIENTED_EDGE('',*,*,#44837,.F.);
#60520=ORIENTED_EDGE('',*,*,#44266,.F.);
#60521=ORIENTED_EDGE('',*,*,#44319,.F.);
#60522=ORIENTED_EDGE('',*,*,#44321,.F.);
#60523=ORIENTED_EDGE('',*,*,#44838,.F.);
#60524=ORIENTED_EDGE('',*,*,#44839,.F.);
#60525=ORIENTED_EDGE('',*,*,#44280,.F.);
#60526=ORIENTED_EDGE('',*,*,#44840,.T.);
#60527=ORIENTED_EDGE('',*,*,#44838,.T.);
#60528=ORIENTED_EDGE('',*,*,#44320,.T.);
#60529=ORIENTED_EDGE('',*,*,#44636,.T.);
#60530=ORIENTED_EDGE('',*,*,#44267,.T.);
#60531=ORIENTED_EDGE('',*,*,#44837,.T.);
#60532=ORIENTED_EDGE('',*,*,#44620,.T.);
#60533=ORIENTED_EDGE('',*,*,#44609,.F.);
#60534=ORIENTED_EDGE('',*,*,#44194,.T.);
#60535=ORIENTED_EDGE('',*,*,#44646,.T.);
#60536=ORIENTED_EDGE('',*,*,#44269,.T.);
#60537=ORIENTED_EDGE('',*,*,#44635,.F.);
#60538=ORIENTED_EDGE('',*,*,#44616,.F.);
#60539=ORIENTED_EDGE('',*,*,#44259,.T.);
#60540=ORIENTED_EDGE('',*,*,#44841,.T.);
#60541=ORIENTED_EDGE('',*,*,#44666,.F.);
#60542=ORIENTED_EDGE('',*,*,#44842,.T.);
#60543=ORIENTED_EDGE('',*,*,#44843,.T.);
#60544=ORIENTED_EDGE('',*,*,#44844,.F.);
#60545=ORIENTED_EDGE('',*,*,#44665,.F.);
#60546=ORIENTED_EDGE('',*,*,#44312,.F.);
#60547=ORIENTED_EDGE('',*,*,#44845,.T.);
#60548=ORIENTED_EDGE('',*,*,#44842,.F.);
#60549=ORIENTED_EDGE('',*,*,#44262,.F.);
#60550=ORIENTED_EDGE('',*,*,#44272,.F.);
#60551=ORIENTED_EDGE('',*,*,#44274,.F.);
#60552=ORIENTED_EDGE('',*,*,#44846,.F.);
#60553=ORIENTED_EDGE('',*,*,#44843,.F.);
#60554=ORIENTED_EDGE('',*,*,#44845,.F.);
#60555=ORIENTED_EDGE('',*,*,#44311,.F.);
#60556=ORIENTED_EDGE('',*,*,#44316,.F.);
#60557=ORIENTED_EDGE('',*,*,#44317,.F.);
#60558=ORIENTED_EDGE('',*,*,#44212,.F.);
#60559=ORIENTED_EDGE('',*,*,#44821,.T.);
#60560=ORIENTED_EDGE('',*,*,#44667,.T.);
#60561=ORIENTED_EDGE('',*,*,#44844,.T.);
#60562=ORIENTED_EDGE('',*,*,#44846,.T.);
#60563=ORIENTED_EDGE('',*,*,#44273,.T.);
#60564=ORIENTED_EDGE('',*,*,#44768,.F.);
#60565=ORIENTED_EDGE('',*,*,#44532,.T.);
#60566=ORIENTED_EDGE('',*,*,#44847,.T.);
#60567=ORIENTED_EDGE('',*,*,#44848,.T.);
#60568=ORIENTED_EDGE('',*,*,#44848,.F.);
#60569=ORIENTED_EDGE('',*,*,#44849,.T.);
#60570=ORIENTED_EDGE('',*,*,#44628,.T.);
#60571=ORIENTED_EDGE('',*,*,#44769,.T.);
#60572=ORIENTED_EDGE('',*,*,#44584,.F.);
#60573=ORIENTED_EDGE('',*,*,#44850,.F.);
#60574=ORIENTED_EDGE('',*,*,#44851,.F.);
#60575=ORIENTED_EDGE('',*,*,#44852,.F.);
#60576=ORIENTED_EDGE('',*,*,#44587,.F.);
#60577=ORIENTED_EDGE('',*,*,#44853,.T.);
#60578=ORIENTED_EDGE('',*,*,#44854,.T.);
#60579=ORIENTED_EDGE('',*,*,#44850,.T.);
#60580=ORIENTED_EDGE('',*,*,#44590,.F.);
#60581=ORIENTED_EDGE('',*,*,#44602,.F.);
#60582=ORIENTED_EDGE('',*,*,#44855,.F.);
#60583=ORIENTED_EDGE('',*,*,#44853,.F.);
#60584=ORIENTED_EDGE('',*,*,#44333,.F.);
#60585=ORIENTED_EDGE('',*,*,#44856,.T.);
#60586=ORIENTED_EDGE('',*,*,#44694,.T.);
#60587=ORIENTED_EDGE('',*,*,#44857,.T.);
#60588=ORIENTED_EDGE('',*,*,#44336,.F.);
#60589=ORIENTED_EDGE('',*,*,#44858,.F.);
#60590=ORIENTED_EDGE('',*,*,#44695,.T.);
#60591=ORIENTED_EDGE('',*,*,#44856,.F.);
#60592=ORIENTED_EDGE('',*,*,#44339,.F.);
#60593=ORIENTED_EDGE('',*,*,#44359,.F.);
#60594=ORIENTED_EDGE('',*,*,#44696,.T.);
#60595=ORIENTED_EDGE('',*,*,#44858,.T.);
#60596=ORIENTED_EDGE('',*,*,#44283,.F.);
#60597=ORIENTED_EDGE('',*,*,#44859,.F.);
#60598=ORIENTED_EDGE('',*,*,#44660,.F.);
#60599=ORIENTED_EDGE('',*,*,#44860,.T.);
#60600=ORIENTED_EDGE('',*,*,#44839,.T.);
#60601=ORIENTED_EDGE('',*,*,#44840,.F.);
#60602=ORIENTED_EDGE('',*,*,#44286,.F.);
#60603=ORIENTED_EDGE('',*,*,#44861,.T.);
#60604=ORIENTED_EDGE('',*,*,#44661,.T.);
#60605=ORIENTED_EDGE('',*,*,#44859,.T.);
#60606=ORIENTED_EDGE('',*,*,#44289,.F.);
#60607=ORIENTED_EDGE('',*,*,#44862,.F.);
#60608=ORIENTED_EDGE('',*,*,#44662,.F.);
#60609=ORIENTED_EDGE('',*,*,#44861,.F.);
#60610=ORIENTED_EDGE('',*,*,#44292,.F.);
#60611=ORIENTED_EDGE('',*,*,#44863,.T.);
#60612=ORIENTED_EDGE('',*,*,#44663,.T.);
#60613=ORIENTED_EDGE('',*,*,#44862,.T.);
#60614=ORIENTED_EDGE('',*,*,#44295,.F.);
#60615=ORIENTED_EDGE('',*,*,#44314,.F.);
#60616=ORIENTED_EDGE('',*,*,#44664,.F.);
#60617=ORIENTED_EDGE('',*,*,#44863,.F.);
#60618=ORIENTED_EDGE('',*,*,#44539,.F.);
#60619=ORIENTED_EDGE('',*,*,#44864,.T.);
#60620=ORIENTED_EDGE('',*,*,#44783,.F.);
#60621=ORIENTED_EDGE('',*,*,#44574,.T.);
#60622=ORIENTED_EDGE('',*,*,#44542,.F.);
#60623=ORIENTED_EDGE('',*,*,#44865,.F.);
#60624=ORIENTED_EDGE('',*,*,#44784,.F.);
#60625=ORIENTED_EDGE('',*,*,#44864,.F.);
#60626=ORIENTED_EDGE('',*,*,#44545,.F.);
#60627=ORIENTED_EDGE('',*,*,#44866,.F.);
#60628=ORIENTED_EDGE('',*,*,#44785,.F.);
#60629=ORIENTED_EDGE('',*,*,#44865,.T.);
#60630=ORIENTED_EDGE('',*,*,#44548,.F.);
#60631=ORIENTED_EDGE('',*,*,#44567,.T.);
#60632=ORIENTED_EDGE('',*,*,#44786,.T.);
#60633=ORIENTED_EDGE('',*,*,#44866,.T.);
#60634=ORIENTED_EDGE('',*,*,#44581,.F.);
#60635=ORIENTED_EDGE('',*,*,#44852,.T.);
#60636=ORIENTED_EDGE('',*,*,#44867,.T.);
#60637=ORIENTED_EDGE('',*,*,#44607,.T.);
#60638=ORIENTED_EDGE('',*,*,#44377,.F.);
#60639=ORIENTED_EDGE('',*,*,#44796,.T.);
#60640=ORIENTED_EDGE('',*,*,#44702,.T.);
#60641=ORIENTED_EDGE('',*,*,#44427,.T.);
#60642=ORIENTED_EDGE('',*,*,#44330,.F.);
#60643=ORIENTED_EDGE('',*,*,#44857,.F.);
#60644=ORIENTED_EDGE('',*,*,#44693,.T.);
#60645=ORIENTED_EDGE('',*,*,#44868,.F.);
#60646=ORIENTED_EDGE('',*,*,#44327,.F.);
#60647=ORIENTED_EDGE('',*,*,#44868,.T.);
#60648=ORIENTED_EDGE('',*,*,#44692,.T.);
#60649=ORIENTED_EDGE('',*,*,#44368,.T.);
#60650=ORIENTED_EDGE('',*,*,#44659,.F.);
#60651=ORIENTED_EDGE('',*,*,#44370,.T.);
#60652=ORIENTED_EDGE('',*,*,#44691,.T.);
#60653=ORIENTED_EDGE('',*,*,#44622,.T.);
#60654=ORIENTED_EDGE('',*,*,#44836,.T.);
#60655=ORIENTED_EDGE('',*,*,#44860,.F.);
#60656=ORIENTED_EDGE('',*,*,#44531,.T.);
#60657=ORIENTED_EDGE('',*,*,#44869,.F.);
#60658=ORIENTED_EDGE('',*,*,#44808,.T.);
#60659=ORIENTED_EDGE('',*,*,#44811,.T.);
#60660=ORIENTED_EDGE('',*,*,#44814,.F.);
#60661=ORIENTED_EDGE('',*,*,#44870,.T.);
#60662=ORIENTED_EDGE('',*,*,#44871,.T.);
#60663=ORIENTED_EDGE('',*,*,#44872,.F.);
#60664=ORIENTED_EDGE('',*,*,#44873,.T.);
#60665=ORIENTED_EDGE('',*,*,#44874,.F.);
#60666=ORIENTED_EDGE('',*,*,#44875,.T.);
#60667=ORIENTED_EDGE('',*,*,#44876,.F.);
#60668=ORIENTED_EDGE('',*,*,#44564,.T.);
#60669=ORIENTED_EDGE('',*,*,#44877,.F.);
#60670=ORIENTED_EDGE('',*,*,#44629,.T.);
#60671=ORIENTED_EDGE('',*,*,#44849,.F.);
#60672=ORIENTED_EDGE('',*,*,#44847,.F.);
#60673=ORIENTED_EDGE('',*,*,#44851,.T.);
#60674=ORIENTED_EDGE('',*,*,#44854,.F.);
#60675=ORIENTED_EDGE('',*,*,#44855,.T.);
#60676=ORIENTED_EDGE('',*,*,#44601,.F.);
#60677=ORIENTED_EDGE('',*,*,#44604,.T.);
#60678=ORIENTED_EDGE('',*,*,#44606,.F.);
#60679=ORIENTED_EDGE('',*,*,#44608,.T.);
#60680=ORIENTED_EDGE('',*,*,#44867,.F.);
#60681=ORIENTED_EDGE('',*,*,#44878,.F.);
#60682=ORIENTED_EDGE('',*,*,#44879,.T.);
#60683=ORIENTED_EDGE('',*,*,#44880,.T.);
#60684=ORIENTED_EDGE('',*,*,#44624,.F.);
#60685=ORIENTED_EDGE('',*,*,#44690,.T.);
#60686=ORIENTED_EDGE('',*,*,#44881,.F.);
#60687=ORIENTED_EDGE('',*,*,#44434,.F.);
#60688=ORIENTED_EDGE('',*,*,#44803,.F.);
#60689=ORIENTED_EDGE('',*,*,#44879,.F.);
#60690=ORIENTED_EDGE('',*,*,#44465,.T.);
#60691=ORIENTED_EDGE('',*,*,#44877,.T.);
#60692=ORIENTED_EDGE('',*,*,#44563,.T.);
#60693=ORIENTED_EDGE('',*,*,#44782,.T.);
#60694=ORIENTED_EDGE('',*,*,#44630,.T.);
#60695=ORIENTED_EDGE('',*,*,#44658,.F.);
#60696=ORIENTED_EDGE('',*,*,#44882,.T.);
#60697=ORIENTED_EDGE('',*,*,#44697,.T.);
#60698=ORIENTED_EDGE('',*,*,#44357,.F.);
#60699=ORIENTED_EDGE('',*,*,#44657,.F.);
#60700=ORIENTED_EDGE('',*,*,#44883,.F.);
#60701=ORIENTED_EDGE('',*,*,#44698,.T.);
#60702=ORIENTED_EDGE('',*,*,#44882,.F.);
#60703=ORIENTED_EDGE('',*,*,#44883,.T.);
#60704=ORIENTED_EDGE('',*,*,#44656,.F.);
#60705=ORIENTED_EDGE('',*,*,#44681,.T.);
#60706=ORIENTED_EDGE('',*,*,#44699,.T.);
#60707=ORIENTED_EDGE('',*,*,#44472,.F.);
#60708=ORIENTED_EDGE('',*,*,#44809,.T.);
#60709=ORIENTED_EDGE('',*,*,#44869,.T.);
#60710=ORIENTED_EDGE('',*,*,#44530,.T.);
#60711=ORIENTED_EDGE('',*,*,#44805,.T.);
#60712=ORIENTED_EDGE('',*,*,#44806,.F.);
#60713=ORIENTED_EDGE('',*,*,#44831,.F.);
#60714=ORIENTED_EDGE('',*,*,#44625,.T.);
#60715=ORIENTED_EDGE('',*,*,#44880,.F.);
#60716=ORIENTED_EDGE('',*,*,#44802,.F.);
#60717=ORIENTED_EDGE('',*,*,#44884,.F.);
#60718=ORIENTED_EDGE('',*,*,#44885,.T.);
#60719=ORIENTED_EDGE('',*,*,#44886,.T.);
#60720=ORIENTED_EDGE('',*,*,#44884,.T.);
#60721=ORIENTED_EDGE('',*,*,#44886,.F.);
#60722=ORIENTED_EDGE('',*,*,#44887,.F.);
#60723=ORIENTED_EDGE('',*,*,#44885,.F.);
#60724=ORIENTED_EDGE('',*,*,#44707,.T.);
#60725=ORIENTED_EDGE('',*,*,#44888,.T.);
#60726=ORIENTED_EDGE('',*,*,#44743,.T.);
#60727=ORIENTED_EDGE('',*,*,#44888,.F.);
#60728=ORIENTED_EDGE('',*,*,#44889,.F.);
#60729=ORIENTED_EDGE('',*,*,#44890,.F.);
#60730=ORIENTED_EDGE('',*,*,#44891,.T.);
#60731=ORIENTED_EDGE('',*,*,#44728,.F.);
#60732=ORIENTED_EDGE('',*,*,#44892,.T.);
#60733=ORIENTED_EDGE('',*,*,#44729,.F.);
#60734=ORIENTED_EDGE('',*,*,#44891,.F.);
#60735=ORIENTED_EDGE('',*,*,#44893,.F.);
#60736=ORIENTED_EDGE('',*,*,#44894,.F.);
#60737=ORIENTED_EDGE('',*,*,#44730,.F.);
#60738=ORIENTED_EDGE('',*,*,#44892,.F.);
#60739=ORIENTED_EDGE('',*,*,#44895,.F.);
#60740=ORIENTED_EDGE('',*,*,#44896,.F.);
#60741=ORIENTED_EDGE('',*,*,#44897,.T.);
#60742=ORIENTED_EDGE('',*,*,#44739,.F.);
#60743=ORIENTED_EDGE('',*,*,#44898,.F.);
#60744=ORIENTED_EDGE('',*,*,#44899,.F.);
#60745=ORIENTED_EDGE('',*,*,#44900,.T.);
#60746=ORIENTED_EDGE('',*,*,#44740,.F.);
#60747=ORIENTED_EDGE('',*,*,#44897,.F.);
#60748=ORIENTED_EDGE('',*,*,#44901,.F.);
#60749=ORIENTED_EDGE('',*,*,#44902,.T.);
#60750=ORIENTED_EDGE('',*,*,#44741,.F.);
#60751=ORIENTED_EDGE('',*,*,#44900,.F.);
#60752=ORIENTED_EDGE('',*,*,#44903,.F.);
#60753=ORIENTED_EDGE('',*,*,#44898,.T.);
#60754=ORIENTED_EDGE('',*,*,#44738,.F.);
#60755=ORIENTED_EDGE('',*,*,#44902,.F.);
#60756=ORIENTED_EDGE('',*,*,#44904,.F.);
#60757=ORIENTED_EDGE('',*,*,#44789,.F.);
#60758=ORIENTED_EDGE('',*,*,#44905,.T.);
#60759=ORIENTED_EDGE('',*,*,#44744,.T.);
#60760=ORIENTED_EDGE('',*,*,#44905,.F.);
#60761=ORIENTED_EDGE('',*,*,#44906,.F.);
#60762=ORIENTED_EDGE('',*,*,#44907,.T.);
#60763=ORIENTED_EDGE('',*,*,#44887,.T.);
#60764=ORIENTED_EDGE('',*,*,#44907,.F.);
#60765=ORIENTED_EDGE('',*,*,#44908,.F.);
#60766=ORIENTED_EDGE('',*,*,#44889,.T.);
#60767=ORIENTED_EDGE('',*,*,#44727,.T.);
#60768=ORIENTED_EDGE('',*,*,#44909,.T.);
#60769=ORIENTED_EDGE('',*,*,#44910,.F.);
#60770=ORIENTED_EDGE('',*,*,#44911,.T.);
#60771=ORIENTED_EDGE('',*,*,#44760,.T.);
#60772=ORIENTED_EDGE('',*,*,#44912,.T.);
#60773=ORIENTED_EDGE('',*,*,#44912,.F.);
#60774=ORIENTED_EDGE('',*,*,#44759,.F.);
#60775=ORIENTED_EDGE('',*,*,#44913,.F.);
#60776=ORIENTED_EDGE('',*,*,#44914,.T.);
#60777=ORIENTED_EDGE('',*,*,#44731,.T.);
#60778=ORIENTED_EDGE('',*,*,#44894,.T.);
#60779=ORIENTED_EDGE('',*,*,#44915,.T.);
#60780=ORIENTED_EDGE('',*,*,#44833,.T.);
#60781=ORIENTED_EDGE('',*,*,#44683,.T.);
#60782=ORIENTED_EDGE('',*,*,#44710,.T.);
#60783=ORIENTED_EDGE('',*,*,#44717,.T.);
#60784=ORIENTED_EDGE('',*,*,#44832,.T.);
#60785=ORIENTED_EDGE('',*,*,#44758,.T.);
#60786=ORIENTED_EDGE('',*,*,#44835,.T.);
#60787=ORIENTED_EDGE('',*,*,#44916,.T.);
#60788=ORIENTED_EDGE('',*,*,#44913,.T.);
#60789=ORIENTED_EDGE('',*,*,#44917,.T.);
#60790=ORIENTED_EDGE('',*,*,#44918,.T.);
#60791=ORIENTED_EDGE('',*,*,#44910,.T.);
#60792=ORIENTED_EDGE('',*,*,#44914,.F.);
#60793=ORIENTED_EDGE('',*,*,#44916,.F.);
#60794=ORIENTED_EDGE('',*,*,#44834,.F.);
#60795=ORIENTED_EDGE('',*,*,#44915,.F.);
#60796=ORIENTED_EDGE('',*,*,#44895,.T.);
#60797=ORIENTED_EDGE('',*,*,#44893,.T.);
#60798=ORIENTED_EDGE('',*,*,#44890,.T.);
#60799=ORIENTED_EDGE('',*,*,#44908,.T.);
#60800=ORIENTED_EDGE('',*,*,#44919,.T.);
#60801=ORIENTED_EDGE('',*,*,#44920,.T.);
#60802=ORIENTED_EDGE('',*,*,#44921,.T.);
#60803=ORIENTED_EDGE('',*,*,#44903,.T.);
#60804=ORIENTED_EDGE('',*,*,#44901,.T.);
#60805=ORIENTED_EDGE('',*,*,#44899,.T.);
#60806=ORIENTED_EDGE('',*,*,#44896,.T.);
#60807=ORIENTED_EDGE('',*,*,#44748,.T.);
#60808=ORIENTED_EDGE('',*,*,#44819,.T.);
#60809=ORIENTED_EDGE('',*,*,#44466,.T.);
#60810=ORIENTED_EDGE('',*,*,#44881,.T.);
#60811=ORIENTED_EDGE('',*,*,#44689,.T.);
#60812=ORIENTED_EDGE('',*,*,#44679,.F.);
#60813=ORIENTED_EDGE('',*,*,#44922,.T.);
#60814=ORIENTED_EDGE('',*,*,#44742,.T.);
#60815=ORIENTED_EDGE('',*,*,#44922,.F.);
#60816=ORIENTED_EDGE('',*,*,#44841,.F.);
#60817=ORIENTED_EDGE('',*,*,#44923,.T.);
#60818=ORIENTED_EDGE('',*,*,#44904,.T.);
#60819=ORIENTED_EDGE('',*,*,#44923,.F.);
#60820=ORIENTED_EDGE('',*,*,#44878,.T.);
#60821=ORIENTED_EDGE('',*,*,#44924,.T.);
#60822=ORIENTED_EDGE('',*,*,#44906,.T.);
#60823=ORIENTED_EDGE('',*,*,#44924,.F.);
#60824=ORIENTED_EDGE('',*,*,#44876,.T.);
#60825=ORIENTED_EDGE('',*,*,#44925,.T.);
#60826=ORIENTED_EDGE('',*,*,#44787,.T.);
#60827=ORIENTED_EDGE('',*,*,#44565,.T.);
#60828=ORIENTED_EDGE('',*,*,#44773,.F.);
#60829=ORIENTED_EDGE('',*,*,#44788,.F.);
#60830=ORIENTED_EDGE('',*,*,#44925,.F.);
#60831=ORIENTED_EDGE('',*,*,#44875,.F.);
#60832=ORIENTED_EDGE('',*,*,#44926,.F.);
#60833=ORIENTED_EDGE('',*,*,#44919,.F.);
#60834=ORIENTED_EDGE('',*,*,#44909,.F.);
#60835=ORIENTED_EDGE('',*,*,#44726,.T.);
#60836=ORIENTED_EDGE('',*,*,#44920,.F.);
#60837=ORIENTED_EDGE('',*,*,#44926,.T.);
#60838=ORIENTED_EDGE('',*,*,#44874,.T.);
#60839=ORIENTED_EDGE('',*,*,#44927,.T.);
#60840=ORIENTED_EDGE('',*,*,#44928,.F.);
#60841=ORIENTED_EDGE('',*,*,#44921,.F.);
#60842=ORIENTED_EDGE('',*,*,#44927,.F.);
#60843=ORIENTED_EDGE('',*,*,#44873,.F.);
#60844=ORIENTED_EDGE('',*,*,#44917,.F.);
#60845=ORIENTED_EDGE('',*,*,#44928,.T.);
#60846=ORIENTED_EDGE('',*,*,#44872,.T.);
#60847=ORIENTED_EDGE('',*,*,#44929,.T.);
#60848=ORIENTED_EDGE('',*,*,#44929,.F.);
#60849=ORIENTED_EDGE('',*,*,#44871,.F.);
#60850=ORIENTED_EDGE('',*,*,#44930,.F.);
#60851=ORIENTED_EDGE('',*,*,#44761,.F.);
#60852=ORIENTED_EDGE('',*,*,#44911,.F.);
#60853=ORIENTED_EDGE('',*,*,#44918,.F.);
#60854=ORIENTED_EDGE('',*,*,#44762,.F.);
#60855=ORIENTED_EDGE('',*,*,#44930,.T.);
#60856=ORIENTED_EDGE('',*,*,#44870,.F.);
#60857=ORIENTED_EDGE('',*,*,#44813,.F.);
#60858=ORIENTED_EDGE('',*,*,#44931,.F.);
#60859=ORIENTED_EDGE('',*,*,#44932,.F.);
#60860=ORIENTED_EDGE('',*,*,#44933,.T.);
#60861=ORIENTED_EDGE('',*,*,#44934,.F.);
#60862=ORIENTED_EDGE('',*,*,#44933,.F.);
#60863=ORIENTED_EDGE('',*,*,#44935,.F.);
#60864=ORIENTED_EDGE('',*,*,#44936,.F.);
#60865=ORIENTED_EDGE('',*,*,#44936,.T.);
#60866=ORIENTED_EDGE('',*,*,#44937,.F.);
#60867=ORIENTED_EDGE('',*,*,#44938,.F.);
#60868=ORIENTED_EDGE('',*,*,#44931,.T.);
#60869=ORIENTED_EDGE('',*,*,#44934,.T.);
#60870=ORIENTED_EDGE('',*,*,#44938,.T.);
#60871=ORIENTED_EDGE('',*,*,#44939,.T.);
#60872=ORIENTED_EDGE('',*,*,#44932,.T.);
#60873=ORIENTED_EDGE('',*,*,#44939,.F.);
#60874=ORIENTED_EDGE('',*,*,#44937,.T.);
#60875=ORIENTED_EDGE('',*,*,#44935,.T.);
#60876=ORIENTED_EDGE('',*,*,#44940,.T.);
#60877=ORIENTED_EDGE('',*,*,#44941,.T.);
#60878=ORIENTED_EDGE('',*,*,#44942,.T.);
#60879=ORIENTED_EDGE('',*,*,#44943,.T.);
#60880=ORIENTED_EDGE('',*,*,#44940,.F.);
#60881=ORIENTED_EDGE('',*,*,#44944,.T.);
#60882=ORIENTED_EDGE('',*,*,#44945,.F.);
#60883=ORIENTED_EDGE('',*,*,#44946,.T.);
#60884=ORIENTED_EDGE('',*,*,#44947,.F.);
#60885=ORIENTED_EDGE('',*,*,#44948,.T.);
#60886=ORIENTED_EDGE('',*,*,#44949,.F.);
#60887=ORIENTED_EDGE('',*,*,#44950,.T.);
#60888=ORIENTED_EDGE('',*,*,#44951,.F.);
#60889=ORIENTED_EDGE('',*,*,#44952,.T.);
#60890=ORIENTED_EDGE('',*,*,#44953,.F.);
#60891=ORIENTED_EDGE('',*,*,#44954,.T.);
#60892=ORIENTED_EDGE('',*,*,#44955,.F.);
#60893=ORIENTED_EDGE('',*,*,#44956,.T.);
#60894=ORIENTED_EDGE('',*,*,#44957,.T.);
#60895=ORIENTED_EDGE('',*,*,#44958,.T.);
#60896=ORIENTED_EDGE('',*,*,#44959,.F.);
#60897=ORIENTED_EDGE('',*,*,#44960,.T.);
#60898=ORIENTED_EDGE('',*,*,#44961,.F.);
#60899=ORIENTED_EDGE('',*,*,#44962,.T.);
#60900=ORIENTED_EDGE('',*,*,#44943,.F.);
#60901=ORIENTED_EDGE('',*,*,#44963,.F.);
#60902=ORIENTED_EDGE('',*,*,#44964,.F.);
#60903=ORIENTED_EDGE('',*,*,#44944,.F.);
#60904=ORIENTED_EDGE('',*,*,#44945,.T.);
#60905=ORIENTED_EDGE('',*,*,#44964,.T.);
#60906=ORIENTED_EDGE('',*,*,#44965,.T.);
#60907=ORIENTED_EDGE('',*,*,#44966,.T.);
#60908=ORIENTED_EDGE('',*,*,#44966,.F.);
#60909=ORIENTED_EDGE('',*,*,#44967,.F.);
#60910=ORIENTED_EDGE('',*,*,#44968,.F.);
#60911=ORIENTED_EDGE('',*,*,#44969,.F.);
#60912=ORIENTED_EDGE('',*,*,#44970,.F.);
#60913=ORIENTED_EDGE('',*,*,#44946,.F.);
#60914=ORIENTED_EDGE('',*,*,#44971,.T.);
#60915=ORIENTED_EDGE('',*,*,#44972,.T.);
#60916=ORIENTED_EDGE('',*,*,#44973,.T.);
#60917=ORIENTED_EDGE('',*,*,#44974,.T.);
#60918=ORIENTED_EDGE('',*,*,#44975,.T.);
#60919=ORIENTED_EDGE('',*,*,#44976,.T.);
#60920=ORIENTED_EDGE('',*,*,#44973,.F.);
#60921=ORIENTED_EDGE('',*,*,#44977,.T.);
#60922=ORIENTED_EDGE('',*,*,#44978,.T.);
#60923=ORIENTED_EDGE('',*,*,#44969,.T.);
#60924=ORIENTED_EDGE('',*,*,#44975,.F.);
#60925=ORIENTED_EDGE('',*,*,#44979,.T.);
#60926=ORIENTED_EDGE('',*,*,#44980,.T.);
#60927=ORIENTED_EDGE('',*,*,#44981,.T.);
#60928=ORIENTED_EDGE('',*,*,#44978,.F.);
#60929=ORIENTED_EDGE('',*,*,#44982,.T.);
#60930=ORIENTED_EDGE('',*,*,#44983,.T.);
#60931=ORIENTED_EDGE('',*,*,#44984,.T.);
#60932=ORIENTED_EDGE('',*,*,#44980,.F.);
#60933=ORIENTED_EDGE('',*,*,#44985,.T.);
#60934=ORIENTED_EDGE('',*,*,#44986,.T.);
#60935=ORIENTED_EDGE('',*,*,#44987,.T.);
#60936=ORIENTED_EDGE('',*,*,#44983,.F.);
#60937=ORIENTED_EDGE('',*,*,#44988,.T.);
#60938=ORIENTED_EDGE('',*,*,#44989,.T.);
#60939=ORIENTED_EDGE('',*,*,#44990,.T.);
#60940=ORIENTED_EDGE('',*,*,#44986,.F.);
#60941=ORIENTED_EDGE('',*,*,#44991,.T.);
#60942=ORIENTED_EDGE('',*,*,#44971,.F.);
#60943=ORIENTED_EDGE('',*,*,#44992,.T.);
#60944=ORIENTED_EDGE('',*,*,#44989,.F.);
#60945=ORIENTED_EDGE('',*,*,#44993,.T.);
#60946=ORIENTED_EDGE('',*,*,#44987,.F.);
#60947=ORIENTED_EDGE('',*,*,#44994,.T.);
#60948=ORIENTED_EDGE('',*,*,#44995,.F.);
#60949=ORIENTED_EDGE('',*,*,#44996,.T.);
#60950=ORIENTED_EDGE('',*,*,#44990,.F.);
#60951=ORIENTED_EDGE('',*,*,#44997,.F.);
#60952=ORIENTED_EDGE('',*,*,#44998,.F.);
#60953=ORIENTED_EDGE('',*,*,#44994,.F.);
#60954=ORIENTED_EDGE('',*,*,#44992,.F.);
#60955=ORIENTED_EDGE('',*,*,#44999,.T.);
#60956=ORIENTED_EDGE('',*,*,#45000,.T.);
#60957=ORIENTED_EDGE('',*,*,#44997,.T.);
#60958=ORIENTED_EDGE('',*,*,#44974,.F.);
#60959=ORIENTED_EDGE('',*,*,#45001,.F.);
#60960=ORIENTED_EDGE('',*,*,#45002,.F.);
#60961=ORIENTED_EDGE('',*,*,#45003,.F.);
#60962=ORIENTED_EDGE('',*,*,#45004,.T.);
#60963=ORIENTED_EDGE('',*,*,#44999,.F.);
#60964=ORIENTED_EDGE('',*,*,#44972,.F.);
#60965=ORIENTED_EDGE('',*,*,#44993,.F.);
#60966=ORIENTED_EDGE('',*,*,#44991,.F.);
#60967=ORIENTED_EDGE('',*,*,#44988,.F.);
#60968=ORIENTED_EDGE('',*,*,#44985,.F.);
#60969=ORIENTED_EDGE('',*,*,#44982,.F.);
#60970=ORIENTED_EDGE('',*,*,#44979,.F.);
#60971=ORIENTED_EDGE('',*,*,#44977,.F.);
#60972=ORIENTED_EDGE('',*,*,#45005,.T.);
#60973=ORIENTED_EDGE('',*,*,#45006,.T.);
#60974=ORIENTED_EDGE('',*,*,#45007,.T.);
#60975=ORIENTED_EDGE('',*,*,#45008,.T.);
#60976=ORIENTED_EDGE('',*,*,#45009,.T.);
#60977=ORIENTED_EDGE('',*,*,#45010,.T.);
#60978=ORIENTED_EDGE('',*,*,#45011,.T.);
#60979=ORIENTED_EDGE('',*,*,#45012,.T.);
#60980=ORIENTED_EDGE('',*,*,#45013,.T.);
#60981=ORIENTED_EDGE('',*,*,#45014,.T.);
#60982=ORIENTED_EDGE('',*,*,#45010,.F.);
#60983=ORIENTED_EDGE('',*,*,#45015,.T.);
#60984=ORIENTED_EDGE('',*,*,#45016,.T.);
#60985=ORIENTED_EDGE('',*,*,#45013,.F.);
#60986=ORIENTED_EDGE('',*,*,#45017,.T.);
#60987=ORIENTED_EDGE('',*,*,#45008,.F.);
#60988=ORIENTED_EDGE('',*,*,#45018,.T.);
#60989=ORIENTED_EDGE('',*,*,#45019,.T.);
#60990=ORIENTED_EDGE('',*,*,#45020,.T.);
#60991=ORIENTED_EDGE('',*,*,#45021,.T.);
#60992=ORIENTED_EDGE('',*,*,#45022,.T.);
#60993=ORIENTED_EDGE('',*,*,#45019,.F.);
#60994=ORIENTED_EDGE('',*,*,#45023,.T.);
#60995=ORIENTED_EDGE('',*,*,#45012,.F.);
#60996=ORIENTED_EDGE('',*,*,#45024,.T.);
#60997=ORIENTED_EDGE('',*,*,#45006,.F.);
#60998=ORIENTED_EDGE('',*,*,#45025,.T.);
#60999=ORIENTED_EDGE('',*,*,#45026,.T.);
#61000=ORIENTED_EDGE('',*,*,#45027,.T.);
#61001=ORIENTED_EDGE('',*,*,#45026,.F.);
#61002=ORIENTED_EDGE('',*,*,#45028,.T.);
#61003=ORIENTED_EDGE('',*,*,#45021,.F.);
#61004=ORIENTED_EDGE('',*,*,#45007,.F.);
#61005=ORIENTED_EDGE('',*,*,#45029,.F.);
#61006=ORIENTED_EDGE('',*,*,#45030,.F.);
#61007=ORIENTED_EDGE('',*,*,#45031,.F.);
#61008=ORIENTED_EDGE('',*,*,#45024,.F.);
#61009=ORIENTED_EDGE('',*,*,#45032,.T.);
#61010=ORIENTED_EDGE('',*,*,#45033,.F.);
#61011=ORIENTED_EDGE('',*,*,#45029,.T.);
#61012=ORIENTED_EDGE('',*,*,#45027,.F.);
#61013=ORIENTED_EDGE('',*,*,#45034,.F.);
#61014=ORIENTED_EDGE('',*,*,#45035,.F.);
#61015=ORIENTED_EDGE('',*,*,#45032,.F.);
#61016=ORIENTED_EDGE('',*,*,#45020,.F.);
#61017=ORIENTED_EDGE('',*,*,#45036,.F.);
#61018=ORIENTED_EDGE('',*,*,#45037,.F.);
#61019=ORIENTED_EDGE('',*,*,#45034,.T.);
#61020=ORIENTED_EDGE('',*,*,#45018,.F.);
#61021=ORIENTED_EDGE('',*,*,#45028,.F.);
#61022=ORIENTED_EDGE('',*,*,#45025,.F.);
#61023=ORIENTED_EDGE('',*,*,#45005,.F.);
#61024=ORIENTED_EDGE('',*,*,#45017,.F.);
#61025=ORIENTED_EDGE('',*,*,#45015,.F.);
#61026=ORIENTED_EDGE('',*,*,#45009,.F.);
#61027=ORIENTED_EDGE('',*,*,#45023,.F.);
#61028=ORIENTED_EDGE('',*,*,#45038,.F.);
#61029=ORIENTED_EDGE('',*,*,#45039,.T.);
#61030=ORIENTED_EDGE('',*,*,#45040,.T.);
#61031=ORIENTED_EDGE('',*,*,#45041,.T.);
#61032=ORIENTED_EDGE('',*,*,#45042,.F.);
#61033=ORIENTED_EDGE('',*,*,#45043,.T.);
#61034=ORIENTED_EDGE('',*,*,#45044,.T.);
#61035=ORIENTED_EDGE('',*,*,#45040,.F.);
#61036=ORIENTED_EDGE('',*,*,#45045,.T.);
#61037=ORIENTED_EDGE('',*,*,#45046,.F.);
#61038=ORIENTED_EDGE('',*,*,#45047,.T.);
#61039=ORIENTED_EDGE('',*,*,#45048,.F.);
#61040=ORIENTED_EDGE('',*,*,#45049,.T.);
#61041=ORIENTED_EDGE('',*,*,#45043,.F.);
#61042=ORIENTED_EDGE('',*,*,#45050,.T.);
#61043=ORIENTED_EDGE('',*,*,#45051,.F.);
#61044=ORIENTED_EDGE('',*,*,#45041,.F.);
#61045=ORIENTED_EDGE('',*,*,#45052,.F.);
#61046=ORIENTED_EDGE('',*,*,#45053,.F.);
#61047=ORIENTED_EDGE('',*,*,#45054,.F.);
#61048=ORIENTED_EDGE('',*,*,#45055,.F.);
#61049=ORIENTED_EDGE('',*,*,#45056,.F.);
#61050=ORIENTED_EDGE('',*,*,#45057,.F.);
#61051=ORIENTED_EDGE('',*,*,#45058,.F.);
#61052=ORIENTED_EDGE('',*,*,#45059,.T.);
#61053=ORIENTED_EDGE('',*,*,#45060,.T.);
#61054=ORIENTED_EDGE('',*,*,#45061,.T.);
#61055=ORIENTED_EDGE('',*,*,#45062,.T.);
#61056=ORIENTED_EDGE('',*,*,#45063,.T.);
#61057=ORIENTED_EDGE('',*,*,#45044,.F.);
#61058=ORIENTED_EDGE('',*,*,#45064,.T.);
#61059=ORIENTED_EDGE('',*,*,#45065,.F.);
#61060=ORIENTED_EDGE('',*,*,#45052,.T.);
#61061=ORIENTED_EDGE('',*,*,#45049,.F.);
#61062=ORIENTED_EDGE('',*,*,#45066,.T.);
#61063=ORIENTED_EDGE('',*,*,#45067,.F.);
#61064=ORIENTED_EDGE('',*,*,#45068,.T.);
#61065=ORIENTED_EDGE('',*,*,#45069,.T.);
#61066=ORIENTED_EDGE('',*,*,#45070,.F.);
#61067=ORIENTED_EDGE('',*,*,#45064,.F.);
#61068=ORIENTED_EDGE('',*,*,#45048,.T.);
#61069=ORIENTED_EDGE('',*,*,#45071,.T.);
#61070=ORIENTED_EDGE('',*,*,#45072,.T.);
#61071=ORIENTED_EDGE('',*,*,#45073,.T.);
#61072=ORIENTED_EDGE('',*,*,#45047,.F.);
#61073=ORIENTED_EDGE('',*,*,#45074,.F.);
#61074=ORIENTED_EDGE('',*,*,#45075,.F.);
#61075=ORIENTED_EDGE('',*,*,#45076,.F.);
#61076=ORIENTED_EDGE('',*,*,#45071,.F.);
#61077=ORIENTED_EDGE('',*,*,#45046,.T.);
#61078=ORIENTED_EDGE('',*,*,#45077,.F.);
#61079=ORIENTED_EDGE('',*,*,#45078,.T.);
#61080=ORIENTED_EDGE('',*,*,#45079,.F.);
#61081=ORIENTED_EDGE('',*,*,#45080,.T.);
#61082=ORIENTED_EDGE('',*,*,#45081,.T.);
#61083=ORIENTED_EDGE('',*,*,#45082,.T.);
#61084=ORIENTED_EDGE('',*,*,#45083,.F.);
#61085=ORIENTED_EDGE('',*,*,#45084,.T.);
#61086=ORIENTED_EDGE('',*,*,#45074,.T.);
#61087=ORIENTED_EDGE('',*,*,#45085,.T.);
#61088=ORIENTED_EDGE('',*,*,#45086,.T.);
#61089=ORIENTED_EDGE('',*,*,#45072,.F.);
#61090=ORIENTED_EDGE('',*,*,#45076,.T.);
#61091=ORIENTED_EDGE('',*,*,#45084,.F.);
#61092=ORIENTED_EDGE('',*,*,#45087,.T.);
#61093=ORIENTED_EDGE('',*,*,#45085,.F.);
#61094=ORIENTED_EDGE('',*,*,#45075,.T.);
#61095=ORIENTED_EDGE('',*,*,#45073,.F.);
#61096=ORIENTED_EDGE('',*,*,#45088,.F.);
#61097=ORIENTED_EDGE('',*,*,#45089,.T.);
#61098=ORIENTED_EDGE('',*,*,#45090,.F.);
#61099=ORIENTED_EDGE('',*,*,#45091,.F.);
#61100=ORIENTED_EDGE('',*,*,#45092,.F.);
#61101=ORIENTED_EDGE('',*,*,#45066,.F.);
#61102=ORIENTED_EDGE('',*,*,#45093,.T.);
#61103=ORIENTED_EDGE('',*,*,#45086,.F.);
#61104=ORIENTED_EDGE('',*,*,#45094,.T.);
#61105=ORIENTED_EDGE('',*,*,#45095,.T.);
#61106=ORIENTED_EDGE('',*,*,#45088,.T.);
#61107=ORIENTED_EDGE('',*,*,#45087,.F.);
#61108=ORIENTED_EDGE('',*,*,#45083,.T.);
#61109=ORIENTED_EDGE('',*,*,#45096,.F.);
#61110=ORIENTED_EDGE('',*,*,#45097,.F.);
#61111=ORIENTED_EDGE('',*,*,#45098,.T.);
#61112=ORIENTED_EDGE('',*,*,#45099,.F.);
#61113=ORIENTED_EDGE('',*,*,#45100,.F.);
#61114=ORIENTED_EDGE('',*,*,#45101,.F.);
#61115=ORIENTED_EDGE('',*,*,#44960,.F.);
#61116=ORIENTED_EDGE('',*,*,#45102,.F.);
#61117=ORIENTED_EDGE('',*,*,#45103,.F.);
#61118=ORIENTED_EDGE('',*,*,#45104,.F.);
#61119=ORIENTED_EDGE('',*,*,#45105,.F.);
#61120=ORIENTED_EDGE('',*,*,#45106,.T.);
#61121=ORIENTED_EDGE('',*,*,#45107,.F.);
#61122=ORIENTED_EDGE('',*,*,#45094,.F.);
#61123=ORIENTED_EDGE('',*,*,#45051,.T.);
#61124=ORIENTED_EDGE('',*,*,#45108,.T.);
#61125=ORIENTED_EDGE('',*,*,#45109,.T.);
#61126=ORIENTED_EDGE('',*,*,#45110,.T.);
#61127=ORIENTED_EDGE('',*,*,#45077,.T.);
#61128=ORIENTED_EDGE('',*,*,#45038,.T.);
#61129=ORIENTED_EDGE('',*,*,#45111,.T.);
#61130=ORIENTED_EDGE('',*,*,#45112,.T.);
#61131=ORIENTED_EDGE('',*,*,#45109,.F.);
#61132=ORIENTED_EDGE('',*,*,#45113,.T.);
#61133=ORIENTED_EDGE('',*,*,#45110,.F.);
#61134=ORIENTED_EDGE('',*,*,#45114,.T.);
#61135=ORIENTED_EDGE('',*,*,#45115,.F.);
#61136=ORIENTED_EDGE('',*,*,#45078,.F.);
#61137=ORIENTED_EDGE('',*,*,#45112,.F.);
#61138=ORIENTED_EDGE('',*,*,#45116,.T.);
#61139=ORIENTED_EDGE('',*,*,#45117,.F.);
#61140=ORIENTED_EDGE('',*,*,#45114,.F.);
#61141=ORIENTED_EDGE('',*,*,#45118,.T.);
#61142=ORIENTED_EDGE('',*,*,#45119,.T.);
#61143=ORIENTED_EDGE('',*,*,#45120,.T.);
#61144=ORIENTED_EDGE('',*,*,#45121,.F.);
#61145=ORIENTED_EDGE('',*,*,#45122,.T.);
#61146=ORIENTED_EDGE('',*,*,#45123,.T.);
#61147=ORIENTED_EDGE('',*,*,#45119,.F.);
#61148=ORIENTED_EDGE('',*,*,#45124,.T.);
#61149=ORIENTED_EDGE('',*,*,#45125,.T.);
#61150=ORIENTED_EDGE('',*,*,#45126,.T.);
#61151=ORIENTED_EDGE('',*,*,#45122,.F.);
#61152=ORIENTED_EDGE('',*,*,#45127,.T.);
#61153=ORIENTED_EDGE('',*,*,#45128,.T.);
#61154=ORIENTED_EDGE('',*,*,#45129,.T.);
#61155=ORIENTED_EDGE('',*,*,#45125,.F.);
#61156=ORIENTED_EDGE('',*,*,#45130,.T.);
#61157=ORIENTED_EDGE('',*,*,#45131,.T.);
#61158=ORIENTED_EDGE('',*,*,#45128,.F.);
#61159=ORIENTED_EDGE('',*,*,#45132,.T.);
#61160=ORIENTED_EDGE('',*,*,#45133,.T.);
#61161=ORIENTED_EDGE('',*,*,#45134,.T.);
#61162=ORIENTED_EDGE('',*,*,#45133,.F.);
#61163=ORIENTED_EDGE('',*,*,#45135,.T.);
#61164=ORIENTED_EDGE('',*,*,#45121,.T.);
#61165=ORIENTED_EDGE('',*,*,#45131,.F.);
#61166=ORIENTED_EDGE('',*,*,#45136,.T.);
#61167=ORIENTED_EDGE('',*,*,#45137,.F.);
#61168=ORIENTED_EDGE('',*,*,#45138,.F.);
#61169=ORIENTED_EDGE('',*,*,#45139,.F.);
#61170=ORIENTED_EDGE('',*,*,#45140,.F.);
#61171=ORIENTED_EDGE('',*,*,#45134,.F.);
#61172=ORIENTED_EDGE('',*,*,#45141,.T.);
#61173=ORIENTED_EDGE('',*,*,#45142,.F.);
#61174=ORIENTED_EDGE('',*,*,#45143,.F.);
#61175=ORIENTED_EDGE('',*,*,#45144,.F.);
#61176=ORIENTED_EDGE('',*,*,#45145,.T.);
#61177=ORIENTED_EDGE('',*,*,#45136,.F.);
#61178=ORIENTED_EDGE('',*,*,#45120,.F.);
#61179=ORIENTED_EDGE('',*,*,#45146,.F.);
#61180=ORIENTED_EDGE('',*,*,#45147,.F.);
#61181=ORIENTED_EDGE('',*,*,#45141,.F.);
#61182=ORIENTED_EDGE('',*,*,#45118,.F.);
#61183=ORIENTED_EDGE('',*,*,#45135,.F.);
#61184=ORIENTED_EDGE('',*,*,#45132,.F.);
#61185=ORIENTED_EDGE('',*,*,#45130,.F.);
#61186=ORIENTED_EDGE('',*,*,#45127,.F.);
#61187=ORIENTED_EDGE('',*,*,#45124,.F.);
#61188=ORIENTED_EDGE('',*,*,#45148,.F.);
#61189=ORIENTED_EDGE('',*,*,#45149,.T.);
#61190=ORIENTED_EDGE('',*,*,#45150,.F.);
#61191=ORIENTED_EDGE('',*,*,#45151,.F.);
#61192=ORIENTED_EDGE('',*,*,#45152,.T.);
#61193=ORIENTED_EDGE('',*,*,#45153,.F.);
#61194=ORIENTED_EDGE('',*,*,#45154,.F.);
#61195=ORIENTED_EDGE('',*,*,#45155,.F.);
#61196=ORIENTED_EDGE('',*,*,#45155,.T.);
#61197=ORIENTED_EDGE('',*,*,#45156,.T.);
#61198=ORIENTED_EDGE('',*,*,#45157,.T.);
#61199=ORIENTED_EDGE('',*,*,#45154,.T.);
#61200=ORIENTED_EDGE('',*,*,#45158,.T.);
#61201=ORIENTED_EDGE('',*,*,#45159,.T.);
#61202=ORIENTED_EDGE('',*,*,#45156,.F.);
#61203=ORIENTED_EDGE('',*,*,#45153,.T.);
#61204=ORIENTED_EDGE('',*,*,#45160,.T.);
#61205=ORIENTED_EDGE('',*,*,#45161,.T.);
#61206=ORIENTED_EDGE('',*,*,#45162,.T.);
#61207=ORIENTED_EDGE('',*,*,#45158,.F.);
#61208=ORIENTED_EDGE('',*,*,#45152,.F.);
#61209=ORIENTED_EDGE('',*,*,#45163,.F.);
#61210=ORIENTED_EDGE('',*,*,#45164,.F.);
#61211=ORIENTED_EDGE('',*,*,#45165,.F.);
#61212=ORIENTED_EDGE('',*,*,#45166,.F.);
#61213=ORIENTED_EDGE('',*,*,#45167,.F.);
#61214=ORIENTED_EDGE('',*,*,#45168,.F.);
#61215=ORIENTED_EDGE('',*,*,#45169,.F.);
#61216=ORIENTED_EDGE('',*,*,#45160,.F.);
#61217=ORIENTED_EDGE('',*,*,#45170,.T.);
#61218=ORIENTED_EDGE('',*,*,#45171,.T.);
#61219=ORIENTED_EDGE('',*,*,#45161,.F.);
#61220=ORIENTED_EDGE('',*,*,#45169,.T.);
#61221=ORIENTED_EDGE('',*,*,#45172,.T.);
#61222=ORIENTED_EDGE('',*,*,#45173,.T.);
#61223=ORIENTED_EDGE('',*,*,#45170,.F.);
#61224=ORIENTED_EDGE('',*,*,#45168,.T.);
#61225=ORIENTED_EDGE('',*,*,#45174,.T.);
#61226=ORIENTED_EDGE('',*,*,#45175,.T.);
#61227=ORIENTED_EDGE('',*,*,#45172,.F.);
#61228=ORIENTED_EDGE('',*,*,#45167,.T.);
#61229=ORIENTED_EDGE('',*,*,#45176,.T.);
#61230=ORIENTED_EDGE('',*,*,#45177,.T.);
#61231=ORIENTED_EDGE('',*,*,#45174,.F.);
#61232=ORIENTED_EDGE('',*,*,#45166,.T.);
#61233=ORIENTED_EDGE('',*,*,#45178,.T.);
#61234=ORIENTED_EDGE('',*,*,#45179,.T.);
#61235=ORIENTED_EDGE('',*,*,#45176,.F.);
#61236=ORIENTED_EDGE('',*,*,#45165,.T.);
#61237=ORIENTED_EDGE('',*,*,#45180,.T.);
#61238=ORIENTED_EDGE('',*,*,#45181,.T.);
#61239=ORIENTED_EDGE('',*,*,#45178,.F.);
#61240=ORIENTED_EDGE('',*,*,#45164,.T.);
#61241=ORIENTED_EDGE('',*,*,#45151,.T.);
#61242=ORIENTED_EDGE('',*,*,#45182,.T.);
#61243=ORIENTED_EDGE('',*,*,#45180,.F.);
#61244=ORIENTED_EDGE('',*,*,#45163,.T.);
#61245=ORIENTED_EDGE('',*,*,#45148,.T.);
#61246=ORIENTED_EDGE('',*,*,#45157,.F.);
#61247=ORIENTED_EDGE('',*,*,#45183,.T.);
#61248=ORIENTED_EDGE('',*,*,#45184,.F.);
#61249=ORIENTED_EDGE('',*,*,#45185,.T.);
#61250=ORIENTED_EDGE('',*,*,#45186,.F.);
#61251=ORIENTED_EDGE('',*,*,#45159,.F.);
#61252=ORIENTED_EDGE('',*,*,#45187,.F.);
#61253=ORIENTED_EDGE('',*,*,#45188,.F.);
#61254=ORIENTED_EDGE('',*,*,#45183,.F.);
#61255=ORIENTED_EDGE('',*,*,#45162,.F.);
#61256=ORIENTED_EDGE('',*,*,#45189,.F.);
#61257=ORIENTED_EDGE('',*,*,#45190,.F.);
#61258=ORIENTED_EDGE('',*,*,#45187,.T.);
#61259=ORIENTED_EDGE('',*,*,#45171,.F.);
#61260=ORIENTED_EDGE('',*,*,#45191,.F.);
#61261=ORIENTED_EDGE('',*,*,#45192,.F.);
#61262=ORIENTED_EDGE('',*,*,#45189,.T.);
#61263=ORIENTED_EDGE('',*,*,#45173,.F.);
#61264=ORIENTED_EDGE('',*,*,#45193,.T.);
#61265=ORIENTED_EDGE('',*,*,#45194,.T.);
#61266=ORIENTED_EDGE('',*,*,#45191,.T.);
#61267=ORIENTED_EDGE('',*,*,#45175,.F.);
#61268=ORIENTED_EDGE('',*,*,#45195,.F.);
#61269=ORIENTED_EDGE('',*,*,#45196,.F.);
#61270=ORIENTED_EDGE('',*,*,#45193,.F.);
#61271=ORIENTED_EDGE('',*,*,#45177,.F.);
#61272=ORIENTED_EDGE('',*,*,#45197,.T.);
#61273=ORIENTED_EDGE('',*,*,#45198,.T.);
#61274=ORIENTED_EDGE('',*,*,#45195,.T.);
#61275=ORIENTED_EDGE('',*,*,#45179,.F.);
#61276=ORIENTED_EDGE('',*,*,#45199,.F.);
#61277=ORIENTED_EDGE('',*,*,#45200,.F.);
#61278=ORIENTED_EDGE('',*,*,#45197,.F.);
#61279=ORIENTED_EDGE('',*,*,#45181,.F.);
#61280=ORIENTED_EDGE('',*,*,#45201,.T.);
#61281=ORIENTED_EDGE('',*,*,#45202,.T.);
#61282=ORIENTED_EDGE('',*,*,#45199,.T.);
#61283=ORIENTED_EDGE('',*,*,#45150,.T.);
#61284=ORIENTED_EDGE('',*,*,#45203,.T.);
#61285=ORIENTED_EDGE('',*,*,#45185,.F.);
#61286=ORIENTED_EDGE('',*,*,#45204,.T.);
#61287=ORIENTED_EDGE('',*,*,#45205,.T.);
#61288=ORIENTED_EDGE('',*,*,#45206,.F.);
#61289=ORIENTED_EDGE('',*,*,#45207,.F.);
#61290=ORIENTED_EDGE('',*,*,#45208,.T.);
#61291=ORIENTED_EDGE('',*,*,#45209,.F.);
#61292=ORIENTED_EDGE('',*,*,#45210,.T.);
#61293=ORIENTED_EDGE('',*,*,#45211,.F.);
#61294=ORIENTED_EDGE('',*,*,#45212,.F.);
#61295=ORIENTED_EDGE('',*,*,#45213,.T.);
#61296=ORIENTED_EDGE('',*,*,#45201,.F.);
#61297=ORIENTED_EDGE('',*,*,#45182,.F.);
#61298=ORIENTED_EDGE('',*,*,#45149,.F.);
#61299=ORIENTED_EDGE('',*,*,#45186,.T.);
#61300=ORIENTED_EDGE('',*,*,#45203,.F.);
#61301=ORIENTED_EDGE('',*,*,#45214,.T.);
#61302=ORIENTED_EDGE('',*,*,#45215,.T.);
#61303=ORIENTED_EDGE('',*,*,#45216,.T.);
#61304=ORIENTED_EDGE('',*,*,#45217,.T.);
#61305=ORIENTED_EDGE('',*,*,#45218,.T.);
#61306=ORIENTED_EDGE('',*,*,#45219,.T.);
#61307=ORIENTED_EDGE('',*,*,#45216,.F.);
#61308=ORIENTED_EDGE('',*,*,#45220,.T.);
#61309=ORIENTED_EDGE('',*,*,#45221,.T.);
#61310=ORIENTED_EDGE('',*,*,#45222,.T.);
#61311=ORIENTED_EDGE('',*,*,#45218,.F.);
#61312=ORIENTED_EDGE('',*,*,#45223,.T.);
#61313=ORIENTED_EDGE('',*,*,#45224,.T.);
#61314=ORIENTED_EDGE('',*,*,#45225,.T.);
#61315=ORIENTED_EDGE('',*,*,#45221,.F.);
#61316=ORIENTED_EDGE('',*,*,#45226,.T.);
#61317=ORIENTED_EDGE('',*,*,#45227,.T.);
#61318=ORIENTED_EDGE('',*,*,#45228,.T.);
#61319=ORIENTED_EDGE('',*,*,#45224,.F.);
#61320=ORIENTED_EDGE('',*,*,#45229,.T.);
#61321=ORIENTED_EDGE('',*,*,#45230,.T.);
#61322=ORIENTED_EDGE('',*,*,#45231,.T.);
#61323=ORIENTED_EDGE('',*,*,#45227,.F.);
#61324=ORIENTED_EDGE('',*,*,#45232,.T.);
#61325=ORIENTED_EDGE('',*,*,#45233,.T.);
#61326=ORIENTED_EDGE('',*,*,#45234,.T.);
#61327=ORIENTED_EDGE('',*,*,#45235,.T.);
#61328=ORIENTED_EDGE('',*,*,#45236,.T.);
#61329=ORIENTED_EDGE('',*,*,#45237,.T.);
#61330=ORIENTED_EDGE('',*,*,#45238,.T.);
#61331=ORIENTED_EDGE('',*,*,#45235,.F.);
#61332=ORIENTED_EDGE('',*,*,#45239,.T.);
#61333=ORIENTED_EDGE('',*,*,#45240,.T.);
#61334=ORIENTED_EDGE('',*,*,#45241,.T.);
#61335=ORIENTED_EDGE('',*,*,#45237,.F.);
#61336=ORIENTED_EDGE('',*,*,#45242,.T.);
#61337=ORIENTED_EDGE('',*,*,#45243,.T.);
#61338=ORIENTED_EDGE('',*,*,#45244,.T.);
#61339=ORIENTED_EDGE('',*,*,#45240,.F.);
#61340=ORIENTED_EDGE('',*,*,#45245,.T.);
#61341=ORIENTED_EDGE('',*,*,#45233,.F.);
#61342=ORIENTED_EDGE('',*,*,#45246,.T.);
#61343=ORIENTED_EDGE('',*,*,#45230,.F.);
#61344=ORIENTED_EDGE('',*,*,#45247,.T.);
#61345=ORIENTED_EDGE('',*,*,#45214,.F.);
#61346=ORIENTED_EDGE('',*,*,#45248,.T.);
#61347=ORIENTED_EDGE('',*,*,#45243,.F.);
#61348=ORIENTED_EDGE('',*,*,#45222,.F.);
#61349=ORIENTED_EDGE('',*,*,#45249,.F.);
#61350=ORIENTED_EDGE('',*,*,#45250,.F.);
#61351=ORIENTED_EDGE('',*,*,#45251,.F.);
#61352=ORIENTED_EDGE('',*,*,#45225,.F.);
#61353=ORIENTED_EDGE('',*,*,#45252,.T.);
#61354=ORIENTED_EDGE('',*,*,#45253,.T.);
#61355=ORIENTED_EDGE('',*,*,#45249,.T.);
#61356=ORIENTED_EDGE('',*,*,#45228,.F.);
#61357=ORIENTED_EDGE('',*,*,#45254,.F.);
#61358=ORIENTED_EDGE('',*,*,#45255,.F.);
#61359=ORIENTED_EDGE('',*,*,#45252,.F.);
#61360=ORIENTED_EDGE('',*,*,#45231,.F.);
#61361=ORIENTED_EDGE('',*,*,#45256,.T.);
#61362=ORIENTED_EDGE('',*,*,#45257,.T.);
#61363=ORIENTED_EDGE('',*,*,#45254,.T.);
#61364=ORIENTED_EDGE('',*,*,#45246,.F.);
#61365=ORIENTED_EDGE('',*,*,#45258,.F.);
#61366=ORIENTED_EDGE('',*,*,#45259,.F.);
#61367=ORIENTED_EDGE('',*,*,#45256,.F.);
#61368=ORIENTED_EDGE('',*,*,#45236,.F.);
#61369=ORIENTED_EDGE('',*,*,#45260,.F.);
#61370=ORIENTED_EDGE('',*,*,#45261,.F.);
#61371=ORIENTED_EDGE('',*,*,#45258,.T.);
#61372=ORIENTED_EDGE('',*,*,#45234,.F.);
#61373=ORIENTED_EDGE('',*,*,#45247,.F.);
#61374=ORIENTED_EDGE('',*,*,#45232,.F.);
#61375=ORIENTED_EDGE('',*,*,#45229,.F.);
#61376=ORIENTED_EDGE('',*,*,#45226,.F.);
#61377=ORIENTED_EDGE('',*,*,#45223,.F.);
#61378=ORIENTED_EDGE('',*,*,#45220,.F.);
#61379=ORIENTED_EDGE('',*,*,#45215,.F.);
#61380=ORIENTED_EDGE('',*,*,#45245,.F.);
#61381=ORIENTED_EDGE('',*,*,#45242,.F.);
#61382=ORIENTED_EDGE('',*,*,#45239,.F.);
#61383=ORIENTED_EDGE('',*,*,#45262,.T.);
#61384=ORIENTED_EDGE('',*,*,#45263,.T.);
#61385=ORIENTED_EDGE('',*,*,#45264,.T.);
#61386=ORIENTED_EDGE('',*,*,#45265,.T.);
#61387=ORIENTED_EDGE('',*,*,#45266,.T.);
#61388=ORIENTED_EDGE('',*,*,#45267,.T.);
#61389=ORIENTED_EDGE('',*,*,#45264,.F.);
#61390=ORIENTED_EDGE('',*,*,#45268,.T.);
#61391=ORIENTED_EDGE('',*,*,#45269,.T.);
#61392=ORIENTED_EDGE('',*,*,#45270,.T.);
#61393=ORIENTED_EDGE('',*,*,#45266,.F.);
#61394=ORIENTED_EDGE('',*,*,#45271,.T.);
#61395=ORIENTED_EDGE('',*,*,#45272,.T.);
#61396=ORIENTED_EDGE('',*,*,#45273,.T.);
#61397=ORIENTED_EDGE('',*,*,#45269,.F.);
#61398=ORIENTED_EDGE('',*,*,#45274,.T.);
#61399=ORIENTED_EDGE('',*,*,#45275,.T.);
#61400=ORIENTED_EDGE('',*,*,#45276,.T.);
#61401=ORIENTED_EDGE('',*,*,#45272,.F.);
#61402=ORIENTED_EDGE('',*,*,#45277,.T.);
#61403=ORIENTED_EDGE('',*,*,#45278,.T.);
#61404=ORIENTED_EDGE('',*,*,#45279,.T.);
#61405=ORIENTED_EDGE('',*,*,#45275,.F.);
#61406=ORIENTED_EDGE('',*,*,#45280,.T.);
#61407=ORIENTED_EDGE('',*,*,#45281,.T.);
#61408=ORIENTED_EDGE('',*,*,#45282,.T.);
#61409=ORIENTED_EDGE('',*,*,#45278,.F.);
#61410=ORIENTED_EDGE('',*,*,#45283,.T.);
#61411=ORIENTED_EDGE('',*,*,#45284,.T.);
#61412=ORIENTED_EDGE('',*,*,#45285,.T.);
#61413=ORIENTED_EDGE('',*,*,#45281,.F.);
#61414=ORIENTED_EDGE('',*,*,#45286,.T.);
#61415=ORIENTED_EDGE('',*,*,#45287,.T.);
#61416=ORIENTED_EDGE('',*,*,#45288,.T.);
#61417=ORIENTED_EDGE('',*,*,#45284,.F.);
#61418=ORIENTED_EDGE('',*,*,#45289,.T.);
#61419=ORIENTED_EDGE('',*,*,#45290,.T.);
#61420=ORIENTED_EDGE('',*,*,#45291,.T.);
#61421=ORIENTED_EDGE('',*,*,#45287,.F.);
#61422=ORIENTED_EDGE('',*,*,#45292,.T.);
#61423=ORIENTED_EDGE('',*,*,#45293,.T.);
#61424=ORIENTED_EDGE('',*,*,#45294,.T.);
#61425=ORIENTED_EDGE('',*,*,#45290,.F.);
#61426=ORIENTED_EDGE('',*,*,#45295,.T.);
#61427=ORIENTED_EDGE('',*,*,#45262,.F.);
#61428=ORIENTED_EDGE('',*,*,#45296,.T.);
#61429=ORIENTED_EDGE('',*,*,#45293,.F.);
#61430=ORIENTED_EDGE('',*,*,#45297,.T.);
#61431=ORIENTED_EDGE('',*,*,#45285,.F.);
#61432=ORIENTED_EDGE('',*,*,#45298,.T.);
#61433=ORIENTED_EDGE('',*,*,#45299,.T.);
#61434=ORIENTED_EDGE('',*,*,#45300,.T.);
#61435=ORIENTED_EDGE('',*,*,#45288,.F.);
#61436=ORIENTED_EDGE('',*,*,#45301,.F.);
#61437=ORIENTED_EDGE('',*,*,#45302,.F.);
#61438=ORIENTED_EDGE('',*,*,#45298,.F.);
#61439=ORIENTED_EDGE('',*,*,#45291,.F.);
#61440=ORIENTED_EDGE('',*,*,#45303,.T.);
#61441=ORIENTED_EDGE('',*,*,#45304,.T.);
#61442=ORIENTED_EDGE('',*,*,#45301,.T.);
#61443=ORIENTED_EDGE('',*,*,#45294,.F.);
#61444=ORIENTED_EDGE('',*,*,#45305,.F.);
#61445=ORIENTED_EDGE('',*,*,#45306,.F.);
#61446=ORIENTED_EDGE('',*,*,#45303,.F.);
#61447=ORIENTED_EDGE('',*,*,#45296,.F.);
#61448=ORIENTED_EDGE('',*,*,#45307,.T.);
#61449=ORIENTED_EDGE('',*,*,#45308,.T.);
#61450=ORIENTED_EDGE('',*,*,#45305,.T.);
#61451=ORIENTED_EDGE('',*,*,#45265,.F.);
#61452=ORIENTED_EDGE('',*,*,#45309,.F.);
#61453=ORIENTED_EDGE('',*,*,#45310,.F.);
#61454=ORIENTED_EDGE('',*,*,#45307,.F.);
#61455=ORIENTED_EDGE('',*,*,#45263,.F.);
#61456=ORIENTED_EDGE('',*,*,#45297,.F.);
#61457=ORIENTED_EDGE('',*,*,#45295,.F.);
#61458=ORIENTED_EDGE('',*,*,#45292,.F.);
#61459=ORIENTED_EDGE('',*,*,#45289,.F.);
#61460=ORIENTED_EDGE('',*,*,#45286,.F.);
#61461=ORIENTED_EDGE('',*,*,#45283,.F.);
#61462=ORIENTED_EDGE('',*,*,#45280,.F.);
#61463=ORIENTED_EDGE('',*,*,#45277,.F.);
#61464=ORIENTED_EDGE('',*,*,#45274,.F.);
#61465=ORIENTED_EDGE('',*,*,#45271,.F.);
#61466=ORIENTED_EDGE('',*,*,#45268,.F.);
#61467=ORIENTED_EDGE('',*,*,#45311,.T.);
#61468=ORIENTED_EDGE('',*,*,#45312,.T.);
#61469=ORIENTED_EDGE('',*,*,#45313,.T.);
#61470=ORIENTED_EDGE('',*,*,#45314,.T.);
#61471=ORIENTED_EDGE('',*,*,#45315,.T.);
#61472=ORIENTED_EDGE('',*,*,#45316,.T.);
#61473=ORIENTED_EDGE('',*,*,#45313,.F.);
#61474=ORIENTED_EDGE('',*,*,#45317,.T.);
#61475=ORIENTED_EDGE('',*,*,#45318,.T.);
#61476=ORIENTED_EDGE('',*,*,#45319,.T.);
#61477=ORIENTED_EDGE('',*,*,#45315,.F.);
#61478=ORIENTED_EDGE('',*,*,#45320,.T.);
#61479=ORIENTED_EDGE('',*,*,#45321,.T.);
#61480=ORIENTED_EDGE('',*,*,#45322,.T.);
#61481=ORIENTED_EDGE('',*,*,#45318,.F.);
#61482=ORIENTED_EDGE('',*,*,#45323,.T.);
#61483=ORIENTED_EDGE('',*,*,#45324,.T.);
#61484=ORIENTED_EDGE('',*,*,#45325,.T.);
#61485=ORIENTED_EDGE('',*,*,#45321,.F.);
#61486=ORIENTED_EDGE('',*,*,#45326,.T.);
#61487=ORIENTED_EDGE('',*,*,#45327,.T.);
#61488=ORIENTED_EDGE('',*,*,#45328,.T.);
#61489=ORIENTED_EDGE('',*,*,#45324,.F.);
#61490=ORIENTED_EDGE('',*,*,#45329,.T.);
#61491=ORIENTED_EDGE('',*,*,#45330,.T.);
#61492=ORIENTED_EDGE('',*,*,#45331,.T.);
#61493=ORIENTED_EDGE('',*,*,#45327,.F.);
#61494=ORIENTED_EDGE('',*,*,#45332,.T.);
#61495=ORIENTED_EDGE('',*,*,#45333,.T.);
#61496=ORIENTED_EDGE('',*,*,#45334,.T.);
#61497=ORIENTED_EDGE('',*,*,#45330,.F.);
#61498=ORIENTED_EDGE('',*,*,#45335,.T.);
#61499=ORIENTED_EDGE('',*,*,#45336,.T.);
#61500=ORIENTED_EDGE('',*,*,#45337,.T.);
#61501=ORIENTED_EDGE('',*,*,#45333,.F.);
#61502=ORIENTED_EDGE('',*,*,#45338,.T.);
#61503=ORIENTED_EDGE('',*,*,#45339,.T.);
#61504=ORIENTED_EDGE('',*,*,#45340,.T.);
#61505=ORIENTED_EDGE('',*,*,#45336,.F.);
#61506=ORIENTED_EDGE('',*,*,#45341,.T.);
#61507=ORIENTED_EDGE('',*,*,#45311,.F.);
#61508=ORIENTED_EDGE('',*,*,#45342,.T.);
#61509=ORIENTED_EDGE('',*,*,#45339,.F.);
#61510=ORIENTED_EDGE('',*,*,#45343,.T.);
#61511=ORIENTED_EDGE('',*,*,#45331,.F.);
#61512=ORIENTED_EDGE('',*,*,#45344,.F.);
#61513=ORIENTED_EDGE('',*,*,#45345,.F.);
#61514=ORIENTED_EDGE('',*,*,#45346,.T.);
#61515=ORIENTED_EDGE('',*,*,#45334,.F.);
#61516=ORIENTED_EDGE('',*,*,#45347,.T.);
#61517=ORIENTED_EDGE('',*,*,#45348,.T.);
#61518=ORIENTED_EDGE('',*,*,#45344,.T.);
#61519=ORIENTED_EDGE('',*,*,#45337,.F.);
#61520=ORIENTED_EDGE('',*,*,#45349,.T.);
#61521=ORIENTED_EDGE('',*,*,#45350,.F.);
#61522=ORIENTED_EDGE('',*,*,#45351,.F.);
#61523=ORIENTED_EDGE('',*,*,#45352,.T.);
#61524=ORIENTED_EDGE('',*,*,#45347,.F.);
#61525=ORIENTED_EDGE('',*,*,#45340,.F.);
#61526=ORIENTED_EDGE('',*,*,#45353,.F.);
#61527=ORIENTED_EDGE('',*,*,#45354,.T.);
#61528=ORIENTED_EDGE('',*,*,#45355,.F.);
#61529=ORIENTED_EDGE('',*,*,#45356,.F.);
#61530=ORIENTED_EDGE('',*,*,#45357,.T.);
#61531=ORIENTED_EDGE('',*,*,#45358,.F.);
#61532=ORIENTED_EDGE('',*,*,#45359,.T.);
#61533=ORIENTED_EDGE('',*,*,#45360,.F.);
#61534=ORIENTED_EDGE('',*,*,#45361,.F.);
#61535=ORIENTED_EDGE('',*,*,#45349,.F.);
#61536=ORIENTED_EDGE('',*,*,#45342,.F.);
#61537=ORIENTED_EDGE('',*,*,#45362,.T.);
#61538=ORIENTED_EDGE('',*,*,#45363,.T.);
#61539=ORIENTED_EDGE('',*,*,#45353,.T.);
#61540=ORIENTED_EDGE('',*,*,#45314,.F.);
#61541=ORIENTED_EDGE('',*,*,#45364,.F.);
#61542=ORIENTED_EDGE('',*,*,#45365,.F.);
#61543=ORIENTED_EDGE('',*,*,#45362,.F.);
#61544=ORIENTED_EDGE('',*,*,#45312,.F.);
#61545=ORIENTED_EDGE('',*,*,#45343,.F.);
#61546=ORIENTED_EDGE('',*,*,#45341,.F.);
#61547=ORIENTED_EDGE('',*,*,#45338,.F.);
#61548=ORIENTED_EDGE('',*,*,#45335,.F.);
#61549=ORIENTED_EDGE('',*,*,#45332,.F.);
#61550=ORIENTED_EDGE('',*,*,#45329,.F.);
#61551=ORIENTED_EDGE('',*,*,#45326,.F.);
#61552=ORIENTED_EDGE('',*,*,#45323,.F.);
#61553=ORIENTED_EDGE('',*,*,#45320,.F.);
#61554=ORIENTED_EDGE('',*,*,#45317,.F.);
#61555=ORIENTED_EDGE('',*,*,#45366,.T.);
#61556=ORIENTED_EDGE('',*,*,#45367,.T.);
#61557=ORIENTED_EDGE('',*,*,#45368,.T.);
#61558=ORIENTED_EDGE('',*,*,#45369,.T.);
#61559=ORIENTED_EDGE('',*,*,#45370,.T.);
#61560=ORIENTED_EDGE('',*,*,#45371,.T.);
#61561=ORIENTED_EDGE('',*,*,#45367,.F.);
#61562=ORIENTED_EDGE('',*,*,#45372,.T.);
#61563=ORIENTED_EDGE('',*,*,#45373,.T.);
#61564=ORIENTED_EDGE('',*,*,#45374,.T.);
#61565=ORIENTED_EDGE('',*,*,#45370,.F.);
#61566=ORIENTED_EDGE('',*,*,#45375,.T.);
#61567=ORIENTED_EDGE('',*,*,#45376,.T.);
#61568=ORIENTED_EDGE('',*,*,#45377,.T.);
#61569=ORIENTED_EDGE('',*,*,#45373,.F.);
#61570=ORIENTED_EDGE('',*,*,#45378,.T.);
#61571=ORIENTED_EDGE('',*,*,#45379,.T.);
#61572=ORIENTED_EDGE('',*,*,#45376,.F.);
#61573=ORIENTED_EDGE('',*,*,#45380,.T.);
#61574=ORIENTED_EDGE('',*,*,#45381,.F.);
#61575=ORIENTED_EDGE('',*,*,#45382,.T.);
#61576=ORIENTED_EDGE('',*,*,#45369,.F.);
#61577=ORIENTED_EDGE('',*,*,#45383,.F.);
#61578=ORIENTED_EDGE('',*,*,#45384,.T.);
#61579=ORIENTED_EDGE('',*,*,#45385,.F.);
#61580=ORIENTED_EDGE('',*,*,#45381,.T.);
#61581=ORIENTED_EDGE('',*,*,#45377,.F.);
#61582=ORIENTED_EDGE('',*,*,#45386,.T.);
#61583=ORIENTED_EDGE('',*,*,#45387,.T.);
#61584=ORIENTED_EDGE('',*,*,#45388,.T.);
#61585=ORIENTED_EDGE('',*,*,#45379,.F.);
#61586=ORIENTED_EDGE('',*,*,#45385,.T.);
#61587=ORIENTED_EDGE('',*,*,#45389,.T.);
#61588=ORIENTED_EDGE('',*,*,#45390,.T.);
#61589=ORIENTED_EDGE('',*,*,#45391,.T.);
#61590=ORIENTED_EDGE('',*,*,#45392,.F.);
#61591=ORIENTED_EDGE('',*,*,#45393,.F.);
#61592=ORIENTED_EDGE('',*,*,#45394,.F.);
#61593=ORIENTED_EDGE('',*,*,#45395,.F.);
#61594=ORIENTED_EDGE('',*,*,#45386,.F.);
#61595=ORIENTED_EDGE('',*,*,#45384,.F.);
#61596=ORIENTED_EDGE('',*,*,#45396,.F.);
#61597=ORIENTED_EDGE('',*,*,#45397,.F.);
#61598=ORIENTED_EDGE('',*,*,#45389,.F.);
#61599=ORIENTED_EDGE('',*,*,#45366,.F.);
#61600=ORIENTED_EDGE('',*,*,#45382,.F.);
#61601=ORIENTED_EDGE('',*,*,#45380,.F.);
#61602=ORIENTED_EDGE('',*,*,#45378,.F.);
#61603=ORIENTED_EDGE('',*,*,#45375,.F.);
#61604=ORIENTED_EDGE('',*,*,#45372,.F.);
#61605=ORIENTED_EDGE('',*,*,#45368,.F.);
#61606=ORIENTED_EDGE('',*,*,#45398,.F.);
#61607=ORIENTED_EDGE('',*,*,#45399,.F.);
#61608=ORIENTED_EDGE('',*,*,#45400,.F.);
#61609=ORIENTED_EDGE('',*,*,#45401,.T.);
#61610=ORIENTED_EDGE('',*,*,#45402,.T.);
#61611=ORIENTED_EDGE('',*,*,#45403,.T.);
#61612=ORIENTED_EDGE('',*,*,#45404,.F.);
#61613=ORIENTED_EDGE('',*,*,#45405,.F.);
#61614=ORIENTED_EDGE('',*,*,#45406,.T.);
#61615=ORIENTED_EDGE('',*,*,#45407,.F.);
#61616=ORIENTED_EDGE('',*,*,#45408,.F.);
#61617=ORIENTED_EDGE('',*,*,#45396,.T.);
#61618=ORIENTED_EDGE('',*,*,#45383,.T.);
#61619=ORIENTED_EDGE('',*,*,#45409,.T.);
#61620=ORIENTED_EDGE('',*,*,#45410,.T.);
#61621=ORIENTED_EDGE('',*,*,#45411,.T.);
#61622=ORIENTED_EDGE('',*,*,#45412,.T.);
#61623=ORIENTED_EDGE('',*,*,#45413,.T.);
#61624=ORIENTED_EDGE('',*,*,#45414,.T.);
#61625=ORIENTED_EDGE('',*,*,#45411,.F.);
#61626=ORIENTED_EDGE('',*,*,#45415,.T.);
#61627=ORIENTED_EDGE('',*,*,#45416,.T.);
#61628=ORIENTED_EDGE('',*,*,#45417,.T.);
#61629=ORIENTED_EDGE('',*,*,#45413,.F.);
#61630=ORIENTED_EDGE('',*,*,#45418,.T.);
#61631=ORIENTED_EDGE('',*,*,#45419,.T.);
#61632=ORIENTED_EDGE('',*,*,#45420,.T.);
#61633=ORIENTED_EDGE('',*,*,#45416,.F.);
#61634=ORIENTED_EDGE('',*,*,#45421,.T.);
#61635=ORIENTED_EDGE('',*,*,#45422,.T.);
#61636=ORIENTED_EDGE('',*,*,#45423,.T.);
#61637=ORIENTED_EDGE('',*,*,#45419,.F.);
#61638=ORIENTED_EDGE('',*,*,#45424,.T.);
#61639=ORIENTED_EDGE('',*,*,#45425,.T.);
#61640=ORIENTED_EDGE('',*,*,#45426,.T.);
#61641=ORIENTED_EDGE('',*,*,#45422,.F.);
#61642=ORIENTED_EDGE('',*,*,#45427,.T.);
#61643=ORIENTED_EDGE('',*,*,#45428,.T.);
#61644=ORIENTED_EDGE('',*,*,#45429,.T.);
#61645=ORIENTED_EDGE('',*,*,#45425,.F.);
#61646=ORIENTED_EDGE('',*,*,#45430,.T.);
#61647=ORIENTED_EDGE('',*,*,#45431,.T.);
#61648=ORIENTED_EDGE('',*,*,#45432,.T.);
#61649=ORIENTED_EDGE('',*,*,#45428,.F.);
#61650=ORIENTED_EDGE('',*,*,#45433,.T.);
#61651=ORIENTED_EDGE('',*,*,#45434,.T.);
#61652=ORIENTED_EDGE('',*,*,#45435,.T.);
#61653=ORIENTED_EDGE('',*,*,#45436,.T.);
#61654=ORIENTED_EDGE('',*,*,#45431,.F.);
#61655=ORIENTED_EDGE('',*,*,#45437,.T.);
#61656=ORIENTED_EDGE('',*,*,#45438,.T.);
#61657=ORIENTED_EDGE('',*,*,#45439,.T.);
#61658=ORIENTED_EDGE('',*,*,#45434,.F.);
#61659=ORIENTED_EDGE('',*,*,#45440,.T.);
#61660=ORIENTED_EDGE('',*,*,#45441,.T.);
#61661=ORIENTED_EDGE('',*,*,#45442,.T.);
#61662=ORIENTED_EDGE('',*,*,#45438,.F.);
#61663=ORIENTED_EDGE('',*,*,#45443,.T.);
#61664=ORIENTED_EDGE('',*,*,#45409,.F.);
#61665=ORIENTED_EDGE('',*,*,#45444,.T.);
#61666=ORIENTED_EDGE('',*,*,#45441,.F.);
#61667=ORIENTED_EDGE('',*,*,#45445,.T.);
#61668=ORIENTED_EDGE('',*,*,#45432,.F.);
#61669=ORIENTED_EDGE('',*,*,#45446,.T.);
#61670=ORIENTED_EDGE('',*,*,#45447,.T.);
#61671=ORIENTED_EDGE('',*,*,#45448,.T.);
#61672=ORIENTED_EDGE('',*,*,#45449,.F.);
#61673=ORIENTED_EDGE('',*,*,#45450,.T.);
#61674=ORIENTED_EDGE('',*,*,#45435,.F.);
#61675=ORIENTED_EDGE('',*,*,#45451,.F.);
#61676=ORIENTED_EDGE('',*,*,#45452,.F.);
#61677=ORIENTED_EDGE('',*,*,#45453,.F.);
#61678=ORIENTED_EDGE('',*,*,#45454,.F.);
#61679=ORIENTED_EDGE('',*,*,#45455,.F.);
#61680=ORIENTED_EDGE('',*,*,#45456,.F.);
#61681=ORIENTED_EDGE('',*,*,#45457,.F.);
#61682=ORIENTED_EDGE('',*,*,#45458,.F.);
#61683=ORIENTED_EDGE('',*,*,#45459,.F.);
#61684=ORIENTED_EDGE('',*,*,#45460,.F.);
#61685=ORIENTED_EDGE('',*,*,#45446,.F.);
#61686=ORIENTED_EDGE('',*,*,#45436,.F.);
#61687=ORIENTED_EDGE('',*,*,#45450,.F.);
#61688=ORIENTED_EDGE('',*,*,#45439,.F.);
#61689=ORIENTED_EDGE('',*,*,#45461,.T.);
#61690=ORIENTED_EDGE('',*,*,#45462,.T.);
#61691=ORIENTED_EDGE('',*,*,#45451,.T.);
#61692=ORIENTED_EDGE('',*,*,#45442,.F.);
#61693=ORIENTED_EDGE('',*,*,#45463,.F.);
#61694=ORIENTED_EDGE('',*,*,#45464,.F.);
#61695=ORIENTED_EDGE('',*,*,#45461,.F.);
#61696=ORIENTED_EDGE('',*,*,#45444,.F.);
#61697=ORIENTED_EDGE('',*,*,#45465,.T.);
#61698=ORIENTED_EDGE('',*,*,#45466,.T.);
#61699=ORIENTED_EDGE('',*,*,#45463,.T.);
#61700=ORIENTED_EDGE('',*,*,#45412,.F.);
#61701=ORIENTED_EDGE('',*,*,#45467,.T.);
#61702=ORIENTED_EDGE('',*,*,#45468,.F.);
#61703=ORIENTED_EDGE('',*,*,#45465,.F.);
#61704=ORIENTED_EDGE('',*,*,#45410,.F.);
#61705=ORIENTED_EDGE('',*,*,#45445,.F.);
#61706=ORIENTED_EDGE('',*,*,#45443,.F.);
#61707=ORIENTED_EDGE('',*,*,#45440,.F.);
#61708=ORIENTED_EDGE('',*,*,#45437,.F.);
#61709=ORIENTED_EDGE('',*,*,#45433,.F.);
#61710=ORIENTED_EDGE('',*,*,#45430,.F.);
#61711=ORIENTED_EDGE('',*,*,#45427,.F.);
#61712=ORIENTED_EDGE('',*,*,#45424,.F.);
#61713=ORIENTED_EDGE('',*,*,#45421,.F.);
#61714=ORIENTED_EDGE('',*,*,#45418,.F.);
#61715=ORIENTED_EDGE('',*,*,#45415,.F.);
#61716=ORIENTED_EDGE('',*,*,#45469,.T.);
#61717=ORIENTED_EDGE('',*,*,#45470,.T.);
#61718=ORIENTED_EDGE('',*,*,#45471,.T.);
#61719=ORIENTED_EDGE('',*,*,#45472,.F.);
#61720=ORIENTED_EDGE('',*,*,#45473,.T.);
#61721=ORIENTED_EDGE('',*,*,#45474,.T.);
#61722=ORIENTED_EDGE('',*,*,#45470,.F.);
#61723=ORIENTED_EDGE('',*,*,#45475,.T.);
#61724=ORIENTED_EDGE('',*,*,#45476,.T.);
#61725=ORIENTED_EDGE('',*,*,#45477,.T.);
#61726=ORIENTED_EDGE('',*,*,#45473,.F.);
#61727=ORIENTED_EDGE('',*,*,#45478,.T.);
#61728=ORIENTED_EDGE('',*,*,#45479,.T.);
#61729=ORIENTED_EDGE('',*,*,#45480,.T.);
#61730=ORIENTED_EDGE('',*,*,#45476,.F.);
#61731=ORIENTED_EDGE('',*,*,#45481,.T.);
#61732=ORIENTED_EDGE('',*,*,#45482,.T.);
#61733=ORIENTED_EDGE('',*,*,#45483,.T.);
#61734=ORIENTED_EDGE('',*,*,#45479,.F.);
#61735=ORIENTED_EDGE('',*,*,#45484,.T.);
#61736=ORIENTED_EDGE('',*,*,#45485,.T.);
#61737=ORIENTED_EDGE('',*,*,#45486,.T.);
#61738=ORIENTED_EDGE('',*,*,#45482,.F.);
#61739=ORIENTED_EDGE('',*,*,#45487,.T.);
#61740=ORIENTED_EDGE('',*,*,#45488,.T.);
#61741=ORIENTED_EDGE('',*,*,#45458,.T.);
#61742=ORIENTED_EDGE('',*,*,#45485,.F.);
#61743=ORIENTED_EDGE('',*,*,#45489,.T.);
#61744=ORIENTED_EDGE('',*,*,#45490,.T.);
#61745=ORIENTED_EDGE('',*,*,#45491,.T.);
#61746=ORIENTED_EDGE('',*,*,#45488,.F.);
#61747=ORIENTED_EDGE('',*,*,#45492,.T.);
#61748=ORIENTED_EDGE('',*,*,#45493,.T.);
#61749=ORIENTED_EDGE('',*,*,#45494,.T.);
#61750=ORIENTED_EDGE('',*,*,#45490,.F.);
#61751=ORIENTED_EDGE('',*,*,#45495,.T.);
#61752=ORIENTED_EDGE('',*,*,#45496,.T.);
#61753=ORIENTED_EDGE('',*,*,#45497,.T.);
#61754=ORIENTED_EDGE('',*,*,#45493,.F.);
#61755=ORIENTED_EDGE('',*,*,#45498,.T.);
#61756=ORIENTED_EDGE('',*,*,#45499,.T.);
#61757=ORIENTED_EDGE('',*,*,#45496,.F.);
#61758=ORIENTED_EDGE('',*,*,#45500,.T.);
#61759=ORIENTED_EDGE('',*,*,#45501,.T.);
#61760=ORIENTED_EDGE('',*,*,#45502,.T.);
#61761=ORIENTED_EDGE('',*,*,#45503,.F.);
#61762=ORIENTED_EDGE('',*,*,#45501,.F.);
#61763=ORIENTED_EDGE('',*,*,#45504,.T.);
#61764=ORIENTED_EDGE('',*,*,#45472,.T.);
#61765=ORIENTED_EDGE('',*,*,#45505,.F.);
#61766=ORIENTED_EDGE('',*,*,#45494,.F.);
#61767=ORIENTED_EDGE('',*,*,#45506,.F.);
#61768=ORIENTED_EDGE('',*,*,#45507,.F.);
#61769=ORIENTED_EDGE('',*,*,#45508,.F.);
#61770=ORIENTED_EDGE('',*,*,#45497,.F.);
#61771=ORIENTED_EDGE('',*,*,#45509,.T.);
#61772=ORIENTED_EDGE('',*,*,#45510,.T.);
#61773=ORIENTED_EDGE('',*,*,#45506,.T.);
#61774=ORIENTED_EDGE('',*,*,#45502,.F.);
#61775=ORIENTED_EDGE('',*,*,#45511,.F.);
#61776=ORIENTED_EDGE('',*,*,#45423,.F.);
#61777=ORIENTED_EDGE('',*,*,#45512,.F.);
#61778=ORIENTED_EDGE('',*,*,#45513,.F.);
#61779=ORIENTED_EDGE('',*,*,#45509,.F.);
#61780=ORIENTED_EDGE('',*,*,#45499,.F.);
#61781=ORIENTED_EDGE('',*,*,#45503,.T.);
#61782=ORIENTED_EDGE('',*,*,#45511,.T.);
#61783=ORIENTED_EDGE('',*,*,#45505,.T.);
#61784=ORIENTED_EDGE('',*,*,#45471,.F.);
#61785=ORIENTED_EDGE('',*,*,#45514,.F.);
#61786=ORIENTED_EDGE('',*,*,#45515,.T.);
#61787=ORIENTED_EDGE('',*,*,#45516,.F.);
#61788=ORIENTED_EDGE('',*,*,#45517,.T.);
#61789=ORIENTED_EDGE('',*,*,#45518,.F.);
#61790=ORIENTED_EDGE('',*,*,#45519,.F.);
#61791=ORIENTED_EDGE('',*,*,#45520,.F.);
#61792=ORIENTED_EDGE('',*,*,#45521,.F.);
#61793=ORIENTED_EDGE('',*,*,#45522,.T.);
#61794=ORIENTED_EDGE('',*,*,#45523,.T.);
#61795=ORIENTED_EDGE('',*,*,#45524,.F.);
#61796=ORIENTED_EDGE('',*,*,#45525,.T.);
#61797=ORIENTED_EDGE('',*,*,#45526,.F.);
#61798=ORIENTED_EDGE('',*,*,#45527,.T.);
#61799=ORIENTED_EDGE('',*,*,#45528,.F.);
#61800=ORIENTED_EDGE('',*,*,#45469,.F.);
#61801=ORIENTED_EDGE('',*,*,#45504,.F.);
#61802=ORIENTED_EDGE('',*,*,#45500,.F.);
#61803=ORIENTED_EDGE('',*,*,#45498,.F.);
#61804=ORIENTED_EDGE('',*,*,#45495,.F.);
#61805=ORIENTED_EDGE('',*,*,#45492,.F.);
#61806=ORIENTED_EDGE('',*,*,#45489,.F.);
#61807=ORIENTED_EDGE('',*,*,#45487,.F.);
#61808=ORIENTED_EDGE('',*,*,#45484,.F.);
#61809=ORIENTED_EDGE('',*,*,#45481,.F.);
#61810=ORIENTED_EDGE('',*,*,#45478,.F.);
#61811=ORIENTED_EDGE('',*,*,#45475,.F.);
#61812=ORIENTED_EDGE('',*,*,#45529,.T.);
#61813=ORIENTED_EDGE('',*,*,#45530,.T.);
#61814=ORIENTED_EDGE('',*,*,#45531,.T.);
#61815=ORIENTED_EDGE('',*,*,#45532,.T.);
#61816=ORIENTED_EDGE('',*,*,#45533,.T.);
#61817=ORIENTED_EDGE('',*,*,#45534,.T.);
#61818=ORIENTED_EDGE('',*,*,#45531,.F.);
#61819=ORIENTED_EDGE('',*,*,#45535,.T.);
#61820=ORIENTED_EDGE('',*,*,#45536,.T.);
#61821=ORIENTED_EDGE('',*,*,#45537,.T.);
#61822=ORIENTED_EDGE('',*,*,#45533,.F.);
#61823=ORIENTED_EDGE('',*,*,#45538,.T.);
#61824=ORIENTED_EDGE('',*,*,#45539,.T.);
#61825=ORIENTED_EDGE('',*,*,#45540,.T.);
#61826=ORIENTED_EDGE('',*,*,#45536,.F.);
#61827=ORIENTED_EDGE('',*,*,#45541,.T.);
#61828=ORIENTED_EDGE('',*,*,#45542,.T.);
#61829=ORIENTED_EDGE('',*,*,#45454,.T.);
#61830=ORIENTED_EDGE('',*,*,#45539,.F.);
#61831=ORIENTED_EDGE('',*,*,#45543,.T.);
#61832=ORIENTED_EDGE('',*,*,#45544,.T.);
#61833=ORIENTED_EDGE('',*,*,#45545,.T.);
#61834=ORIENTED_EDGE('',*,*,#45542,.F.);
#61835=ORIENTED_EDGE('',*,*,#45546,.T.);
#61836=ORIENTED_EDGE('',*,*,#45547,.T.);
#61837=ORIENTED_EDGE('',*,*,#45548,.T.);
#61838=ORIENTED_EDGE('',*,*,#45544,.F.);
#61839=ORIENTED_EDGE('',*,*,#45549,.T.);
#61840=ORIENTED_EDGE('',*,*,#45550,.T.);
#61841=ORIENTED_EDGE('',*,*,#45551,.T.);
#61842=ORIENTED_EDGE('',*,*,#45547,.F.);
#61843=ORIENTED_EDGE('',*,*,#45552,.T.);
#61844=ORIENTED_EDGE('',*,*,#45553,.T.);
#61845=ORIENTED_EDGE('',*,*,#45554,.T.);
#61846=ORIENTED_EDGE('',*,*,#45550,.F.);
#61847=ORIENTED_EDGE('',*,*,#45555,.T.);
#61848=ORIENTED_EDGE('',*,*,#45529,.F.);
#61849=ORIENTED_EDGE('',*,*,#45556,.T.);
#61850=ORIENTED_EDGE('',*,*,#45553,.F.);
#61851=ORIENTED_EDGE('',*,*,#45557,.T.);
#61852=ORIENTED_EDGE('',*,*,#45548,.F.);
#61853=ORIENTED_EDGE('',*,*,#45558,.F.);
#61854=ORIENTED_EDGE('',*,*,#45559,.F.);
#61855=ORIENTED_EDGE('',*,*,#45560,.F.);
#61856=ORIENTED_EDGE('',*,*,#45551,.F.);
#61857=ORIENTED_EDGE('',*,*,#45561,.T.);
#61858=ORIENTED_EDGE('',*,*,#45562,.T.);
#61859=ORIENTED_EDGE('',*,*,#45558,.T.);
#61860=ORIENTED_EDGE('',*,*,#45554,.F.);
#61861=ORIENTED_EDGE('',*,*,#45563,.F.);
#61862=ORIENTED_EDGE('',*,*,#45564,.T.);
#61863=ORIENTED_EDGE('',*,*,#45561,.F.);
#61864=ORIENTED_EDGE('',*,*,#45556,.F.);
#61865=ORIENTED_EDGE('',*,*,#45565,.T.);
#61866=ORIENTED_EDGE('',*,*,#45566,.T.);
#61867=ORIENTED_EDGE('',*,*,#45563,.T.);
#61868=ORIENTED_EDGE('',*,*,#45532,.F.);
#61869=ORIENTED_EDGE('',*,*,#45567,.F.);
#61870=ORIENTED_EDGE('',*,*,#45568,.F.);
#61871=ORIENTED_EDGE('',*,*,#45569,.F.);
#61872=ORIENTED_EDGE('',*,*,#45570,.T.);
#61873=ORIENTED_EDGE('',*,*,#45571,.F.);
#61874=ORIENTED_EDGE('',*,*,#45572,.T.);
#61875=ORIENTED_EDGE('',*,*,#45573,.F.);
#61876=ORIENTED_EDGE('',*,*,#45574,.F.);
#61877=ORIENTED_EDGE('',*,*,#45575,.F.);
#61878=ORIENTED_EDGE('',*,*,#45576,.F.);
#61879=ORIENTED_EDGE('',*,*,#45577,.T.);
#61880=ORIENTED_EDGE('',*,*,#45578,.F.);
#61881=ORIENTED_EDGE('',*,*,#45579,.T.);
#61882=ORIENTED_EDGE('',*,*,#45565,.F.);
#61883=ORIENTED_EDGE('',*,*,#45530,.F.);
#61884=ORIENTED_EDGE('',*,*,#45557,.F.);
#61885=ORIENTED_EDGE('',*,*,#45555,.F.);
#61886=ORIENTED_EDGE('',*,*,#45552,.F.);
#61887=ORIENTED_EDGE('',*,*,#45549,.F.);
#61888=ORIENTED_EDGE('',*,*,#45546,.F.);
#61889=ORIENTED_EDGE('',*,*,#45543,.F.);
#61890=ORIENTED_EDGE('',*,*,#45541,.F.);
#61891=ORIENTED_EDGE('',*,*,#45538,.F.);
#61892=ORIENTED_EDGE('',*,*,#45535,.F.);
#61893=ORIENTED_EDGE('',*,*,#45414,.F.);
#61894=ORIENTED_EDGE('',*,*,#45580,.T.);
#61895=ORIENTED_EDGE('',*,*,#45581,.T.);
#61896=ORIENTED_EDGE('',*,*,#45467,.F.);
#61897=ORIENTED_EDGE('',*,*,#45417,.F.);
#61898=ORIENTED_EDGE('',*,*,#45582,.F.);
#61899=ORIENTED_EDGE('',*,*,#45583,.F.);
#61900=ORIENTED_EDGE('',*,*,#45580,.F.);
#61901=ORIENTED_EDGE('',*,*,#45420,.F.);
#61902=ORIENTED_EDGE('',*,*,#45528,.T.);
#61903=ORIENTED_EDGE('',*,*,#45584,.T.);
#61904=ORIENTED_EDGE('',*,*,#45582,.T.);
#61905=ORIENTED_EDGE('',*,*,#45371,.F.);
#61906=ORIENTED_EDGE('',*,*,#45585,.T.);
#61907=ORIENTED_EDGE('',*,*,#45586,.T.);
#61908=ORIENTED_EDGE('',*,*,#45398,.T.);
#61909=ORIENTED_EDGE('',*,*,#45374,.F.);
#61910=ORIENTED_EDGE('',*,*,#45388,.F.);
#61911=ORIENTED_EDGE('',*,*,#45587,.F.);
#61912=ORIENTED_EDGE('',*,*,#45585,.F.);
#61913=ORIENTED_EDGE('',*,*,#45588,.T.);
#61914=ORIENTED_EDGE('',*,*,#45589,.T.);
#61915=ORIENTED_EDGE('',*,*,#45590,.T.);
#61916=ORIENTED_EDGE('',*,*,#45591,.T.);
#61917=ORIENTED_EDGE('',*,*,#45592,.F.);
#61918=ORIENTED_EDGE('',*,*,#45591,.F.);
#61919=ORIENTED_EDGE('',*,*,#45593,.F.);
#61920=ORIENTED_EDGE('',*,*,#45594,.F.);
#61921=ORIENTED_EDGE('',*,*,#45595,.F.);
#61922=ORIENTED_EDGE('',*,*,#45596,.F.);
#61923=ORIENTED_EDGE('',*,*,#45597,.F.);
#61924=ORIENTED_EDGE('',*,*,#45598,.F.);
#61925=ORIENTED_EDGE('',*,*,#45589,.F.);
#61926=ORIENTED_EDGE('',*,*,#45599,.F.);
#61927=ORIENTED_EDGE('',*,*,#45600,.F.);
#61928=ORIENTED_EDGE('',*,*,#45601,.F.);
#61929=ORIENTED_EDGE('',*,*,#45602,.T.);
#61930=ORIENTED_EDGE('',*,*,#45598,.T.);
#61931=ORIENTED_EDGE('',*,*,#45603,.T.);
#61932=ORIENTED_EDGE('',*,*,#45526,.T.);
#61933=ORIENTED_EDGE('',*,*,#45426,.F.);
#61934=ORIENTED_EDGE('',*,*,#45604,.T.);
#61935=ORIENTED_EDGE('',*,*,#45605,.T.);
#61936=ORIENTED_EDGE('',*,*,#45512,.T.);
#61937=ORIENTED_EDGE('',*,*,#45606,.T.);
#61938=ORIENTED_EDGE('',*,*,#45607,.T.);
#61939=ORIENTED_EDGE('',*,*,#45608,.T.);
#61940=ORIENTED_EDGE('',*,*,#45594,.T.);
#61941=ORIENTED_EDGE('',*,*,#45609,.F.);
#61942=ORIENTED_EDGE('',*,*,#45610,.T.);
#61943=ORIENTED_EDGE('',*,*,#45611,.T.);
#61944=ORIENTED_EDGE('',*,*,#45600,.T.);
#61945=ORIENTED_EDGE('',*,*,#45610,.F.);
#61946=ORIENTED_EDGE('',*,*,#45612,.T.);
#61947=ORIENTED_EDGE('',*,*,#45613,.F.);
#61948=ORIENTED_EDGE('',*,*,#45614,.F.);
#61949=ORIENTED_EDGE('',*,*,#45607,.F.);
#61950=ORIENTED_EDGE('',*,*,#45615,.F.);
#61951=ORIENTED_EDGE('',*,*,#45616,.F.);
#61952=ORIENTED_EDGE('',*,*,#45617,.F.);
#61953=ORIENTED_EDGE('',*,*,#45618,.F.);
#61954=ORIENTED_EDGE('',*,*,#45616,.T.);
#61955=ORIENTED_EDGE('',*,*,#45619,.F.);
#61956=ORIENTED_EDGE('',*,*,#45620,.F.);
#61957=ORIENTED_EDGE('',*,*,#45621,.F.);
#61958=ORIENTED_EDGE('',*,*,#45622,.F.);
#61959=ORIENTED_EDGE('',*,*,#45623,.F.);
#61960=ORIENTED_EDGE('',*,*,#45624,.T.);
#61961=ORIENTED_EDGE('',*,*,#45622,.T.);
#61962=ORIENTED_EDGE('',*,*,#45624,.F.);
#61963=ORIENTED_EDGE('',*,*,#45625,.F.);
#61964=ORIENTED_EDGE('',*,*,#45626,.T.);
#61965=ORIENTED_EDGE('',*,*,#45621,.T.);
#61966=ORIENTED_EDGE('',*,*,#45626,.F.);
#61967=ORIENTED_EDGE('',*,*,#45244,.F.);
#61968=ORIENTED_EDGE('',*,*,#45627,.F.);
#61969=ORIENTED_EDGE('',*,*,#45628,.T.);
#61970=ORIENTED_EDGE('',*,*,#45629,.T.);
#61971=ORIENTED_EDGE('',*,*,#45630,.F.);
#61972=ORIENTED_EDGE('',*,*,#45631,.F.);
#61973=ORIENTED_EDGE('',*,*,#45632,.F.);
#61974=ORIENTED_EDGE('',*,*,#45633,.F.);
#61975=ORIENTED_EDGE('',*,*,#45634,.T.);
#61976=ORIENTED_EDGE('',*,*,#45635,.F.);
#61977=ORIENTED_EDGE('',*,*,#45248,.F.);
#61978=ORIENTED_EDGE('',*,*,#45636,.T.);
#61979=ORIENTED_EDGE('',*,*,#45637,.F.);
#61980=ORIENTED_EDGE('',*,*,#45627,.T.);
#61981=ORIENTED_EDGE('',*,*,#45217,.F.);
#61982=ORIENTED_EDGE('',*,*,#45638,.F.);
#61983=ORIENTED_EDGE('',*,*,#45639,.F.);
#61984=ORIENTED_EDGE('',*,*,#45636,.F.);
#61985=ORIENTED_EDGE('',*,*,#45219,.F.);
#61986=ORIENTED_EDGE('',*,*,#45251,.T.);
#61987=ORIENTED_EDGE('',*,*,#45640,.T.);
#61988=ORIENTED_EDGE('',*,*,#45638,.T.);
#61989=ORIENTED_EDGE('',*,*,#45641,.T.);
#61990=ORIENTED_EDGE('',*,*,#45642,.T.);
#61991=ORIENTED_EDGE('',*,*,#45643,.T.);
#61992=ORIENTED_EDGE('',*,*,#45633,.T.);
#61993=ORIENTED_EDGE('',*,*,#45644,.T.);
#61994=ORIENTED_EDGE('',*,*,#45645,.T.);
#61995=ORIENTED_EDGE('',*,*,#45646,.T.);
#61996=ORIENTED_EDGE('',*,*,#45647,.T.);
#61997=ORIENTED_EDGE('',*,*,#45647,.F.);
#61998=ORIENTED_EDGE('',*,*,#45648,.F.);
#61999=ORIENTED_EDGE('',*,*,#45649,.F.);
#62000=ORIENTED_EDGE('',*,*,#45650,.F.);
#62001=ORIENTED_EDGE('',*,*,#45238,.F.);
#62002=ORIENTED_EDGE('',*,*,#45651,.T.);
#62003=ORIENTED_EDGE('',*,*,#45652,.T.);
#62004=ORIENTED_EDGE('',*,*,#45260,.T.);
#62005=ORIENTED_EDGE('',*,*,#45645,.F.);
#62006=ORIENTED_EDGE('',*,*,#45653,.F.);
#62007=ORIENTED_EDGE('',*,*,#45654,.F.);
#62008=ORIENTED_EDGE('',*,*,#45655,.F.);
#62009=ORIENTED_EDGE('',*,*,#45656,.F.);
#62010=ORIENTED_EDGE('',*,*,#45657,.T.);
#62011=ORIENTED_EDGE('',*,*,#45658,.T.);
#62012=ORIENTED_EDGE('',*,*,#45654,.T.);
#62013=ORIENTED_EDGE('',*,*,#45659,.T.);
#62014=ORIENTED_EDGE('',*,*,#45660,.T.);
#62015=ORIENTED_EDGE('',*,*,#45661,.T.);
#62016=ORIENTED_EDGE('',*,*,#45662,.T.);
#62017=ORIENTED_EDGE('',*,*,#45660,.F.);
#62018=ORIENTED_EDGE('',*,*,#45663,.F.);
#62019=ORIENTED_EDGE('',*,*,#45629,.F.);
#62020=ORIENTED_EDGE('',*,*,#45664,.F.);
#62021=ORIENTED_EDGE('',*,*,#45665,.F.);
#62022=ORIENTED_EDGE('',*,*,#45666,.T.);
#62023=ORIENTED_EDGE('',*,*,#45667,.F.);
#62024=ORIENTED_EDGE('',*,*,#45666,.F.);
#62025=ORIENTED_EDGE('',*,*,#45668,.T.);
#62026=ORIENTED_EDGE('',*,*,#45669,.T.);
#62027=ORIENTED_EDGE('',*,*,#45670,.T.);
#62028=ORIENTED_EDGE('',*,*,#45631,.T.);
#62029=ORIENTED_EDGE('',*,*,#45671,.T.);
#62030=ORIENTED_EDGE('',*,*,#45672,.T.);
#62031=ORIENTED_EDGE('',*,*,#45673,.T.);
#62032=ORIENTED_EDGE('',*,*,#45674,.T.);
#62033=ORIENTED_EDGE('',*,*,#45675,.F.);
#62034=ORIENTED_EDGE('',*,*,#45676,.T.);
#62035=ORIENTED_EDGE('',*,*,#45677,.F.);
#62036=ORIENTED_EDGE('',*,*,#45678,.F.);
#62037=ORIENTED_EDGE('',*,*,#45402,.F.);
#62038=ORIENTED_EDGE('',*,*,#45679,.T.);
#62039=ORIENTED_EDGE('',*,*,#45680,.F.);
#62040=ORIENTED_EDGE('',*,*,#45681,.F.);
#62041=ORIENTED_EDGE('',*,*,#45682,.F.);
#62042=ORIENTED_EDGE('',*,*,#45683,.T.);
#62043=ORIENTED_EDGE('',*,*,#45684,.F.);
#62044=ORIENTED_EDGE('',*,*,#45683,.F.);
#62045=ORIENTED_EDGE('',*,*,#45685,.T.);
#62046=ORIENTED_EDGE('',*,*,#45686,.T.);
#62047=ORIENTED_EDGE('',*,*,#45687,.F.);
#62048=ORIENTED_EDGE('',*,*,#45687,.T.);
#62049=ORIENTED_EDGE('',*,*,#45688,.T.);
#62050=ORIENTED_EDGE('',*,*,#45684,.T.);
#62051=ORIENTED_EDGE('',*,*,#45688,.F.);
#62052=ORIENTED_EDGE('',*,*,#45689,.F.);
#62053=ORIENTED_EDGE('',*,*,#45690,.T.);
#62054=ORIENTED_EDGE('',*,*,#45691,.F.);
#62055=ORIENTED_EDGE('',*,*,#45690,.F.);
#62056=ORIENTED_EDGE('',*,*,#45692,.T.);
#62057=ORIENTED_EDGE('',*,*,#45693,.T.);
#62058=ORIENTED_EDGE('',*,*,#45694,.F.);
#62059=ORIENTED_EDGE('',*,*,#45694,.T.);
#62060=ORIENTED_EDGE('',*,*,#45695,.T.);
#62061=ORIENTED_EDGE('',*,*,#45691,.T.);
#62062=ORIENTED_EDGE('',*,*,#45695,.F.);
#62063=ORIENTED_EDGE('',*,*,#45696,.T.);
#62064=ORIENTED_EDGE('',*,*,#45686,.F.);
#62065=ORIENTED_EDGE('',*,*,#45697,.T.);
#62066=ORIENTED_EDGE('',*,*,#45394,.T.);
#62067=ORIENTED_EDGE('',*,*,#45698,.T.);
#62068=ORIENTED_EDGE('',*,*,#45699,.F.);
#62069=ORIENTED_EDGE('',*,*,#45700,.F.);
#62070=ORIENTED_EDGE('',*,*,#45701,.T.);
#62071=ORIENTED_EDGE('',*,*,#45702,.F.);
#62072=ORIENTED_EDGE('',*,*,#45703,.F.);
#62073=ORIENTED_EDGE('',*,*,#45704,.T.);
#62074=ORIENTED_EDGE('',*,*,#45705,.F.);
#62075=ORIENTED_EDGE('',*,*,#45706,.F.);
#62076=ORIENTED_EDGE('',*,*,#45707,.T.);
#62077=ORIENTED_EDGE('',*,*,#45708,.F.);
#62078=ORIENTED_EDGE('',*,*,#45709,.F.);
#62079=ORIENTED_EDGE('',*,*,#45700,.T.);
#62080=ORIENTED_EDGE('',*,*,#45710,.F.);
#62081=ORIENTED_EDGE('',*,*,#45711,.T.);
#62082=ORIENTED_EDGE('',*,*,#45712,.F.);
#62083=ORIENTED_EDGE('',*,*,#45701,.F.);
#62084=ORIENTED_EDGE('',*,*,#45712,.T.);
#62085=ORIENTED_EDGE('',*,*,#45713,.T.);
#62086=ORIENTED_EDGE('',*,*,#45714,.T.);
#62087=ORIENTED_EDGE('',*,*,#45715,.F.);
#62088=ORIENTED_EDGE('',*,*,#45702,.T.);
#62089=ORIENTED_EDGE('',*,*,#45715,.T.);
#62090=ORIENTED_EDGE('',*,*,#45716,.T.);
#62091=ORIENTED_EDGE('',*,*,#45717,.F.);
#62092=ORIENTED_EDGE('',*,*,#45706,.T.);
#62093=ORIENTED_EDGE('',*,*,#45718,.F.);
#62094=ORIENTED_EDGE('',*,*,#45719,.T.);
#62095=ORIENTED_EDGE('',*,*,#45720,.F.);
#62096=ORIENTED_EDGE('',*,*,#45707,.F.);
#62097=ORIENTED_EDGE('',*,*,#45720,.T.);
#62098=ORIENTED_EDGE('',*,*,#45721,.T.);
#62099=ORIENTED_EDGE('',*,*,#45722,.T.);
#62100=ORIENTED_EDGE('',*,*,#45723,.F.);
#62101=ORIENTED_EDGE('',*,*,#45708,.T.);
#62102=ORIENTED_EDGE('',*,*,#45723,.T.);
#62103=ORIENTED_EDGE('',*,*,#45724,.T.);
#62104=ORIENTED_EDGE('',*,*,#45725,.F.);
#62105=ORIENTED_EDGE('',*,*,#45721,.F.);
#62106=ORIENTED_EDGE('',*,*,#45726,.T.);
#62107=ORIENTED_EDGE('',*,*,#45722,.F.);
#62108=ORIENTED_EDGE('',*,*,#45727,.T.);
#62109=ORIENTED_EDGE('',*,*,#45727,.F.);
#62110=ORIENTED_EDGE('',*,*,#45719,.F.);
#62111=ORIENTED_EDGE('',*,*,#45728,.F.);
#62112=ORIENTED_EDGE('',*,*,#45724,.F.);
#62113=ORIENTED_EDGE('',*,*,#45726,.F.);
#62114=ORIENTED_EDGE('',*,*,#45713,.F.);
#62115=ORIENTED_EDGE('',*,*,#45729,.T.);
#62116=ORIENTED_EDGE('',*,*,#45714,.F.);
#62117=ORIENTED_EDGE('',*,*,#45730,.T.);
#62118=ORIENTED_EDGE('',*,*,#45730,.F.);
#62119=ORIENTED_EDGE('',*,*,#45711,.F.);
#62120=ORIENTED_EDGE('',*,*,#45731,.F.);
#62121=ORIENTED_EDGE('',*,*,#45716,.F.);
#62122=ORIENTED_EDGE('',*,*,#45729,.F.);
#62123=ORIENTED_EDGE('',*,*,#45732,.T.);
#62124=ORIENTED_EDGE('',*,*,#45733,.F.);
#62125=ORIENTED_EDGE('',*,*,#45734,.F.);
#62126=ORIENTED_EDGE('',*,*,#45735,.T.);
#62127=ORIENTED_EDGE('',*,*,#45736,.T.);
#62128=ORIENTED_EDGE('',*,*,#45735,.F.);
#62129=ORIENTED_EDGE('',*,*,#45737,.F.);
#62130=ORIENTED_EDGE('',*,*,#45738,.T.);
#62131=ORIENTED_EDGE('',*,*,#45739,.T.);
#62132=ORIENTED_EDGE('',*,*,#45738,.F.);
#62133=ORIENTED_EDGE('',*,*,#45740,.F.);
#62134=ORIENTED_EDGE('',*,*,#45741,.F.);
#62135=ORIENTED_EDGE('',*,*,#45742,.F.);
#62136=ORIENTED_EDGE('',*,*,#45704,.F.);
#62137=ORIENTED_EDGE('',*,*,#45743,.F.);
#62138=ORIENTED_EDGE('',*,*,#45732,.F.);
#62139=ORIENTED_EDGE('',*,*,#45736,.F.);
#62140=ORIENTED_EDGE('',*,*,#45739,.F.);
#62141=ORIENTED_EDGE('',*,*,#45744,.T.);
#62142=ORIENTED_EDGE('',*,*,#45745,.F.);
#62143=ORIENTED_EDGE('',*,*,#45746,.F.);
#62144=ORIENTED_EDGE('',*,*,#45747,.T.);
#62145=ORIENTED_EDGE('',*,*,#45748,.T.);
#62146=ORIENTED_EDGE('',*,*,#45747,.F.);
#62147=ORIENTED_EDGE('',*,*,#45749,.F.);
#62148=ORIENTED_EDGE('',*,*,#45750,.T.);
#62149=ORIENTED_EDGE('',*,*,#45751,.T.);
#62150=ORIENTED_EDGE('',*,*,#45750,.F.);
#62151=ORIENTED_EDGE('',*,*,#45752,.F.);
#62152=ORIENTED_EDGE('',*,*,#45753,.F.);
#62153=ORIENTED_EDGE('',*,*,#45754,.F.);
#62154=ORIENTED_EDGE('',*,*,#45698,.F.);
#62155=ORIENTED_EDGE('',*,*,#45755,.F.);
#62156=ORIENTED_EDGE('',*,*,#45744,.F.);
#62157=ORIENTED_EDGE('',*,*,#45748,.F.);
#62158=ORIENTED_EDGE('',*,*,#45751,.F.);
#62159=ORIENTED_EDGE('',*,*,#45756,.F.);
#62160=ORIENTED_EDGE('',*,*,#45757,.T.);
#62161=ORIENTED_EDGE('',*,*,#45758,.T.);
#62162=ORIENTED_EDGE('',*,*,#45669,.F.);
#62163=ORIENTED_EDGE('',*,*,#45759,.F.);
#62164=ORIENTED_EDGE('',*,*,#45205,.F.);
#62165=ORIENTED_EDGE('',*,*,#45760,.T.);
#62166=ORIENTED_EDGE('',*,*,#45642,.F.);
#62167=ORIENTED_EDGE('',*,*,#45761,.T.);
#62168=ORIENTED_EDGE('',*,*,#45391,.F.);
#62169=ORIENTED_EDGE('',*,*,#45762,.F.);
#62170=ORIENTED_EDGE('',*,*,#45407,.T.);
#62171=ORIENTED_EDGE('',*,*,#45763,.T.);
#62172=ORIENTED_EDGE('',*,*,#45764,.F.);
#62173=ORIENTED_EDGE('',*,*,#45390,.F.);
#62174=ORIENTED_EDGE('',*,*,#45397,.T.);
#62175=ORIENTED_EDGE('',*,*,#45408,.T.);
#62176=ORIENTED_EDGE('',*,*,#45762,.T.);
#62177=ORIENTED_EDGE('',*,*,#45765,.F.);
#62178=ORIENTED_EDGE('',*,*,#45764,.T.);
#62179=ORIENTED_EDGE('',*,*,#45766,.F.);
#62180=ORIENTED_EDGE('',*,*,#45767,.F.);
#62181=ORIENTED_EDGE('',*,*,#45768,.T.);
#62182=ORIENTED_EDGE('',*,*,#45769,.T.);
#62183=ORIENTED_EDGE('',*,*,#45770,.F.);
#62184=ORIENTED_EDGE('',*,*,#45771,.T.);
#62185=ORIENTED_EDGE('',*,*,#45772,.F.);
#62186=ORIENTED_EDGE('',*,*,#45773,.T.);
#62187=ORIENTED_EDGE('',*,*,#45774,.T.);
#62188=ORIENTED_EDGE('',*,*,#45775,.F.);
#62189=ORIENTED_EDGE('',*,*,#45776,.F.);
#62190=ORIENTED_EDGE('',*,*,#45775,.T.);
#62191=ORIENTED_EDGE('',*,*,#45777,.T.);
#62192=ORIENTED_EDGE('',*,*,#45778,.T.);
#62193=ORIENTED_EDGE('',*,*,#45779,.T.);
#62194=ORIENTED_EDGE('',*,*,#45780,.F.);
#62195=ORIENTED_EDGE('',*,*,#45770,.T.);
#62196=ORIENTED_EDGE('',*,*,#45781,.T.);
#62197=ORIENTED_EDGE('',*,*,#45773,.F.);
#62198=ORIENTED_EDGE('',*,*,#45782,.F.);
#62199=ORIENTED_EDGE('',*,*,#45783,.F.);
#62200=ORIENTED_EDGE('',*,*,#45784,.F.);
#62201=ORIENTED_EDGE('',*,*,#45785,.F.);
#62202=ORIENTED_EDGE('',*,*,#45786,.T.);
#62203=ORIENTED_EDGE('',*,*,#45783,.T.);
#62204=ORIENTED_EDGE('',*,*,#45786,.F.);
#62205=ORIENTED_EDGE('',*,*,#45787,.T.);
#62206=ORIENTED_EDGE('',*,*,#45788,.F.);
#62207=ORIENTED_EDGE('',*,*,#45693,.F.);
#62208=ORIENTED_EDGE('',*,*,#45789,.T.);
#62209=ORIENTED_EDGE('',*,*,#45790,.T.);
#62210=ORIENTED_EDGE('',*,*,#45791,.F.);
#62211=ORIENTED_EDGE('',*,*,#45792,.F.);
#62212=ORIENTED_EDGE('',*,*,#45771,.F.);
#62213=ORIENTED_EDGE('',*,*,#45780,.T.);
#62214=ORIENTED_EDGE('',*,*,#45779,.F.);
#62215=ORIENTED_EDGE('',*,*,#45793,.T.);
#62216=ORIENTED_EDGE('',*,*,#45794,.T.);
#62217=ORIENTED_EDGE('',*,*,#45791,.T.);
#62218=ORIENTED_EDGE('',*,*,#45795,.F.);
#62219=ORIENTED_EDGE('',*,*,#45790,.F.);
#62220=ORIENTED_EDGE('',*,*,#45796,.F.);
#62221=ORIENTED_EDGE('',*,*,#45793,.F.);
#62222=ORIENTED_EDGE('',*,*,#45782,.T.);
#62223=ORIENTED_EDGE('',*,*,#45772,.T.);
#62224=ORIENTED_EDGE('',*,*,#45776,.T.);
#62225=ORIENTED_EDGE('',*,*,#45797,.T.);
#62226=ORIENTED_EDGE('',*,*,#45798,.F.);
#62227=ORIENTED_EDGE('',*,*,#45799,.T.);
#62228=ORIENTED_EDGE('',*,*,#45797,.F.);
#62229=ORIENTED_EDGE('',*,*,#45778,.F.);
#62230=ORIENTED_EDGE('',*,*,#45800,.F.);
#62231=ORIENTED_EDGE('',*,*,#45801,.F.);
#62232=ORIENTED_EDGE('',*,*,#45802,.F.);
#62233=ORIENTED_EDGE('',*,*,#45803,.T.);
#62234=ORIENTED_EDGE('',*,*,#45804,.T.);
#62235=ORIENTED_EDGE('',*,*,#45787,.F.);
#62236=ORIENTED_EDGE('',*,*,#45795,.T.);
#62237=ORIENTED_EDGE('',*,*,#45799,.F.);
#62238=ORIENTED_EDGE('',*,*,#45805,.T.);
#62239=ORIENTED_EDGE('',*,*,#45806,.F.);
#62240=ORIENTED_EDGE('',*,*,#45802,.T.);
#62241=ORIENTED_EDGE('',*,*,#45798,.T.);
#62242=ORIENTED_EDGE('',*,*,#45761,.F.);
#62243=ORIENTED_EDGE('',*,*,#45765,.T.);
#62244=ORIENTED_EDGE('',*,*,#45807,.T.);
#62245=ORIENTED_EDGE('',*,*,#45392,.T.);
#62246=ORIENTED_EDGE('',*,*,#45808,.F.);
#62247=ORIENTED_EDGE('',*,*,#45803,.F.);
#62248=ORIENTED_EDGE('',*,*,#45806,.T.);
#62249=ORIENTED_EDGE('',*,*,#45809,.F.);
#62250=ORIENTED_EDGE('',*,*,#45810,.F.);
#62251=ORIENTED_EDGE('',*,*,#45811,.F.);
#62252=ORIENTED_EDGE('',*,*,#45809,.T.);
#62253=ORIENTED_EDGE('',*,*,#45805,.F.);
#62254=ORIENTED_EDGE('',*,*,#45801,.T.);
#62255=ORIENTED_EDGE('',*,*,#45812,.T.);
#62256=ORIENTED_EDGE('',*,*,#45813,.F.);
#62257=ORIENTED_EDGE('',*,*,#45814,.F.);
#62258=ORIENTED_EDGE('',*,*,#45678,.T.);
#62259=ORIENTED_EDGE('',*,*,#45815,.F.);
#62260=ORIENTED_EDGE('',*,*,#45816,.T.);
#62261=ORIENTED_EDGE('',*,*,#45817,.T.);
#62262=ORIENTED_EDGE('',*,*,#45810,.T.);
#62263=ORIENTED_EDGE('',*,*,#45818,.T.);
#62264=ORIENTED_EDGE('',*,*,#45813,.T.);
#62265=ORIENTED_EDGE('',*,*,#45819,.F.);
#62266=ORIENTED_EDGE('',*,*,#45820,.F.);
#62267=ORIENTED_EDGE('',*,*,#45676,.F.);
#62268=ORIENTED_EDGE('',*,*,#45821,.F.);
#62269=ORIENTED_EDGE('',*,*,#45822,.F.);
#62270=ORIENTED_EDGE('',*,*,#45821,.T.);
#62271=ORIENTED_EDGE('',*,*,#45675,.T.);
#62272=ORIENTED_EDGE('',*,*,#45814,.T.);
#62273=ORIENTED_EDGE('',*,*,#45818,.F.);
#62274=ORIENTED_EDGE('',*,*,#45812,.F.);
#62275=ORIENTED_EDGE('',*,*,#45800,.T.);
#62276=ORIENTED_EDGE('',*,*,#45777,.F.);
#62277=ORIENTED_EDGE('',*,*,#45774,.F.);
#62278=ORIENTED_EDGE('',*,*,#45781,.F.);
#62279=ORIENTED_EDGE('',*,*,#45769,.F.);
#62280=ORIENTED_EDGE('',*,*,#45823,.T.);
#62281=ORIENTED_EDGE('',*,*,#45824,.T.);
#62282=ORIENTED_EDGE('',*,*,#45766,.T.);
#62283=ORIENTED_EDGE('',*,*,#45763,.F.);
#62284=ORIENTED_EDGE('',*,*,#45406,.F.);
#62285=ORIENTED_EDGE('',*,*,#45825,.F.);
#62286=ORIENTED_EDGE('',*,*,#45403,.F.);
#62287=ORIENTED_EDGE('',*,*,#45681,.T.);
#62288=ORIENTED_EDGE('',*,*,#45826,.F.);
#62289=ORIENTED_EDGE('',*,*,#45827,.T.);
#62290=ORIENTED_EDGE('',*,*,#45673,.F.);
#62291=ORIENTED_EDGE('',*,*,#45828,.F.);
#62292=ORIENTED_EDGE('',*,*,#45829,.F.);
#62293=ORIENTED_EDGE('',*,*,#45826,.T.);
#62294=ORIENTED_EDGE('',*,*,#45680,.T.);
#62295=ORIENTED_EDGE('',*,*,#45830,.T.);
#62296=ORIENTED_EDGE('',*,*,#45831,.F.);
#62297=ORIENTED_EDGE('',*,*,#45832,.F.);
#62298=ORIENTED_EDGE('',*,*,#45613,.T.);
#62299=ORIENTED_EDGE('',*,*,#45833,.F.);
#62300=ORIENTED_EDGE('',*,*,#45830,.F.);
#62301=ORIENTED_EDGE('',*,*,#45679,.F.);
#62302=ORIENTED_EDGE('',*,*,#45401,.F.);
#62303=ORIENTED_EDGE('',*,*,#45834,.F.);
#62304=ORIENTED_EDGE('',*,*,#45835,.F.);
#62305=ORIENTED_EDGE('',*,*,#45671,.F.);
#62306=ORIENTED_EDGE('',*,*,#45836,.F.);
#62307=ORIENTED_EDGE('',*,*,#45757,.F.);
#62308=ORIENTED_EDGE('',*,*,#45837,.F.);
#62309=ORIENTED_EDGE('',*,*,#45816,.F.);
#62310=ORIENTED_EDGE('',*,*,#45815,.T.);
#62311=ORIENTED_EDGE('',*,*,#45677,.T.);
#62312=ORIENTED_EDGE('',*,*,#45820,.T.);
#62313=ORIENTED_EDGE('',*,*,#45834,.T.);
#62314=ORIENTED_EDGE('',*,*,#45819,.T.);
#62315=ORIENTED_EDGE('',*,*,#45822,.T.);
#62316=ORIENTED_EDGE('',*,*,#45838,.T.);
#62317=ORIENTED_EDGE('',*,*,#45829,.T.);
#62318=ORIENTED_EDGE('',*,*,#45839,.T.);
#62319=ORIENTED_EDGE('',*,*,#45404,.T.);
#62320=ORIENTED_EDGE('',*,*,#45825,.T.);
#62321=ORIENTED_EDGE('',*,*,#45831,.T.);
#62322=ORIENTED_EDGE('',*,*,#45833,.T.);
#62323=ORIENTED_EDGE('',*,*,#45400,.T.);
#62324=ORIENTED_EDGE('',*,*,#45840,.T.);
#62325=ORIENTED_EDGE('',*,*,#45832,.T.);
#62326=ORIENTED_EDGE('',*,*,#45840,.F.);
#62327=ORIENTED_EDGE('',*,*,#45399,.T.);
#62328=ORIENTED_EDGE('',*,*,#45586,.F.);
#62329=ORIENTED_EDGE('',*,*,#45587,.T.);
#62330=ORIENTED_EDGE('',*,*,#45387,.F.);
#62331=ORIENTED_EDGE('',*,*,#45395,.T.);
#62332=ORIENTED_EDGE('',*,*,#45697,.F.);
#62333=ORIENTED_EDGE('',*,*,#45685,.F.);
#62334=ORIENTED_EDGE('',*,*,#45696,.F.);
#62335=ORIENTED_EDGE('',*,*,#45393,.T.);
#62336=ORIENTED_EDGE('',*,*,#45807,.F.);
#62337=ORIENTED_EDGE('',*,*,#45767,.T.);
#62338=ORIENTED_EDGE('',*,*,#45824,.F.);
#62339=ORIENTED_EDGE('',*,*,#45405,.T.);
#62340=ORIENTED_EDGE('',*,*,#45839,.F.);
#62341=ORIENTED_EDGE('',*,*,#45828,.T.);
#62342=ORIENTED_EDGE('',*,*,#45672,.F.);
#62343=ORIENTED_EDGE('',*,*,#45835,.T.);
#62344=ORIENTED_EDGE('',*,*,#45838,.F.);
#62345=ORIENTED_EDGE('',*,*,#45823,.F.);
#62346=ORIENTED_EDGE('',*,*,#45768,.F.);
#62347=ORIENTED_EDGE('',*,*,#45792,.T.);
#62348=ORIENTED_EDGE('',*,*,#45794,.F.);
#62349=ORIENTED_EDGE('',*,*,#45796,.T.);
#62350=ORIENTED_EDGE('',*,*,#45789,.F.);
#62351=ORIENTED_EDGE('',*,*,#45692,.F.);
#62352=ORIENTED_EDGE('',*,*,#45788,.T.);
#62353=ORIENTED_EDGE('',*,*,#45804,.F.);
#62354=ORIENTED_EDGE('',*,*,#45808,.T.);
#62355=ORIENTED_EDGE('',*,*,#45811,.T.);
#62356=ORIENTED_EDGE('',*,*,#45817,.F.);
#62357=ORIENTED_EDGE('',*,*,#45837,.T.);
#62358=ORIENTED_EDGE('',*,*,#45756,.T.);
#62359=ORIENTED_EDGE('',*,*,#45668,.F.);
#62360=ORIENTED_EDGE('',*,*,#45630,.T.);
#62361=ORIENTED_EDGE('',*,*,#45663,.T.);
#62362=ORIENTED_EDGE('',*,*,#45659,.F.);
#62363=ORIENTED_EDGE('',*,*,#45841,.T.);
#62364=ORIENTED_EDGE('',*,*,#45619,.T.);
#62365=ORIENTED_EDGE('',*,*,#45615,.T.);
#62366=ORIENTED_EDGE('',*,*,#45606,.F.);
#62367=ORIENTED_EDGE('',*,*,#45593,.T.);
#62368=ORIENTED_EDGE('',*,*,#45590,.F.);
#62369=ORIENTED_EDGE('',*,*,#45601,.T.);
#62370=ORIENTED_EDGE('',*,*,#45611,.F.);
#62371=ORIENTED_EDGE('',*,*,#45614,.T.);
#62372=ORIENTED_EDGE('',*,*,#45623,.T.);
#62373=ORIENTED_EDGE('',*,*,#45842,.T.);
#62374=ORIENTED_EDGE('',*,*,#45740,.T.);
#62375=ORIENTED_EDGE('',*,*,#45737,.T.);
#62376=ORIENTED_EDGE('',*,*,#45734,.T.);
#62377=ORIENTED_EDGE('',*,*,#45843,.T.);
#62378=ORIENTED_EDGE('',*,*,#45752,.T.);
#62379=ORIENTED_EDGE('',*,*,#45749,.T.);
#62380=ORIENTED_EDGE('',*,*,#45746,.T.);
#62381=ORIENTED_EDGE('',*,*,#45844,.F.);
#62382=ORIENTED_EDGE('',*,*,#45620,.T.);
#62383=ORIENTED_EDGE('',*,*,#45841,.F.);
#62384=ORIENTED_EDGE('',*,*,#45662,.F.);
#62385=ORIENTED_EDGE('',*,*,#45845,.F.);
#62386=ORIENTED_EDGE('',*,*,#45657,.F.);
#62387=ORIENTED_EDGE('',*,*,#45689,.T.);
#62388=ORIENTED_EDGE('',*,*,#45682,.T.);
#62389=ORIENTED_EDGE('',*,*,#45785,.T.);
#62390=ORIENTED_EDGE('',*,*,#45846,.T.);
#62391=ORIENTED_EDGE('',*,*,#45847,.T.);
#62392=ORIENTED_EDGE('',*,*,#45848,.T.);
#62393=ORIENTED_EDGE('',*,*,#45849,.T.);
#62394=ORIENTED_EDGE('',*,*,#45850,.T.);
#62395=ORIENTED_EDGE('',*,*,#45851,.T.);
#62396=ORIENTED_EDGE('',*,*,#45852,.T.);
#62397=ORIENTED_EDGE('',*,*,#45056,.T.);
#62398=ORIENTED_EDGE('',*,*,#45853,.T.);
#62399=ORIENTED_EDGE('',*,*,#45854,.T.);
#62400=ORIENTED_EDGE('',*,*,#45855,.F.);
#62401=ORIENTED_EDGE('',*,*,#45856,.T.);
#62402=ORIENTED_EDGE('',*,*,#45106,.F.);
#62403=ORIENTED_EDGE('',*,*,#45857,.F.);
#62404=ORIENTED_EDGE('',*,*,#45858,.T.);
#62405=ORIENTED_EDGE('',*,*,#45859,.F.);
#62406=ORIENTED_EDGE('',*,*,#45860,.F.);
#62407=ORIENTED_EDGE('',*,*,#45861,.F.);
#62408=ORIENTED_EDGE('',*,*,#45143,.T.);
#62409=ORIENTED_EDGE('',*,*,#45862,.F.);
#62410=ORIENTED_EDGE('',*,*,#45849,.F.);
#62411=ORIENTED_EDGE('',*,*,#45863,.F.);
#62412=ORIENTED_EDGE('',*,*,#45851,.F.);
#62413=ORIENTED_EDGE('',*,*,#45864,.F.);
#62414=ORIENTED_EDGE('',*,*,#45856,.F.);
#62415=ORIENTED_EDGE('',*,*,#45865,.T.);
#62416=ORIENTED_EDGE('',*,*,#45089,.F.);
#62417=ORIENTED_EDGE('',*,*,#45095,.F.);
#62418=ORIENTED_EDGE('',*,*,#45107,.T.);
#62419=ORIENTED_EDGE('',*,*,#45866,.F.);
#62420=ORIENTED_EDGE('',*,*,#45867,.F.);
#62421=ORIENTED_EDGE('',*,*,#45868,.F.);
#62422=ORIENTED_EDGE('',*,*,#45054,.T.);
#62423=ORIENTED_EDGE('',*,*,#45869,.F.);
#62424=ORIENTED_EDGE('',*,*,#45870,.F.);
#62425=ORIENTED_EDGE('',*,*,#45871,.T.);
#62426=ORIENTED_EDGE('',*,*,#45872,.T.);
#62427=ORIENTED_EDGE('',*,*,#45873,.T.);
#62428=ORIENTED_EDGE('',*,*,#45873,.F.);
#62429=ORIENTED_EDGE('',*,*,#45874,.F.);
#62430=ORIENTED_EDGE('',*,*,#45875,.F.);
#62431=ORIENTED_EDGE('',*,*,#45876,.T.);
#62432=ORIENTED_EDGE('',*,*,#45877,.T.);
#62433=ORIENTED_EDGE('',*,*,#45878,.T.);
#62434=ORIENTED_EDGE('',*,*,#45879,.T.);
#62435=ORIENTED_EDGE('',*,*,#45880,.F.);
#62436=ORIENTED_EDGE('',*,*,#45058,.T.);
#62437=ORIENTED_EDGE('',*,*,#45881,.T.);
#62438=ORIENTED_EDGE('',*,*,#45882,.T.);
#62439=ORIENTED_EDGE('',*,*,#45871,.F.);
#62440=ORIENTED_EDGE('',*,*,#45883,.T.);
#62441=ORIENTED_EDGE('',*,*,#45884,.T.);
#62442=ORIENTED_EDGE('',*,*,#45885,.T.);
#62443=ORIENTED_EDGE('',*,*,#45882,.F.);
#62444=ORIENTED_EDGE('',*,*,#45886,.F.);
#62445=ORIENTED_EDGE('',*,*,#45887,.T.);
#62446=ORIENTED_EDGE('',*,*,#45888,.T.);
#62447=ORIENTED_EDGE('',*,*,#45889,.T.);
#62448=ORIENTED_EDGE('',*,*,#45888,.F.);
#62449=ORIENTED_EDGE('',*,*,#45889,.F.);
#62450=ORIENTED_EDGE('',*,*,#45890,.F.);
#62451=ORIENTED_EDGE('',*,*,#45887,.F.);
#62452=ORIENTED_EDGE('',*,*,#45891,.T.);
#62453=ORIENTED_EDGE('',*,*,#45892,.T.);
#62454=ORIENTED_EDGE('',*,*,#45891,.F.);
#62455=ORIENTED_EDGE('',*,*,#45890,.T.);
#62456=ORIENTED_EDGE('',*,*,#45893,.T.);
#62457=ORIENTED_EDGE('',*,*,#45894,.T.);
#62458=ORIENTED_EDGE('',*,*,#45893,.F.);
#62459=ORIENTED_EDGE('',*,*,#45895,.F.);
#62460=ORIENTED_EDGE('',*,*,#45896,.T.);
#62461=ORIENTED_EDGE('',*,*,#45897,.T.);
#62462=ORIENTED_EDGE('',*,*,#45896,.F.);
#62463=ORIENTED_EDGE('',*,*,#45865,.F.);
#62464=ORIENTED_EDGE('',*,*,#45855,.T.);
#62465=ORIENTED_EDGE('',*,*,#45898,.T.);
#62466=ORIENTED_EDGE('',*,*,#45090,.T.);
#62467=ORIENTED_EDGE('',*,*,#45899,.T.);
#62468=ORIENTED_EDGE('',*,*,#45900,.T.);
#62469=ORIENTED_EDGE('',*,*,#45901,.F.);
#62470=ORIENTED_EDGE('',*,*,#45900,.F.);
#62471=ORIENTED_EDGE('',*,*,#45123,.F.);
#62472=ORIENTED_EDGE('',*,*,#45902,.T.);
#62473=ORIENTED_EDGE('',*,*,#45903,.T.);
#62474=ORIENTED_EDGE('',*,*,#45146,.T.);
#62475=ORIENTED_EDGE('',*,*,#45904,.T.);
#62476=ORIENTED_EDGE('',*,*,#45905,.T.);
#62477=ORIENTED_EDGE('',*,*,#45906,.T.);
#62478=ORIENTED_EDGE('',*,*,#45905,.F.);
#62479=ORIENTED_EDGE('',*,*,#45906,.F.);
#62480=ORIENTED_EDGE('',*,*,#45907,.T.);
#62481=ORIENTED_EDGE('',*,*,#45908,.T.);
#62482=ORIENTED_EDGE('',*,*,#45907,.F.);
#62483=ORIENTED_EDGE('',*,*,#45909,.T.);
#62484=ORIENTED_EDGE('',*,*,#45910,.T.);
#62485=ORIENTED_EDGE('',*,*,#45911,.T.);
#62486=ORIENTED_EDGE('',*,*,#45912,.T.);
#62487=ORIENTED_EDGE('',*,*,#45913,.F.);
#62488=ORIENTED_EDGE('',*,*,#45914,.F.);
#62489=ORIENTED_EDGE('',*,*,#45915,.F.);
#62490=ORIENTED_EDGE('',*,*,#45916,.F.);
#62491=ORIENTED_EDGE('',*,*,#45917,.T.);
#62492=ORIENTED_EDGE('',*,*,#45918,.T.);
#62493=ORIENTED_EDGE('',*,*,#45913,.T.);
#62494=ORIENTED_EDGE('',*,*,#45919,.T.);
#62495=ORIENTED_EDGE('',*,*,#45102,.T.);
#62496=ORIENTED_EDGE('',*,*,#44959,.T.);
#62497=ORIENTED_EDGE('',*,*,#45920,.T.);
#62498=ORIENTED_EDGE('',*,*,#45921,.T.);
#62499=ORIENTED_EDGE('',*,*,#45920,.F.);
#62500=ORIENTED_EDGE('',*,*,#44958,.F.);
#62501=ORIENTED_EDGE('',*,*,#45922,.F.);
#62502=ORIENTED_EDGE('',*,*,#45923,.F.);
#62503=ORIENTED_EDGE('',*,*,#45924,.F.);
#62504=ORIENTED_EDGE('',*,*,#45922,.T.);
#62505=ORIENTED_EDGE('',*,*,#44957,.F.);
#62506=ORIENTED_EDGE('',*,*,#45925,.F.);
#62507=ORIENTED_EDGE('',*,*,#45011,.F.);
#62508=ORIENTED_EDGE('',*,*,#45926,.F.);
#62509=ORIENTED_EDGE('',*,*,#45927,.T.);
#62510=ORIENTED_EDGE('',*,*,#45928,.T.);
#62511=ORIENTED_EDGE('',*,*,#45929,.F.);
#62512=ORIENTED_EDGE('',*,*,#45930,.F.);
#62513=ORIENTED_EDGE('',*,*,#45931,.T.);
#62514=ORIENTED_EDGE('',*,*,#45932,.F.);
#62515=ORIENTED_EDGE('',*,*,#45933,.T.);
#62516=ORIENTED_EDGE('',*,*,#45934,.F.);
#62517=ORIENTED_EDGE('',*,*,#45933,.F.);
#62518=ORIENTED_EDGE('',*,*,#45014,.F.);
#62519=ORIENTED_EDGE('',*,*,#45935,.F.);
#62520=ORIENTED_EDGE('',*,*,#45936,.F.);
#62521=ORIENTED_EDGE('',*,*,#45926,.T.);
#62522=ORIENTED_EDGE('',*,*,#45016,.F.);
#62523=ORIENTED_EDGE('',*,*,#45031,.T.);
#62524=ORIENTED_EDGE('',*,*,#45937,.F.);
#62525=ORIENTED_EDGE('',*,*,#45938,.T.);
#62526=ORIENTED_EDGE('',*,*,#45939,.T.);
#62527=ORIENTED_EDGE('',*,*,#45935,.T.);
#62528=ORIENTED_EDGE('',*,*,#45486,.F.);
#62529=ORIENTED_EDGE('',*,*,#45457,.T.);
#62530=ORIENTED_EDGE('',*,*,#45940,.T.);
#62531=ORIENTED_EDGE('',*,*,#45941,.T.);
#62532=ORIENTED_EDGE('',*,*,#45942,.F.);
#62533=ORIENTED_EDGE('',*,*,#45943,.T.);
#62534=ORIENTED_EDGE('',*,*,#45930,.T.);
#62535=ORIENTED_EDGE('',*,*,#45937,.T.);
#62536=ORIENTED_EDGE('',*,*,#45030,.T.);
#62537=ORIENTED_EDGE('',*,*,#45944,.T.);
#62538=ORIENTED_EDGE('',*,*,#45945,.T.);
#62539=ORIENTED_EDGE('',*,*,#45946,.F.);
#62540=ORIENTED_EDGE('',*,*,#45491,.F.);
#62541=ORIENTED_EDGE('',*,*,#45508,.T.);
#62542=ORIENTED_EDGE('',*,*,#45947,.T.);
#62543=ORIENTED_EDGE('',*,*,#45459,.T.);
#62544=ORIENTED_EDGE('',*,*,#45449,.T.);
#62545=ORIENTED_EDGE('',*,*,#45948,.T.);
#62546=ORIENTED_EDGE('',*,*,#45949,.F.);
#62547=ORIENTED_EDGE('',*,*,#45950,.T.);
#62548=ORIENTED_EDGE('',*,*,#45948,.F.);
#62549=ORIENTED_EDGE('',*,*,#45951,.T.);
#62550=ORIENTED_EDGE('',*,*,#45952,.T.);
#62551=ORIENTED_EDGE('',*,*,#45951,.F.);
#62552=ORIENTED_EDGE('',*,*,#45950,.F.);
#62553=ORIENTED_EDGE('',*,*,#45953,.T.);
#62554=ORIENTED_EDGE('',*,*,#45954,.T.);
#62555=ORIENTED_EDGE('',*,*,#45953,.F.);
#62556=ORIENTED_EDGE('',*,*,#45952,.F.);
#62557=ORIENTED_EDGE('',*,*,#45954,.F.);
#62558=ORIENTED_EDGE('',*,*,#45955,.T.);
#62559=ORIENTED_EDGE('',*,*,#45956,.T.);
#62560=ORIENTED_EDGE('',*,*,#45944,.F.);
#62561=ORIENTED_EDGE('',*,*,#45033,.T.);
#62562=ORIENTED_EDGE('',*,*,#45957,.T.);
#62563=ORIENTED_EDGE('',*,*,#45958,.F.);
#62564=ORIENTED_EDGE('',*,*,#45912,.F.);
#62565=ORIENTED_EDGE('',*,*,#45959,.T.);
#62566=ORIENTED_EDGE('',*,*,#45915,.T.);
#62567=ORIENTED_EDGE('',*,*,#45960,.F.);
#62568=ORIENTED_EDGE('',*,*,#45961,.T.);
#62569=ORIENTED_EDGE('',*,*,#45093,.F.);
#62570=ORIENTED_EDGE('',*,*,#45961,.F.);
#62571=ORIENTED_EDGE('',*,*,#45908,.F.);
#62572=ORIENTED_EDGE('',*,*,#45960,.T.);
#62573=ORIENTED_EDGE('',*,*,#45934,.T.);
#62574=ORIENTED_EDGE('',*,*,#45962,.T.);
#62575=ORIENTED_EDGE('',*,*,#45892,.F.);
#62576=ORIENTED_EDGE('',*,*,#45962,.F.);
#62577=ORIENTED_EDGE('',*,*,#45963,.F.);
#62578=ORIENTED_EDGE('',*,*,#45964,.F.);
#62579=ORIENTED_EDGE('',*,*,#45965,.T.);
#62580=ORIENTED_EDGE('',*,*,#45966,.T.);
#62581=ORIENTED_EDGE('',*,*,#45964,.T.);
#62582=ORIENTED_EDGE('',*,*,#45966,.F.);
#62583=ORIENTED_EDGE('',*,*,#45967,.T.);
#62584=ORIENTED_EDGE('',*,*,#45092,.T.);
#62585=ORIENTED_EDGE('',*,*,#45968,.T.);
#62586=ORIENTED_EDGE('',*,*,#45969,.T.);
#62587=ORIENTED_EDGE('',*,*,#45067,.T.);
#62588=ORIENTED_EDGE('',*,*,#45970,.T.);
#62589=ORIENTED_EDGE('',*,*,#45869,.T.);
#62590=ORIENTED_EDGE('',*,*,#45053,.T.);
#62591=ORIENTED_EDGE('',*,*,#45065,.T.);
#62592=ORIENTED_EDGE('',*,*,#45070,.T.);
#62593=ORIENTED_EDGE('',*,*,#45971,.T.);
#62594=ORIENTED_EDGE('',*,*,#45972,.T.);
#62595=ORIENTED_EDGE('',*,*,#45973,.T.);
#62596=ORIENTED_EDGE('',*,*,#45862,.T.);
#62597=ORIENTED_EDGE('',*,*,#45142,.T.);
#62598=ORIENTED_EDGE('',*,*,#45147,.T.);
#62599=ORIENTED_EDGE('',*,*,#45903,.F.);
#62600=ORIENTED_EDGE('',*,*,#45974,.T.);
#62601=ORIENTED_EDGE('',*,*,#45897,.F.);
#62602=ORIENTED_EDGE('',*,*,#45899,.F.);
#62603=ORIENTED_EDGE('',*,*,#45894,.F.);
#62604=ORIENTED_EDGE('',*,*,#45975,.T.);
#62605=ORIENTED_EDGE('',*,*,#45963,.T.);
#62606=ORIENTED_EDGE('',*,*,#45975,.F.);
#62607=ORIENTED_EDGE('',*,*,#45976,.F.);
#62608=ORIENTED_EDGE('',*,*,#45977,.F.);
#62609=ORIENTED_EDGE('',*,*,#45877,.F.);
#62610=ORIENTED_EDGE('',*,*,#45978,.F.);
#62611=ORIENTED_EDGE('',*,*,#45080,.F.);
#62612=ORIENTED_EDGE('',*,*,#45979,.F.);
#62613=ORIENTED_EDGE('',*,*,#45068,.F.);
#62614=ORIENTED_EDGE('',*,*,#45969,.F.);
#62615=ORIENTED_EDGE('',*,*,#45870,.T.);
#62616=ORIENTED_EDGE('',*,*,#45879,.F.);
#62617=ORIENTED_EDGE('',*,*,#45980,.F.);
#62618=ORIENTED_EDGE('',*,*,#45117,.T.);
#62619=ORIENTED_EDGE('',*,*,#45981,.F.);
#62620=ORIENTED_EDGE('',*,*,#45061,.F.);
#62621=ORIENTED_EDGE('',*,*,#45982,.F.);
#62622=ORIENTED_EDGE('',*,*,#45883,.F.);
#62623=ORIENTED_EDGE('',*,*,#45062,.F.);
#62624=ORIENTED_EDGE('',*,*,#45981,.T.);
#62625=ORIENTED_EDGE('',*,*,#45983,.T.);
#62626=ORIENTED_EDGE('',*,*,#45060,.F.);
#62627=ORIENTED_EDGE('',*,*,#45984,.T.);
#62628=ORIENTED_EDGE('',*,*,#45884,.F.);
#62629=ORIENTED_EDGE('',*,*,#45982,.T.);
#62630=ORIENTED_EDGE('',*,*,#45880,.T.);
#62631=ORIENTED_EDGE('',*,*,#45885,.F.);
#62632=ORIENTED_EDGE('',*,*,#45984,.F.);
#62633=ORIENTED_EDGE('',*,*,#45059,.F.);
#62634=ORIENTED_EDGE('',*,*,#45985,.F.);
#62635=ORIENTED_EDGE('',*,*,#45986,.T.);
#62636=ORIENTED_EDGE('',*,*,#45875,.T.);
#62637=ORIENTED_EDGE('',*,*,#45987,.F.);
#62638=ORIENTED_EDGE('',*,*,#45988,.F.);
#62639=ORIENTED_EDGE('',*,*,#45989,.F.);
#62640=ORIENTED_EDGE('',*,*,#45985,.T.);
#62641=ORIENTED_EDGE('',*,*,#45990,.F.);
#62642=ORIENTED_EDGE('',*,*,#45097,.T.);
#62643=ORIENTED_EDGE('',*,*,#45991,.F.);
#62644=ORIENTED_EDGE('',*,*,#45992,.F.);
#62645=ORIENTED_EDGE('',*,*,#45993,.T.);
#62646=ORIENTED_EDGE('',*,*,#45994,.F.);
#62647=ORIENTED_EDGE('',*,*,#45995,.F.);
#62648=ORIENTED_EDGE('',*,*,#45996,.T.);
#62649=ORIENTED_EDGE('',*,*,#45997,.F.);
#62650=ORIENTED_EDGE('',*,*,#45998,.F.);
#62651=ORIENTED_EDGE('',*,*,#45999,.F.);
#62652=ORIENTED_EDGE('',*,*,#45997,.T.);
#62653=ORIENTED_EDGE('',*,*,#46000,.T.);
#62654=ORIENTED_EDGE('',*,*,#45992,.T.);
#62655=ORIENTED_EDGE('',*,*,#46001,.F.);
#62656=ORIENTED_EDGE('',*,*,#45137,.T.);
#62657=ORIENTED_EDGE('',*,*,#45145,.F.);
#62658=ORIENTED_EDGE('',*,*,#46002,.T.);
#62659=ORIENTED_EDGE('',*,*,#46003,.F.);
#62660=ORIENTED_EDGE('',*,*,#46004,.F.);
#62661=ORIENTED_EDGE('',*,*,#46005,.F.);
#62662=ORIENTED_EDGE('',*,*,#46002,.F.);
#62663=ORIENTED_EDGE('',*,*,#45144,.T.);
#62664=ORIENTED_EDGE('',*,*,#45861,.T.);
#62665=ORIENTED_EDGE('',*,*,#46006,.T.);
#62666=ORIENTED_EDGE('',*,*,#45858,.F.);
#62667=ORIENTED_EDGE('',*,*,#46007,.F.);
#62668=ORIENTED_EDGE('',*,*,#46008,.F.);
#62669=ORIENTED_EDGE('',*,*,#46007,.T.);
#62670=ORIENTED_EDGE('',*,*,#45857,.T.);
#62671=ORIENTED_EDGE('',*,*,#45105,.T.);
#62672=ORIENTED_EDGE('',*,*,#46009,.F.);
#62673=ORIENTED_EDGE('',*,*,#46001,.T.);
#62674=ORIENTED_EDGE('',*,*,#46010,.F.);
#62675=ORIENTED_EDGE('',*,*,#46009,.T.);
#62676=ORIENTED_EDGE('',*,*,#45994,.T.);
#62677=ORIENTED_EDGE('',*,*,#46011,.T.);
#62678=ORIENTED_EDGE('',*,*,#45138,.T.);
#62679=ORIENTED_EDGE('',*,*,#46012,.F.);
#62680=ORIENTED_EDGE('',*,*,#46008,.T.);
#62681=ORIENTED_EDGE('',*,*,#46013,.F.);
#62682=ORIENTED_EDGE('',*,*,#46010,.T.);
#62683=ORIENTED_EDGE('',*,*,#46005,.T.);
#62684=ORIENTED_EDGE('',*,*,#46014,.F.);
#62685=ORIENTED_EDGE('',*,*,#45991,.T.);
#62686=ORIENTED_EDGE('',*,*,#46015,.F.);
#62687=ORIENTED_EDGE('',*,*,#45999,.T.);
#62688=ORIENTED_EDGE('',*,*,#46014,.T.);
#62689=ORIENTED_EDGE('',*,*,#46004,.T.);
#62690=ORIENTED_EDGE('',*,*,#46012,.T.);
#62691=ORIENTED_EDGE('',*,*,#45998,.T.);
#62692=ORIENTED_EDGE('',*,*,#46015,.T.);
#62693=ORIENTED_EDGE('',*,*,#46003,.T.);
#62694=ORIENTED_EDGE('',*,*,#46013,.T.);
#62695=ORIENTED_EDGE('',*,*,#45104,.T.);
#62696=ORIENTED_EDGE('',*,*,#46016,.T.);
#62697=ORIENTED_EDGE('',*,*,#45995,.T.);
#62698=ORIENTED_EDGE('',*,*,#46017,.F.);
#62699=ORIENTED_EDGE('',*,*,#45972,.F.);
#62700=ORIENTED_EDGE('',*,*,#46018,.T.);
#62701=ORIENTED_EDGE('',*,*,#45976,.T.);
#62702=ORIENTED_EDGE('',*,*,#45968,.F.);
#62703=ORIENTED_EDGE('',*,*,#45091,.T.);
#62704=ORIENTED_EDGE('',*,*,#45898,.F.);
#62705=ORIENTED_EDGE('',*,*,#45854,.F.);
#62706=ORIENTED_EDGE('',*,*,#46019,.F.);
#62707=ORIENTED_EDGE('',*,*,#46020,.F.);
#62708=ORIENTED_EDGE('',*,*,#45866,.T.);
#62709=ORIENTED_EDGE('',*,*,#45970,.F.);
#62710=ORIENTED_EDGE('',*,*,#46017,.T.);
#62711=ORIENTED_EDGE('',*,*,#45126,.F.);
#62712=ORIENTED_EDGE('',*,*,#46021,.F.);
#62713=ORIENTED_EDGE('',*,*,#46022,.F.);
#62714=ORIENTED_EDGE('',*,*,#45847,.F.);
#62715=ORIENTED_EDGE('',*,*,#46023,.F.);
#62716=ORIENTED_EDGE('',*,*,#46024,.F.);
#62717=ORIENTED_EDGE('',*,*,#45974,.F.);
#62718=ORIENTED_EDGE('',*,*,#45902,.F.);
#62719=ORIENTED_EDGE('',*,*,#46025,.T.);
#62720=ORIENTED_EDGE('',*,*,#46023,.T.);
#62721=ORIENTED_EDGE('',*,*,#45846,.F.);
#62722=ORIENTED_EDGE('',*,*,#45864,.T.);
#62723=ORIENTED_EDGE('',*,*,#45850,.F.);
#62724=ORIENTED_EDGE('',*,*,#45055,.T.);
#62725=ORIENTED_EDGE('',*,*,#45868,.T.);
#62726=ORIENTED_EDGE('',*,*,#45867,.T.);
#62727=ORIENTED_EDGE('',*,*,#46020,.T.);
#62728=ORIENTED_EDGE('',*,*,#46019,.T.);
#62729=ORIENTED_EDGE('',*,*,#45853,.F.);
#62730=ORIENTED_EDGE('',*,*,#46006,.F.);
#62731=ORIENTED_EDGE('',*,*,#45860,.T.);
#62732=ORIENTED_EDGE('',*,*,#45973,.F.);
#62733=ORIENTED_EDGE('',*,*,#46024,.T.);
#62734=ORIENTED_EDGE('',*,*,#46025,.F.);
#62735=ORIENTED_EDGE('',*,*,#45859,.T.);
#62736=ORIENTED_EDGE('',*,*,#46026,.F.);
#62737=ORIENTED_EDGE('',*,*,#45988,.T.);
#62738=ORIENTED_EDGE('',*,*,#46027,.F.);
#62739=ORIENTED_EDGE('',*,*,#46028,.T.);
#62740=ORIENTED_EDGE('',*,*,#45082,.F.);
#62741=ORIENTED_EDGE('',*,*,#46029,.T.);
#62742=ORIENTED_EDGE('',*,*,#46027,.T.);
#62743=ORIENTED_EDGE('',*,*,#45096,.T.);
#62744=ORIENTED_EDGE('',*,*,#45270,.F.);
#62745=ORIENTED_EDGE('',*,*,#46030,.F.);
#62746=ORIENTED_EDGE('',*,*,#46031,.F.);
#62747=ORIENTED_EDGE('',*,*,#46032,.F.);
#62748=ORIENTED_EDGE('',*,*,#45267,.F.);
#62749=ORIENTED_EDGE('',*,*,#46032,.T.);
#62750=ORIENTED_EDGE('',*,*,#46033,.T.);
#62751=ORIENTED_EDGE('',*,*,#45309,.T.);
#62752=ORIENTED_EDGE('',*,*,#45273,.F.);
#62753=ORIENTED_EDGE('',*,*,#46034,.F.);
#62754=ORIENTED_EDGE('',*,*,#46035,.F.);
#62755=ORIENTED_EDGE('',*,*,#46030,.T.);
#62756=ORIENTED_EDGE('',*,*,#45129,.F.);
#62757=ORIENTED_EDGE('',*,*,#45140,.T.);
#62758=ORIENTED_EDGE('',*,*,#46036,.T.);
#62759=ORIENTED_EDGE('',*,*,#46021,.T.);
#62760=ORIENTED_EDGE('',*,*,#46037,.F.);
#62761=ORIENTED_EDGE('',*,*,#46038,.F.);
#62762=ORIENTED_EDGE('',*,*,#46039,.F.);
#62763=ORIENTED_EDGE('',*,*,#46040,.T.);
#62764=ORIENTED_EDGE('',*,*,#45925,.T.);
#62765=ORIENTED_EDGE('',*,*,#44956,.F.);
#62766=ORIENTED_EDGE('',*,*,#45932,.T.);
#62767=ORIENTED_EDGE('',*,*,#46041,.F.);
#62768=ORIENTED_EDGE('',*,*,#46042,.T.);
#62769=ORIENTED_EDGE('',*,*,#46043,.T.);
#62770=ORIENTED_EDGE('',*,*,#46039,.T.);
#62771=ORIENTED_EDGE('',*,*,#46044,.F.);
#62772=ORIENTED_EDGE('',*,*,#46045,.T.);
#62773=ORIENTED_EDGE('',*,*,#46046,.T.);
#62774=ORIENTED_EDGE('',*,*,#46047,.T.);
#62775=ORIENTED_EDGE('',*,*,#46048,.F.);
#62776=ORIENTED_EDGE('',*,*,#46049,.F.);
#62777=ORIENTED_EDGE('',*,*,#46050,.F.);
#62778=ORIENTED_EDGE('',*,*,#46045,.F.);
#62779=ORIENTED_EDGE('',*,*,#46051,.F.);
#62780=ORIENTED_EDGE('',*,*,#46052,.T.);
#62781=ORIENTED_EDGE('',*,*,#46053,.T.);
#62782=ORIENTED_EDGE('',*,*,#46049,.T.);
#62783=ORIENTED_EDGE('',*,*,#46054,.T.);
#62784=ORIENTED_EDGE('',*,*,#46055,.T.);
#62785=ORIENTED_EDGE('',*,*,#45037,.T.);
#62786=ORIENTED_EDGE('',*,*,#45942,.T.);
#62787=ORIENTED_EDGE('',*,*,#45929,.T.);
#62788=ORIENTED_EDGE('',*,*,#46056,.F.);
#62789=ORIENTED_EDGE('',*,*,#46057,.T.);
#62790=ORIENTED_EDGE('',*,*,#46058,.F.);
#62791=ORIENTED_EDGE('',*,*,#45945,.F.);
#62792=ORIENTED_EDGE('',*,*,#45956,.F.);
#62793=ORIENTED_EDGE('',*,*,#46059,.T.);
#62794=ORIENTED_EDGE('',*,*,#46060,.F.);
#62795=ORIENTED_EDGE('',*,*,#45648,.T.);
#62796=ORIENTED_EDGE('',*,*,#45646,.F.);
#62797=ORIENTED_EDGE('',*,*,#45655,.T.);
#62798=ORIENTED_EDGE('',*,*,#45658,.F.);
#62799=ORIENTED_EDGE('',*,*,#45845,.T.);
#62800=ORIENTED_EDGE('',*,*,#45661,.F.);
#62801=ORIENTED_EDGE('',*,*,#45664,.T.);
#62802=ORIENTED_EDGE('',*,*,#45628,.F.);
#62803=ORIENTED_EDGE('',*,*,#45637,.T.);
#62804=ORIENTED_EDGE('',*,*,#45639,.T.);
#62805=ORIENTED_EDGE('',*,*,#45640,.F.);
#62806=ORIENTED_EDGE('',*,*,#45250,.T.);
#62807=ORIENTED_EDGE('',*,*,#45253,.F.);
#62808=ORIENTED_EDGE('',*,*,#45255,.T.);
#62809=ORIENTED_EDGE('',*,*,#45257,.F.);
#62810=ORIENTED_EDGE('',*,*,#45259,.T.);
#62811=ORIENTED_EDGE('',*,*,#45261,.T.);
#62812=ORIENTED_EDGE('',*,*,#45652,.F.);
#62813=ORIENTED_EDGE('',*,*,#45665,.T.);
#62814=ORIENTED_EDGE('',*,*,#45276,.F.);
#62815=ORIENTED_EDGE('',*,*,#46061,.T.);
#62816=ORIENTED_EDGE('',*,*,#46062,.T.);
#62817=ORIENTED_EDGE('',*,*,#46034,.T.);
#62818=ORIENTED_EDGE('',*,*,#44976,.F.);
#62819=ORIENTED_EDGE('',*,*,#44968,.T.);
#62820=ORIENTED_EDGE('',*,*,#46063,.F.);
#62821=ORIENTED_EDGE('',*,*,#45001,.T.);
#62822=ORIENTED_EDGE('',*,*,#44941,.F.);
#62823=ORIENTED_EDGE('',*,*,#44962,.F.);
#62824=ORIENTED_EDGE('',*,*,#46064,.F.);
#62825=ORIENTED_EDGE('',*,*,#46065,.F.);
#62826=ORIENTED_EDGE('',*,*,#46066,.F.);
#62827=ORIENTED_EDGE('',*,*,#46064,.T.);
#62828=ORIENTED_EDGE('',*,*,#44961,.T.);
#62829=ORIENTED_EDGE('',*,*,#45101,.T.);
#62830=ORIENTED_EDGE('',*,*,#46067,.F.);
#62831=ORIENTED_EDGE('',*,*,#46068,.F.);
#62832=ORIENTED_EDGE('',*,*,#46069,.F.);
#62833=ORIENTED_EDGE('',*,*,#46070,.T.);
#62834=ORIENTED_EDGE('',*,*,#46071,.F.);
#62835=ORIENTED_EDGE('',*,*,#45099,.T.);
#62836=ORIENTED_EDGE('',*,*,#46072,.T.);
#62837=ORIENTED_EDGE('',*,*,#46068,.T.);
#62838=ORIENTED_EDGE('',*,*,#46073,.F.);
#62839=ORIENTED_EDGE('',*,*,#46074,.F.);
#62840=ORIENTED_EDGE('',*,*,#46075,.F.);
#62841=ORIENTED_EDGE('',*,*,#46076,.F.);
#62842=ORIENTED_EDGE('',*,*,#44952,.F.);
#62843=ORIENTED_EDGE('',*,*,#46077,.F.);
#62844=ORIENTED_EDGE('',*,*,#46078,.F.);
#62845=ORIENTED_EDGE('',*,*,#46079,.F.);
#62846=ORIENTED_EDGE('',*,*,#44953,.T.);
#62847=ORIENTED_EDGE('',*,*,#46076,.T.);
#62848=ORIENTED_EDGE('',*,*,#46080,.T.);
#62849=ORIENTED_EDGE('',*,*,#46081,.T.);
#62850=ORIENTED_EDGE('',*,*,#46082,.F.);
#62851=ORIENTED_EDGE('',*,*,#44954,.F.);
#62852=ORIENTED_EDGE('',*,*,#46081,.F.);
#62853=ORIENTED_EDGE('',*,*,#46083,.F.);
#62854=ORIENTED_EDGE('',*,*,#44955,.T.);
#62855=ORIENTED_EDGE('',*,*,#46082,.T.);
#62856=ORIENTED_EDGE('',*,*,#46084,.T.);
#62857=ORIENTED_EDGE('',*,*,#46037,.T.);
#62858=ORIENTED_EDGE('',*,*,#46085,.F.);
#62859=ORIENTED_EDGE('',*,*,#46086,.T.);
#62860=ORIENTED_EDGE('',*,*,#46057,.F.);
#62861=ORIENTED_EDGE('',*,*,#46087,.F.);
#62862=ORIENTED_EDGE('',*,*,#45299,.F.);
#62863=ORIENTED_EDGE('',*,*,#45302,.T.);
#62864=ORIENTED_EDGE('',*,*,#45304,.F.);
#62865=ORIENTED_EDGE('',*,*,#45306,.T.);
#62866=ORIENTED_EDGE('',*,*,#45308,.F.);
#62867=ORIENTED_EDGE('',*,*,#45310,.T.);
#62868=ORIENTED_EDGE('',*,*,#46033,.F.);
#62869=ORIENTED_EDGE('',*,*,#46031,.T.);
#62870=ORIENTED_EDGE('',*,*,#46035,.T.);
#62871=ORIENTED_EDGE('',*,*,#46062,.F.);
#62872=ORIENTED_EDGE('',*,*,#46088,.T.);
#62873=ORIENTED_EDGE('',*,*,#46046,.F.);
#62874=ORIENTED_EDGE('',*,*,#46050,.T.);
#62875=ORIENTED_EDGE('',*,*,#46053,.F.);
#62876=ORIENTED_EDGE('',*,*,#46089,.T.);
#62877=ORIENTED_EDGE('',*,*,#46090,.F.);
#62878=ORIENTED_EDGE('',*,*,#46089,.F.);
#62879=ORIENTED_EDGE('',*,*,#46052,.F.);
#62880=ORIENTED_EDGE('',*,*,#46091,.F.);
#62881=ORIENTED_EDGE('',*,*,#46085,.T.);
#62882=ORIENTED_EDGE('',*,*,#46090,.T.);
#62883=ORIENTED_EDGE('',*,*,#46092,.T.);
#62884=ORIENTED_EDGE('',*,*,#46093,.T.);
#62885=ORIENTED_EDGE('',*,*,#46060,.T.);
#62886=ORIENTED_EDGE('',*,*,#46094,.T.);
#62887=ORIENTED_EDGE('',*,*,#46095,.T.);
#62888=ORIENTED_EDGE('',*,*,#45649,.T.);
#62889=ORIENTED_EDGE('',*,*,#46096,.F.);
#62890=ORIENTED_EDGE('',*,*,#46097,.F.);
#62891=ORIENTED_EDGE('',*,*,#46070,.F.);
#62892=ORIENTED_EDGE('',*,*,#46098,.F.);
#62893=ORIENTED_EDGE('',*,*,#46099,.F.);
#62894=ORIENTED_EDGE('',*,*,#46098,.T.);
#62895=ORIENTED_EDGE('',*,*,#46069,.T.);
#62896=ORIENTED_EDGE('',*,*,#46072,.F.);
#62897=ORIENTED_EDGE('',*,*,#45098,.F.);
#62898=ORIENTED_EDGE('',*,*,#45990,.T.);
#62899=ORIENTED_EDGE('',*,*,#45987,.T.);
#62900=ORIENTED_EDGE('',*,*,#45874,.T.);
#62901=ORIENTED_EDGE('',*,*,#45872,.F.);
#62902=ORIENTED_EDGE('',*,*,#45886,.T.);
#62903=ORIENTED_EDGE('',*,*,#45881,.F.);
#62904=ORIENTED_EDGE('',*,*,#45057,.T.);
#62905=ORIENTED_EDGE('',*,*,#45852,.F.);
#62906=ORIENTED_EDGE('',*,*,#45863,.T.);
#62907=ORIENTED_EDGE('',*,*,#45848,.F.);
#62908=ORIENTED_EDGE('',*,*,#46022,.T.);
#62909=ORIENTED_EDGE('',*,*,#46036,.F.);
#62910=ORIENTED_EDGE('',*,*,#45139,.T.);
#62911=ORIENTED_EDGE('',*,*,#46011,.F.);
#62912=ORIENTED_EDGE('',*,*,#45993,.F.);
#62913=ORIENTED_EDGE('',*,*,#46000,.F.);
#62914=ORIENTED_EDGE('',*,*,#45996,.F.);
#62915=ORIENTED_EDGE('',*,*,#46016,.F.);
#62916=ORIENTED_EDGE('',*,*,#45103,.T.);
#62917=ORIENTED_EDGE('',*,*,#45921,.F.);
#62918=ORIENTED_EDGE('',*,*,#45923,.T.);
#62919=ORIENTED_EDGE('',*,*,#45924,.T.);
#62920=ORIENTED_EDGE('',*,*,#46040,.F.);
#62921=ORIENTED_EDGE('',*,*,#46043,.F.);
#62922=ORIENTED_EDGE('',*,*,#46100,.T.);
#62923=ORIENTED_EDGE('',*,*,#46101,.F.);
#62924=ORIENTED_EDGE('',*,*,#45909,.F.);
#62925=ORIENTED_EDGE('',*,*,#45958,.T.);
#62926=ORIENTED_EDGE('',*,*,#45914,.T.);
#62927=ORIENTED_EDGE('',*,*,#45918,.F.);
#62928=ORIENTED_EDGE('',*,*,#46102,.T.);
#62929=ORIENTED_EDGE('',*,*,#45901,.T.);
#62930=ORIENTED_EDGE('',*,*,#46099,.T.);
#62931=ORIENTED_EDGE('',*,*,#46103,.T.);
#62932=ORIENTED_EDGE('',*,*,#46104,.T.);
#62933=ORIENTED_EDGE('',*,*,#46096,.T.);
#62934=ORIENTED_EDGE('',*,*,#46105,.T.);
#62935=ORIENTED_EDGE('',*,*,#46106,.F.);
#62936=ORIENTED_EDGE('',*,*,#46103,.F.);
#62937=ORIENTED_EDGE('',*,*,#46102,.F.);
#62938=ORIENTED_EDGE('',*,*,#45917,.F.);
#62939=ORIENTED_EDGE('',*,*,#46107,.T.);
#62940=ORIENTED_EDGE('',*,*,#46108,.F.);
#62941=ORIENTED_EDGE('',*,*,#46109,.F.);
#62942=ORIENTED_EDGE('',*,*,#46110,.T.);
#62943=ORIENTED_EDGE('',*,*,#46108,.T.);
#62944=ORIENTED_EDGE('',*,*,#46111,.T.);
#62945=ORIENTED_EDGE('',*,*,#45003,.T.);
#62946=ORIENTED_EDGE('',*,*,#46112,.F.);
#62947=ORIENTED_EDGE('',*,*,#46113,.F.);
#62948=ORIENTED_EDGE('',*,*,#46114,.T.);
#62949=ORIENTED_EDGE('',*,*,#45949,.T.);
#62950=ORIENTED_EDGE('',*,*,#46114,.F.);
#62951=ORIENTED_EDGE('',*,*,#46065,.T.);
#62952=ORIENTED_EDGE('',*,*,#46066,.T.);
#62953=ORIENTED_EDGE('',*,*,#45100,.T.);
#62954=ORIENTED_EDGE('',*,*,#46071,.T.);
#62955=ORIENTED_EDGE('',*,*,#46067,.T.);
#62956=ORIENTED_EDGE('',*,*,#46097,.T.);
#62957=ORIENTED_EDGE('',*,*,#46104,.F.);
#62958=ORIENTED_EDGE('',*,*,#46106,.T.);
#62959=ORIENTED_EDGE('',*,*,#46115,.F.);
#62960=ORIENTED_EDGE('',*,*,#46116,.F.);
#62961=ORIENTED_EDGE('',*,*,#46109,.T.);
#62962=ORIENTED_EDGE('',*,*,#46110,.F.);
#62963=ORIENTED_EDGE('',*,*,#45002,.T.);
#62964=ORIENTED_EDGE('',*,*,#46063,.T.);
#62965=ORIENTED_EDGE('',*,*,#44967,.T.);
#62966=ORIENTED_EDGE('',*,*,#44965,.F.);
#62967=ORIENTED_EDGE('',*,*,#44963,.T.);
#62968=ORIENTED_EDGE('',*,*,#44942,.F.);
#62969=ORIENTED_EDGE('',*,*,#46105,.F.);
#62970=ORIENTED_EDGE('',*,*,#46116,.T.);
#62971=ORIENTED_EDGE('',*,*,#46117,.T.);
#62972=ORIENTED_EDGE('',*,*,#46112,.T.);
#62973=ORIENTED_EDGE('',*,*,#46113,.T.);
#62974=ORIENTED_EDGE('',*,*,#46117,.F.);
#62975=ORIENTED_EDGE('',*,*,#46115,.T.);
#62976=ORIENTED_EDGE('',*,*,#45537,.F.);
#62977=ORIENTED_EDGE('',*,*,#46118,.F.);
#62978=ORIENTED_EDGE('',*,*,#46119,.F.);
#62979=ORIENTED_EDGE('',*,*,#46120,.F.);
#62980=ORIENTED_EDGE('',*,*,#45190,.T.);
#62981=ORIENTED_EDGE('',*,*,#45192,.T.);
#62982=ORIENTED_EDGE('',*,*,#45194,.F.);
#62983=ORIENTED_EDGE('',*,*,#45196,.T.);
#62984=ORIENTED_EDGE('',*,*,#45198,.F.);
#62985=ORIENTED_EDGE('',*,*,#45200,.T.);
#62986=ORIENTED_EDGE('',*,*,#45202,.F.);
#62987=ORIENTED_EDGE('',*,*,#45213,.F.);
#62988=ORIENTED_EDGE('',*,*,#46121,.F.);
#62989=ORIENTED_EDGE('',*,*,#46122,.F.);
#62990=ORIENTED_EDGE('',*,*,#46123,.F.);
#62991=ORIENTED_EDGE('',*,*,#45515,.F.);
#62992=ORIENTED_EDGE('',*,*,#46124,.F.);
#62993=ORIENTED_EDGE('',*,*,#46125,.F.);
#62994=ORIENTED_EDGE('',*,*,#46126,.F.);
#62995=ORIENTED_EDGE('',*,*,#46127,.T.);
#62996=ORIENTED_EDGE('',*,*,#45940,.F.);
#62997=ORIENTED_EDGE('',*,*,#45456,.T.);
#62998=ORIENTED_EDGE('',*,*,#46128,.F.);
#62999=ORIENTED_EDGE('',*,*,#45559,.T.);
#63000=ORIENTED_EDGE('',*,*,#45562,.F.);
#63001=ORIENTED_EDGE('',*,*,#45564,.F.);
#63002=ORIENTED_EDGE('',*,*,#45566,.F.);
#63003=ORIENTED_EDGE('',*,*,#45579,.F.);
#63004=ORIENTED_EDGE('',*,*,#46129,.F.);
#63005=ORIENTED_EDGE('',*,*,#46130,.F.);
#63006=ORIENTED_EDGE('',*,*,#46131,.F.);
#63007=ORIENTED_EDGE('',*,*,#45354,.F.);
#63008=ORIENTED_EDGE('',*,*,#45363,.F.);
#63009=ORIENTED_EDGE('',*,*,#45365,.T.);
#63010=ORIENTED_EDGE('',*,*,#46132,.F.);
#63011=ORIENTED_EDGE('',*,*,#46133,.T.);
#63012=ORIENTED_EDGE('',*,*,#46134,.F.);
#63013=ORIENTED_EDGE('',*,*,#46135,.T.);
#63014=ORIENTED_EDGE('',*,*,#46136,.T.);
#63015=ORIENTED_EDGE('',*,*,#45345,.T.);
#63016=ORIENTED_EDGE('',*,*,#45348,.F.);
#63017=ORIENTED_EDGE('',*,*,#45352,.F.);
#63018=ORIENTED_EDGE('',*,*,#46137,.F.);
#63019=ORIENTED_EDGE('',*,*,#46138,.F.);
#63020=ORIENTED_EDGE('',*,*,#45927,.F.);
#63021=ORIENTED_EDGE('',*,*,#45936,.T.);
#63022=ORIENTED_EDGE('',*,*,#45939,.F.);
#63023=ORIENTED_EDGE('',*,*,#46139,.F.);
#63024=ORIENTED_EDGE('',*,*,#45634,.F.);
#63025=ORIENTED_EDGE('',*,*,#45643,.F.);
#63026=ORIENTED_EDGE('',*,*,#45760,.F.);
#63027=ORIENTED_EDGE('',*,*,#45204,.F.);
#63028=ORIENTED_EDGE('',*,*,#45184,.T.);
#63029=ORIENTED_EDGE('',*,*,#45188,.T.);
#63030=ORIENTED_EDGE('',*,*,#45534,.F.);
#63031=ORIENTED_EDGE('',*,*,#46120,.T.);
#63032=ORIENTED_EDGE('',*,*,#46140,.T.);
#63033=ORIENTED_EDGE('',*,*,#45567,.T.);
#63034=ORIENTED_EDGE('',*,*,#46141,.F.);
#63035=ORIENTED_EDGE('',*,*,#45357,.F.);
#63036=ORIENTED_EDGE('',*,*,#46142,.F.);
#63037=ORIENTED_EDGE('',*,*,#45575,.T.);
#63038=ORIENTED_EDGE('',*,*,#46143,.T.);
#63039=ORIENTED_EDGE('',*,*,#45967,.F.);
#63040=ORIENTED_EDGE('',*,*,#45965,.F.);
#63041=ORIENTED_EDGE('',*,*,#46143,.F.);
#63042=ORIENTED_EDGE('',*,*,#45574,.T.);
#63043=ORIENTED_EDGE('',*,*,#46144,.F.);
#63044=ORIENTED_EDGE('',*,*,#45517,.F.);
#63045=ORIENTED_EDGE('',*,*,#46145,.F.);
#63046=ORIENTED_EDGE('',*,*,#46146,.F.);
#63047=ORIENTED_EDGE('',*,*,#46147,.F.);
#63048=ORIENTED_EDGE('',*,*,#46148,.F.);
#63049=ORIENTED_EDGE('',*,*,#46149,.F.);
#63050=ORIENTED_EDGE('',*,*,#46150,.F.);
#63051=ORIENTED_EDGE('',*,*,#46151,.T.);
#63052=ORIENTED_EDGE('',*,*,#46152,.F.);
#63053=ORIENTED_EDGE('',*,*,#46153,.F.);
#63054=ORIENTED_EDGE('',*,*,#46154,.F.);
#63055=ORIENTED_EDGE('',*,*,#46155,.F.);
#63056=ORIENTED_EDGE('',*,*,#46156,.F.);
#63057=ORIENTED_EDGE('',*,*,#45208,.F.);
#63058=ORIENTED_EDGE('',*,*,#46157,.F.);
#63059=ORIENTED_EDGE('',*,*,#46153,.T.);
#63060=ORIENTED_EDGE('',*,*,#46158,.F.);
#63061=ORIENTED_EDGE('',*,*,#45523,.F.);
#63062=ORIENTED_EDGE('',*,*,#46159,.F.);
#63063=ORIENTED_EDGE('',*,*,#46146,.T.);
#63064=ORIENTED_EDGE('',*,*,#46160,.F.);
#63065=ORIENTED_EDGE('',*,*,#46122,.T.);
#63066=ORIENTED_EDGE('',*,*,#46145,.T.);
#63067=ORIENTED_EDGE('',*,*,#45516,.T.);
#63068=ORIENTED_EDGE('',*,*,#46123,.T.);
#63069=ORIENTED_EDGE('',*,*,#46160,.T.);
#63070=ORIENTED_EDGE('',*,*,#46161,.F.);
#63071=ORIENTED_EDGE('',*,*,#46147,.T.);
#63072=ORIENTED_EDGE('',*,*,#46159,.T.);
#63073=ORIENTED_EDGE('',*,*,#46121,.T.);
#63074=ORIENTED_EDGE('',*,*,#45212,.T.);
#63075=ORIENTED_EDGE('',*,*,#46162,.T.);
#63076=ORIENTED_EDGE('',*,*,#46154,.T.);
#63077=ORIENTED_EDGE('',*,*,#46157,.T.);
#63078=ORIENTED_EDGE('',*,*,#45207,.T.);
#63079=ORIENTED_EDGE('',*,*,#46163,.T.);
#63080=ORIENTED_EDGE('',*,*,#45524,.T.);
#63081=ORIENTED_EDGE('',*,*,#46158,.T.);
#63082=ORIENTED_EDGE('',*,*,#46152,.T.);
#63083=ORIENTED_EDGE('',*,*,#46164,.T.);
#63084=ORIENTED_EDGE('',*,*,#45360,.T.);
#63085=ORIENTED_EDGE('',*,*,#46165,.T.);
#63086=ORIENTED_EDGE('',*,*,#46150,.T.);
#63087=ORIENTED_EDGE('',*,*,#46166,.T.);
#63088=ORIENTED_EDGE('',*,*,#46148,.T.);
#63089=ORIENTED_EDGE('',*,*,#46167,.T.);
#63090=ORIENTED_EDGE('',*,*,#45571,.T.);
#63091=ORIENTED_EDGE('',*,*,#46168,.F.);
#63092=ORIENTED_EDGE('',*,*,#46169,.F.);
#63093=ORIENTED_EDGE('',*,*,#46170,.F.);
#63094=ORIENTED_EDGE('',*,*,#46130,.T.);
#63095=ORIENTED_EDGE('',*,*,#46171,.T.);
#63096=ORIENTED_EDGE('',*,*,#46168,.T.);
#63097=ORIENTED_EDGE('',*,*,#46129,.T.);
#63098=ORIENTED_EDGE('',*,*,#45578,.T.);
#63099=ORIENTED_EDGE('',*,*,#46172,.F.);
#63100=ORIENTED_EDGE('',*,*,#45355,.T.);
#63101=ORIENTED_EDGE('',*,*,#46131,.T.);
#63102=ORIENTED_EDGE('',*,*,#46170,.T.);
#63103=ORIENTED_EDGE('',*,*,#46173,.T.);
#63104=ORIENTED_EDGE('',*,*,#46174,.F.);
#63105=ORIENTED_EDGE('',*,*,#46173,.F.);
#63106=ORIENTED_EDGE('',*,*,#46169,.T.);
#63107=ORIENTED_EDGE('',*,*,#46171,.F.);
#63108=ORIENTED_EDGE('',*,*,#45577,.F.);
#63109=ORIENTED_EDGE('',*,*,#45576,.T.);
#63110=ORIENTED_EDGE('',*,*,#46142,.T.);
#63111=ORIENTED_EDGE('',*,*,#45356,.T.);
#63112=ORIENTED_EDGE('',*,*,#46172,.T.);
#63113=ORIENTED_EDGE('',*,*,#46174,.T.);
#63114=ORIENTED_EDGE('',*,*,#45211,.T.);
#63115=ORIENTED_EDGE('',*,*,#46175,.T.);
#63116=ORIENTED_EDGE('',*,*,#45518,.T.);
#63117=ORIENTED_EDGE('',*,*,#46144,.T.);
#63118=ORIENTED_EDGE('',*,*,#46161,.T.);
#63119=ORIENTED_EDGE('',*,*,#45521,.T.);
#63120=ORIENTED_EDGE('',*,*,#46176,.T.);
#63121=ORIENTED_EDGE('',*,*,#46177,.F.);
#63122=ORIENTED_EDGE('',*,*,#45522,.F.);
#63123=ORIENTED_EDGE('',*,*,#46177,.T.);
#63124=ORIENTED_EDGE('',*,*,#46178,.T.);
#63125=ORIENTED_EDGE('',*,*,#45209,.T.);
#63126=ORIENTED_EDGE('',*,*,#46156,.T.);
#63127=ORIENTED_EDGE('',*,*,#46179,.F.);
#63128=ORIENTED_EDGE('',*,*,#45572,.F.);
#63129=ORIENTED_EDGE('',*,*,#46167,.F.);
#63130=ORIENTED_EDGE('',*,*,#46151,.F.);
#63131=ORIENTED_EDGE('',*,*,#46165,.F.);
#63132=ORIENTED_EDGE('',*,*,#45359,.F.);
#63133=ORIENTED_EDGE('',*,*,#45358,.T.);
#63134=ORIENTED_EDGE('',*,*,#46141,.T.);
#63135=ORIENTED_EDGE('',*,*,#45573,.T.);
#63136=ORIENTED_EDGE('',*,*,#46179,.T.);
#63137=ORIENTED_EDGE('',*,*,#46180,.T.);
#63138=ORIENTED_EDGE('',*,*,#46181,.T.);
#63139=ORIENTED_EDGE('',*,*,#46137,.T.);
#63140=ORIENTED_EDGE('',*,*,#45351,.T.);
#63141=ORIENTED_EDGE('',*,*,#45316,.F.);
#63142=ORIENTED_EDGE('',*,*,#46182,.T.);
#63143=ORIENTED_EDGE('',*,*,#46132,.T.);
#63144=ORIENTED_EDGE('',*,*,#45364,.T.);
#63145=ORIENTED_EDGE('',*,*,#45322,.F.);
#63146=ORIENTED_EDGE('',*,*,#46183,.T.);
#63147=ORIENTED_EDGE('',*,*,#46134,.T.);
#63148=ORIENTED_EDGE('',*,*,#46184,.T.);
#63149=ORIENTED_EDGE('',*,*,#45319,.F.);
#63150=ORIENTED_EDGE('',*,*,#46184,.F.);
#63151=ORIENTED_EDGE('',*,*,#46133,.F.);
#63152=ORIENTED_EDGE('',*,*,#46182,.F.);
#63153=ORIENTED_EDGE('',*,*,#45540,.F.);
#63154=ORIENTED_EDGE('',*,*,#45453,.T.);
#63155=ORIENTED_EDGE('',*,*,#46185,.T.);
#63156=ORIENTED_EDGE('',*,*,#46118,.T.);
#63157=ORIENTED_EDGE('',*,*,#44949,.T.);
#63158=ORIENTED_EDGE('',*,*,#46186,.T.);
#63159=ORIENTED_EDGE('',*,*,#46187,.T.);
#63160=ORIENTED_EDGE('',*,*,#46188,.T.);
#63161=ORIENTED_EDGE('',*,*,#46189,.F.);
#63162=ORIENTED_EDGE('',*,*,#44950,.F.);
#63163=ORIENTED_EDGE('',*,*,#46188,.F.);
#63164=ORIENTED_EDGE('',*,*,#46190,.F.);
#63165=ORIENTED_EDGE('',*,*,#44951,.T.);
#63166=ORIENTED_EDGE('',*,*,#46189,.T.);
#63167=ORIENTED_EDGE('',*,*,#46191,.T.);
#63168=ORIENTED_EDGE('',*,*,#46077,.T.);
#63169=ORIENTED_EDGE('',*,*,#46192,.F.);
#63170=ORIENTED_EDGE('',*,*,#46078,.T.);
#63171=ORIENTED_EDGE('',*,*,#46191,.F.);
#63172=ORIENTED_EDGE('',*,*,#46190,.T.);
#63173=ORIENTED_EDGE('',*,*,#46187,.F.);
#63174=ORIENTED_EDGE('',*,*,#46193,.F.);
#63175=ORIENTED_EDGE('',*,*,#44995,.T.);
#63176=ORIENTED_EDGE('',*,*,#44998,.T.);
#63177=ORIENTED_EDGE('',*,*,#45000,.F.);
#63178=ORIENTED_EDGE('',*,*,#45004,.F.);
#63179=ORIENTED_EDGE('',*,*,#46111,.F.);
#63180=ORIENTED_EDGE('',*,*,#46107,.F.);
#63181=ORIENTED_EDGE('',*,*,#45919,.F.);
#63182=ORIENTED_EDGE('',*,*,#45916,.T.);
#63183=ORIENTED_EDGE('',*,*,#45959,.F.);
#63184=ORIENTED_EDGE('',*,*,#45911,.F.);
#63185=ORIENTED_EDGE('',*,*,#46194,.F.);
#63186=ORIENTED_EDGE('',*,*,#46180,.F.);
#63187=ORIENTED_EDGE('',*,*,#45350,.T.);
#63188=ORIENTED_EDGE('',*,*,#45361,.T.);
#63189=ORIENTED_EDGE('',*,*,#46164,.F.);
#63190=ORIENTED_EDGE('',*,*,#46149,.T.);
#63191=ORIENTED_EDGE('',*,*,#46166,.F.);
#63192=ORIENTED_EDGE('',*,*,#45570,.F.);
#63193=ORIENTED_EDGE('',*,*,#46192,.T.);
#63194=ORIENTED_EDGE('',*,*,#45569,.T.);
#63195=ORIENTED_EDGE('',*,*,#46195,.T.);
#63196=ORIENTED_EDGE('',*,*,#46079,.T.);
#63197=ORIENTED_EDGE('',*,*,#45545,.F.);
#63198=ORIENTED_EDGE('',*,*,#45560,.T.);
#63199=ORIENTED_EDGE('',*,*,#46128,.T.);
#63200=ORIENTED_EDGE('',*,*,#45455,.T.);
#63201=ORIENTED_EDGE('',*,*,#45483,.F.);
#63202=ORIENTED_EDGE('',*,*,#45941,.F.);
#63203=ORIENTED_EDGE('',*,*,#46127,.F.);
#63204=ORIENTED_EDGE('',*,*,#46196,.F.);
#63205=ORIENTED_EDGE('',*,*,#45480,.F.);
#63206=ORIENTED_EDGE('',*,*,#46196,.T.);
#63207=ORIENTED_EDGE('',*,*,#46126,.T.);
#63208=ORIENTED_EDGE('',*,*,#46197,.T.);
#63209=ORIENTED_EDGE('',*,*,#45477,.F.);
#63210=ORIENTED_EDGE('',*,*,#46197,.F.);
#63211=ORIENTED_EDGE('',*,*,#46125,.T.);
#63212=ORIENTED_EDGE('',*,*,#46198,.F.);
#63213=ORIENTED_EDGE('',*,*,#45474,.F.);
#63214=ORIENTED_EDGE('',*,*,#46198,.T.);
#63215=ORIENTED_EDGE('',*,*,#46124,.T.);
#63216=ORIENTED_EDGE('',*,*,#45514,.T.);
#63217=ORIENTED_EDGE('',*,*,#45241,.F.);
#63218=ORIENTED_EDGE('',*,*,#45635,.T.);
#63219=ORIENTED_EDGE('',*,*,#46139,.T.);
#63220=ORIENTED_EDGE('',*,*,#45938,.F.);
#63221=ORIENTED_EDGE('',*,*,#45946,.T.);
#63222=ORIENTED_EDGE('',*,*,#46058,.T.);
#63223=ORIENTED_EDGE('',*,*,#45651,.F.);
#63224=ORIENTED_EDGE('',*,*,#45328,.F.);
#63225=ORIENTED_EDGE('',*,*,#45346,.F.);
#63226=ORIENTED_EDGE('',*,*,#46136,.F.);
#63227=ORIENTED_EDGE('',*,*,#46199,.T.);
#63228=ORIENTED_EDGE('',*,*,#45325,.F.);
#63229=ORIENTED_EDGE('',*,*,#46199,.F.);
#63230=ORIENTED_EDGE('',*,*,#46135,.F.);
#63231=ORIENTED_EDGE('',*,*,#46183,.F.);
#63232=ORIENTED_EDGE('',*,*,#45282,.F.);
#63233=ORIENTED_EDGE('',*,*,#45300,.F.);
#63234=ORIENTED_EDGE('',*,*,#46087,.T.);
#63235=ORIENTED_EDGE('',*,*,#46056,.T.);
#63236=ORIENTED_EDGE('',*,*,#45928,.F.);
#63237=ORIENTED_EDGE('',*,*,#46138,.T.);
#63238=ORIENTED_EDGE('',*,*,#46181,.F.);
#63239=ORIENTED_EDGE('',*,*,#46194,.T.);
#63240=ORIENTED_EDGE('',*,*,#45910,.F.);
#63241=ORIENTED_EDGE('',*,*,#46101,.T.);
#63242=ORIENTED_EDGE('',*,*,#46200,.T.);
#63243=ORIENTED_EDGE('',*,*,#45279,.F.);
#63244=ORIENTED_EDGE('',*,*,#46200,.F.);
#63245=ORIENTED_EDGE('',*,*,#46100,.F.);
#63246=ORIENTED_EDGE('',*,*,#46042,.F.);
#63247=ORIENTED_EDGE('',*,*,#46201,.F.);
#63248=ORIENTED_EDGE('',*,*,#46047,.F.);
#63249=ORIENTED_EDGE('',*,*,#46088,.F.);
#63250=ORIENTED_EDGE('',*,*,#46061,.F.);
#63251=ORIENTED_EDGE('',*,*,#45904,.F.);
#63252=ORIENTED_EDGE('',*,*,#44984,.F.);
#63253=ORIENTED_EDGE('',*,*,#44996,.F.);
#63254=ORIENTED_EDGE('',*,*,#46193,.T.);
#63255=ORIENTED_EDGE('',*,*,#46186,.F.);
#63256=ORIENTED_EDGE('',*,*,#44948,.F.);
#63257=ORIENTED_EDGE('',*,*,#46202,.F.);
#63258=ORIENTED_EDGE('',*,*,#44981,.F.);
#63259=ORIENTED_EDGE('',*,*,#46202,.T.);
#63260=ORIENTED_EDGE('',*,*,#44947,.T.);
#63261=ORIENTED_EDGE('',*,*,#44970,.T.);
#63262=ORIENTED_EDGE('',*,*,#45081,.F.);
#63263=ORIENTED_EDGE('',*,*,#45978,.T.);
#63264=ORIENTED_EDGE('',*,*,#45876,.F.);
#63265=ORIENTED_EDGE('',*,*,#45986,.F.);
#63266=ORIENTED_EDGE('',*,*,#45989,.T.);
#63267=ORIENTED_EDGE('',*,*,#46026,.T.);
#63268=ORIENTED_EDGE('',*,*,#46028,.F.);
#63269=ORIENTED_EDGE('',*,*,#46029,.F.);
#63270=ORIENTED_EDGE('',*,*,#45979,.T.);
#63271=ORIENTED_EDGE('',*,*,#45079,.T.);
#63272=ORIENTED_EDGE('',*,*,#45115,.T.);
#63273=ORIENTED_EDGE('',*,*,#45980,.T.);
#63274=ORIENTED_EDGE('',*,*,#45878,.F.);
#63275=ORIENTED_EDGE('',*,*,#45977,.T.);
#63276=ORIENTED_EDGE('',*,*,#46018,.F.);
#63277=ORIENTED_EDGE('',*,*,#45971,.F.);
#63278=ORIENTED_EDGE('',*,*,#45069,.F.);
#63279=ORIENTED_EDGE('',*,*,#45039,.F.);
#63280=ORIENTED_EDGE('',*,*,#45113,.F.);
#63281=ORIENTED_EDGE('',*,*,#45108,.F.);
#63282=ORIENTED_EDGE('',*,*,#45050,.F.);
#63283=ORIENTED_EDGE('',*,*,#45045,.F.);
#63284=ORIENTED_EDGE('',*,*,#45042,.T.);
#63285=ORIENTED_EDGE('',*,*,#45063,.F.);
#63286=ORIENTED_EDGE('',*,*,#45983,.F.);
#63287=ORIENTED_EDGE('',*,*,#45116,.F.);
#63288=ORIENTED_EDGE('',*,*,#45111,.F.);
#63289=ORIENTED_EDGE('',*,*,#46054,.F.);
#63290=ORIENTED_EDGE('',*,*,#46086,.F.);
#63291=ORIENTED_EDGE('',*,*,#46093,.F.);
#63292=ORIENTED_EDGE('',*,*,#46203,.F.);
#63293=ORIENTED_EDGE('',*,*,#46204,.F.);
#63294=ORIENTED_EDGE('',*,*,#46205,.F.);
#63295=ORIENTED_EDGE('',*,*,#46204,.T.);
#63296=ORIENTED_EDGE('',*,*,#46206,.T.);
#63297=ORIENTED_EDGE('',*,*,#46207,.T.);
#63298=ORIENTED_EDGE('',*,*,#46208,.F.);
#63299=ORIENTED_EDGE('',*,*,#46207,.F.);
#63300=ORIENTED_EDGE('',*,*,#46209,.F.);
#63301=ORIENTED_EDGE('',*,*,#46094,.F.);
#63302=ORIENTED_EDGE('',*,*,#46059,.F.);
#63303=ORIENTED_EDGE('',*,*,#45955,.F.);
#63304=ORIENTED_EDGE('',*,*,#46210,.F.);
#63305=ORIENTED_EDGE('',*,*,#45022,.F.);
#63306=ORIENTED_EDGE('',*,*,#45931,.F.);
#63307=ORIENTED_EDGE('',*,*,#45943,.F.);
#63308=ORIENTED_EDGE('',*,*,#45036,.T.);
#63309=ORIENTED_EDGE('',*,*,#46205,.T.);
#63310=ORIENTED_EDGE('',*,*,#46208,.T.);
#63311=ORIENTED_EDGE('',*,*,#46210,.T.);
#63312=ORIENTED_EDGE('',*,*,#45957,.F.);
#63313=ORIENTED_EDGE('',*,*,#45035,.T.);
#63314=ORIENTED_EDGE('',*,*,#46055,.F.);
#63315=ORIENTED_EDGE('',*,*,#45784,.T.);
#63316=ORIENTED_EDGE('',*,*,#46211,.T.);
#63317=ORIENTED_EDGE('',*,*,#45519,.T.);
#63318=ORIENTED_EDGE('',*,*,#46175,.F.);
#63319=ORIENTED_EDGE('',*,*,#45210,.F.);
#63320=ORIENTED_EDGE('',*,*,#46178,.F.);
#63321=ORIENTED_EDGE('',*,*,#46176,.F.);
#63322=ORIENTED_EDGE('',*,*,#45520,.T.);
#63323=ORIENTED_EDGE('',*,*,#46211,.F.);
#63324=ORIENTED_EDGE('',*,*,#46095,.F.);
#63325=ORIENTED_EDGE('',*,*,#46209,.T.);
#63326=ORIENTED_EDGE('',*,*,#46206,.F.);
#63327=ORIENTED_EDGE('',*,*,#46203,.T.);
#63328=ORIENTED_EDGE('',*,*,#46092,.F.);
#63329=ORIENTED_EDGE('',*,*,#46091,.T.);
#63330=ORIENTED_EDGE('',*,*,#46051,.T.);
#63331=ORIENTED_EDGE('',*,*,#46048,.T.);
#63332=ORIENTED_EDGE('',*,*,#46044,.T.);
#63333=ORIENTED_EDGE('',*,*,#46201,.T.);
#63334=ORIENTED_EDGE('',*,*,#46041,.T.);
#63335=ORIENTED_EDGE('',*,*,#46038,.T.);
#63336=ORIENTED_EDGE('',*,*,#46084,.F.);
#63337=ORIENTED_EDGE('',*,*,#46083,.T.);
#63338=ORIENTED_EDGE('',*,*,#46080,.F.);
#63339=ORIENTED_EDGE('',*,*,#46075,.T.);
#63340=ORIENTED_EDGE('',*,*,#46212,.F.);
#63341=ORIENTED_EDGE('',*,*,#45595,.T.);
#63342=ORIENTED_EDGE('',*,*,#45608,.F.);
#63343=ORIENTED_EDGE('',*,*,#45617,.T.);
#63344=ORIENTED_EDGE('',*,*,#45618,.T.);
#63345=ORIENTED_EDGE('',*,*,#45844,.T.);
#63346=ORIENTED_EDGE('',*,*,#45745,.T.);
#63347=ORIENTED_EDGE('',*,*,#45755,.T.);
#63348=ORIENTED_EDGE('',*,*,#45703,.T.);
#63349=ORIENTED_EDGE('',*,*,#45717,.T.);
#63350=ORIENTED_EDGE('',*,*,#45731,.T.);
#63351=ORIENTED_EDGE('',*,*,#45710,.T.);
#63352=ORIENTED_EDGE('',*,*,#45699,.T.);
#63353=ORIENTED_EDGE('',*,*,#45754,.T.);
#63354=ORIENTED_EDGE('',*,*,#45753,.T.);
#63355=ORIENTED_EDGE('',*,*,#45843,.F.);
#63356=ORIENTED_EDGE('',*,*,#45733,.T.);
#63357=ORIENTED_EDGE('',*,*,#45743,.T.);
#63358=ORIENTED_EDGE('',*,*,#45709,.T.);
#63359=ORIENTED_EDGE('',*,*,#45725,.T.);
#63360=ORIENTED_EDGE('',*,*,#45728,.T.);
#63361=ORIENTED_EDGE('',*,*,#45718,.T.);
#63362=ORIENTED_EDGE('',*,*,#45705,.T.);
#63363=ORIENTED_EDGE('',*,*,#45742,.T.);
#63364=ORIENTED_EDGE('',*,*,#45741,.T.);
#63365=ORIENTED_EDGE('',*,*,#45842,.F.);
#63366=ORIENTED_EDGE('',*,*,#45656,.T.);
#63367=ORIENTED_EDGE('',*,*,#45653,.T.);
#63368=ORIENTED_EDGE('',*,*,#45644,.F.);
#63369=ORIENTED_EDGE('',*,*,#45650,.T.);
#63370=ORIENTED_EDGE('',*,*,#45895,.T.);
#63371=ORIENTED_EDGE('',*,*,#45667,.T.);
#63372=ORIENTED_EDGE('',*,*,#45625,.T.);
#63373=ORIENTED_EDGE('',*,*,#46212,.T.);
#63374=ORIENTED_EDGE('',*,*,#46074,.T.);
#63375=ORIENTED_EDGE('',*,*,#46213,.T.);
#63376=ORIENTED_EDGE('',*,*,#45596,.T.);
#63377=ORIENTED_EDGE('',*,*,#46213,.F.);
#63378=ORIENTED_EDGE('',*,*,#46073,.T.);
#63379=ORIENTED_EDGE('',*,*,#46195,.F.);
#63380=ORIENTED_EDGE('',*,*,#45568,.T.);
#63381=ORIENTED_EDGE('',*,*,#46140,.F.);
#63382=ORIENTED_EDGE('',*,*,#46119,.T.);
#63383=ORIENTED_EDGE('',*,*,#46185,.F.);
#63384=ORIENTED_EDGE('',*,*,#45452,.T.);
#63385=ORIENTED_EDGE('',*,*,#45462,.F.);
#63386=ORIENTED_EDGE('',*,*,#45464,.T.);
#63387=ORIENTED_EDGE('',*,*,#45466,.F.);
#63388=ORIENTED_EDGE('',*,*,#45468,.T.);
#63389=ORIENTED_EDGE('',*,*,#45581,.F.);
#63390=ORIENTED_EDGE('',*,*,#45583,.T.);
#63391=ORIENTED_EDGE('',*,*,#45584,.F.);
#63392=ORIENTED_EDGE('',*,*,#45527,.F.);
#63393=ORIENTED_EDGE('',*,*,#45603,.F.);
#63394=ORIENTED_EDGE('',*,*,#45597,.T.);
#63395=ORIENTED_EDGE('',*,*,#45429,.F.);
#63396=ORIENTED_EDGE('',*,*,#45448,.F.);
#63397=ORIENTED_EDGE('',*,*,#46214,.F.);
#63398=ORIENTED_EDGE('',*,*,#45604,.F.);
#63399=ORIENTED_EDGE('',*,*,#46214,.T.);
#63400=ORIENTED_EDGE('',*,*,#45447,.F.);
#63401=ORIENTED_EDGE('',*,*,#45460,.T.);
#63402=ORIENTED_EDGE('',*,*,#45947,.F.);
#63403=ORIENTED_EDGE('',*,*,#45507,.T.);
#63404=ORIENTED_EDGE('',*,*,#45510,.F.);
#63405=ORIENTED_EDGE('',*,*,#45513,.T.);
#63406=ORIENTED_EDGE('',*,*,#45605,.F.);
#63407=ORIENTED_EDGE('',*,*,#45525,.F.);
#63408=ORIENTED_EDGE('',*,*,#46163,.F.);
#63409=ORIENTED_EDGE('',*,*,#46155,.T.);
#63410=ORIENTED_EDGE('',*,*,#46162,.F.);
#63411=ORIENTED_EDGE('',*,*,#45206,.T.);
#63412=ORIENTED_EDGE('',*,*,#45759,.T.);
#63413=ORIENTED_EDGE('',*,*,#45641,.F.);
#63414=ORIENTED_EDGE('',*,*,#45632,.T.);
#63415=ORIENTED_EDGE('',*,*,#45670,.F.);
#63416=ORIENTED_EDGE('',*,*,#45758,.F.);
#63417=ORIENTED_EDGE('',*,*,#45836,.T.);
#63418=ORIENTED_EDGE('',*,*,#45674,.F.);
#63419=ORIENTED_EDGE('',*,*,#45827,.F.);
#63420=ORIENTED_EDGE('',*,*,#45612,.F.);
#63421=ORIENTED_EDGE('',*,*,#45609,.T.);
#63422=ORIENTED_EDGE('',*,*,#45599,.T.);
#63423=ORIENTED_EDGE('',*,*,#45588,.F.);
#63424=ORIENTED_EDGE('',*,*,#45592,.T.);
#63425=ORIENTED_EDGE('',*,*,#45602,.F.);
#87130=CYLINDRICAL_SURFACE('',#95342,0.4);
#87131=CYLINDRICAL_SURFACE('',#95369,0.4);
#87132=CYLINDRICAL_SURFACE('',#95373,12.);
#87133=CYLINDRICAL_SURFACE('',#95377,0.8);
#87134=CYLINDRICAL_SURFACE('',#95380,0.8);
#87135=CYLINDRICAL_SURFACE('',#95384,0.4);
#87136=CYLINDRICAL_SURFACE('',#95397,0.4);
#87137=CYLINDRICAL_SURFACE('',#95402,0.4);
#87138=CYLINDRICAL_SURFACE('',#95408,0.4);
#87139=CYLINDRICAL_SURFACE('',#95428,0.8);
#87140=CYLINDRICAL_SURFACE('',#95430,13.2);
#87141=CYLINDRICAL_SURFACE('',#95432,0.6);
#87142=CYLINDRICAL_SURFACE('',#95434,3.15);
#87143=CYLINDRICAL_SURFACE('',#95441,0.8);
#87144=CYLINDRICAL_SURFACE('',#95453,0.4);
#87145=CYLINDRICAL_SURFACE('',#95458,0.4);
#87146=CYLINDRICAL_SURFACE('',#95470,0.4);
#87147=CYLINDRICAL_SURFACE('',#95480,0.6);
#87148=CYLINDRICAL_SURFACE('',#95484,0.6);
#87149=CYLINDRICAL_SURFACE('',#95486,0.6);
#87150=CYLINDRICAL_SURFACE('',#95488,9.70000001490116);
#87151=CYLINDRICAL_SURFACE('',#95491,0.4);
#87152=CYLINDRICAL_SURFACE('',#95512,0.4);
#87153=CYLINDRICAL_SURFACE('',#95521,0.4);
#87154=CYLINDRICAL_SURFACE('',#95526,5.40000000000001);
#87155=CYLINDRICAL_SURFACE('',#95528,0.6);
#87156=CYLINDRICAL_SURFACE('',#95531,0.6);
#87157=CYLINDRICAL_SURFACE('',#95554,0.4);
#87158=CYLINDRICAL_SURFACE('',#95560,0.4);
#87159=CYLINDRICAL_SURFACE('',#95565,0.4);
#87160=CYLINDRICAL_SURFACE('',#95577,0.4);
#87161=CYLINDRICAL_SURFACE('',#95578,0.8);
#87162=CYLINDRICAL_SURFACE('',#95581,0.6);
#87163=CYLINDRICAL_SURFACE('',#95583,3.1);
#87164=CYLINDRICAL_SURFACE('',#95585,0.800000000000001);
#87165=CYLINDRICAL_SURFACE('',#95588,4.8);
#87166=CYLINDRICAL_SURFACE('',#95617,0.4);
#87167=CYLINDRICAL_SURFACE('',#95621,17.3949617393671);
#87168=CYLINDRICAL_SURFACE('',#95623,0.8);
#87169=CYLINDRICAL_SURFACE('',#95626,0.8);
#87170=CYLINDRICAL_SURFACE('',#95628,9.3949617393671);
#87171=CYLINDRICAL_SURFACE('',#95654,0.4);
#87172=CYLINDRICAL_SURFACE('',#95659,0.4);
#87173=CYLINDRICAL_SURFACE('',#95664,0.4);
#87174=CYLINDRICAL_SURFACE('',#95682,0.8);
#87175=CYLINDRICAL_SURFACE('',#95685,0.8);
#87176=CYLINDRICAL_SURFACE('',#95687,18.9949617393671);
#87177=CYLINDRICAL_SURFACE('',#95689,0.6);
#87178=CYLINDRICAL_SURFACE('',#95691,9.7);
#87179=CYLINDRICAL_SURFACE('',#95693,0.6);
#87180=CYLINDRICAL_SURFACE('',#95695,3.6);
#87181=CYLINDRICAL_SURFACE('',#95711,0.4);
#87182=CYLINDRICAL_SURFACE('',#95729,12.);
#87183=CYLINDRICAL_SURFACE('',#95733,0.8);
#87184=CYLINDRICAL_SURFACE('',#95735,10.0999999997296);
#87185=CYLINDRICAL_SURFACE('',#95737,0.8);
#87186=CYLINDRICAL_SURFACE('',#95739,4.65);
#87187=CYLINDRICAL_SURFACE('',#95742,0.4);
#87188=CYLINDRICAL_SURFACE('',#95748,0.4);
#87189=CYLINDRICAL_SURFACE('',#95766,0.6);
#87190=CYLINDRICAL_SURFACE('',#95768,13.2);
#87191=CYLINDRICAL_SURFACE('',#95770,0.6);
#87192=CYLINDRICAL_SURFACE('',#95776,0.4);
#87193=CYLINDRICAL_SURFACE('',#95778,8.5);
#87194=CYLINDRICAL_SURFACE('',#95788,0.4);
#87195=CYLINDRICAL_SURFACE('',#95796,0.8);
#87196=CYLINDRICAL_SURFACE('',#95815,4.2);
#87197=CYLINDRICAL_SURFACE('',#95837,0.8);
#87198=CYLINDRICAL_SURFACE('',#95859,0.8);
#87199=CYLINDRICAL_SURFACE('',#95861,0.8);
#87200=CYLINDRICAL_SURFACE('',#95863,0.8);
#87201=CYLINDRICAL_SURFACE('',#95875,0.8);
#87202=CYLINDRICAL_SURFACE('',#95878,0.8);
#87203=CYLINDRICAL_SURFACE('',#95892,0.8);
#87204=CYLINDRICAL_SURFACE('',#95893,0.8);
#87205=CYLINDRICAL_SURFACE('',#95896,5.4);
#87206=CYLINDRICAL_SURFACE('',#95897,7.99496173936711);
#87207=CYLINDRICAL_SURFACE('',#95898,0.8);
#87208=CYLINDRICAL_SURFACE('',#95900,0.8);
#87209=CYLINDRICAL_SURFACE('',#95902,0.6);
#87210=CYLINDRICAL_SURFACE('',#95904,9.7);
#87211=CYLINDRICAL_SURFACE('',#95906,0.6);
#87212=CYLINDRICAL_SURFACE('',#95908,23.7449617393671);
#87213=CYLINDRICAL_SURFACE('',#95910,0.4);
#87214=CYLINDRICAL_SURFACE('',#95912,7.8);
#87215=CYLINDRICAL_SURFACE('',#95914,0.8);
#87216=CYLINDRICAL_SURFACE('',#95916,0.6);
#87217=CYLINDRICAL_SURFACE('',#95921,3.2);
#87218=CYLINDRICAL_SURFACE('',#95922,0.8);
#87219=CYLINDRICAL_SURFACE('',#95924,0.8);
#87220=CYLINDRICAL_SURFACE('',#95926,0.8);
#87221=CYLINDRICAL_SURFACE('',#95927,0.8);
#87222=CYLINDRICAL_SURFACE('',#95928,10.0999999997296);
#87223=CYLINDRICAL_SURFACE('',#95929,0.8);
#87224=CYLINDRICAL_SURFACE('',#95930,0.8);
#87225=CYLINDRICAL_SURFACE('',#95931,4.65);
#87226=CYLINDRICAL_SURFACE('',#95937,3.60000000004514);
#87227=CYLINDRICAL_SURFACE('',#95942,0.6);
#87228=CYLINDRICAL_SURFACE('',#95943,0.6);
#87229=CYLINDRICAL_SURFACE('',#95944,0.6);
#87230=CYLINDRICAL_SURFACE('',#95947,3.43614417320658);
#87231=CYLINDRICAL_SURFACE('',#95949,10.45);
#87232=CYLINDRICAL_SURFACE('',#95953,0.6);
#87233=CYLINDRICAL_SURFACE('',#95954,100.);
#87234=CYLINDRICAL_SURFACE('',#95956,0.8);
#87235=CYLINDRICAL_SURFACE('',#95959,0.6);
#87236=CYLINDRICAL_SURFACE('',#95961,3.6);
#87237=CYLINDRICAL_SURFACE('',#95963,0.6);
#87238=CYLINDRICAL_SURFACE('',#95964,3.7);
#87239=CYLINDRICAL_SURFACE('',#95965,3.6);
#87240=CYLINDRICAL_SURFACE('',#95967,0.6);
#87241=CYLINDRICAL_SURFACE('',#95969,0.6);
#87242=CYLINDRICAL_SURFACE('',#95970,3.2);
#87243=CYLINDRICAL_SURFACE('',#95971,0.8);
#87244=CYLINDRICAL_SURFACE('',#95972,13.4);
#87245=CYLINDRICAL_SURFACE('',#95974,0.8);
#87246=CYLINDRICAL_SURFACE('',#95975,0.6);
#87247=CYLINDRICAL_SURFACE('',#95977,0.6);
#87248=CYLINDRICAL_SURFACE('',#95978,9.70000001490116);
#87249=CYLINDRICAL_SURFACE('',#95979,0.6);
#87250=CYLINDRICAL_SURFACE('',#95980,0.79999999999745);
#87251=CYLINDRICAL_SURFACE('',#95991,4.);
#87252=CYLINDRICAL_SURFACE('',#95992,3.75);
#87253=CYLINDRICAL_SURFACE('',#95994,0.4);
#87254=CYLINDRICAL_SURFACE('',#95996,0.8);
#87255=CYLINDRICAL_SURFACE('',#96000,1.6);
#87256=CYLINDRICAL_SURFACE('',#96004,1.55);
#87257=CYLINDRICAL_SURFACE('',#96005,3.25);
#87258=CYLINDRICAL_SURFACE('',#96008,3.25);
#87259=CYLINDRICAL_SURFACE('',#96010,1.6);
#87260=CYLINDRICAL_SURFACE('',#96013,1.6);
#87261=CYLINDRICAL_SURFACE('',#96018,3.05);
#87262=CYLINDRICAL_SURFACE('',#96019,2.);
#87263=CYLINDRICAL_SURFACE('',#96021,1.58);
#87264=CYLINDRICAL_SURFACE('',#96023,2.);
#87265=CYLINDRICAL_SURFACE('',#96026,10.9);
#87266=CYLINDRICAL_SURFACE('',#96028,4.);
#87267=CYLINDRICAL_SURFACE('',#96029,1.);
#87268=CYLINDRICAL_SURFACE('',#96035,1.6);
#87269=CYLINDRICAL_SURFACE('',#96036,1.55);
#87270=CYLINDRICAL_SURFACE('',#96038,0.4);
#87271=CYLINDRICAL_SURFACE('',#96040,1.);
#87272=CYLINDRICAL_SURFACE('',#96042,2.);
#87273=CYLINDRICAL_SURFACE('',#96045,3.3);
#87274=CYLINDRICAL_SURFACE('',#96050,6.4499999999938);
#87275=CYLINDRICAL_SURFACE('',#96051,11.65);
#87276=CYLINDRICAL_SURFACE('',#96052,0.8);
#87277=CYLINDRICAL_SURFACE('',#96067,5.);
#87278=CYLINDRICAL_SURFACE('',#96069,0.8);
#87279=CYLINDRICAL_SURFACE('',#96080,0.4);
#87280=CYLINDRICAL_SURFACE('',#96085,0.4);
#87281=CYLINDRICAL_SURFACE('',#96096,0.8);
#87282=CYLINDRICAL_SURFACE('',#96098,10.6);
#87283=CYLINDRICAL_SURFACE('',#96100,0.6);
#87284=CYLINDRICAL_SURFACE('',#96102,4.65);
#87285=CYLINDRICAL_SURFACE('',#96114,0.4);
#87286=CYLINDRICAL_SURFACE('',#96129,0.4);
#87287=CYLINDRICAL_SURFACE('',#96130,4.);
#87288=CYLINDRICAL_SURFACE('',#96132,9.3949617393671);
#87289=CYLINDRICAL_SURFACE('',#96135,17.3949617393671);
#87290=CYLINDRICAL_SURFACE('',#96149,11.55);
#87291=CYLINDRICAL_SURFACE('',#96151,0.599999999999999);
#87292=CYLINDRICAL_SURFACE('',#96152,3.8);
#87293=CYLINDRICAL_SURFACE('',#96155,0.4);
#87294=CYLINDRICAL_SURFACE('',#96164,0.4);
#87295=CYLINDRICAL_SURFACE('',#96169,0.6);
#87296=CYLINDRICAL_SURFACE('',#96172,0.4);
#87297=CYLINDRICAL_SURFACE('',#96174,0.4);
#87298=CYLINDRICAL_SURFACE('',#96192,0.4);
#87299=CYLINDRICAL_SURFACE('',#96194,0.4);
#87300=CYLINDRICAL_SURFACE('',#96198,3.8);
#87301=CYLINDRICAL_SURFACE('',#96218,0.4);
#87302=CYLINDRICAL_SURFACE('',#96222,0.4);
#87303=CYLINDRICAL_SURFACE('',#96226,0.4);
#87304=CYLINDRICAL_SURFACE('',#96232,0.600000000000001);
#87305=CYLINDRICAL_SURFACE('',#96234,3.6);
#87306=CYLINDRICAL_SURFACE('',#96236,3.7);
#87307=CYLINDRICAL_SURFACE('',#96239,0.6);
#87308=CYLINDRICAL_SURFACE('',#96242,0.6);
#87309=CYLINDRICAL_SURFACE('',#96245,0.6);
#87310=CYLINDRICAL_SURFACE('',#96247,9.2);
#87311=CYLINDRICAL_SURFACE('',#96261,0.4);
#87312=CYLINDRICAL_SURFACE('',#96267,0.4);
#87313=CYLINDRICAL_SURFACE('',#96284,0.4);
#87314=CYLINDRICAL_SURFACE('',#96292,0.8);
#87315=CYLINDRICAL_SURFACE('',#96295,0.8);
#87316=CYLINDRICAL_SURFACE('',#96297,7.69496173936711);
#87317=CYLINDRICAL_SURFACE('',#96299,5.7);
#87318=CYLINDRICAL_SURFACE('',#96302,0.4);
#87319=CYLINDRICAL_SURFACE('',#96308,0.4);
#87320=CYLINDRICAL_SURFACE('',#96317,0.4);
#87321=CYLINDRICAL_SURFACE('',#96333,0.4);
#87322=CYLINDRICAL_SURFACE('',#96337,0.6);
#87323=CYLINDRICAL_SURFACE('',#96339,19.0949617393671);
#87324=CYLINDRICAL_SURFACE('',#96341,0.8);
#87325=CYLINDRICAL_SURFACE('',#96344,0.8);
#87326=CYLINDRICAL_SURFACE('',#96348,0.4);
#87327=CYLINDRICAL_SURFACE('',#96354,0.4);
#87328=CYLINDRICAL_SURFACE('',#96359,0.4);
#87329=CYLINDRICAL_SURFACE('',#96382,6.6);
#87330=CYLINDRICAL_SURFACE('',#96384,0.6);
#87331=CYLINDRICAL_SURFACE('',#96386,22.5949617393671);
#87332=CYLINDRICAL_SURFACE('',#96389,9.2);
#87333=CYLINDRICAL_SURFACE('',#96393,0.6);
#87334=CYLINDRICAL_SURFACE('',#96411,0.4);
#87335=CYLINDRICAL_SURFACE('',#96413,0.4);
#87336=CYLINDRICAL_SURFACE('',#96415,0.6);
#87337=CYLINDRICAL_SURFACE('',#96421,3.7);
#87338=CYLINDRICAL_SURFACE('',#96423,11.65);
#87339=CYLINDRICAL_SURFACE('',#96426,0.4);
#87340=CYLINDRICAL_SURFACE('',#96433,0.4);
#87341=CYLINDRICAL_SURFACE('',#96445,0.4);
#87342=CYLINDRICAL_SURFACE('',#96458,0.4);
#87343=CYLINDRICAL_SURFACE('',#96462,0.6);
#87344=CYLINDRICAL_SURFACE('',#96464,3.5);
#87345=CYLINDRICAL_SURFACE('',#96471,0.6);
#87346=CYLINDRICAL_SURFACE('',#96474,0.800000000000001);
#87347=CYLINDRICAL_SURFACE('',#96485,0.4);
#87348=CYLINDRICAL_SURFACE('',#96490,0.4);
#87349=CYLINDRICAL_SURFACE('',#96501,0.4);
#87350=CYLINDRICAL_SURFACE('',#96513,0.6);
#87351=CYLINDRICAL_SURFACE('',#96516,9.2);
#87352=CYLINDRICAL_SURFACE('',#96533,0.4);
#87353=CYLINDRICAL_SURFACE('',#96544,0.4);
#87354=CYLINDRICAL_SURFACE('',#96549,0.4);
#87355=CYLINDRICAL_SURFACE('',#96554,0.6);
#87356=CYLINDRICAL_SURFACE('',#96557,0.6);
#87357=CYLINDRICAL_SURFACE('',#96559,9.2);
#87358=CYLINDRICAL_SURFACE('',#96566,0.8);
#87359=CYLINDRICAL_SURFACE('',#96569,0.6);
#87360=CYLINDRICAL_SURFACE('',#96571,0.6);
#87361=CYLINDRICAL_SURFACE('',#96573,3.2);
#87362=CYLINDRICAL_SURFACE('',#96575,0.399999999999999);
#87363=CYLINDRICAL_SURFACE('',#96580,0.4);
#87364=CYLINDRICAL_SURFACE('',#96583,0.6);
#87365=CYLINDRICAL_SURFACE('',#96585,0.8);
#87366=CYLINDRICAL_SURFACE('',#96588,0.8);
#87367=CYLINDRICAL_SURFACE('',#96591,3.43614417320659);
#87368=CYLINDRICAL_SURFACE('',#96595,3.60000000004514);
#87369=CYLINDRICAL_SURFACE('',#96601,1.6);
#87370=CYLINDRICAL_SURFACE('',#96603,2.8);
#87371=CYLINDRICAL_SURFACE('',#96606,0.4);
#87372=CYLINDRICAL_SURFACE('',#96608,4.2);
#87373=CYLINDRICAL_SURFACE('',#96610,0.800000000000001);
#87374=CYLINDRICAL_SURFACE('',#96612,0.4);
#87375=CYLINDRICAL_SURFACE('',#96615,0.8);
#87376=CYLINDRICAL_SURFACE('',#96619,0.6);
#87377=CYLINDRICAL_SURFACE('',#96622,4.);
#87378=CYLINDRICAL_SURFACE('',#96625,0.8);
#87379=CYLINDRICAL_SURFACE('',#96628,4.2);
#87380=CYLINDRICAL_SURFACE('',#96631,1.55);
#87381=CYLINDRICAL_SURFACE('',#96634,0.4);
#87382=CYLINDRICAL_SURFACE('',#96637,0.75);
#87383=CYLINDRICAL_SURFACE('',#96640,2.5);
#87384=CYLINDRICAL_SURFACE('',#96641,2.5);
#87385=CYLINDRICAL_SURFACE('',#96642,1.3);
#87386=CYLINDRICAL_SURFACE('',#96649,1.3);
#87387=CYLINDRICAL_SURFACE('',#96664,2.5);
#87388=CYLINDRICAL_SURFACE('',#96669,2.5);
#87389=CYLINDRICAL_SURFACE('',#96676,2.5);
#87390=CYLINDRICAL_SURFACE('',#96681,2.5);
#87391=CYLINDRICAL_SURFACE('',#96684,1.3);
#87392=CYLINDRICAL_SURFACE('',#96690,1.3);
#87393=CYLINDRICAL_SURFACE('',#96697,3.6);
#87394=CYLINDRICAL_SURFACE('',#96700,0.6);
#87395=CYLINDRICAL_SURFACE('',#96705,3.6);
#87396=CYLINDRICAL_SURFACE('',#96710,2.);
#87397=CYLINDRICAL_SURFACE('',#96715,0.6);
#87398=CYLINDRICAL_SURFACE('',#96719,3.7);
#87399=CYLINDRICAL_SURFACE('',#96720,0.6);
#87400=CYLINDRICAL_SURFACE('',#96726,0.6);
#87401=CYLINDRICAL_SURFACE('',#96728,5.79999999999998);
#87402=CYLINDRICAL_SURFACE('',#96730,0.6);
#87403=CYLINDRICAL_SURFACE('',#96733,1.);
#87404=CYLINDRICAL_SURFACE('',#96735,11.55);
#87405=CYLINDRICAL_SURFACE('',#96737,0.6);
#87406=CYLINDRICAL_SURFACE('',#96740,10.45);
#87407=CYLINDRICAL_SURFACE('',#96745,10.35);
#87408=CYLINDRICAL_SURFACE('',#96749,1.);
#87409=CYLINDRICAL_SURFACE('',#96750,1.);
#87410=CYLINDRICAL_SURFACE('',#96751,1.);
#87411=CYLINDRICAL_SURFACE('',#96754,0.6);
#87412=CYLINDRICAL_SURFACE('',#96756,0.599999999999999);
#87413=CYLINDRICAL_SURFACE('',#96761,2.8);
#87414=CYLINDRICAL_SURFACE('',#96764,3.6);
#87415=CYLINDRICAL_SURFACE('',#96767,0.4);
#87416=CYLINDRICAL_SURFACE('',#96768,24.9449617393673);
#87417=CYLINDRICAL_SURFACE('',#96769,0.6);
#87418=CYLINDRICAL_SURFACE('',#96771,6.44999999999379);
#87419=CYLINDRICAL_SURFACE('',#96773,1.);
#87420=CYLINDRICAL_SURFACE('',#96775,11.65);
#87421=CYLINDRICAL_SURFACE('',#96782,4.15);
#87422=CYLINDRICAL_SURFACE('',#96786,2.8);
#87423=CYLINDRICAL_SURFACE('',#96789,2.85);
#87424=CYLINDRICAL_SURFACE('',#96790,1.6);
#87425=CYLINDRICAL_SURFACE('',#96793,0.6);
#87426=CYLINDRICAL_SURFACE('',#96797,2.);
#87427=CYLINDRICAL_SURFACE('',#96799,0.4);
#87428=CYLINDRICAL_SURFACE('',#96802,10.35);
#87429=CYLINDRICAL_SURFACE('',#96805,0.75);
#87430=CYLINDRICAL_SURFACE('',#96808,10.);
#87431=CYLINDRICAL_SURFACE('',#96811,0.4);
#87432=CYLINDRICAL_SURFACE('',#96813,2.5);
#87433=CYLINDRICAL_SURFACE('',#96815,3.1);
#87434=CYLINDRICAL_SURFACE('',#96819,2.5);
#87435=CYLINDRICAL_SURFACE('',#96821,0.6);
#87436=CYLINDRICAL_SURFACE('',#96827,0.6);
#87437=CYLINDRICAL_SURFACE('',#96834,1.55);
#87438=CYLINDRICAL_SURFACE('',#96836,2.);
#87439=CYLINDRICAL_SURFACE('',#96843,23.7449617393671);
#87440=CYLINDRICAL_SURFACE('',#96846,1.65);
#87441=CYLINDRICAL_SURFACE('',#96862,2.1);
#87442=CYLINDRICAL_SURFACE('',#96863,5.35);
#87443=CYLINDRICAL_SURFACE('',#96867,3.3);
#87444=CYLINDRICAL_SURFACE('',#96874,2.2);
#87445=CYLINDRICAL_SURFACE('',#96877,0.75);
#87446=CYLINDRICAL_SURFACE('',#96882,0.5);
#87447=CYLINDRICAL_SURFACE('',#96887,3.2);
#87448=CYLINDRICAL_SURFACE('',#96889,0.4);
#87449=CYLINDRICAL_SURFACE('',#96894,0.4);
#87450=CYLINDRICAL_SURFACE('',#96899,0.4);
#87451=CYLINDRICAL_SURFACE('',#96903,0.4);
#87452=CYLINDRICAL_SURFACE('',#96905,2.8);
#87453=CYLINDRICAL_SURFACE('',#96907,0.6);
#87454=CYLINDRICAL_SURFACE('',#96908,24.9449617393673);
#87455=CYLINDRICAL_SURFACE('',#96911,0.6);
#87456=CYLINDRICAL_SURFACE('',#96917,0.6);
#87457=CYLINDRICAL_SURFACE('',#96919,4.1);
#87458=CYLINDRICAL_SURFACE('',#96921,0.6);
#87459=CYLINDRICAL_SURFACE('',#96924,1.);
#87460=CYLINDRICAL_SURFACE('',#96927,2.5);
#87461=CYLINDRICAL_SURFACE('',#96931,1.);
#87462=CYLINDRICAL_SURFACE('',#96940,0.6);
#87463=CYLINDRICAL_SURFACE('',#96942,0.8);
#87464=CYLINDRICAL_SURFACE('',#96945,0.8);
#87465=CYLINDRICAL_SURFACE('',#96948,0.8);
#87466=CYLINDRICAL_SURFACE('',#96952,0.8);
#87467=CYLINDRICAL_SURFACE('',#96955,0.8);
#87468=CYLINDRICAL_SURFACE('',#96961,0.8);
#87469=CYLINDRICAL_SURFACE('',#96963,0.8);
#87470=CYLINDRICAL_SURFACE('',#96965,5.25);
#87471=CYLINDRICAL_SURFACE('',#96972,0.4);
#87472=CYLINDRICAL_SURFACE('',#96974,10.45);
#87473=CYLINDRICAL_SURFACE('',#96978,0.4);
#87474=CYLINDRICAL_SURFACE('',#96981,3.05);
#87475=CYLINDRICAL_SURFACE('',#97003,0.6);
#87476=CYLINDRICAL_SURFACE('',#97005,1.);
#87477=CYLINDRICAL_SURFACE('',#97019,0.2);
#87478=CYLINDRICAL_SURFACE('',#97020,0.2);
#87479=CYLINDRICAL_SURFACE('',#97021,0.2);
#87480=CYLINDRICAL_SURFACE('',#97023,0.2);
#87481=CYLINDRICAL_SURFACE('',#97025,0.2);
#87482=CYLINDRICAL_SURFACE('',#97028,0.2);
#87483=CYLINDRICAL_SURFACE('',#97032,0.2);
#87484=CYLINDRICAL_SURFACE('',#97034,0.2);
#87485=CYLINDRICAL_SURFACE('',#97043,0.4);
#87486=CYLINDRICAL_SURFACE('',#97045,0.6);
#87487=CYLINDRICAL_SURFACE('',#97046,0.6);
#87488=CYLINDRICAL_SURFACE('',#97048,0.6);
#87489=CYLINDRICAL_SURFACE('',#97050,0.4);
#87490=CYLINDRICAL_SURFACE('',#97052,10.6);
#87491=CYLINDRICAL_SURFACE('',#97054,0.4);
#87492=CYLINDRICAL_SURFACE('',#97059,0.4);
#87493=CYLINDRICAL_SURFACE('',#97061,0.6);
#87494=CYLINDRICAL_SURFACE('',#97063,0.6);
#87495=CYLINDRICAL_SURFACE('',#97065,0.6);
#87496=CYLINDRICAL_SURFACE('',#97066,4.8);
#87497=CYLINDRICAL_SURFACE('',#97067,3.7);
#87498=CYLINDRICAL_SURFACE('',#97069,7.8);
#87499=CYLINDRICAL_SURFACE('',#97072,0.8);
#87500=CYLINDRICAL_SURFACE('',#97078,0.8);
#87501=CYLINDRICAL_SURFACE('',#97082,4.);
#87502=CYLINDRICAL_SURFACE('',#97084,1.);
#87503=CYLINDRICAL_SURFACE('',#97087,0.8);
#89049=ADVANCED_FACE('',(#6585),#87130,.F.);
#89050=ADVANCED_FACE('',(#6586),#2221,.T.);
#89051=ADVANCED_FACE('',(#6587),#1621,.F.);
#89052=ADVANCED_FACE('',(#6588),#2222,.T.);
#89053=ADVANCED_FACE('',(#6589),#1622,.F.);
#89054=ADVANCED_FACE('',(#6590),#2223,.T.);
#89055=ADVANCED_FACE('',(#6591),#1623,.F.);
#89056=ADVANCED_FACE('',(#6592),#2224,.T.);
#89057=ADVANCED_FACE('',(#6593),#87131,.F.);
#89058=ADVANCED_FACE('',(#6594),#2225,.T.);
#89059=ADVANCED_FACE('',(#6595),#87132,.F.);
#89060=ADVANCED_FACE('',(#6596),#87133,.F.);
#89061=ADVANCED_FACE('',(#6597),#5352,.T.);
#89062=ADVANCED_FACE('',(#6598),#87134,.F.);
#89063=ADVANCED_FACE('',(#6599),#5353,.T.);
#89064=ADVANCED_FACE('',(#6600),#5354,.T.);
#89065=ADVANCED_FACE('',(#6601),#87135,.F.);
#89066=ADVANCED_FACE('',(#6602),#2226,.T.);
#89067=ADVANCED_FACE('',(#6603),#1624,.F.);
#89068=ADVANCED_FACE('',(#6604),#2227,.T.);
#89069=ADVANCED_FACE('',(#6605),#87136,.F.);
#89070=ADVANCED_FACE('',(#6606),#2228,.T.);
#89071=ADVANCED_FACE('',(#6607),#87137,.F.);
#89072=ADVANCED_FACE('',(#6608),#1625,.F.);
#89073=ADVANCED_FACE('',(#6609),#87138,.F.);
#89074=ADVANCED_FACE('',(#6610),#2229,.T.);
#89075=ADVANCED_FACE('',(#6611),#1626,.F.);
#89076=ADVANCED_FACE('',(#6612),#2230,.T.);
#89077=ADVANCED_FACE('',(#6613),#1627,.F.);
#89078=ADVANCED_FACE('',(#6614),#2231,.T.);
#89079=ADVANCED_FACE('',(#6615),#5355,.T.);
#89080=ADVANCED_FACE('',(#6616),#87139,.F.);
#89081=ADVANCED_FACE('',(#6617),#87140,.T.);
#89082=ADVANCED_FACE('',(#6618),#87141,.F.);
#89083=ADVANCED_FACE('',(#6619),#87142,.T.);
#89084=ADVANCED_FACE('',(#6620),#87143,.F.);
#89085=ADVANCED_FACE('',(#6621),#5356,.F.);
#89086=ADVANCED_FACE('',(#6622),#5357,.F.);
#89087=ADVANCED_FACE('',(#6623),#1628,.F.);
#89088=ADVANCED_FACE('',(#6624),#2232,.T.);
#89089=ADVANCED_FACE('',(#6625),#87144,.F.);
#89090=ADVANCED_FACE('',(#6626),#2233,.T.);
#89091=ADVANCED_FACE('',(#6627),#87145,.F.);
#89092=ADVANCED_FACE('',(#6628),#2234,.T.);
#89093=ADVANCED_FACE('',(#6629),#1629,.F.);
#89094=ADVANCED_FACE('',(#6630),#2235,.T.);
#89095=ADVANCED_FACE('',(#6631),#87146,.F.);
#89096=ADVANCED_FACE('',(#6632),#2236,.T.);
#89097=ADVANCED_FACE('',(#6633),#1630,.F.);
#89098=ADVANCED_FACE('',(#6634),#2237,.T.);
#89099=ADVANCED_FACE('',(#6635),#87147,.F.);
#89100=ADVANCED_FACE('',(#6636),#5358,.F.);
#89101=ADVANCED_FACE('',(#6637),#87148,.F.);
#89102=ADVANCED_FACE('',(#6638),#87149,.F.);
#89103=ADVANCED_FACE('',(#6639),#87150,.T.);
#89104=ADVANCED_FACE('',(#6640),#5359,.F.);
#89105=ADVANCED_FACE('',(#6641),#87151,.F.);
#89106=ADVANCED_FACE('',(#6642),#2238,.T.);
#89107=ADVANCED_FACE('',(#6643),#1631,.F.);
#89108=ADVANCED_FACE('',(#6644),#2239,.T.);
#89109=ADVANCED_FACE('',(#6645),#1632,.F.);
#89110=ADVANCED_FACE('',(#6646),#1633,.F.);
#89111=ADVANCED_FACE('',(#6647),#87152,.F.);
#89112=ADVANCED_FACE('',(#6648),#1634,.F.);
#89113=ADVANCED_FACE('',(#6649),#2240,.T.);
#89114=ADVANCED_FACE('',(#6650),#87153,.F.);
#89115=ADVANCED_FACE('',(#6651),#2241,.T.);
#89116=ADVANCED_FACE('',(#6652),#5360,.F.);
#89117=ADVANCED_FACE('',(#6653),#87154,.T.);
#89118=ADVANCED_FACE('',(#6654),#87155,.F.);
#89119=ADVANCED_FACE('',(#6655),#5361,.F.);
#89120=ADVANCED_FACE('',(#6656),#87156,.F.);
#89121=ADVANCED_FACE('',(#6657),#5362,.F.);
#89122=ADVANCED_FACE('',(#6658),#5363,.T.);
#89123=ADVANCED_FACE('',(#6659),#1635,.F.);
#89124=ADVANCED_FACE('',(#6660),#2242,.T.);
#89125=ADVANCED_FACE('',(#6661),#1636,.F.);
#89126=ADVANCED_FACE('',(#6662),#1637,.F.);
#89127=ADVANCED_FACE('',(#6663),#2243,.T.);
#89128=ADVANCED_FACE('',(#6664),#87157,.F.);
#89129=ADVANCED_FACE('',(#6665),#1638,.F.);
#89130=ADVANCED_FACE('',(#6666),#87158,.F.);
#89131=ADVANCED_FACE('',(#6667),#2244,.T.);
#89132=ADVANCED_FACE('',(#6668),#87159,.F.);
#89133=ADVANCED_FACE('',(#6669),#2245,.T.);
#89134=ADVANCED_FACE('',(#6670),#1639,.F.);
#89135=ADVANCED_FACE('',(#6671),#2246,.T.);
#89136=ADVANCED_FACE('',(#6672),#87160,.F.);
#89137=ADVANCED_FACE('',(#6673),#87161,.F.);
#89138=ADVANCED_FACE('',(#6674),#5364,.F.);
#89139=ADVANCED_FACE('',(#6675),#87162,.F.);
#89140=ADVANCED_FACE('',(#6676),#87163,.T.);
#89141=ADVANCED_FACE('',(#6677),#87164,.F.);
#89142=ADVANCED_FACE('',(#6678),#5365,.F.);
#89143=ADVANCED_FACE('',(#6679),#87165,.T.);
#89144=ADVANCED_FACE('',(#6680),#5366,.T.);
#89145=ADVANCED_FACE('',(#6681),#1640,.F.);
#89146=ADVANCED_FACE('',(#6682),#1641,.F.);
#89147=ADVANCED_FACE('',(#6683),#2247,.T.);
#89148=ADVANCED_FACE('',(#6684),#1642,.F.);
#89149=ADVANCED_FACE('',(#6685),#2248,.T.);
#89150=ADVANCED_FACE('',(#6686),#1643,.F.);
#89151=ADVANCED_FACE('',(#6687),#2249,.T.);
#89152=ADVANCED_FACE('',(#6688),#87166,.F.);
#89153=ADVANCED_FACE('',(#6689),#2250,.T.);
#89154=ADVANCED_FACE('',(#6690),#87167,.F.);
#89155=ADVANCED_FACE('',(#6691),#87168,.F.);
#89156=ADVANCED_FACE('',(#6692),#5367,.T.);
#89157=ADVANCED_FACE('',(#6693),#87169,.F.);
#89158=ADVANCED_FACE('',(#6694),#87170,.T.);
#89159=ADVANCED_FACE('',(#6695),#5368,.T.);
#89160=ADVANCED_FACE('',(#6696),#1644,.F.);
#89161=ADVANCED_FACE('',(#6697),#2251,.T.);
#89162=ADVANCED_FACE('',(#6698),#1645,.F.);
#89163=ADVANCED_FACE('',(#6699),#1646,.F.);
#89164=ADVANCED_FACE('',(#6700),#1647,.F.);
#89165=ADVANCED_FACE('',(#6701),#2252,.T.);
#89166=ADVANCED_FACE('',(#6702),#87171,.F.);
#89167=ADVANCED_FACE('',(#6703),#2253,.T.);
#89168=ADVANCED_FACE('',(#6704),#87172,.F.);
#89169=ADVANCED_FACE('',(#6705),#2254,.T.);
#89170=ADVANCED_FACE('',(#6706),#87173,.F.);
#89171=ADVANCED_FACE('',(#6707),#2255,.T.);
#89172=ADVANCED_FACE('',(#6708),#1648,.F.);
#89173=ADVANCED_FACE('',(#6709),#2256,.T.);
#89174=ADVANCED_FACE('',(#6710),#1649,.F.);
#89175=ADVANCED_FACE('',(#6711),#2257,.T.);
#89176=ADVANCED_FACE('',(#6712),#87174,.F.);
#89177=ADVANCED_FACE('',(#6713),#5369,.T.);
#89178=ADVANCED_FACE('',(#6714),#87175,.F.);
#89179=ADVANCED_FACE('',(#6715),#87176,.T.);
#89180=ADVANCED_FACE('',(#6716),#87177,.F.);
#89181=ADVANCED_FACE('',(#6717),#87178,.T.);
#89182=ADVANCED_FACE('',(#6718),#87179,.F.);
#89183=ADVANCED_FACE('',(#6719),#87180,.T.);
#89184=ADVANCED_FACE('',(#6720),#5370,.T.);
#89185=ADVANCED_FACE('',(#6721),#1650,.F.);
#89186=ADVANCED_FACE('',(#6722),#2258,.T.);
#89187=ADVANCED_FACE('',(#6723),#1651,.F.);
#89188=ADVANCED_FACE('',(#6724),#87181,.F.);
#89189=ADVANCED_FACE('',(#6725),#2259,.T.);
#89190=ADVANCED_FACE('',(#6726),#1652,.F.);
#89191=ADVANCED_FACE('',(#6727),#2260,.T.);
#89192=ADVANCED_FACE('',(#6728),#1653,.F.);
#89193=ADVANCED_FACE('',(#6729),#2261,.T.);
#89194=ADVANCED_FACE('',(#6730),#87182,.F.);
#89195=ADVANCED_FACE('',(#6731),#87183,.F.);
#89196=ADVANCED_FACE('',(#6732),#87184,.T.);
#89197=ADVANCED_FACE('',(#6733),#87185,.F.);
#89198=ADVANCED_FACE('',(#6734),#87186,.T.);
#89199=ADVANCED_FACE('',(#6735),#5371,.T.);
#89200=ADVANCED_FACE('',(#6736),#87187,.F.);
#89201=ADVANCED_FACE('',(#6737),#2262,.T.);
#89202=ADVANCED_FACE('',(#6738),#87188,.F.);
#89203=ADVANCED_FACE('',(#6739),#2263,.T.);
#89204=ADVANCED_FACE('',(#6740),#1654,.F.);
#89205=ADVANCED_FACE('',(#6741),#2264,.T.);
#89206=ADVANCED_FACE('',(#6742),#1655,.F.);
#89207=ADVANCED_FACE('',(#6743),#2265,.T.);
#89208=ADVANCED_FACE('',(#6744),#87189,.F.);
#89209=ADVANCED_FACE('',(#6745),#87190,.T.);
#89210=ADVANCED_FACE('',(#6746),#87191,.F.);
#89211=ADVANCED_FACE('',(#6747),#5372,.F.);
#89212=ADVANCED_FACE('',(#6748),#5373,.T.);
#89213=ADVANCED_FACE('',(#6749),#6205,.T.);
#89214=ADVANCED_FACE('',(#6750),#6206,.T.);
#89215=ADVANCED_FACE('',(#6751),#6207,.T.);
#89216=ADVANCED_FACE('',(#6752),#87192,.T.);
#89217=ADVANCED_FACE('',(#6753),#87193,.F.);
#89218=ADVANCED_FACE('',(#6754),#4672,.T.);
#89219=ADVANCED_FACE('',(#6755),#87194,.T.);
#89220=ADVANCED_FACE('',(#6756),#5374,.T.);
#89221=ADVANCED_FACE('',(#6757),#5375,.F.);
#89222=ADVANCED_FACE('',(#6758),#87195,.T.);
#89223=ADVANCED_FACE('',(#6759,#5126),#5376,.T.);
#89224=ADVANCED_FACE('',(#6760),#87196,.F.);
#89225=ADVANCED_FACE('',(#6761,#5127,#5128),#5377,.T.);
#89226=ADVANCED_FACE('',(#6762),#5378,.T.);
#89227=ADVANCED_FACE('',(#6763),#87197,.T.);
#89228=ADVANCED_FACE('',(#6764),#5379,.F.);
#89229=ADVANCED_FACE('',(#6765,#5129,#5130,#5131,#5132,#5133),#5380,.F.);
#89230=ADVANCED_FACE('',(#6766),#87198,.F.);
#89231=ADVANCED_FACE('',(#6767),#5381,.F.);
#89232=ADVANCED_FACE('',(#6768),#87199,.F.);
#89233=ADVANCED_FACE('',(#6769),#87200,.T.);
#89234=ADVANCED_FACE('',(#6770),#5382,.F.);
#89235=ADVANCED_FACE('',(#6771),#5383,.T.);
#89236=ADVANCED_FACE('',(#6772),#87201,.T.);
#89237=ADVANCED_FACE('',(#6773),#5384,.F.);
#89238=ADVANCED_FACE('',(#6774),#87202,.T.);
#89239=ADVANCED_FACE('',(#6775,#5134),#5385,.T.);
#89240=ADVANCED_FACE('',(#6776),#87203,.F.);
#89241=ADVANCED_FACE('',(#6777),#87204,.T.);
#89242=ADVANCED_FACE('',(#6778),#5386,.F.);
#89243=ADVANCED_FACE('',(#6779),#5387,.F.);
#89244=ADVANCED_FACE('',(#6780),#87205,.T.);
#89245=ADVANCED_FACE('',(#6781),#87206,.F.);
#89246=ADVANCED_FACE('',(#6782),#87207,.F.);
#89247=ADVANCED_FACE('',(#6783),#5388,.T.);
#89248=ADVANCED_FACE('',(#6784),#87208,.T.);
#89249=ADVANCED_FACE('',(#6785),#5389,.T.);
#89250=ADVANCED_FACE('',(#6786),#87209,.F.);
#89251=ADVANCED_FACE('',(#6787),#87210,.T.);
#89252=ADVANCED_FACE('',(#6788),#87211,.F.);
#89253=ADVANCED_FACE('',(#6789),#87212,.F.);
#89254=ADVANCED_FACE('',(#6790),#87213,.T.);
#89255=ADVANCED_FACE('',(#6791),#87214,.T.);
#89256=ADVANCED_FACE('',(#6792),#87215,.F.);
#89257=ADVANCED_FACE('',(#6793),#5390,.F.);
#89258=ADVANCED_FACE('',(#6794),#87216,.F.);
#89259=ADVANCED_FACE('',(#6795),#5391,.F.);
#89260=ADVANCED_FACE('',(#6796),#5392,.T.);
#89261=ADVANCED_FACE('',(#6797),#87217,.T.);
#89262=ADVANCED_FACE('',(#6798),#87218,.F.);
#89263=ADVANCED_FACE('',(#6799),#5393,.T.);
#89264=ADVANCED_FACE('',(#6800),#87219,.F.);
#89265=ADVANCED_FACE('',(#6801),#5394,.T.);
#89266=ADVANCED_FACE('',(#6802),#87220,.T.);
#89267=ADVANCED_FACE('',(#6803),#87221,.F.);
#89268=ADVANCED_FACE('',(#6804),#87222,.T.);
#89269=ADVANCED_FACE('',(#6805),#87223,.F.);
#89270=ADVANCED_FACE('',(#6806),#87224,.F.);
#89271=ADVANCED_FACE('',(#6807),#87225,.T.);
#89272=ADVANCED_FACE('',(#6808),#5395,.F.);
#89273=ADVANCED_FACE('',(#6809),#4673,.F.);
#89274=ADVANCED_FACE('',(#6810),#5396,.T.);
#89275=ADVANCED_FACE('',(#6811),#5397,.T.);
#89276=ADVANCED_FACE('',(#6812),#87226,.T.);
#89277=ADVANCED_FACE('',(#6813),#5398,.T.);
#89278=ADVANCED_FACE('',(#6814),#87227,.F.);
#89279=ADVANCED_FACE('',(#6815),#87228,.F.);
#89280=ADVANCED_FACE('',(#6816),#87229,.F.);
#89281=ADVANCED_FACE('',(#6817,#5135),#5399,.T.);
#89282=ADVANCED_FACE('',(#6818),#87230,.T.);
#89283=ADVANCED_FACE('',(#6819),#87231,.F.);
#89284=ADVANCED_FACE('',(#6820),#5400,.T.);
#89285=ADVANCED_FACE('',(#6821),#87232,.F.);
#89286=ADVANCED_FACE('',(#6822),#87233,.F.);
#89287=ADVANCED_FACE('',(#6823),#87234,.T.);
#89288=ADVANCED_FACE('',(#6824),#5401,.F.);
#89289=ADVANCED_FACE('',(#6825),#87235,.F.);
#89290=ADVANCED_FACE('',(#6826),#87236,.T.);
#89291=ADVANCED_FACE('',(#6827),#87237,.F.);
#89292=ADVANCED_FACE('',(#6828),#87238,.T.);
#89293=ADVANCED_FACE('',(#6829),#87239,.F.);
#89294=ADVANCED_FACE('',(#6830),#5402,.F.);
#89295=ADVANCED_FACE('',(#6831),#87240,.F.);
#89296=ADVANCED_FACE('',(#6832),#5403,.F.);
#89297=ADVANCED_FACE('',(#6833),#87241,.F.);
#89298=ADVANCED_FACE('',(#6834),#87242,.T.);
#89299=ADVANCED_FACE('',(#6835),#87243,.F.);
#89300=ADVANCED_FACE('',(#6836),#87244,.F.);
#89301=ADVANCED_FACE('',(#6837),#5404,.F.);
#89302=ADVANCED_FACE('',(#6838),#87245,.F.);
#89303=ADVANCED_FACE('',(#6839),#87246,.F.);
#89304=ADVANCED_FACE('',(#6840),#87247,.F.);
#89305=ADVANCED_FACE('',(#6841),#87248,.T.);
#89306=ADVANCED_FACE('',(#6842),#87249,.F.);
#89307=ADVANCED_FACE('',(#6843),#87250,.T.);
#89308=ADVANCED_FACE('',(#6844,#5136,#5137),#5405,.T.);
#89309=ADVANCED_FACE('',(#6845),#4674,.F.);
#89310=ADVANCED_FACE('',(#6846),#87251,.F.);
#89311=ADVANCED_FACE('',(#6847),#87252,.T.);
#89312=ADVANCED_FACE('',(#6848),#5406,.F.);
#89313=ADVANCED_FACE('',(#6849),#87253,.T.);
#89314=ADVANCED_FACE('',(#6850),#5407,.F.);
#89315=ADVANCED_FACE('',(#6851),#87254,.F.);
#89316=ADVANCED_FACE('',(#6852),#5408,.T.);
#89317=ADVANCED_FACE('',(#6853),#5409,.T.);
#89318=ADVANCED_FACE('',(#6854),#87255,.F.);
#89319=ADVANCED_FACE('',(#6855,#5138),#5410,.T.);
#89320=ADVANCED_FACE('',(#6856),#87256,.F.);
#89321=ADVANCED_FACE('',(#6857),#87257,.T.);
#89322=ADVANCED_FACE('',(#6858),#5411,.T.);
#89323=ADVANCED_FACE('',(#6859),#87258,.T.);
#89324=ADVANCED_FACE('',(#6860),#87259,.F.);
#89325=ADVANCED_FACE('',(#6861),#5412,.F.);
#89326=ADVANCED_FACE('',(#6862),#87260,.F.);
#89327=ADVANCED_FACE('',(#6863),#5413,.F.);
#89328=ADVANCED_FACE('',(#6864),#5414,.T.);
#89329=ADVANCED_FACE('',(#6865),#87261,.F.);
#89330=ADVANCED_FACE('',(#6866),#87262,.F.);
#89331=ADVANCED_FACE('',(#6867),#87263,.F.);
#89332=ADVANCED_FACE('',(#6868),#87264,.F.);
#89333=ADVANCED_FACE('',(#6869),#5415,.F.);
#89334=ADVANCED_FACE('',(#6870),#87265,.F.);
#89335=ADVANCED_FACE('',(#6871),#87266,.T.);
#89336=ADVANCED_FACE('',(#6872),#87267,.T.);
#89337=ADVANCED_FACE('',(#6873,#5139),#5416,.T.);
#89338=ADVANCED_FACE('',(#6874),#4675,.T.);
#89339=ADVANCED_FACE('',(#6875),#87268,.F.);
#89340=ADVANCED_FACE('',(#6876),#87269,.F.);
#89341=ADVANCED_FACE('',(#6877),#4676,.F.);
#89342=ADVANCED_FACE('',(#6878),#87270,.T.);
#89343=ADVANCED_FACE('',(#6879),#5417,.T.);
#89344=ADVANCED_FACE('',(#6880),#87271,.T.);
#89345=ADVANCED_FACE('',(#6881),#5418,.F.);
#89346=ADVANCED_FACE('',(#6882),#87272,.F.);
#89347=ADVANCED_FACE('',(#6883),#5419,.F.);
#89348=ADVANCED_FACE('',(#6884),#5420,.F.);
#89349=ADVANCED_FACE('',(#6885),#87273,.T.);
#89350=ADVANCED_FACE('',(#6886),#5421,.T.);
#89351=ADVANCED_FACE('',(#6887),#5422,.T.);
#89352=ADVANCED_FACE('',(#6888),#87274,.T.);
#89353=ADVANCED_FACE('',(#6889),#87275,.T.);
#89354=ADVANCED_FACE('',(#6890),#87276,.T.);
#89355=ADVANCED_FACE('',(#6891),#5423,.T.);
#89356=ADVANCED_FACE('',(#6892),#87277,.F.);
#89357=ADVANCED_FACE('',(#6893),#87278,.T.);
#89358=ADVANCED_FACE('',(#6894),#5424,.T.);
#89359=ADVANCED_FACE('',(#6895),#1656,.F.);
#89360=ADVANCED_FACE('',(#6896),#2266,.T.);
#89361=ADVANCED_FACE('',(#6897),#87279,.F.);
#89362=ADVANCED_FACE('',(#6898),#2267,.T.);
#89363=ADVANCED_FACE('',(#6899),#87280,.F.);
#89364=ADVANCED_FACE('',(#6900),#2268,.T.);
#89365=ADVANCED_FACE('',(#6901),#1657,.F.);
#89366=ADVANCED_FACE('',(#6902),#2269,.T.);
#89367=ADVANCED_FACE('',(#6903),#87281,.F.);
#89368=ADVANCED_FACE('',(#6904),#87282,.T.);
#89369=ADVANCED_FACE('',(#6905),#87283,.F.);
#89370=ADVANCED_FACE('',(#6906),#87284,.T.);
#89371=ADVANCED_FACE('',(#6907),#5425,.T.);
#89372=ADVANCED_FACE('',(#6908),#1658,.F.);
#89373=ADVANCED_FACE('',(#6909),#1659,.F.);
#89374=ADVANCED_FACE('',(#6910),#87285,.F.);
#89375=ADVANCED_FACE('',(#6911),#1660,.F.);
#89376=ADVANCED_FACE('',(#6912),#1661,.F.);
#89377=ADVANCED_FACE('',(#6913),#1662,.F.);
#89378=ADVANCED_FACE('',(#6914),#1663,.F.);
#89379=ADVANCED_FACE('',(#6915),#87286,.F.);
#89380=ADVANCED_FACE('',(#6916),#87287,.F.);
#89381=ADVANCED_FACE('',(#6917),#87288,.T.);
#89382=ADVANCED_FACE('',(#6918),#5426,.T.);
#89383=ADVANCED_FACE('',(#6919),#87289,.F.);
#89384=ADVANCED_FACE('',(#6920),#5427,.T.);
#89385=ADVANCED_FACE('',(#6921),#1664,.F.);
#89386=ADVANCED_FACE('',(#6922),#2270,.T.);
#89387=ADVANCED_FACE('',(#6923),#1665,.F.);
#89388=ADVANCED_FACE('',(#6924),#87290,.T.);
#89389=ADVANCED_FACE('',(#6925),#87291,.F.);
#89390=ADVANCED_FACE('',(#6926),#87292,.T.);
#89391=ADVANCED_FACE('',(#6927),#87293,.F.);
#89392=ADVANCED_FACE('',(#6928),#5428,.T.);
#89393=ADVANCED_FACE('',(#6929),#5429,.T.);
#89394=ADVANCED_FACE('',(#6930),#2271,.T.);
#89395=ADVANCED_FACE('',(#6931),#87294,.F.);
#89396=ADVANCED_FACE('',(#6932,#5140),#5430,.F.);
#89397=ADVANCED_FACE('',(#6933),#87295,.F.);
#89398=ADVANCED_FACE('',(#6934),#5431,.F.);
#89399=ADVANCED_FACE('',(#6935),#87296,.F.);
#89400=ADVANCED_FACE('',(#6936),#87297,.F.);
#89401=ADVANCED_FACE('',(#6937),#5432,.T.);
#89402=ADVANCED_FACE('',(#6938),#5433,.T.);
#89403=ADVANCED_FACE('',(#6939),#1666,.F.);
#89404=ADVANCED_FACE('',(#6940),#2272,.T.);
#89405=ADVANCED_FACE('',(#6941),#1667,.F.);
#89406=ADVANCED_FACE('',(#6942),#2273,.T.);
#89407=ADVANCED_FACE('',(#6943),#87298,.F.);
#89408=ADVANCED_FACE('',(#6944),#87299,.F.);
#89409=ADVANCED_FACE('',(#6945),#5434,.F.);
#89410=ADVANCED_FACE('',(#6946),#5435,.T.);
#89411=ADVANCED_FACE('',(#6947),#87300,.T.);
#89412=ADVANCED_FACE('',(#6948),#5436,.T.);
#89413=ADVANCED_FACE('',(#6949),#1668,.F.);
#89414=ADVANCED_FACE('',(#6950),#2274,.T.);
#89415=ADVANCED_FACE('',(#6951),#1669,.F.);
#89416=ADVANCED_FACE('',(#6952),#1670,.F.);
#89417=ADVANCED_FACE('',(#6953),#5437,.T.);
#89418=ADVANCED_FACE('',(#6954),#87301,.F.);
#89419=ADVANCED_FACE('',(#6955),#2275,.T.);
#89420=ADVANCED_FACE('',(#6956),#87302,.F.);
#89421=ADVANCED_FACE('',(#6957),#2276,.T.);
#89422=ADVANCED_FACE('',(#6958),#87303,.F.);
#89423=ADVANCED_FACE('',(#6959),#2277,.T.);
#89424=ADVANCED_FACE('',(#6960),#1671,.F.);
#89425=ADVANCED_FACE('',(#6961),#87304,.F.);
#89426=ADVANCED_FACE('',(#6962),#87305,.F.);
#89427=ADVANCED_FACE('',(#6963),#87306,.T.);
#89428=ADVANCED_FACE('',(#6964),#5438,.F.);
#89429=ADVANCED_FACE('',(#6965),#87307,.F.);
#89430=ADVANCED_FACE('',(#6966),#5439,.F.);
#89431=ADVANCED_FACE('',(#6967),#87308,.F.);
#89432=ADVANCED_FACE('',(#6968),#5440,.T.);
#89433=ADVANCED_FACE('',(#6969),#87309,.F.);
#89434=ADVANCED_FACE('',(#6970),#87310,.F.);
#89435=ADVANCED_FACE('',(#6971),#135,.T.);
#89436=ADVANCED_FACE('',(#6972),#1672,.F.);
#89437=ADVANCED_FACE('',(#6973),#2278,.T.);
#89438=ADVANCED_FACE('',(#6974),#87311,.F.);
#89439=ADVANCED_FACE('',(#6975),#1673,.F.);
#89440=ADVANCED_FACE('',(#6976),#87312,.F.);
#89441=ADVANCED_FACE('',(#6977),#2279,.T.);
#89442=ADVANCED_FACE('',(#6978),#1674,.F.);
#89443=ADVANCED_FACE('',(#6979),#2280,.T.);
#89444=ADVANCED_FACE('',(#6980),#1675,.F.);
#89445=ADVANCED_FACE('',(#6981),#87313,.F.);
#89446=ADVANCED_FACE('',(#6982),#1676,.F.);
#89447=ADVANCED_FACE('',(#6983),#136,.F.);
#89448=ADVANCED_FACE('',(#6984),#5441,.T.);
#89449=ADVANCED_FACE('',(#6985),#87314,.T.);
#89450=ADVANCED_FACE('',(#6986),#5442,.T.);
#89451=ADVANCED_FACE('',(#6987),#87315,.F.);
#89452=ADVANCED_FACE('',(#6988),#87316,.F.);
#89453=ADVANCED_FACE('',(#6989),#87317,.T.);
#89454=ADVANCED_FACE('',(#6990),#5443,.T.);
#89455=ADVANCED_FACE('',(#6991),#87318,.F.);
#89456=ADVANCED_FACE('',(#6992),#2281,.T.);
#89457=ADVANCED_FACE('',(#6993),#87319,.F.);
#89458=ADVANCED_FACE('',(#6994),#1677,.F.);
#89459=ADVANCED_FACE('',(#6995),#2282,.T.);
#89460=ADVANCED_FACE('',(#6996),#87320,.F.);
#89461=ADVANCED_FACE('',(#6997),#1678,.F.);
#89462=ADVANCED_FACE('',(#6998),#2283,.T.);
#89463=ADVANCED_FACE('',(#6999),#1679,.F.);
#89464=ADVANCED_FACE('',(#7000),#2284,.T.);
#89465=ADVANCED_FACE('',(#7001),#87321,.F.);
#89466=ADVANCED_FACE('',(#7002),#2285,.T.);
#89467=ADVANCED_FACE('',(#7003),#87322,.F.);
#89468=ADVANCED_FACE('',(#7004),#87323,.T.);
#89469=ADVANCED_FACE('',(#7005),#87324,.F.);
#89470=ADVANCED_FACE('',(#7006),#5444,.T.);
#89471=ADVANCED_FACE('',(#7007),#87325,.F.);
#89472=ADVANCED_FACE('',(#7008),#5445,.F.);
#89473=ADVANCED_FACE('',(#7009),#5446,.T.);
#89474=ADVANCED_FACE('',(#7010),#87326,.F.);
#89475=ADVANCED_FACE('',(#7011),#2286,.T.);
#89476=ADVANCED_FACE('',(#7012),#87327,.F.);
#89477=ADVANCED_FACE('',(#7013),#2287,.T.);
#89478=ADVANCED_FACE('',(#7014),#87328,.F.);
#89479=ADVANCED_FACE('',(#7015),#1680,.F.);
#89480=ADVANCED_FACE('',(#7016),#1681,.F.);
#89481=ADVANCED_FACE('',(#7017),#2288,.T.);
#89482=ADVANCED_FACE('',(#7018),#1682,.F.);
#89483=ADVANCED_FACE('',(#7019),#1683,.F.);
#89484=ADVANCED_FACE('',(#7020),#2289,.T.);
#89485=ADVANCED_FACE('',(#7021),#87329,.F.);
#89486=ADVANCED_FACE('',(#7022),#87330,.F.);
#89487=ADVANCED_FACE('',(#7023),#87331,.F.);
#89488=ADVANCED_FACE('',(#7024),#87332,.F.);
#89489=ADVANCED_FACE('',(#7025),#87333,.F.);
#89490=ADVANCED_FACE('',(#7026),#5447,.T.);
#89491=ADVANCED_FACE('',(#7027),#5448,.T.);
#89492=ADVANCED_FACE('',(#7028),#1684,.F.);
#89493=ADVANCED_FACE('',(#7029),#2290,.T.);
#89494=ADVANCED_FACE('',(#7030),#1685,.F.);
#89495=ADVANCED_FACE('',(#7031),#2291,.T.);
#89496=ADVANCED_FACE('',(#7032),#87334,.F.);
#89497=ADVANCED_FACE('',(#7033),#87335,.F.);
#89498=ADVANCED_FACE('',(#7034),#87336,.F.);
#89499=ADVANCED_FACE('',(#7035),#5449,.F.);
#89500=ADVANCED_FACE('',(#7036),#87337,.T.);
#89501=ADVANCED_FACE('',(#7037),#5450,.T.);
#89502=ADVANCED_FACE('',(#7038),#87338,.T.);
#89503=ADVANCED_FACE('',(#7039),#87339,.F.);
#89504=ADVANCED_FACE('',(#7040),#1686,.F.);
#89505=ADVANCED_FACE('',(#7041),#87340,.F.);
#89506=ADVANCED_FACE('',(#7042),#2292,.T.);
#89507=ADVANCED_FACE('',(#7043),#1687,.F.);
#89508=ADVANCED_FACE('',(#7044),#2293,.T.);
#89509=ADVANCED_FACE('',(#7045),#87341,.F.);
#89510=ADVANCED_FACE('',(#7046),#2294,.T.);
#89511=ADVANCED_FACE('',(#7047),#1688,.F.);
#89512=ADVANCED_FACE('',(#7048),#2295,.T.);
#89513=ADVANCED_FACE('',(#7049),#87342,.F.);
#89514=ADVANCED_FACE('',(#7050),#2296,.T.);
#89515=ADVANCED_FACE('',(#7051),#87343,.F.);
#89516=ADVANCED_FACE('',(#7052),#87344,.T.);
#89517=ADVANCED_FACE('',(#7053),#87345,.F.);
#89518=ADVANCED_FACE('',(#7054),#5451,.F.);
#89519=ADVANCED_FACE('',(#7055),#87346,.F.);
#89520=ADVANCED_FACE('',(#7056),#5452,.T.);
#89521=ADVANCED_FACE('',(#7057),#5453,.T.);
#89522=ADVANCED_FACE('',(#7058),#1689,.F.);
#89523=ADVANCED_FACE('',(#7059),#2297,.T.);
#89524=ADVANCED_FACE('',(#7060),#87347,.F.);
#89525=ADVANCED_FACE('',(#7061),#2298,.T.);
#89526=ADVANCED_FACE('',(#7062),#87348,.F.);
#89527=ADVANCED_FACE('',(#7063),#2299,.T.);
#89528=ADVANCED_FACE('',(#7064),#1690,.F.);
#89529=ADVANCED_FACE('',(#7065),#2300,.T.);
#89530=ADVANCED_FACE('',(#7066),#87349,.F.);
#89531=ADVANCED_FACE('',(#7067),#2301,.T.);
#89532=ADVANCED_FACE('',(#7068),#1691,.F.);
#89533=ADVANCED_FACE('',(#7069),#1692,.F.);
#89534=ADVANCED_FACE('',(#7070),#5454,.F.);
#89535=ADVANCED_FACE('',(#7071),#87350,.F.);
#89536=ADVANCED_FACE('',(#7072),#137,.T.);
#89537=ADVANCED_FACE('',(#7073),#87351,.F.);
#89538=ADVANCED_FACE('',(#7074),#5455,.T.);
#89539=ADVANCED_FACE('',(#7075),#1693,.F.);
#89540=ADVANCED_FACE('',(#7076),#2302,.T.);
#89541=ADVANCED_FACE('',(#7077),#87352,.F.);
#89542=ADVANCED_FACE('',(#7078),#2303,.T.);
#89543=ADVANCED_FACE('',(#7079),#1694,.F.);
#89544=ADVANCED_FACE('',(#7080),#2304,.T.);
#89545=ADVANCED_FACE('',(#7081),#87353,.F.);
#89546=ADVANCED_FACE('',(#7082),#2305,.T.);
#89547=ADVANCED_FACE('',(#7083),#87354,.F.);
#89548=ADVANCED_FACE('',(#7084),#2306,.T.);
#89549=ADVANCED_FACE('',(#7085),#5456,.F.);
#89550=ADVANCED_FACE('',(#7086),#87355,.F.);
#89551=ADVANCED_FACE('',(#7087),#5457,.T.);
#89552=ADVANCED_FACE('',(#7088),#87356,.F.);
#89553=ADVANCED_FACE('',(#7089),#87357,.F.);
#89554=ADVANCED_FACE('',(#7090),#5458,.T.);
#89555=ADVANCED_FACE('',(#7091),#87358,.T.);
#89556=ADVANCED_FACE('',(#7092),#5459,.T.);
#89557=ADVANCED_FACE('',(#7093),#87359,.F.);
#89558=ADVANCED_FACE('',(#7094),#87360,.F.);
#89559=ADVANCED_FACE('',(#7095),#87361,.T.);
#89560=ADVANCED_FACE('',(#7096),#87362,.T.);
#89561=ADVANCED_FACE('',(#7097),#5460,.F.);
#89562=ADVANCED_FACE('',(#7098),#5461,.T.);
#89563=ADVANCED_FACE('',(#7099),#87363,.T.);
#89564=ADVANCED_FACE('',(#7100),#87364,.F.);
#89565=ADVANCED_FACE('',(#7101),#87365,.T.);
#89566=ADVANCED_FACE('',(#7102),#87366,.F.);
#89567=ADVANCED_FACE('',(#7103),#87367,.T.);
#89568=ADVANCED_FACE('',(#7104),#5462,.F.);
#89569=ADVANCED_FACE('',(#7105),#87368,.T.);
#89570=ADVANCED_FACE('',(#7106,#5141),#5463,.T.);
#89571=ADVANCED_FACE('',(#7107),#87369,.F.);
#89572=ADVANCED_FACE('',(#7108),#87370,.F.);
#89573=ADVANCED_FACE('',(#7109),#5464,.T.);
#89574=ADVANCED_FACE('',(#7110),#87371,.F.);
#89575=ADVANCED_FACE('',(#7111),#87372,.T.);
#89576=ADVANCED_FACE('',(#7112),#87373,.F.);
#89577=ADVANCED_FACE('',(#7113),#87374,.T.);
#89578=ADVANCED_FACE('',(#7114),#87375,.T.);
#89579=ADVANCED_FACE('',(#7115),#5465,.F.);
#89580=ADVANCED_FACE('',(#7116),#87376,.F.);
#89581=ADVANCED_FACE('',(#7117),#5466,.T.);
#89582=ADVANCED_FACE('',(#7118),#87377,.T.);
#89583=ADVANCED_FACE('',(#7119),#87378,.T.);
#89584=ADVANCED_FACE('',(#7120),#87379,.F.);
#89585=ADVANCED_FACE('',(#7121),#87380,.F.);
#89586=ADVANCED_FACE('',(#7122),#87381,.T.);
#89587=ADVANCED_FACE('',(#7123),#87382,.T.);
#89588=ADVANCED_FACE('',(#7124),#87383,.F.);
#89589=ADVANCED_FACE('',(#7125),#87384,.F.);
#89590=ADVANCED_FACE('',(#7126),#87385,.F.);
#89591=ADVANCED_FACE('',(#7127,#5142),#5467,.T.);
#89592=ADVANCED_FACE('',(#7128),#4677,.F.);
#89593=ADVANCED_FACE('',(#7129),#87386,.F.);
#89594=ADVANCED_FACE('',(#7130,#5143),#5468,.T.);
#89595=ADVANCED_FACE('',(#7131),#4678,.F.);
#89596=ADVANCED_FACE('',(#7132),#4679,.T.);
#89597=ADVANCED_FACE('',(#7133),#5469,.T.);
#89598=ADVANCED_FACE('',(#7134),#5470,.T.);
#89599=ADVANCED_FACE('',(#7135),#5471,.F.);
#89600=ADVANCED_FACE('',(#7136),#87387,.F.);
#89601=ADVANCED_FACE('',(#7137),#5472,.F.);
#89602=ADVANCED_FACE('',(#7138),#5473,.F.);
#89603=ADVANCED_FACE('',(#7139),#87388,.F.);
#89604=ADVANCED_FACE('',(#7140),#5474,.F.);
#89605=ADVANCED_FACE('',(#7141),#138,.F.);
#89606=ADVANCED_FACE('',(#7142),#87389,.F.);
#89607=ADVANCED_FACE('',(#7143),#139,.F.);
#89608=ADVANCED_FACE('',(#7144),#87390,.F.);
#89609=ADVANCED_FACE('',(#7145),#5475,.F.);
#89610=ADVANCED_FACE('',(#7146),#87391,.F.);
#89611=ADVANCED_FACE('',(#7147),#5476,.F.);
#89612=ADVANCED_FACE('',(#7148),#4680,.F.);
#89613=ADVANCED_FACE('',(#7149),#5477,.F.);
#89614=ADVANCED_FACE('',(#7150),#87392,.F.);
#89615=ADVANCED_FACE('',(#7151),#5478,.F.);
#89616=ADVANCED_FACE('',(#7152),#4681,.F.);
#89617=ADVANCED_FACE('',(#7153),#5479,.F.);
#89618=ADVANCED_FACE('',(#7154),#5480,.F.);
#89619=ADVANCED_FACE('',(#7155),#87393,.T.);
#89620=ADVANCED_FACE('',(#7156),#5481,.F.);
#89621=ADVANCED_FACE('',(#7157),#5482,.F.);
#89622=ADVANCED_FACE('',(#7158),#87394,.F.);
#89623=ADVANCED_FACE('',(#7159),#5483,.T.);
#89624=ADVANCED_FACE('',(#7160),#5484,.F.);
#89625=ADVANCED_FACE('',(#7161),#87395,.T.);
#89626=ADVANCED_FACE('',(#7162,#5144),#5485,.T.);
#89627=ADVANCED_FACE('',(#7163),#87396,.F.);
#89628=ADVANCED_FACE('',(#7164),#4682,.T.);
#89629=ADVANCED_FACE('',(#7165),#5486,.F.);
#89630=ADVANCED_FACE('',(#7166),#87397,.F.);
#89631=ADVANCED_FACE('',(#7167),#5487,.F.);
#89632=ADVANCED_FACE('',(#7168),#87398,.T.);
#89633=ADVANCED_FACE('',(#7169),#87399,.F.);
#89634=ADVANCED_FACE('',(#7170),#5488,.T.);
#89635=ADVANCED_FACE('',(#7171),#87400,.F.);
#89636=ADVANCED_FACE('',(#7172),#87401,.T.);
#89637=ADVANCED_FACE('',(#7173),#87402,.F.);
#89638=ADVANCED_FACE('',(#7174),#5489,.F.);
#89639=ADVANCED_FACE('',(#7175),#87403,.T.);
#89640=ADVANCED_FACE('',(#7176),#5490,.F.);
#89641=ADVANCED_FACE('',(#7177),#87404,.T.);
#89642=ADVANCED_FACE('',(#7178),#87405,.F.);
#89643=ADVANCED_FACE('',(#7179),#5491,.F.);
#89644=ADVANCED_FACE('',(#7180),#87406,.F.);
#89645=ADVANCED_FACE('',(#7181),#5492,.F.);
#89646=ADVANCED_FACE('',(#7182),#87407,.F.);
#89647=ADVANCED_FACE('',(#7183),#87408,.T.);
#89648=ADVANCED_FACE('',(#7184),#87409,.T.);
#89649=ADVANCED_FACE('',(#7185),#87410,.T.);
#89650=ADVANCED_FACE('',(#7186,#5145),#5493,.T.);
#89651=ADVANCED_FACE('',(#7187,#5146,#5147,#5148),#5494,.T.);
#89652=ADVANCED_FACE('',(#7188),#87411,.F.);
#89653=ADVANCED_FACE('',(#7189),#87412,.F.);
#89654=ADVANCED_FACE('',(#7190),#4683,.T.);
#89655=ADVANCED_FACE('',(#7191),#87413,.T.);
#89656=ADVANCED_FACE('',(#7192),#87414,.T.);
#89657=ADVANCED_FACE('',(#7193),#87415,.F.);
#89658=ADVANCED_FACE('',(#7194),#87416,.T.);
#89659=ADVANCED_FACE('',(#7195),#87417,.F.);
#89660=ADVANCED_FACE('',(#7196),#87418,.T.);
#89661=ADVANCED_FACE('',(#7197),#87419,.F.);
#89662=ADVANCED_FACE('',(#7198),#87420,.T.);
#89663=ADVANCED_FACE('',(#7199),#4684,.F.);
#89664=ADVANCED_FACE('',(#7200,#5149),#5495,.T.);
#89665=ADVANCED_FACE('',(#7201),#87421,.F.);
#89666=ADVANCED_FACE('',(#7202),#4685,.F.);
#89667=ADVANCED_FACE('',(#7203),#87422,.F.);
#89668=ADVANCED_FACE('',(#7204),#87423,.T.);
#89669=ADVANCED_FACE('',(#7205),#87424,.F.);
#89670=ADVANCED_FACE('',(#7206),#87425,.F.);
#89671=ADVANCED_FACE('',(#7207),#4686,.F.);
#89672=ADVANCED_FACE('',(#7208),#87426,.F.);
#89673=ADVANCED_FACE('',(#7209),#87427,.T.);
#89674=ADVANCED_FACE('',(#7210),#87428,.F.);
#89675=ADVANCED_FACE('',(#7211),#87429,.T.);
#89676=ADVANCED_FACE('',(#7212),#87430,.T.);
#89677=ADVANCED_FACE('',(#7213),#5496,.T.);
#89678=ADVANCED_FACE('',(#7214),#87431,.T.);
#89679=ADVANCED_FACE('',(#7215),#87432,.F.);
#89680=ADVANCED_FACE('',(#7216),#87433,.F.);
#89681=ADVANCED_FACE('',(#7217),#5497,.T.);
#89682=ADVANCED_FACE('',(#7218),#87434,.F.);
#89683=ADVANCED_FACE('',(#7219),#87435,.F.);
#89684=ADVANCED_FACE('',(#7220),#4687,.F.);
#89685=ADVANCED_FACE('',(#7221),#4688,.F.);
#89686=ADVANCED_FACE('',(#7222),#87436,.F.);
#89687=ADVANCED_FACE('',(#7223,#5150),#5498,.T.);
#89688=ADVANCED_FACE('',(#7224,#5151),#5499,.T.);
#89689=ADVANCED_FACE('',(#7225),#87437,.F.);
#89690=ADVANCED_FACE('',(#7226),#87438,.F.);
#89691=ADVANCED_FACE('',(#7227),#5500,.F.);
#89692=ADVANCED_FACE('',(#7228),#5501,.T.);
#89693=ADVANCED_FACE('',(#7229),#4689,.T.);
#89694=ADVANCED_FACE('',(#7230),#87439,.F.);
#89695=ADVANCED_FACE('',(#7231),#87440,.F.);
#89696=ADVANCED_FACE('',(#7232,#5152),#5502,.T.);
#89697=ADVANCED_FACE('',(#7233),#4690,.F.);
#89698=ADVANCED_FACE('',(#7234,#5153),#5503,.T.);
#89699=ADVANCED_FACE('',(#7235),#4691,.F.);
#89700=ADVANCED_FACE('',(#7236),#4692,.T.);
#89701=ADVANCED_FACE('',(#7237),#4693,.T.);
#89702=ADVANCED_FACE('',(#7238),#4694,.T.);
#89703=ADVANCED_FACE('',(#7239,#5154),#5504,.T.);
#89704=ADVANCED_FACE('',(#7240),#87441,.F.);
#89705=ADVANCED_FACE('',(#7241),#87442,.T.);
#89706=ADVANCED_FACE('',(#7242),#87443,.T.);
#89707=ADVANCED_FACE('',(#7243),#4695,.T.);
#89708=ADVANCED_FACE('',(#7244),#4696,.T.);
#89709=ADVANCED_FACE('',(#7245),#87444,.T.);
#89710=ADVANCED_FACE('',(#7246),#5505,.F.);
#89711=ADVANCED_FACE('',(#7247),#87445,.F.);
#89712=ADVANCED_FACE('',(#7248),#5506,.T.);
#89713=ADVANCED_FACE('',(#7249),#5507,.T.);
#89714=ADVANCED_FACE('',(#7250),#87446,.T.);
#89715=ADVANCED_FACE('',(#7251),#1695,.F.);
#89716=ADVANCED_FACE('',(#7252),#87447,.T.);
#89717=ADVANCED_FACE('',(#7253),#87448,.F.);
#89718=ADVANCED_FACE('',(#7254),#140,.F.);
#89719=ADVANCED_FACE('',(#7255),#87449,.F.);
#89720=ADVANCED_FACE('',(#7256),#141,.F.);
#89721=ADVANCED_FACE('',(#7257),#87450,.F.);
#89722=ADVANCED_FACE('',(#7258),#6208,.T.);
#89723=ADVANCED_FACE('',(#7259),#1696,.F.);
#89724=ADVANCED_FACE('',(#7260),#87451,.F.);
#89725=ADVANCED_FACE('',(#7261),#87452,.T.);
#89726=ADVANCED_FACE('',(#7262),#87453,.F.);
#89727=ADVANCED_FACE('',(#7263),#87454,.T.);
#89728=ADVANCED_FACE('',(#7264),#4697,.T.);
#89729=ADVANCED_FACE('',(#7265),#87455,.F.);
#89730=ADVANCED_FACE('',(#7266),#6209,.T.);
#89731=ADVANCED_FACE('',(#7267),#1697,.F.);
#89732=ADVANCED_FACE('',(#7268),#5508,.F.);
#89733=ADVANCED_FACE('',(#7269),#87456,.F.);
#89734=ADVANCED_FACE('',(#7270),#87457,.T.);
#89735=ADVANCED_FACE('',(#7271),#87458,.F.);
#89736=ADVANCED_FACE('',(#7272,#5155),#5509,.T.);
#89737=ADVANCED_FACE('',(#7273),#87459,.T.);
#89738=ADVANCED_FACE('',(#7274),#87460,.F.);
#89739=ADVANCED_FACE('',(#7275),#5510,.F.);
#89740=ADVANCED_FACE('',(#7276),#87461,.T.);
#89741=ADVANCED_FACE('',(#7277),#4698,.F.);
#89742=ADVANCED_FACE('',(#7278,#5156),#5511,.F.);
#89743=ADVANCED_FACE('',(#7279),#87462,.F.);
#89744=ADVANCED_FACE('',(#7280),#87463,.F.);
#89745=ADVANCED_FACE('',(#7281),#5512,.T.);
#89746=ADVANCED_FACE('',(#7282),#87464,.F.);
#89747=ADVANCED_FACE('',(#7283),#5513,.F.);
#89748=ADVANCED_FACE('',(#7284),#87465,.F.);
#89749=ADVANCED_FACE('',(#7285),#5514,.F.);
#89750=ADVANCED_FACE('',(#7286),#87466,.T.);
#89751=ADVANCED_FACE('',(#7287),#5515,.F.);
#89752=ADVANCED_FACE('',(#7288),#87467,.T.);
#89753=ADVANCED_FACE('',(#7289),#5516,.F.);
#89754=ADVANCED_FACE('',(#7290),#5517,.T.);
#89755=ADVANCED_FACE('',(#7291),#87468,.T.);
#89756=ADVANCED_FACE('',(#7292),#87469,.F.);
#89757=ADVANCED_FACE('',(#7293),#87470,.F.);
#89758=ADVANCED_FACE('',(#7294,#5157),#5518,.T.);
#89759=ADVANCED_FACE('',(#7295),#87471,.T.);
#89760=ADVANCED_FACE('',(#7296),#87472,.F.);
#89761=ADVANCED_FACE('',(#7297),#87473,.T.);
#89762=ADVANCED_FACE('',(#7298),#87474,.F.);
#89763=ADVANCED_FACE('',(#7299),#5519,.T.);
#89764=ADVANCED_FACE('',(#7300),#4699,.F.);
#89765=ADVANCED_FACE('',(#7301),#5520,.F.);
#89766=ADVANCED_FACE('',(#7302),#5521,.T.);
#89767=ADVANCED_FACE('',(#7303),#87475,.F.);
#89768=ADVANCED_FACE('',(#7304),#87476,.F.);
#89769=ADVANCED_FACE('',(#7305),#5522,.F.);
#89770=ADVANCED_FACE('',(#7306),#5523,.F.);
#89771=ADVANCED_FACE('',(#7307),#5524,.F.);
#89772=ADVANCED_FACE('',(#7308),#5525,.F.);
#89773=ADVANCED_FACE('',(#7309),#5526,.F.);
#89774=ADVANCED_FACE('',(#7310),#87477,.T.);
#89775=ADVANCED_FACE('',(#7311),#87478,.T.);
#89776=ADVANCED_FACE('',(#7312),#87479,.T.);
#89777=ADVANCED_FACE('',(#7313),#87480,.T.);
#89778=ADVANCED_FACE('',(#7314),#87481,.T.);
#89779=ADVANCED_FACE('',(#7315),#87482,.T.);
#89780=ADVANCED_FACE('',(#7316),#5527,.F.);
#89781=ADVANCED_FACE('',(#7317),#87483,.T.);
#89782=ADVANCED_FACE('',(#7318),#87484,.T.);
#89783=ADVANCED_FACE('',(#7319),#5528,.F.);
#89784=ADVANCED_FACE('',(#7320),#6210,.F.);
#89785=ADVANCED_FACE('',(#7321),#6211,.F.);
#89786=ADVANCED_FACE('',(#7322),#6212,.F.);
#89787=ADVANCED_FACE('',(#7323),#6213,.F.);
#89788=ADVANCED_FACE('',(#7324),#5529,.F.);
#89789=ADVANCED_FACE('',(#7325),#6214,.F.);
#89790=ADVANCED_FACE('',(#7326),#87485,.T.);
#89791=ADVANCED_FACE('',(#7327),#87486,.F.);
#89792=ADVANCED_FACE('',(#7328),#87487,.F.);
#89793=ADVANCED_FACE('',(#7329),#5530,.F.);
#89794=ADVANCED_FACE('',(#7330),#87488,.F.);
#89795=ADVANCED_FACE('',(#7331),#87489,.T.);
#89796=ADVANCED_FACE('',(#7332),#87490,.F.);
#89797=ADVANCED_FACE('',(#7333),#87491,.T.);
#89798=ADVANCED_FACE('',(#7334),#5531,.T.);
#89799=ADVANCED_FACE('',(#7335),#87492,.T.);
#89800=ADVANCED_FACE('',(#7336),#87493,.F.);
#89801=ADVANCED_FACE('',(#7337),#5532,.F.);
#89802=ADVANCED_FACE('',(#7338),#87494,.F.);
#89803=ADVANCED_FACE('',(#7339),#5533,.T.);
#89804=ADVANCED_FACE('',(#7340),#87495,.F.);
#89805=ADVANCED_FACE('',(#7341),#87496,.T.);
#89806=ADVANCED_FACE('',(#7342),#87497,.T.);
#89807=ADVANCED_FACE('',(#7343),#5534,.F.);
#89808=ADVANCED_FACE('',(#7344),#87498,.T.);
#89809=ADVANCED_FACE('',(#7345,#5158),#5535,.T.);
#89810=ADVANCED_FACE('',(#7346),#5536,.T.);
#89811=ADVANCED_FACE('',(#7347),#87499,.F.);
#89812=ADVANCED_FACE('',(#7348),#4700,.T.);
#89813=ADVANCED_FACE('',(#7349),#4701,.T.);
#89814=ADVANCED_FACE('',(#7350),#5537,.T.);
#89815=ADVANCED_FACE('',(#7351),#5538,.T.);
#89816=ADVANCED_FACE('',(#7352),#5539,.F.);
#89817=ADVANCED_FACE('',(#7353),#87500,.F.);
#89818=ADVANCED_FACE('',(#7354),#5540,.F.);
#89819=ADVANCED_FACE('',(#7355),#87501,.F.);
#89820=ADVANCED_FACE('',(#7356),#5541,.T.);
#89821=ADVANCED_FACE('',(#7357),#87502,.F.);
#89822=ADVANCED_FACE('',(#7358,#5159,#5160,#5161),#5542,.T.);
#89823=ADVANCED_FACE('',(#7359),#87503,.F.);
#89824=ADVANCED_FACE('',(#7360),#5543,.T.);
#89825=ADVANCED_FACE('',(#7361),#5544,.F.);
#89826=ADVANCED_FACE('',(#7362),#5545,.T.);
#89827=ADVANCED_FACE('',(#7363),#5546,.T.);
#94626=CLOSED_SHELL('',(#89049,#89050,#89051,#89052,#89053,#89054,#89055,
#89056,#89057,#89058,#89059,#89060,#89061,#89062,#89063,#89064,#89065,#89066,
#89067,#89068,#89069,#89070,#89071,#89072,#89073,#89074,#89075,#89076,#89077,
#89078,#89079,#89080,#89081,#89082,#89083,#89084,#89085,#89086,#89087,#89088,
#89089,#89090,#89091,#89092,#89093,#89094,#89095,#89096,#89097,#89098,#89099,
#89100,#89101,#89102,#89103,#89104,#89105,#89106,#89107,#89108,#89109,#89110,
#89111,#89112,#89113,#89114,#89115,#89116,#89117,#89118,#89119,#89120,#89121,
#89122,#89123,#89124,#89125,#89126,#89127,#89128,#89129,#89130,#89131,#89132,
#89133,#89134,#89135,#89136,#89137,#89138,#89139,#89140,#89141,#89142,#89143,
#89144,#89145,#89146,#89147,#89148,#89149,#89150,#89151,#89152,#89153,#89154,
#89155,#89156,#89157,#89158,#89159,#89160,#89161,#89162,#89163,#89164,#89165,
#89166,#89167,#89168,#89169,#89170,#89171,#89172,#89173,#89174,#89175,#89176,
#89177,#89178,#89179,#89180,#89181,#89182,#89183,#89184,#89185,#89186,#89187,
#89188,#89189,#89190,#89191,#89192,#89193,#89194,#89195,#89196,#89197,#89198,
#89199,#89200,#89201,#89202,#89203,#89204,#89205,#89206,#89207,#89208,#89209,
#89210,#89211,#89212,#89213,#89214,#89215,#89216,#89217,#89218,#89219,#89220,
#89221,#89222,#89223,#89224,#89225,#89226,#89227,#89228,#89229,#89230,#89231,
#89232,#89233,#89234,#89235,#89236,#89237,#89238,#89239,#89240,#89241,#89242,
#89243,#89244,#89245,#89246,#89247,#89248,#89249,#89250,#89251,#89252,#89253,
#89254,#89255,#89256,#89257,#89258,#89259,#89260,#89261,#89262,#89263,#89264,
#89265,#89266,#89267,#89268,#89269,#89270,#89271,#89272,#89273,#89274,#89275,
#89276,#89277,#89278,#89279,#89280,#89281,#89282,#89283,#89284,#89285,#89286,
#89287,#89288,#89289,#89290,#89291,#89292,#89293,#89294,#89295,#89296,#89297,
#89298,#89299,#89300,#89301,#89302,#89303,#89304,#89305,#89306,#89307,#89308,
#89309,#89310,#89311,#89312,#89313,#89314,#89315,#89316,#89317,#89318,#89319,
#89320,#89321,#89322,#89323,#89324,#89325,#89326,#89327,#89328,#89329,#89330,
#89331,#89332,#89333,#89334,#89335,#89336,#89337,#89338,#89339,#89340,#89341,
#89342,#89343,#89344,#89345,#89346,#89347,#89348));
#94627=CLOSED_SHELL('',(#89349,#89350,#89351,#89352,#89353));
#94628=CLOSED_SHELL('',(#89354,#89355,#89356,#89357,#89358,#89359,#89360,
#89361,#89362,#89363,#89364,#89365,#89366,#89367,#89368,#89369,#89370,#89371,
#89372,#89373,#89374,#89375,#89376,#89377,#89378,#89379,#89380,#89381,#89382,
#89383,#89384,#89385,#89386,#89387,#89388,#89389,#89390,#89391,#89392,#89393,
#89394,#89395,#89396,#89397,#89398,#89399,#89400,#89401,#89402,#89403,#89404,
#89405,#89406,#89407,#89408,#89409,#89410,#89411,#89412,#89413,#89414,#89415,
#89416,#89417,#89418,#89419,#89420,#89421,#89422,#89423,#89424,#89425,#89426,
#89427,#89428,#89429,#89430,#89431,#89432,#89433,#89434,#89435,#89436,#89437,
#89438,#89439,#89440,#89441,#89442,#89443,#89444,#89445,#89446,#89447,#89448,
#89449,#89450,#89451,#89452,#89453,#89454,#89455,#89456,#89457,#89458,#89459,
#89460,#89461,#89462,#89463,#89464,#89465,#89466,#89467,#89468,#89469,#89470,
#89471,#89472,#89473,#89474,#89475,#89476,#89477,#89478,#89479,#89480,#89481,
#89482,#89483,#89484,#89485,#89486,#89487,#89488,#89489,#89490,#89491,#89492,
#89493,#89494,#89495,#89496,#89497,#89498,#89499,#89500,#89501,#89502,#89503,
#89504,#89505,#89506,#89507,#89508,#89509,#89510,#89511,#89512,#89513,#89514,
#89515,#89516,#89517,#89518,#89519,#89520,#89521,#89522,#89523,#89524,#89525,
#89526,#89527,#89528,#89529,#89530,#89531,#89532,#89533,#89534,#89535,#89536,
#89537,#89538,#89539,#89540,#89541,#89542,#89543,#89544,#89545,#89546,#89547,
#89548,#89549,#89550,#89551,#89552,#89553,#89554,#89555,#89556,#89557,#89558,
#89559,#89560,#89561,#89562,#89563,#89564,#89565,#89566,#89567,#89568,#89569,
#89570,#89571,#89572,#89573,#89574,#89575,#89576,#89577,#89578,#89579,#89580,
#89581,#89582,#89583,#89584,#89585,#89586,#89587,#89588,#89589,#89590,#89591,
#89592,#89593,#89594,#89595,#89596,#89597,#89598,#89599,#89600,#89601,#89602,
#89603,#89604,#89605,#89606,#89607,#89608,#89609,#89610,#89611,#89612,#89613,
#89614,#89615,#89616,#89617,#89618,#89619,#89620,#89621,#89622,#89623,#89624,
#89625,#89626,#89627,#89628,#89629,#89630,#89631,#89632,#89633,#89634,#89635,
#89636,#89637,#89638,#89639,#89640,#89641,#89642,#89643,#89644,#89645,#89646,
#89647,#89648,#89649,#89650,#89651,#89652,#89653,#89654,#89655,#89656,#89657,
#89658,#89659,#89660,#89661,#89662,#89663,#89664,#89665,#89666,#89667,#89668,
#89669,#89670,#89671,#89672,#89673,#89674,#89675,#89676,#89677,#89678,#89679,
#89680,#89681,#89682,#89683,#89684,#89685,#89686,#89687,#89688,#89689,#89690,
#89691,#89692,#89693,#89694,#89695,#89696,#89697,#89698,#89699,#89700,#89701,
#89702,#89703,#89704,#89705,#89706,#89707,#89708,#89709,#89710,#89711,#89712,
#89713,#89714,#89715,#89716,#89717,#89718,#89719,#89720,#89721,#89722,#89723,
#89724,#89725,#89726,#89727,#89728,#89729,#89730,#89731,#89732,#89733,#89734,
#89735,#89736,#89737,#89738,#89739,#89740,#89741,#89742,#89743,#89744,#89745,
#89746,#89747,#89748,#89749,#89750,#89751,#89752,#89753,#89754,#89755,#89756,
#89757,#89758,#89759,#89760,#89761,#89762,#89763,#89764,#89765,#89766,#89767,
#89768,#89769,#89770,#89771,#89772,#89773,#89774,#89775,#89776,#89777,#89778,
#89779,#89780,#89781,#89782,#89783,#89784,#89785,#89786,#89787,#89788,#89789,
#89790,#89791,#89792,#89793,#89794,#89795,#89796,#89797,#89798,#89799,#89800,
#89801,#89802,#89803,#89804,#89805,#89806,#89807,#89808,#89809,#89810,#89811,
#89812,#89813,#89814,#89815,#89816,#89817,#89818,#89819,#89820,#89821,#89822,
#89823,#89824,#89825,#89826,#89827));
#95341=AXIS2_PLACEMENT_3D('',#138715,#106742,#106743);
#95342=AXIS2_PLACEMENT_3D('',#138716,#106744,#106745);
#95343=AXIS2_PLACEMENT_3D('',#138719,#106746,#106747);
#95344=AXIS2_PLACEMENT_3D('',#138723,#106749,#106750);
#95345=AXIS2_PLACEMENT_3D('',#138742,#106752,#106753);
#95346=AXIS2_PLACEMENT_3D('',#138743,#106754,#106755);
#95347=AXIS2_PLACEMENT_3D('',#138744,#106756,#106757);
#95348=AXIS2_PLACEMENT_3D('',#138745,#106758,#106759);
#95349=AXIS2_PLACEMENT_3D('',#138748,#106760,#106761);
#95350=AXIS2_PLACEMENT_3D('',#138749,#106762,#106763);
#95351=AXIS2_PLACEMENT_3D('',#138750,#106764,#106765);
#95352=AXIS2_PLACEMENT_3D('',#138768,#106766,#106767);
#95353=AXIS2_PLACEMENT_3D('',#138769,#106768,#106769);
#95354=AXIS2_PLACEMENT_3D('',#138770,#106770,#106771);
#95355=AXIS2_PLACEMENT_3D('',#138771,#106772,#106773);
#95356=AXIS2_PLACEMENT_3D('',#138774,#106774,#106775);
#95357=AXIS2_PLACEMENT_3D('',#138775,#106776,#106777);
#95358=AXIS2_PLACEMENT_3D('',#138776,#106778,#106779);
#95359=AXIS2_PLACEMENT_3D('',#138794,#106780,#106781);
#95360=AXIS2_PLACEMENT_3D('',#138795,#106782,#106783);
#95361=AXIS2_PLACEMENT_3D('',#138796,#106784,#106785);
#95362=AXIS2_PLACEMENT_3D('',#138797,#106786,#106787);
#95363=AXIS2_PLACEMENT_3D('',#138800,#106788,#106789);
#95364=AXIS2_PLACEMENT_3D('',#138801,#106790,#106791);
#95365=AXIS2_PLACEMENT_3D('',#138802,#106792,#106793);
#95366=AXIS2_PLACEMENT_3D('',#138814,#106794,#106795);
#95367=AXIS2_PLACEMENT_3D('',#138815,#106796,#106797);
#95368=AXIS2_PLACEMENT_3D('',#138816,#106798,#106799);
#95369=AXIS2_PLACEMENT_3D('',#138817,#106800,#106801);
#95370=AXIS2_PLACEMENT_3D('',#138820,#106802,#106803);
#95371=AXIS2_PLACEMENT_3D('',#138832,#106806,#106807);
#95372=AXIS2_PLACEMENT_3D('',#138833,#106808,#106809);
#95373=AXIS2_PLACEMENT_3D('',#138834,#106810,#106811);
#95374=AXIS2_PLACEMENT_3D('',#138838,#106813,#106814);
#95375=AXIS2_PLACEMENT_3D('',#138842,#106816,#106817);
#95376=AXIS2_PLACEMENT_3D('',#138856,#106820,#106821);
#95377=AXIS2_PLACEMENT_3D('',#138858,#106823,#106824);
#95378=AXIS2_PLACEMENT_3D('',#138861,#106826,#106827);
#95379=AXIS2_PLACEMENT_3D('',#138862,#106828,#106829);
#95380=AXIS2_PLACEMENT_3D('',#138866,#106832,#106833);
#95381=AXIS2_PLACEMENT_3D('',#138869,#106835,#106836);
#95382=AXIS2_PLACEMENT_3D('',#138870,#106837,#106838);
#95383=AXIS2_PLACEMENT_3D('',#138874,#106841,#106842);
#95384=AXIS2_PLACEMENT_3D('',#138875,#106843,#106844);
#95385=AXIS2_PLACEMENT_3D('',#138878,#106845,#106846);
#95386=AXIS2_PLACEMENT_3D('',#138882,#106848,#106849);
#95387=AXIS2_PLACEMENT_3D('',#138895,#106851,#106852);
#95388=AXIS2_PLACEMENT_3D('',#138896,#106853,#106854);
#95389=AXIS2_PLACEMENT_3D('',#138897,#106855,#106856);
#95390=AXIS2_PLACEMENT_3D('',#138898,#106857,#106858);
#95391=AXIS2_PLACEMENT_3D('',#138901,#106859,#106860);
#95392=AXIS2_PLACEMENT_3D('',#138902,#106861,#106862);
#95393=AXIS2_PLACEMENT_3D('',#138903,#106863,#106864);
#95394=AXIS2_PLACEMENT_3D('',#138921,#106865,#106866);
#95395=AXIS2_PLACEMENT_3D('',#138922,#106867,#106868);
#95396=AXIS2_PLACEMENT_3D('',#138923,#106869,#106870);
#95397=AXIS2_PLACEMENT_3D('',#138924,#106871,#106872);
#95398=AXIS2_PLACEMENT_3D('',#138927,#106873,#106874);
#95399=AXIS2_PLACEMENT_3D('',#138941,#106877,#106878);
#95400=AXIS2_PLACEMENT_3D('',#138942,#106879,#106880);
#95401=AXIS2_PLACEMENT_3D('',#138943,#106881,#106882);
#95402=AXIS2_PLACEMENT_3D('',#138944,#106883,#106884);
#95403=AXIS2_PLACEMENT_3D('',#138947,#106885,#106886);
#95404=AXIS2_PLACEMENT_3D('',#138950,#106889,#106890);
#95405=AXIS2_PLACEMENT_3D('',#138953,#106891,#106892);
#95406=AXIS2_PLACEMENT_3D('',#138954,#106893,#106894);
#95407=AXIS2_PLACEMENT_3D('',#138955,#106895,#106896);
#95408=AXIS2_PLACEMENT_3D('',#138956,#106897,#106898);
#95409=AXIS2_PLACEMENT_3D('',#138959,#106899,#106900);
#95410=AXIS2_PLACEMENT_3D('',#138979,#106903,#106904);
#95411=AXIS2_PLACEMENT_3D('',#138980,#106905,#106906);
#95412=AXIS2_PLACEMENT_3D('',#138981,#106907,#106908);
#95413=AXIS2_PLACEMENT_3D('',#138982,#106909,#106910);
#95414=AXIS2_PLACEMENT_3D('',#138985,#106911,#106912);
#95415=AXIS2_PLACEMENT_3D('',#138986,#106913,#106914);
#95416=AXIS2_PLACEMENT_3D('',#138987,#106915,#106916);
#95417=AXIS2_PLACEMENT_3D('',#138999,#106917,#106918);
#95418=AXIS2_PLACEMENT_3D('',#139000,#106919,#106920);
#95419=AXIS2_PLACEMENT_3D('',#139001,#106921,#106922);
#95420=AXIS2_PLACEMENT_3D('',#139002,#106923,#106924);
#95421=AXIS2_PLACEMENT_3D('',#139005,#106925,#106926);
#95422=AXIS2_PLACEMENT_3D('',#139007,#106927,#106928);
#95423=AXIS2_PLACEMENT_3D('',#139008,#106929,#106930);
#95424=AXIS2_PLACEMENT_3D('',#139009,#106931,#106932);
#95425=AXIS2_PLACEMENT_3D('',#139019,#106933,#106934);
#95426=AXIS2_PLACEMENT_3D('',#139020,#106935,#106936);
#95427=AXIS2_PLACEMENT_3D('',#139021,#106937,#106938);
#95428=AXIS2_PLACEMENT_3D('',#139027,#106942,#106943);
#95429=AXIS2_PLACEMENT_3D('',#139030,#106945,#106946);
#95430=AXIS2_PLACEMENT_3D('',#139031,#106947,#106948);
#95431=AXIS2_PLACEMENT_3D('',#139034,#106950,#106951);
#95432=AXIS2_PLACEMENT_3D('',#139035,#106952,#106953);
#95433=AXIS2_PLACEMENT_3D('',#139038,#106955,#106956);
#95434=AXIS2_PLACEMENT_3D('',#139039,#106957,#106958);
#95435=AXIS2_PLACEMENT_3D('',#139041,#106959,#106960);
#95436=AXIS2_PLACEMENT_3D('',#139046,#106963,#106964);
#95437=AXIS2_PLACEMENT_3D('',#139050,#106966,#106967);
#95438=AXIS2_PLACEMENT_3D('',#139054,#106969,#106970);
#95439=AXIS2_PLACEMENT_3D('',#139058,#106972,#106973);
#95440=AXIS2_PLACEMENT_3D('',#139061,#106975,#106976);
#95441=AXIS2_PLACEMENT_3D('',#139062,#106977,#106978);
#95442=AXIS2_PLACEMENT_3D('',#139065,#106980,#106981);
#95443=AXIS2_PLACEMENT_3D('',#139066,#106982,#106983);
#95444=AXIS2_PLACEMENT_3D('',#139070,#106986,#106987);
#95445=AXIS2_PLACEMENT_3D('',#139071,#106988,#106989);
#95446=AXIS2_PLACEMENT_3D('',#139074,#106990,#106991);
#95447=AXIS2_PLACEMENT_3D('',#139076,#106992,#106993);
#95448=AXIS2_PLACEMENT_3D('',#139078,#106994,#106995);
#95449=AXIS2_PLACEMENT_3D('',#139079,#106996,#106997);
#95450=AXIS2_PLACEMENT_3D('',#139091,#106998,#106999);
#95451=AXIS2_PLACEMENT_3D('',#139092,#107000,#107001);
#95452=AXIS2_PLACEMENT_3D('',#139093,#107002,#107003);
#95453=AXIS2_PLACEMENT_3D('',#139094,#107004,#107005);
#95454=AXIS2_PLACEMENT_3D('',#139097,#107006,#107007);
#95455=AXIS2_PLACEMENT_3D('',#139117,#107010,#107011);
#95456=AXIS2_PLACEMENT_3D('',#139118,#107012,#107013);
#95457=AXIS2_PLACEMENT_3D('',#139119,#107014,#107015);
#95458=AXIS2_PLACEMENT_3D('',#139120,#107016,#107017);
#95459=AXIS2_PLACEMENT_3D('',#139123,#107018,#107019);
#95460=AXIS2_PLACEMENT_3D('',#139143,#107022,#107023);
#95461=AXIS2_PLACEMENT_3D('',#139144,#107024,#107025);
#95462=AXIS2_PLACEMENT_3D('',#139145,#107026,#107027);
#95463=AXIS2_PLACEMENT_3D('',#139146,#107028,#107029);
#95464=AXIS2_PLACEMENT_3D('',#139149,#107030,#107031);
#95465=AXIS2_PLACEMENT_3D('',#139150,#107032,#107033);
#95466=AXIS2_PLACEMENT_3D('',#139151,#107034,#107035);
#95467=AXIS2_PLACEMENT_3D('',#139163,#107036,#107037);
#95468=AXIS2_PLACEMENT_3D('',#139164,#107038,#107039);
#95469=AXIS2_PLACEMENT_3D('',#139165,#107040,#107041);
#95470=AXIS2_PLACEMENT_3D('',#139166,#107042,#107043);
#95471=AXIS2_PLACEMENT_3D('',#139169,#107044,#107045);
#95472=AXIS2_PLACEMENT_3D('',#139182,#107048,#107049);
#95473=AXIS2_PLACEMENT_3D('',#139183,#107050,#107051);
#95474=AXIS2_PLACEMENT_3D('',#139184,#107052,#107053);
#95475=AXIS2_PLACEMENT_3D('',#139185,#107054,#107055);
#95476=AXIS2_PLACEMENT_3D('',#139187,#107056,#107057);
#95477=AXIS2_PLACEMENT_3D('',#139188,#107058,#107059);
#95478=AXIS2_PLACEMENT_3D('',#139198,#107060,#107061);
#95479=AXIS2_PLACEMENT_3D('',#139199,#107062,#107063);
#95480=AXIS2_PLACEMENT_3D('',#139200,#107064,#107065);
#95481=AXIS2_PLACEMENT_3D('',#139204,#107067,#107068);
#95482=AXIS2_PLACEMENT_3D('',#139208,#107070,#107071);
#95483=AXIS2_PLACEMENT_3D('',#139210,#107073,#107074);
#95484=AXIS2_PLACEMENT_3D('',#139214,#107077,#107078);
#95485=AXIS2_PLACEMENT_3D('',#139215,#107079,#107080);
#95486=AXIS2_PLACEMENT_3D('',#139216,#107081,#107082);
#95487=AXIS2_PLACEMENT_3D('',#139219,#107084,#107085);
#95488=AXIS2_PLACEMENT_3D('',#139220,#107086,#107087);
#95489=AXIS2_PLACEMENT_3D('',#139223,#107089,#107090);
#95490=AXIS2_PLACEMENT_3D('',#139224,#107091,#107092);
#95491=AXIS2_PLACEMENT_3D('',#139225,#107093,#107094);
#95492=AXIS2_PLACEMENT_3D('',#139228,#107095,#107096);
#95493=AXIS2_PLACEMENT_3D('',#139232,#107098,#107099);
#95494=AXIS2_PLACEMENT_3D('',#139245,#107101,#107102);
#95495=AXIS2_PLACEMENT_3D('',#139246,#107103,#107104);
#95496=AXIS2_PLACEMENT_3D('',#139247,#107105,#107106);
#95497=AXIS2_PLACEMENT_3D('',#139248,#107107,#107108);
#95498=AXIS2_PLACEMENT_3D('',#139251,#107109,#107110);
#95499=AXIS2_PLACEMENT_3D('',#139252,#107111,#107112);
#95500=AXIS2_PLACEMENT_3D('',#139253,#107113,#107114);
#95501=AXIS2_PLACEMENT_3D('',#139265,#107115,#107116);
#95502=AXIS2_PLACEMENT_3D('',#139266,#107117,#107118);
#95503=AXIS2_PLACEMENT_3D('',#139267,#107119,#107120);
#95504=AXIS2_PLACEMENT_3D('',#139268,#107121,#107122);
#95505=AXIS2_PLACEMENT_3D('',#139271,#107123,#107124);
#95506=AXIS2_PLACEMENT_3D('',#139272,#107125,#107126);
#95507=AXIS2_PLACEMENT_3D('',#139273,#107127,#107128);
#95508=AXIS2_PLACEMENT_3D('',#139274,#107129,#107130);
#95509=AXIS2_PLACEMENT_3D('',#139277,#107131,#107132);
#95510=AXIS2_PLACEMENT_3D('',#139278,#107133,#107134);
#95511=AXIS2_PLACEMENT_3D('',#139279,#107135,#107136);
#95512=AXIS2_PLACEMENT_3D('',#139280,#107137,#107138);
#95513=AXIS2_PLACEMENT_3D('',#139283,#107139,#107140);
#95514=AXIS2_PLACEMENT_3D('',#139286,#107143,#107144);
#95515=AXIS2_PLACEMENT_3D('',#139289,#107145,#107146);
#95516=AXIS2_PLACEMENT_3D('',#139290,#107147,#107148);
#95517=AXIS2_PLACEMENT_3D('',#139291,#107149,#107150);
#95518=AXIS2_PLACEMENT_3D('',#139309,#107151,#107152);
#95519=AXIS2_PLACEMENT_3D('',#139310,#107153,#107154);
#95520=AXIS2_PLACEMENT_3D('',#139311,#107155,#107156);
#95521=AXIS2_PLACEMENT_3D('',#139312,#107157,#107158);
#95522=AXIS2_PLACEMENT_3D('',#139315,#107159,#107160);
#95523=AXIS2_PLACEMENT_3D('',#139327,#107163,#107164);
#95524=AXIS2_PLACEMENT_3D('',#139328,#107165,#107166);
#95525=AXIS2_PLACEMENT_3D('',#139329,#107167,#107168);
#95526=AXIS2_PLACEMENT_3D('',#139339,#107174,#107175);
#95527=AXIS2_PLACEMENT_3D('',#139342,#107177,#107178);
#95528=AXIS2_PLACEMENT_3D('',#139343,#107179,#107180);
#95529=AXIS2_PLACEMENT_3D('',#139346,#107182,#107183);
#95530=AXIS2_PLACEMENT_3D('',#139347,#107184,#107185);
#95531=AXIS2_PLACEMENT_3D('',#139351,#107188,#107189);
#95532=AXIS2_PLACEMENT_3D('',#139354,#107191,#107192);
#95533=AXIS2_PLACEMENT_3D('',#139355,#107193,#107194);
#95534=AXIS2_PLACEMENT_3D('',#139363,#107199,#107200);
#95535=AXIS2_PLACEMENT_3D('',#139364,#107201,#107202);
#95536=AXIS2_PLACEMENT_3D('',#139367,#107203,#107204);
#95537=AXIS2_PLACEMENT_3D('',#139369,#107205,#107206);
#95538=AXIS2_PLACEMENT_3D('',#139371,#107207,#107208);
#95539=AXIS2_PLACEMENT_3D('',#139372,#107209,#107210);
#95540=AXIS2_PLACEMENT_3D('',#139390,#107211,#107212);
#95541=AXIS2_PLACEMENT_3D('',#139391,#107213,#107214);
#95542=AXIS2_PLACEMENT_3D('',#139392,#107215,#107216);
#95543=AXIS2_PLACEMENT_3D('',#139393,#107217,#107218);
#95544=AXIS2_PLACEMENT_3D('',#139396,#107219,#107220);
#95545=AXIS2_PLACEMENT_3D('',#139397,#107221,#107222);
#95546=AXIS2_PLACEMENT_3D('',#139398,#107223,#107224);
#95547=AXIS2_PLACEMENT_3D('',#139399,#107225,#107226);
#95548=AXIS2_PLACEMENT_3D('',#139402,#107227,#107228);
#95549=AXIS2_PLACEMENT_3D('',#139403,#107229,#107230);
#95550=AXIS2_PLACEMENT_3D('',#139404,#107231,#107232);
#95551=AXIS2_PLACEMENT_3D('',#139422,#107233,#107234);
#95552=AXIS2_PLACEMENT_3D('',#139423,#107235,#107236);
#95553=AXIS2_PLACEMENT_3D('',#139424,#107237,#107238);
#95554=AXIS2_PLACEMENT_3D('',#139425,#107239,#107240);
#95555=AXIS2_PLACEMENT_3D('',#139428,#107241,#107242);
#95556=AXIS2_PLACEMENT_3D('',#139431,#107245,#107246);
#95557=AXIS2_PLACEMENT_3D('',#139434,#107247,#107248);
#95558=AXIS2_PLACEMENT_3D('',#139435,#107249,#107250);
#95559=AXIS2_PLACEMENT_3D('',#139436,#107251,#107252);
#95560=AXIS2_PLACEMENT_3D('',#139437,#107253,#107254);
#95561=AXIS2_PLACEMENT_3D('',#139440,#107255,#107256);
#95562=AXIS2_PLACEMENT_3D('',#139454,#107259,#107260);
#95563=AXIS2_PLACEMENT_3D('',#139455,#107261,#107262);
#95564=AXIS2_PLACEMENT_3D('',#139456,#107263,#107264);
#95565=AXIS2_PLACEMENT_3D('',#139457,#107265,#107266);
#95566=AXIS2_PLACEMENT_3D('',#139460,#107267,#107268);
#95567=AXIS2_PLACEMENT_3D('',#139480,#107271,#107272);
#95568=AXIS2_PLACEMENT_3D('',#139481,#107273,#107274);
#95569=AXIS2_PLACEMENT_3D('',#139482,#107275,#107276);
#95570=AXIS2_PLACEMENT_3D('',#139483,#107277,#107278);
#95571=AXIS2_PLACEMENT_3D('',#139486,#107279,#107280);
#95572=AXIS2_PLACEMENT_3D('',#139487,#107281,#107282);
#95573=AXIS2_PLACEMENT_3D('',#139488,#107283,#107284);
#95574=AXIS2_PLACEMENT_3D('',#139506,#107285,#107286);
#95575=AXIS2_PLACEMENT_3D('',#139507,#107287,#107288);
#95576=AXIS2_PLACEMENT_3D('',#139508,#107289,#107290);
#95577=AXIS2_PLACEMENT_3D('',#139509,#107291,#107292);
#95578=AXIS2_PLACEMENT_3D('',#139512,#107295,#107296);
#95579=AXIS2_PLACEMENT_3D('',#139516,#107298,#107299);
#95580=AXIS2_PLACEMENT_3D('',#139518,#107301,#107302);
#95581=AXIS2_PLACEMENT_3D('',#139522,#107305,#107306);
#95582=AXIS2_PLACEMENT_3D('',#139525,#107308,#107309);
#95583=AXIS2_PLACEMENT_3D('',#139526,#107310,#107311);
#95584=AXIS2_PLACEMENT_3D('',#139529,#107313,#107314);
#95585=AXIS2_PLACEMENT_3D('',#139530,#107315,#107316);
#95586=AXIS2_PLACEMENT_3D('',#139533,#107318,#107319);
#95587=AXIS2_PLACEMENT_3D('',#139534,#107320,#107321);
#95588=AXIS2_PLACEMENT_3D('',#139538,#107324,#107325);
#95589=AXIS2_PLACEMENT_3D('',#139541,#107327,#107328);
#95590=AXIS2_PLACEMENT_3D('',#139542,#107329,#107330);
#95591=AXIS2_PLACEMENT_3D('',#139543,#107331,#107332);
#95592=AXIS2_PLACEMENT_3D('',#139546,#107333,#107334);
#95593=AXIS2_PLACEMENT_3D('',#139548,#107335,#107336);
#95594=AXIS2_PLACEMENT_3D('',#139550,#107337,#107338);
#95595=AXIS2_PLACEMENT_3D('',#139551,#107339,#107340);
#95596=AXIS2_PLACEMENT_3D('',#139552,#107341,#107342);
#95597=AXIS2_PLACEMENT_3D('',#139555,#107343,#107344);
#95598=AXIS2_PLACEMENT_3D('',#139556,#107345,#107346);
#95599=AXIS2_PLACEMENT_3D('',#139557,#107347,#107348);
#95600=AXIS2_PLACEMENT_3D('',#139575,#107349,#107350);
#95601=AXIS2_PLACEMENT_3D('',#139576,#107351,#107352);
#95602=AXIS2_PLACEMENT_3D('',#139577,#107353,#107354);
#95603=AXIS2_PLACEMENT_3D('',#139578,#107355,#107356);
#95604=AXIS2_PLACEMENT_3D('',#139581,#107357,#107358);
#95605=AXIS2_PLACEMENT_3D('',#139582,#107359,#107360);
#95606=AXIS2_PLACEMENT_3D('',#139583,#107361,#107362);
#95607=AXIS2_PLACEMENT_3D('',#139595,#107363,#107364);
#95608=AXIS2_PLACEMENT_3D('',#139596,#107365,#107366);
#95609=AXIS2_PLACEMENT_3D('',#139597,#107367,#107368);
#95610=AXIS2_PLACEMENT_3D('',#139598,#107369,#107370);
#95611=AXIS2_PLACEMENT_3D('',#139601,#107371,#107372);
#95612=AXIS2_PLACEMENT_3D('',#139602,#107373,#107374);
#95613=AXIS2_PLACEMENT_3D('',#139603,#107375,#107376);
#95614=AXIS2_PLACEMENT_3D('',#139621,#107377,#107378);
#95615=AXIS2_PLACEMENT_3D('',#139622,#107379,#107380);
#95616=AXIS2_PLACEMENT_3D('',#139623,#107381,#107382);
#95617=AXIS2_PLACEMENT_3D('',#139624,#107383,#107384);
#95618=AXIS2_PLACEMENT_3D('',#139627,#107385,#107386);
#95619=AXIS2_PLACEMENT_3D('',#139639,#107389,#107390);
#95620=AXIS2_PLACEMENT_3D('',#139640,#107391,#107392);
#95621=AXIS2_PLACEMENT_3D('',#139641,#107393,#107394);
#95622=AXIS2_PLACEMENT_3D('',#139645,#107396,#107397);
#95623=AXIS2_PLACEMENT_3D('',#139647,#107399,#107400);
#95624=AXIS2_PLACEMENT_3D('',#139650,#107402,#107403);
#95625=AXIS2_PLACEMENT_3D('',#139651,#107404,#107405);
#95626=AXIS2_PLACEMENT_3D('',#139655,#107408,#107409);
#95627=AXIS2_PLACEMENT_3D('',#139658,#107411,#107412);
#95628=AXIS2_PLACEMENT_3D('',#139659,#107413,#107414);
#95629=AXIS2_PLACEMENT_3D('',#139662,#107416,#107417);
#95630=AXIS2_PLACEMENT_3D('',#139663,#107418,#107419);
#95631=AXIS2_PLACEMENT_3D('',#139664,#107420,#107421);
#95632=AXIS2_PLACEMENT_3D('',#139667,#107422,#107423);
#95633=AXIS2_PLACEMENT_3D('',#139669,#107424,#107425);
#95634=AXIS2_PLACEMENT_3D('',#139671,#107426,#107427);
#95635=AXIS2_PLACEMENT_3D('',#139672,#107428,#107429);
#95636=AXIS2_PLACEMENT_3D('',#139684,#107430,#107431);
#95637=AXIS2_PLACEMENT_3D('',#139685,#107432,#107433);
#95638=AXIS2_PLACEMENT_3D('',#139686,#107434,#107435);
#95639=AXIS2_PLACEMENT_3D('',#139687,#107436,#107437);
#95640=AXIS2_PLACEMENT_3D('',#139690,#107438,#107439);
#95641=AXIS2_PLACEMENT_3D('',#139691,#107440,#107441);
#95642=AXIS2_PLACEMENT_3D('',#139692,#107442,#107443);
#95643=AXIS2_PLACEMENT_3D('',#139693,#107444,#107445);
#95644=AXIS2_PLACEMENT_3D('',#139696,#107446,#107447);
#95645=AXIS2_PLACEMENT_3D('',#139697,#107448,#107449);
#95646=AXIS2_PLACEMENT_3D('',#139698,#107450,#107451);
#95647=AXIS2_PLACEMENT_3D('',#139699,#107452,#107453);
#95648=AXIS2_PLACEMENT_3D('',#139702,#107454,#107455);
#95649=AXIS2_PLACEMENT_3D('',#139703,#107456,#107457);
#95650=AXIS2_PLACEMENT_3D('',#139704,#107458,#107459);
#95651=AXIS2_PLACEMENT_3D('',#139716,#107460,#107461);
#95652=AXIS2_PLACEMENT_3D('',#139717,#107462,#107463);
#95653=AXIS2_PLACEMENT_3D('',#139718,#107464,#107465);
#95654=AXIS2_PLACEMENT_3D('',#139719,#107466,#107467);
#95655=AXIS2_PLACEMENT_3D('',#139722,#107468,#107469);
#95656=AXIS2_PLACEMENT_3D('',#139742,#107472,#107473);
#95657=AXIS2_PLACEMENT_3D('',#139743,#107474,#107475);
#95658=AXIS2_PLACEMENT_3D('',#139744,#107476,#107477);
#95659=AXIS2_PLACEMENT_3D('',#139745,#107478,#107479);
#95660=AXIS2_PLACEMENT_3D('',#139748,#107480,#107481);
#95661=AXIS2_PLACEMENT_3D('',#139762,#107484,#107485);
#95662=AXIS2_PLACEMENT_3D('',#139763,#107486,#107487);
#95663=AXIS2_PLACEMENT_3D('',#139764,#107488,#107489);
#95664=AXIS2_PLACEMENT_3D('',#139765,#107490,#107491);
#95665=AXIS2_PLACEMENT_3D('',#139768,#107492,#107493);
#95666=AXIS2_PLACEMENT_3D('',#139782,#107496,#107497);
#95667=AXIS2_PLACEMENT_3D('',#139783,#107498,#107499);
#95668=AXIS2_PLACEMENT_3D('',#139784,#107500,#107501);
#95669=AXIS2_PLACEMENT_3D('',#139785,#107502,#107503);
#95670=AXIS2_PLACEMENT_3D('',#139788,#107504,#107505);
#95671=AXIS2_PLACEMENT_3D('',#139789,#107506,#107507);
#95672=AXIS2_PLACEMENT_3D('',#139790,#107508,#107509);
#95673=AXIS2_PLACEMENT_3D('',#139802,#107510,#107511);
#95674=AXIS2_PLACEMENT_3D('',#139803,#107512,#107513);
#95675=AXIS2_PLACEMENT_3D('',#139804,#107514,#107515);
#95676=AXIS2_PLACEMENT_3D('',#139805,#107516,#107517);
#95677=AXIS2_PLACEMENT_3D('',#139808,#107518,#107519);
#95678=AXIS2_PLACEMENT_3D('',#139809,#107520,#107521);
#95679=AXIS2_PLACEMENT_3D('',#139810,#107522,#107523);
#95680=AXIS2_PLACEMENT_3D('',#139826,#107524,#107525);
#95681=AXIS2_PLACEMENT_3D('',#139827,#107526,#107527);
#95682=AXIS2_PLACEMENT_3D('',#139828,#107528,#107529);
#95683=AXIS2_PLACEMENT_3D('',#139832,#107531,#107532);
#95684=AXIS2_PLACEMENT_3D('',#139834,#107534,#107535);
#95685=AXIS2_PLACEMENT_3D('',#139838,#107538,#107539);
#95686=AXIS2_PLACEMENT_3D('',#139841,#107541,#107542);
#95687=AXIS2_PLACEMENT_3D('',#139842,#107543,#107544);
#95688=AXIS2_PLACEMENT_3D('',#139845,#107546,#107547);
#95689=AXIS2_PLACEMENT_3D('',#139846,#107548,#107549);
#95690=AXIS2_PLACEMENT_3D('',#139849,#107551,#107552);
#95691=AXIS2_PLACEMENT_3D('',#139850,#107553,#107554);
#95692=AXIS2_PLACEMENT_3D('',#139853,#107556,#107557);
#95693=AXIS2_PLACEMENT_3D('',#139854,#107558,#107559);
#95694=AXIS2_PLACEMENT_3D('',#139857,#107561,#107562);
#95695=AXIS2_PLACEMENT_3D('',#139858,#107563,#107564);
#95696=AXIS2_PLACEMENT_3D('',#139862,#107566,#107567);
#95697=AXIS2_PLACEMENT_3D('',#139865,#107569,#107570);
#95698=AXIS2_PLACEMENT_3D('',#139866,#107571,#107572);
#95699=AXIS2_PLACEMENT_3D('',#139867,#107573,#107574);
#95700=AXIS2_PLACEMENT_3D('',#139870,#107575,#107576);
#95701=AXIS2_PLACEMENT_3D('',#139872,#107577,#107578);
#95702=AXIS2_PLACEMENT_3D('',#139874,#107579,#107580);
#95703=AXIS2_PLACEMENT_3D('',#139875,#107581,#107582);
#95704=AXIS2_PLACEMENT_3D('',#139893,#107583,#107584);
#95705=AXIS2_PLACEMENT_3D('',#139894,#107585,#107586);
#95706=AXIS2_PLACEMENT_3D('',#139895,#107587,#107588);
#95707=AXIS2_PLACEMENT_3D('',#139896,#107589,#107590);
#95708=AXIS2_PLACEMENT_3D('',#139899,#107591,#107592);
#95709=AXIS2_PLACEMENT_3D('',#139900,#107593,#107594);
#95710=AXIS2_PLACEMENT_3D('',#139901,#107595,#107596);
#95711=AXIS2_PLACEMENT_3D('',#139902,#107597,#107598);
#95712=AXIS2_PLACEMENT_3D('',#139905,#107599,#107600);
#95713=AXIS2_PLACEMENT_3D('',#139919,#107603,#107604);
#95714=AXIS2_PLACEMENT_3D('',#139920,#107605,#107606);
#95715=AXIS2_PLACEMENT_3D('',#139921,#107607,#107608);
#95716=AXIS2_PLACEMENT_3D('',#139922,#107609,#107610);
#95717=AXIS2_PLACEMENT_3D('',#139925,#107611,#107612);
#95718=AXIS2_PLACEMENT_3D('',#139926,#107613,#107614);
#95719=AXIS2_PLACEMENT_3D('',#139927,#107615,#107616);
#95720=AXIS2_PLACEMENT_3D('',#139945,#107617,#107618);
#95721=AXIS2_PLACEMENT_3D('',#139946,#107619,#107620);
#95722=AXIS2_PLACEMENT_3D('',#139947,#107621,#107622);
#95723=AXIS2_PLACEMENT_3D('',#139948,#107623,#107624);
#95724=AXIS2_PLACEMENT_3D('',#139951,#107625,#107626);
#95725=AXIS2_PLACEMENT_3D('',#139952,#107627,#107628);
#95726=AXIS2_PLACEMENT_3D('',#139953,#107629,#107630);
#95727=AXIS2_PLACEMENT_3D('',#139969,#107631,#107632);
#95728=AXIS2_PLACEMENT_3D('',#139970,#107633,#107634);
#95729=AXIS2_PLACEMENT_3D('',#139971,#107635,#107636);
#95730=AXIS2_PLACEMENT_3D('',#139975,#107638,#107639);
#95731=AXIS2_PLACEMENT_3D('',#139979,#107641,#107642);
#95732=AXIS2_PLACEMENT_3D('',#139983,#107644,#107645);
#95733=AXIS2_PLACEMENT_3D('',#139985,#107647,#107648);
#95734=AXIS2_PLACEMENT_3D('',#139988,#107650,#107651);
#95735=AXIS2_PLACEMENT_3D('',#139989,#107652,#107653);
#95736=AXIS2_PLACEMENT_3D('',#139992,#107655,#107656);
#95737=AXIS2_PLACEMENT_3D('',#139993,#107657,#107658);
#95738=AXIS2_PLACEMENT_3D('',#139996,#107660,#107661);
#95739=AXIS2_PLACEMENT_3D('',#139997,#107662,#107663);
#95740=AXIS2_PLACEMENT_3D('',#140000,#107665,#107666);
#95741=AXIS2_PLACEMENT_3D('',#140001,#107667,#107668);
#95742=AXIS2_PLACEMENT_3D('',#140002,#107669,#107670);
#95743=AXIS2_PLACEMENT_3D('',#140005,#107671,#107672);
#95744=AXIS2_PLACEMENT_3D('',#140009,#107674,#107675);
#95745=AXIS2_PLACEMENT_3D('',#140022,#107677,#107678);
#95746=AXIS2_PLACEMENT_3D('',#140023,#107679,#107680);
#95747=AXIS2_PLACEMENT_3D('',#140024,#107681,#107682);
#95748=AXIS2_PLACEMENT_3D('',#140025,#107683,#107684);
#95749=AXIS2_PLACEMENT_3D('',#140028,#107685,#107686);
#95750=AXIS2_PLACEMENT_3D('',#140048,#107689,#107690);
#95751=AXIS2_PLACEMENT_3D('',#140049,#107691,#107692);
#95752=AXIS2_PLACEMENT_3D('',#140050,#107693,#107694);
#95753=AXIS2_PLACEMENT_3D('',#140051,#107695,#107696);
#95754=AXIS2_PLACEMENT_3D('',#140054,#107697,#107698);
#95755=AXIS2_PLACEMENT_3D('',#140055,#107699,#107700);
#95756=AXIS2_PLACEMENT_3D('',#140056,#107701,#107702);
#95757=AXIS2_PLACEMENT_3D('',#140074,#107703,#107704);
#95758=AXIS2_PLACEMENT_3D('',#140075,#107705,#107706);
#95759=AXIS2_PLACEMENT_3D('',#140076,#107707,#107708);
#95760=AXIS2_PLACEMENT_3D('',#140077,#107709,#107710);
#95761=AXIS2_PLACEMENT_3D('',#140080,#107711,#107712);
#95762=AXIS2_PLACEMENT_3D('',#140081,#107713,#107714);
#95763=AXIS2_PLACEMENT_3D('',#140082,#107715,#107716);
#95764=AXIS2_PLACEMENT_3D('',#140098,#107717,#107718);
#95765=AXIS2_PLACEMENT_3D('',#140099,#107719,#107720);
#95766=AXIS2_PLACEMENT_3D('',#140100,#107721,#107722);
#95767=AXIS2_PLACEMENT_3D('',#140104,#107724,#107725);
#95768=AXIS2_PLACEMENT_3D('',#140106,#107727,#107728);
#95769=AXIS2_PLACEMENT_3D('',#140109,#107730,#107731);
#95770=AXIS2_PLACEMENT_3D('',#140110,#107732,#107733);
#95771=AXIS2_PLACEMENT_3D('',#140113,#107735,#107736);
#95772=AXIS2_PLACEMENT_3D('',#140114,#107737,#107738);
#95773=AXIS2_PLACEMENT_3D('',#140118,#107741,#107742);
#95774=AXIS2_PLACEMENT_3D('',#140208,#107743,#107744);
#95775=AXIS2_PLACEMENT_3D('',#140243,#107745,#107746);
#95776=AXIS2_PLACEMENT_3D('',#140327,#107747,#107748);
#95777=AXIS2_PLACEMENT_3D('',#140330,#107750,#107751);
#95778=AXIS2_PLACEMENT_3D('',#140331,#107752,#107753);
#95779=AXIS2_PLACEMENT_3D('',#140335,#107755,#107756);
#95780=AXIS2_PLACEMENT_3D('',#140339,#107758,#107759);
#95781=AXIS2_PLACEMENT_3D('',#140348,#107760,#107761);
#95782=AXIS2_PLACEMENT_3D('',#140358,#107762,#107763);
#95783=AXIS2_PLACEMENT_3D('',#140362,#107765,#107766);
#95784=AXIS2_PLACEMENT_3D('',#140366,#107768,#107769);
#95785=AXIS2_PLACEMENT_3D('',#140369,#107771,#107772);
#95786=AXIS2_PLACEMENT_3D('',#140370,#107773,#107774);
#95787=AXIS2_PLACEMENT_3D('',#140371,#107775,#107776);
#95788=AXIS2_PLACEMENT_3D('',#140384,#107777,#107778);
#95789=AXIS2_PLACEMENT_3D('',#140386,#107779,#107780);
#95790=AXIS2_PLACEMENT_3D('',#140388,#107781,#107782);
#95791=AXIS2_PLACEMENT_3D('',#140390,#107784,#107785);
#95792=AXIS2_PLACEMENT_3D('',#140394,#107787,#107788);
#95793=AXIS2_PLACEMENT_3D('',#140401,#107792,#107793);
#95794=AXIS2_PLACEMENT_3D('',#140402,#107794,#107795);
#95795=AXIS2_PLACEMENT_3D('',#140403,#107796,#107797);
#95796=AXIS2_PLACEMENT_3D('',#140411,#107802,#107803);
#95797=AXIS2_PLACEMENT_3D('',#140414,#107804,#107805);
#95798=AXIS2_PLACEMENT_3D('',#140418,#107807,#107808);
#95799=AXIS2_PLACEMENT_3D('',#140420,#107810,#107811);
#95800=AXIS2_PLACEMENT_3D('',#140422,#107812,#107813);
#95801=AXIS2_PLACEMENT_3D('',#140426,#107815,#107816);
#95802=AXIS2_PLACEMENT_3D('',#140429,#107818,#107819);
#95803=AXIS2_PLACEMENT_3D('',#140433,#107821,#107822);
#95804=AXIS2_PLACEMENT_3D('',#140437,#107824,#107825);
#95805=AXIS2_PLACEMENT_3D('',#140438,#107826,#107827);
#95806=AXIS2_PLACEMENT_3D('',#140440,#107828,#107829);
#95807=AXIS2_PLACEMENT_3D('',#140442,#107830,#107831);
#95808=AXIS2_PLACEMENT_3D('',#140444,#107832,#107833);
#95809=AXIS2_PLACEMENT_3D('',#140446,#107834,#107835);
#95810=AXIS2_PLACEMENT_3D('',#140448,#107836,#107837);
#95811=AXIS2_PLACEMENT_3D('',#140452,#107839,#107840);
#95812=AXIS2_PLACEMENT_3D('',#140460,#107844,#107845);
#95813=AXIS2_PLACEMENT_3D('',#140464,#107847,#107848);
#95814=AXIS2_PLACEMENT_3D('',#140467,#107850,#107851);
#95815=AXIS2_PLACEMENT_3D('',#140468,#107852,#107853);
#95816=AXIS2_PLACEMENT_3D('',#140470,#107854,#107855);
#95817=AXIS2_PLACEMENT_3D('',#140472,#107857,#107858);
#95818=AXIS2_PLACEMENT_3D('',#140476,#107860,#107861);
#95819=AXIS2_PLACEMENT_3D('',#140480,#107863,#107864);
#95820=AXIS2_PLACEMENT_3D('',#140484,#107866,#107867);
#95821=AXIS2_PLACEMENT_3D('',#140488,#107869,#107870);
#95822=AXIS2_PLACEMENT_3D('',#140489,#107871,#107872);
#95823=AXIS2_PLACEMENT_3D('',#140490,#107873,#107874);
#95824=AXIS2_PLACEMENT_3D('',#140492,#107875,#107876);
#95825=AXIS2_PLACEMENT_3D('',#140494,#107877,#107878);
#95826=AXIS2_PLACEMENT_3D('',#140496,#107879,#107880);
#95827=AXIS2_PLACEMENT_3D('',#140498,#107881,#107882);
#95828=AXIS2_PLACEMENT_3D('',#140499,#107883,#107884);
#95829=AXIS2_PLACEMENT_3D('',#140503,#107886,#107887);
#95830=AXIS2_PLACEMENT_3D('',#140507,#107889,#107890);
#95831=AXIS2_PLACEMENT_3D('',#140510,#107892,#107893);
#95832=AXIS2_PLACEMENT_3D('',#140512,#107894,#107895);
#95833=AXIS2_PLACEMENT_3D('',#140514,#107896,#107897);
#95834=AXIS2_PLACEMENT_3D('',#140516,#107898,#107899);
#95835=AXIS2_PLACEMENT_3D('',#140519,#107901,#107902);
#95836=AXIS2_PLACEMENT_3D('',#140520,#107903,#107904);
#95837=AXIS2_PLACEMENT_3D('',#140526,#107908,#107909);
#95838=AXIS2_PLACEMENT_3D('',#140530,#107911,#107912);
#95839=AXIS2_PLACEMENT_3D('',#140532,#107914,#107915);
#95840=AXIS2_PLACEMENT_3D('',#140536,#107918,#107919);
#95841=AXIS2_PLACEMENT_3D('',#140539,#107921,#107922);
#95842=AXIS2_PLACEMENT_3D('',#140541,#107923,#107924);
#95843=AXIS2_PLACEMENT_3D('',#140545,#107926,#107927);
#95844=AXIS2_PLACEMENT_3D('',#140548,#107929,#107930);
#95845=AXIS2_PLACEMENT_3D('',#140550,#107931,#107932);
#95846=AXIS2_PLACEMENT_3D('',#140554,#107934,#107935);
#95847=AXIS2_PLACEMENT_3D('',#140558,#107937,#107938);
#95848=AXIS2_PLACEMENT_3D('',#140560,#107939,#107940);
#95849=AXIS2_PLACEMENT_3D('',#140564,#107942,#107943);
#95850=AXIS2_PLACEMENT_3D('',#140566,#107944,#107945);
#95851=AXIS2_PLACEMENT_3D('',#140570,#107947,#107948);
#95852=AXIS2_PLACEMENT_3D('',#140574,#107950,#107951);
#95853=AXIS2_PLACEMENT_3D('',#140577,#107953,#107954);
#95854=AXIS2_PLACEMENT_3D('',#140582,#107956,#107957);
#95855=AXIS2_PLACEMENT_3D('',#140585,#107959,#107960);
#95856=AXIS2_PLACEMENT_3D('',#140587,#107961,#107962);
#95857=AXIS2_PLACEMENT_3D('',#140589,#107963,#107964);
#95858=AXIS2_PLACEMENT_3D('',#140591,#107965,#107966);
#95859=AXIS2_PLACEMENT_3D('',#140592,#107967,#107968);
#95860=AXIS2_PLACEMENT_3D('',#140594,#107970,#107971);
#95861=AXIS2_PLACEMENT_3D('',#140602,#107974,#107975);
#95862=AXIS2_PLACEMENT_3D('',#140604,#107976,#107977);
#95863=AXIS2_PLACEMENT_3D('',#140606,#107979,#107980);
#95864=AXIS2_PLACEMENT_3D('',#140610,#107982,#107983);
#95865=AXIS2_PLACEMENT_3D('',#140612,#107985,#107986);
#95866=AXIS2_PLACEMENT_3D('',#140620,#107989,#107990);
#95867=AXIS2_PLACEMENT_3D('',#140624,#107992,#107993);
#95868=AXIS2_PLACEMENT_3D('',#140628,#107995,#107996);
#95869=AXIS2_PLACEMENT_3D('',#140634,#107999,#108000);
#95870=AXIS2_PLACEMENT_3D('',#140636,#108001,#108002);
#95871=AXIS2_PLACEMENT_3D('',#140640,#108004,#108005);
#95872=AXIS2_PLACEMENT_3D('',#140643,#108007,#108008);
#95873=AXIS2_PLACEMENT_3D('',#140644,#108009,#108010);
#95874=AXIS2_PLACEMENT_3D('',#140645,#108011,#108012);
#95875=AXIS2_PLACEMENT_3D('',#140646,#108013,#108014);
#95876=AXIS2_PLACEMENT_3D('',#140650,#108016,#108017);
#95877=AXIS2_PLACEMENT_3D('',#140652,#108019,#108020);
#95878=AXIS2_PLACEMENT_3D('',#140656,#108023,#108024);
#95879=AXIS2_PLACEMENT_3D('',#140657,#108025,#108026);
#95880=AXIS2_PLACEMENT_3D('',#140658,#108027,#108028);
#95881=AXIS2_PLACEMENT_3D('',#140660,#108029,#108030);
#95882=AXIS2_PLACEMENT_3D('',#140662,#108031,#108032);
#95883=AXIS2_PLACEMENT_3D('',#140664,#108033,#108034);
#95884=AXIS2_PLACEMENT_3D('',#140666,#108035,#108036);
#95885=AXIS2_PLACEMENT_3D('',#140667,#108037,#108038);
#95886=AXIS2_PLACEMENT_3D('',#140668,#108039,#108040);
#95887=AXIS2_PLACEMENT_3D('',#140670,#108041,#108042);
#95888=AXIS2_PLACEMENT_3D('',#140672,#108043,#108044);
#95889=AXIS2_PLACEMENT_3D('',#140675,#108046,#108047);
#95890=AXIS2_PLACEMENT_3D('',#140677,#108048,#108049);
#95891=AXIS2_PLACEMENT_3D('',#140680,#108051,#108052);
#95892=AXIS2_PLACEMENT_3D('',#140681,#108053,#108054);
#95893=AXIS2_PLACEMENT_3D('',#140683,#108056,#108057);
#95894=AXIS2_PLACEMENT_3D('',#140686,#108060,#108061);
#95895=AXIS2_PLACEMENT_3D('',#140688,#108063,#108064);
#95896=AXIS2_PLACEMENT_3D('',#140690,#108066,#108067);
#95897=AXIS2_PLACEMENT_3D('',#140693,#108070,#108071);
#95898=AXIS2_PLACEMENT_3D('',#140695,#108073,#108074);
#95899=AXIS2_PLACEMENT_3D('',#140697,#108076,#108077);
#95900=AXIS2_PLACEMENT_3D('',#140699,#108079,#108080);
#95901=AXIS2_PLACEMENT_3D('',#140701,#108082,#108083);
#95902=AXIS2_PLACEMENT_3D('',#140702,#108084,#108085);
#95903=AXIS2_PLACEMENT_3D('',#140706,#108087,#108088);
#95904=AXIS2_PLACEMENT_3D('',#140708,#108090,#108091);
#95905=AXIS2_PLACEMENT_3D('',#140711,#108093,#108094);
#95906=AXIS2_PLACEMENT_3D('',#140712,#108095,#108096);
#95907=AXIS2_PLACEMENT_3D('',#140713,#108097,#108098);
#95908=AXIS2_PLACEMENT_3D('',#140714,#108099,#108100);
#95909=AXIS2_PLACEMENT_3D('',#140718,#108102,#108103);
#95910=AXIS2_PLACEMENT_3D('',#140720,#108105,#108106);
#95911=AXIS2_PLACEMENT_3D('',#140723,#108108,#108109);
#95912=AXIS2_PLACEMENT_3D('',#140724,#108110,#108111);
#95913=AXIS2_PLACEMENT_3D('',#140728,#108114,#108115);
#95914=AXIS2_PLACEMENT_3D('',#140729,#108116,#108117);
#95915=AXIS2_PLACEMENT_3D('',#140731,#108119,#108120);
#95916=AXIS2_PLACEMENT_3D('',#140733,#108122,#108123);
#95917=AXIS2_PLACEMENT_3D('',#140735,#108125,#108126);
#95918=AXIS2_PLACEMENT_3D('',#140736,#108127,#108128);
#95919=AXIS2_PLACEMENT_3D('',#140737,#108129,#108130);
#95920=AXIS2_PLACEMENT_3D('',#140738,#108131,#108132);
#95921=AXIS2_PLACEMENT_3D('',#140739,#108133,#108134);
#95922=AXIS2_PLACEMENT_3D('',#140742,#108137,#108138);
#95923=AXIS2_PLACEMENT_3D('',#140744,#108140,#108141);
#95924=AXIS2_PLACEMENT_3D('',#140746,#108143,#108144);
#95925=AXIS2_PLACEMENT_3D('',#140748,#108146,#108147);
#95926=AXIS2_PLACEMENT_3D('',#140750,#108149,#108150);
#95927=AXIS2_PLACEMENT_3D('',#140751,#108151,#108152);
#95928=AXIS2_PLACEMENT_3D('',#140754,#108155,#108156);
#95929=AXIS2_PLACEMENT_3D('',#140756,#108158,#108159);
#95930=AXIS2_PLACEMENT_3D('',#140757,#108160,#108161);
#95931=AXIS2_PLACEMENT_3D('',#140759,#108163,#108164);
#95932=AXIS2_PLACEMENT_3D('',#140760,#108165,#108166);
#95933=AXIS2_PLACEMENT_3D('',#140762,#108168,#108169);
#95934=AXIS2_PLACEMENT_3D('',#140763,#108170,#108171);
#95935=AXIS2_PLACEMENT_3D('',#140764,#108172,#108173);
#95936=AXIS2_PLACEMENT_3D('',#140766,#108175,#108176);
#95937=AXIS2_PLACEMENT_3D('',#140772,#108180,#108181);
#95938=AXIS2_PLACEMENT_3D('',#140773,#108182,#108183);
#95939=AXIS2_PLACEMENT_3D('',#140775,#108184,#108185);
#95940=AXIS2_PLACEMENT_3D('',#140776,#108186,#108187);
#95941=AXIS2_PLACEMENT_3D('',#140778,#108188,#108189);
#95942=AXIS2_PLACEMENT_3D('',#140780,#108191,#108192);
#95943=AXIS2_PLACEMENT_3D('',#140782,#108194,#108195);
#95944=AXIS2_PLACEMENT_3D('',#140783,#108196,#108197);
#95945=AXIS2_PLACEMENT_3D('',#140784,#108198,#108199);
#95946=AXIS2_PLACEMENT_3D('',#140786,#108200,#108201);
#95947=AXIS2_PLACEMENT_3D('',#140787,#108202,#108203);
#95948=AXIS2_PLACEMENT_3D('',#140791,#108205,#108206);
#95949=AXIS2_PLACEMENT_3D('',#140793,#108208,#108209);
#95950=AXIS2_PLACEMENT_3D('',#140794,#108210,#108211);
#95951=AXIS2_PLACEMENT_3D('',#140795,#108212,#108213);
#95952=AXIS2_PLACEMENT_3D('',#140796,#108214,#108215);
#95953=AXIS2_PLACEMENT_3D('',#140797,#108216,#108217);
#95954=AXIS2_PLACEMENT_3D('',#140798,#108218,#108219);
#95955=AXIS2_PLACEMENT_3D('',#140800,#108220,#108221);
#95956=AXIS2_PLACEMENT_3D('',#140802,#108223,#108224);
#95957=AXIS2_PLACEMENT_3D('',#140803,#108225,#108226);
#95958=AXIS2_PLACEMENT_3D('',#140804,#108227,#108228);
#95959=AXIS2_PLACEMENT_3D('',#140810,#108232,#108233);
#95960=AXIS2_PLACEMENT_3D('',#140813,#108235,#108236);
#95961=AXIS2_PLACEMENT_3D('',#140814,#108237,#108238);
#95962=AXIS2_PLACEMENT_3D('',#140815,#108239,#108240);
#95963=AXIS2_PLACEMENT_3D('',#140816,#108241,#108242);
#95964=AXIS2_PLACEMENT_3D('',#140819,#108245,#108246);
#95965=AXIS2_PLACEMENT_3D('',#140821,#108248,#108249);
#95966=AXIS2_PLACEMENT_3D('',#140822,#108250,#108251);
#95967=AXIS2_PLACEMENT_3D('',#140825,#108254,#108255);
#95968=AXIS2_PLACEMENT_3D('',#140827,#108257,#108258);
#95969=AXIS2_PLACEMENT_3D('',#140829,#108260,#108261);
#95970=AXIS2_PLACEMENT_3D('',#140831,#108263,#108264);
#95971=AXIS2_PLACEMENT_3D('',#140832,#108265,#108266);
#95972=AXIS2_PLACEMENT_3D('',#140834,#108268,#108269);
#95973=AXIS2_PLACEMENT_3D('',#140836,#108271,#108272);
#95974=AXIS2_PLACEMENT_3D('',#140838,#108274,#108275);
#95975=AXIS2_PLACEMENT_3D('',#140839,#108276,#108277);
#95976=AXIS2_PLACEMENT_3D('',#140840,#108278,#108279);
#95977=AXIS2_PLACEMENT_3D('',#140841,#108280,#108281);
#95978=AXIS2_PLACEMENT_3D('',#140842,#108282,#108283);
#95979=AXIS2_PLACEMENT_3D('',#140844,#108285,#108286);
#95980=AXIS2_PLACEMENT_3D('',#140845,#108287,#108288);
#95981=AXIS2_PLACEMENT_3D('',#140846,#108289,#108290);
#95982=AXIS2_PLACEMENT_3D('',#140847,#108291,#108292);
#95983=AXIS2_PLACEMENT_3D('',#140853,#108295,#108296);
#95984=AXIS2_PLACEMENT_3D('',#140857,#108298,#108299);
#95985=AXIS2_PLACEMENT_3D('',#140860,#108301,#108302);
#95986=AXIS2_PLACEMENT_3D('',#140861,#108303,#108304);
#95987=AXIS2_PLACEMENT_3D('',#140863,#108305,#108306);
#95988=AXIS2_PLACEMENT_3D('',#140864,#108307,#108308);
#95989=AXIS2_PLACEMENT_3D('',#140865,#108309,#108310);
#95990=AXIS2_PLACEMENT_3D('',#140866,#108311,#108312);
#95991=AXIS2_PLACEMENT_3D('',#140868,#108314,#108315);
#95992=AXIS2_PLACEMENT_3D('',#140869,#108316,#108317);
#95993=AXIS2_PLACEMENT_3D('',#140870,#108318,#108319);
#95994=AXIS2_PLACEMENT_3D('',#140872,#108321,#108322);
#95995=AXIS2_PLACEMENT_3D('',#140874,#108324,#108325);
#95996=AXIS2_PLACEMENT_3D('',#140875,#108326,#108327);
#95997=AXIS2_PLACEMENT_3D('',#140876,#108328,#108329);
#95998=AXIS2_PLACEMENT_3D('',#140877,#108330,#108331);
#95999=AXIS2_PLACEMENT_3D('',#140879,#108332,#108333);
#96000=AXIS2_PLACEMENT_3D('',#140880,#108334,#108335);
#96001=AXIS2_PLACEMENT_3D('',#140882,#108336,#108337);
#96002=AXIS2_PLACEMENT_3D('',#140884,#108339,#108340);
#96003=AXIS2_PLACEMENT_3D('',#140886,#108341,#108342);
#96004=AXIS2_PLACEMENT_3D('',#140887,#108343,#108344);
#96005=AXIS2_PLACEMENT_3D('',#140889,#108346,#108347);
#96006=AXIS2_PLACEMENT_3D('',#140893,#108349,#108350);
#96007=AXIS2_PLACEMENT_3D('',#140895,#108352,#108353);
#96008=AXIS2_PLACEMENT_3D('',#140899,#108356,#108357);
#96009=AXIS2_PLACEMENT_3D('',#140902,#108359,#108360);
#96010=AXIS2_PLACEMENT_3D('',#140903,#108361,#108362);
#96011=AXIS2_PLACEMENT_3D('',#140906,#108363,#108364);
#96012=AXIS2_PLACEMENT_3D('',#140909,#108367,#108368);
#96013=AXIS2_PLACEMENT_3D('',#140913,#108371,#108372);
#96014=AXIS2_PLACEMENT_3D('',#140915,#108373,#108374);
#96015=AXIS2_PLACEMENT_3D('',#140917,#108376,#108377);
#96016=AXIS2_PLACEMENT_3D('',#140919,#108379,#108380);
#96017=AXIS2_PLACEMENT_3D('',#140921,#108381,#108382);
#96018=AXIS2_PLACEMENT_3D('',#140922,#108383,#108384);
#96019=AXIS2_PLACEMENT_3D('',#140924,#108386,#108387);
#96020=AXIS2_PLACEMENT_3D('',#140926,#108388,#108389);
#96021=AXIS2_PLACEMENT_3D('',#140928,#108391,#108392);
#96022=AXIS2_PLACEMENT_3D('',#140930,#108393,#108394);
#96023=AXIS2_PLACEMENT_3D('',#140932,#108396,#108397);
#96024=AXIS2_PLACEMENT_3D('',#140935,#108398,#108399);
#96025=AXIS2_PLACEMENT_3D('',#140938,#108402,#108403);
#96026=AXIS2_PLACEMENT_3D('',#140942,#108406,#108407);
#96027=AXIS2_PLACEMENT_3D('',#140943,#108408,#108409);
#96028=AXIS2_PLACEMENT_3D('',#140944,#108410,#108411);
#96029=AXIS2_PLACEMENT_3D('',#140945,#108412,#108413);
#96030=AXIS2_PLACEMENT_3D('',#140946,#108414,#108415);
#96031=AXIS2_PLACEMENT_3D('',#140947,#108416,#108417);
#96032=AXIS2_PLACEMENT_3D('',#140950,#108418,#108419);
#96033=AXIS2_PLACEMENT_3D('',#140955,#108422,#108423);
#96034=AXIS2_PLACEMENT_3D('',#140957,#108425,#108426);
#96035=AXIS2_PLACEMENT_3D('',#140958,#108427,#108428);
#96036=AXIS2_PLACEMENT_3D('',#140960,#108430,#108431);
#96037=AXIS2_PLACEMENT_3D('',#140962,#108433,#108434);
#96038=AXIS2_PLACEMENT_3D('',#140964,#108436,#108437);
#96039=AXIS2_PLACEMENT_3D('',#140966,#108439,#108440);
#96040=AXIS2_PLACEMENT_3D('',#140968,#108442,#108443);
#96041=AXIS2_PLACEMENT_3D('',#140970,#108445,#108446);
#96042=AXIS2_PLACEMENT_3D('',#140972,#108448,#108449);
#96043=AXIS2_PLACEMENT_3D('',#140974,#108451,#108452);
#96044=AXIS2_PLACEMENT_3D('',#140976,#108454,#108455);
#96045=AXIS2_PLACEMENT_3D('',#140977,#108456,#108457);
#96046=AXIS2_PLACEMENT_3D('',#141000,#108459,#108460);
#96047=AXIS2_PLACEMENT_3D('',#141006,#108464,#108465);
#96048=AXIS2_PLACEMENT_3D('',#141008,#108466,#108467);
#96049=AXIS2_PLACEMENT_3D('',#141009,#108468,#108469);
#96050=AXIS2_PLACEMENT_3D('',#141010,#108470,#108471);
#96051=AXIS2_PLACEMENT_3D('',#141012,#108473,#108474);
#96052=AXIS2_PLACEMENT_3D('',#141013,#108475,#108476);
#96053=AXIS2_PLACEMENT_3D('',#141016,#108477,#108478);
#96054=AXIS2_PLACEMENT_3D('',#141020,#108480,#108481);
#96055=AXIS2_PLACEMENT_3D('',#141022,#108483,#108484);
#96056=AXIS2_PLACEMENT_3D('',#141024,#108485,#108486);
#96057=AXIS2_PLACEMENT_3D('',#141026,#108487,#108488);
#96058=AXIS2_PLACEMENT_3D('',#141030,#108490,#108491);
#96059=AXIS2_PLACEMENT_3D('',#141034,#108493,#108494);
#96060=AXIS2_PLACEMENT_3D('',#141036,#108495,#108496);
#96061=AXIS2_PLACEMENT_3D('',#141038,#108497,#108498);
#96062=AXIS2_PLACEMENT_3D('',#141042,#108500,#108501);
#96063=AXIS2_PLACEMENT_3D('',#141046,#108503,#108504);
#96064=AXIS2_PLACEMENT_3D('',#141050,#108506,#108507);
#96065=AXIS2_PLACEMENT_3D('',#141054,#108509,#108510);
#96066=AXIS2_PLACEMENT_3D('',#141058,#108512,#108513);
#96067=AXIS2_PLACEMENT_3D('',#141060,#108515,#108516);
#96068=AXIS2_PLACEMENT_3D('',#141062,#108517,#108518);
#96069=AXIS2_PLACEMENT_3D('',#141064,#108520,#108521);
#96070=AXIS2_PLACEMENT_3D('',#141066,#108522,#108523);
#96071=AXIS2_PLACEMENT_3D('',#141068,#108525,#108526);
#96072=AXIS2_PLACEMENT_3D('',#141076,#108531,#108532);
#96073=AXIS2_PLACEMENT_3D('',#141079,#108533,#108534);
#96074=AXIS2_PLACEMENT_3D('',#141081,#108535,#108536);
#96075=AXIS2_PLACEMENT_3D('',#141083,#108537,#108538);
#96076=AXIS2_PLACEMENT_3D('',#141084,#108539,#108540);
#96077=AXIS2_PLACEMENT_3D('',#141101,#108541,#108542);
#96078=AXIS2_PLACEMENT_3D('',#141102,#108543,#108544);
#96079=AXIS2_PLACEMENT_3D('',#141103,#108545,#108546);
#96080=AXIS2_PLACEMENT_3D('',#141104,#108547,#108548);
#96081=AXIS2_PLACEMENT_3D('',#141106,#108549,#108550);
#96082=AXIS2_PLACEMENT_3D('',#141119,#108552,#108553);
#96083=AXIS2_PLACEMENT_3D('',#141120,#108554,#108555);
#96084=AXIS2_PLACEMENT_3D('',#141121,#108556,#108557);
#96085=AXIS2_PLACEMENT_3D('',#141122,#108558,#108559);
#96086=AXIS2_PLACEMENT_3D('',#141125,#108560,#108561);
#96087=AXIS2_PLACEMENT_3D('',#141145,#108564,#108565);
#96088=AXIS2_PLACEMENT_3D('',#141146,#108566,#108567);
#96089=AXIS2_PLACEMENT_3D('',#141147,#108568,#108569);
#96090=AXIS2_PLACEMENT_3D('',#141148,#108570,#108571);
#96091=AXIS2_PLACEMENT_3D('',#141151,#108572,#108573);
#96092=AXIS2_PLACEMENT_3D('',#141152,#108574,#108575);
#96093=AXIS2_PLACEMENT_3D('',#141153,#108576,#108577);
#96094=AXIS2_PLACEMENT_3D('',#141169,#108578,#108579);
#96095=AXIS2_PLACEMENT_3D('',#141170,#108580,#108581);
#96096=AXIS2_PLACEMENT_3D('',#141171,#108582,#108583);
#96097=AXIS2_PLACEMENT_3D('',#141175,#108585,#108586);
#96098=AXIS2_PLACEMENT_3D('',#141177,#108588,#108589);
#96099=AXIS2_PLACEMENT_3D('',#141180,#108591,#108592);
#96100=AXIS2_PLACEMENT_3D('',#141181,#108593,#108594);
#96101=AXIS2_PLACEMENT_3D('',#141184,#108596,#108597);
#96102=AXIS2_PLACEMENT_3D('',#141185,#108598,#108599);
#96103=AXIS2_PLACEMENT_3D('',#141189,#108601,#108602);
#96104=AXIS2_PLACEMENT_3D('',#141192,#108604,#108605);
#96105=AXIS2_PLACEMENT_3D('',#141193,#108606,#108607);
#96106=AXIS2_PLACEMENT_3D('',#141194,#108608,#108609);
#96107=AXIS2_PLACEMENT_3D('',#141197,#108610,#108611);
#96108=AXIS2_PLACEMENT_3D('',#141199,#108612,#108613);
#96109=AXIS2_PLACEMENT_3D('',#141201,#108614,#108615);
#96110=AXIS2_PLACEMENT_3D('',#141216,#108616,#108617);
#96111=AXIS2_PLACEMENT_3D('',#141219,#108618,#108619);
#96112=AXIS2_PLACEMENT_3D('',#141221,#108620,#108621);
#96113=AXIS2_PLACEMENT_3D('',#141223,#108622,#108623);
#96114=AXIS2_PLACEMENT_3D('',#141238,#108624,#108625);
#96115=AXIS2_PLACEMENT_3D('',#141241,#108626,#108627);
#96116=AXIS2_PLACEMENT_3D('',#141244,#108630,#108631);
#96117=AXIS2_PLACEMENT_3D('',#141245,#108632,#108633);
#96118=AXIS2_PLACEMENT_3D('',#141246,#108634,#108635);
#96119=AXIS2_PLACEMENT_3D('',#141247,#108636,#108637);
#96120=AXIS2_PLACEMENT_3D('',#141250,#108638,#108639);
#96121=AXIS2_PLACEMENT_3D('',#141252,#108640,#108641);
#96122=AXIS2_PLACEMENT_3D('',#141254,#108642,#108643);
#96123=AXIS2_PLACEMENT_3D('',#141269,#108644,#108645);
#96124=AXIS2_PLACEMENT_3D('',#141270,#108646,#108647);
#96125=AXIS2_PLACEMENT_3D('',#141271,#108648,#108649);
#96126=AXIS2_PLACEMENT_3D('',#141272,#108650,#108651);
#96127=AXIS2_PLACEMENT_3D('',#141274,#108652,#108653);
#96128=AXIS2_PLACEMENT_3D('',#141276,#108654,#108655);
#96129=AXIS2_PLACEMENT_3D('',#141293,#108656,#108657);
#96130=AXIS2_PLACEMENT_3D('',#141296,#108660,#108661);
#96131=AXIS2_PLACEMENT_3D('',#141300,#108663,#108664);
#96132=AXIS2_PLACEMENT_3D('',#141302,#108666,#108667);
#96133=AXIS2_PLACEMENT_3D('',#141305,#108669,#108670);
#96134=AXIS2_PLACEMENT_3D('',#141306,#108671,#108672);
#96135=AXIS2_PLACEMENT_3D('',#141310,#108675,#108676);
#96136=AXIS2_PLACEMENT_3D('',#141313,#108678,#108679);
#96137=AXIS2_PLACEMENT_3D('',#141314,#108680,#108681);
#96138=AXIS2_PLACEMENT_3D('',#141315,#108682,#108683);
#96139=AXIS2_PLACEMENT_3D('',#141331,#108684,#108685);
#96140=AXIS2_PLACEMENT_3D('',#141333,#108686,#108687);
#96141=AXIS2_PLACEMENT_3D('',#141335,#108688,#108689);
#96142=AXIS2_PLACEMENT_3D('',#141361,#108690,#108691);
#96143=AXIS2_PLACEMENT_3D('',#141362,#108692,#108693);
#96144=AXIS2_PLACEMENT_3D('',#141363,#108694,#108695);
#96145=AXIS2_PLACEMENT_3D('',#141364,#108696,#108697);
#96146=AXIS2_PLACEMENT_3D('',#141374,#108698,#108699);
#96147=AXIS2_PLACEMENT_3D('',#141390,#108700,#108701);
#96148=AXIS2_PLACEMENT_3D('',#141392,#108702,#108703);
#96149=AXIS2_PLACEMENT_3D('',#141399,#108704,#108705);
#96150=AXIS2_PLACEMENT_3D('',#141417,#108709,#108710);
#96151=AXIS2_PLACEMENT_3D('',#141455,#108713,#108714);
#96152=AXIS2_PLACEMENT_3D('',#141470,#108716,#108717);
#96153=AXIS2_PLACEMENT_3D('',#141474,#108719,#108720);
#96154=AXIS2_PLACEMENT_3D('',#141507,#108721,#108722);
#96155=AXIS2_PLACEMENT_3D('',#141508,#108723,#108724);
#96156=AXIS2_PLACEMENT_3D('',#141512,#108726,#108727);
#96157=AXIS2_PLACEMENT_3D('',#141514,#108729,#108730);
#96158=AXIS2_PLACEMENT_3D('',#141519,#108733,#108734);
#96159=AXIS2_PLACEMENT_3D('',#141520,#108735,#108736);
#96160=AXIS2_PLACEMENT_3D('',#141522,#108737,#108738);
#96161=AXIS2_PLACEMENT_3D('',#141546,#108742,#108743);
#96162=AXIS2_PLACEMENT_3D('',#141557,#108744,#108745);
#96163=AXIS2_PLACEMENT_3D('',#141558,#108746,#108747);
#96164=AXIS2_PLACEMENT_3D('',#141559,#108748,#108749);
#96165=AXIS2_PLACEMENT_3D('',#141561,#108751,#108752);
#96166=AXIS2_PLACEMENT_3D('',#141565,#108754,#108755);
#96167=AXIS2_PLACEMENT_3D('',#141567,#108756,#108757);
#96168=AXIS2_PLACEMENT_3D('',#141574,#108759,#108760);
#96169=AXIS2_PLACEMENT_3D('',#141575,#108761,#108762);
#96170=AXIS2_PLACEMENT_3D('',#141592,#108764,#108765);
#96171=AXIS2_PLACEMENT_3D('',#141594,#108766,#108767);
#96172=AXIS2_PLACEMENT_3D('',#141617,#108778,#108779);
#96173=AXIS2_PLACEMENT_3D('',#141621,#108781,#108782);
#96174=AXIS2_PLACEMENT_3D('',#141623,#108784,#108785);
#96175=AXIS2_PLACEMENT_3D('',#141625,#108786,#108787);
#96176=AXIS2_PLACEMENT_3D('',#141628,#108790,#108791);
#96177=AXIS2_PLACEMENT_3D('',#141634,#108793,#108794);
#96178=AXIS2_PLACEMENT_3D('',#141638,#108797,#108798);
#96179=AXIS2_PLACEMENT_3D('',#141641,#108799,#108800);
#96180=AXIS2_PLACEMENT_3D('',#141643,#108801,#108802);
#96181=AXIS2_PLACEMENT_3D('',#141645,#108803,#108804);
#96182=AXIS2_PLACEMENT_3D('',#141679,#108805,#108806);
#96183=AXIS2_PLACEMENT_3D('',#141680,#108807,#108808);
#96184=AXIS2_PLACEMENT_3D('',#141681,#108809,#108810);
#96185=AXIS2_PLACEMENT_3D('',#141682,#108811,#108812);
#96186=AXIS2_PLACEMENT_3D('',#141685,#108813,#108814);
#96187=AXIS2_PLACEMENT_3D('',#141686,#108815,#108816);
#96188=AXIS2_PLACEMENT_3D('',#141687,#108817,#108818);
#96189=AXIS2_PLACEMENT_3D('',#141699,#108819,#108820);
#96190=AXIS2_PLACEMENT_3D('',#141700,#108821,#108822);
#96191=AXIS2_PLACEMENT_3D('',#141701,#108823,#108824);
#96192=AXIS2_PLACEMENT_3D('',#141702,#108825,#108826);
#96193=AXIS2_PLACEMENT_3D('',#141707,#108829,#108830);
#96194=AXIS2_PLACEMENT_3D('',#141708,#108831,#108832);
#96195=AXIS2_PLACEMENT_3D('',#141711,#108835,#108836);
#96196=AXIS2_PLACEMENT_3D('',#141715,#108838,#108839);
#96197=AXIS2_PLACEMENT_3D('',#141721,#108843,#108844);
#96198=AXIS2_PLACEMENT_3D('',#141743,#108848,#108849);
#96199=AXIS2_PLACEMENT_3D('',#141746,#108851,#108852);
#96200=AXIS2_PLACEMENT_3D('',#141747,#108853,#108854);
#96201=AXIS2_PLACEMENT_3D('',#141748,#108855,#108856);
#96202=AXIS2_PLACEMENT_3D('',#141756,#108857,#108858);
#96203=AXIS2_PLACEMENT_3D('',#141778,#108859,#108860);
#96204=AXIS2_PLACEMENT_3D('',#141821,#108861,#108862);
#96205=AXIS2_PLACEMENT_3D('',#141822,#108863,#108864);
#96206=AXIS2_PLACEMENT_3D('',#141823,#108865,#108866);
#96207=AXIS2_PLACEMENT_3D('',#141825,#108867,#108868);
#96208=AXIS2_PLACEMENT_3D('',#141826,#108869,#108870);
#96209=AXIS2_PLACEMENT_3D('',#141827,#108871,#108872);
#96210=AXIS2_PLACEMENT_3D('',#141829,#108873,#108874);
#96211=AXIS2_PLACEMENT_3D('',#141831,#108875,#108876);
#96212=AXIS2_PLACEMENT_3D('',#141832,#108877,#108878);
#96213=AXIS2_PLACEMENT_3D('',#141833,#108879,#108880);
#96214=AXIS2_PLACEMENT_3D('',#141835,#108881,#108882);
#96215=AXIS2_PLACEMENT_3D('',#141837,#108883,#108884);
#96216=AXIS2_PLACEMENT_3D('',#141841,#108886,#108887);
#96217=AXIS2_PLACEMENT_3D('',#141845,#108889,#108890);
#96218=AXIS2_PLACEMENT_3D('',#141847,#108892,#108893);
#96219=AXIS2_PLACEMENT_3D('',#141849,#108894,#108895);
#96220=AXIS2_PLACEMENT_3D('',#141861,#108897,#108898);
#96221=AXIS2_PLACEMENT_3D('',#141862,#108899,#108900);
#96222=AXIS2_PLACEMENT_3D('',#141863,#108901,#108902);
#96223=AXIS2_PLACEMENT_3D('',#141865,#108903,#108904);
#96224=AXIS2_PLACEMENT_3D('',#141877,#108906,#108907);
#96225=AXIS2_PLACEMENT_3D('',#141878,#108908,#108909);
#96226=AXIS2_PLACEMENT_3D('',#141879,#108910,#108911);
#96227=AXIS2_PLACEMENT_3D('',#141881,#108912,#108913);
#96228=AXIS2_PLACEMENT_3D('',#141893,#108915,#108916);
#96229=AXIS2_PLACEMENT_3D('',#141894,#108917,#108918);
#96230=AXIS2_PLACEMENT_3D('',#141895,#108919,#108920);
#96231=AXIS2_PLACEMENT_3D('',#141896,#108921,#108922);
#96232=AXIS2_PLACEMENT_3D('',#141897,#108923,#108924);
#96233=AXIS2_PLACEMENT_3D('',#141901,#108926,#108927);
#96234=AXIS2_PLACEMENT_3D('',#141913,#108929,#108930);
#96235=AXIS2_PLACEMENT_3D('',#141916,#108932,#108933);
#96236=AXIS2_PLACEMENT_3D('',#141917,#108934,#108935);
#96237=AXIS2_PLACEMENT_3D('',#141920,#108937,#108938);
#96238=AXIS2_PLACEMENT_3D('',#141921,#108939,#108940);
#96239=AXIS2_PLACEMENT_3D('',#141925,#108943,#108944);
#96240=AXIS2_PLACEMENT_3D('',#141928,#108946,#108947);
#96241=AXIS2_PLACEMENT_3D('',#141929,#108948,#108949);
#96242=AXIS2_PLACEMENT_3D('',#141933,#108952,#108953);
#96243=AXIS2_PLACEMENT_3D('',#141936,#108955,#108956);
#96244=AXIS2_PLACEMENT_3D('',#141937,#108957,#108958);
#96245=AXIS2_PLACEMENT_3D('',#141941,#108961,#108962);
#96246=AXIS2_PLACEMENT_3D('',#141944,#108964,#108965);
#96247=AXIS2_PLACEMENT_3D('',#141945,#108966,#108967);
#96248=AXIS2_PLACEMENT_3D('',#141972,#108968,#108969);
#96249=AXIS2_PLACEMENT_3D('',#141976,#108971,#108972);
#96250=AXIS2_PLACEMENT_3D('',#141980,#108974,#108975);
#96251=AXIS2_PLACEMENT_3D('',#142029,#108977,#108978);
#96252=AXIS2_PLACEMENT_3D('',#142030,#108979,#108980);
#96253=AXIS2_PLACEMENT_3D('',#142031,#108981,#108982);
#96254=AXIS2_PLACEMENT_3D('',#142034,#108983,#108984);
#96255=AXIS2_PLACEMENT_3D('',#142036,#108985,#108986);
#96256=AXIS2_PLACEMENT_3D('',#142038,#108987,#108988);
#96257=AXIS2_PLACEMENT_3D('',#142039,#108989,#108990);
#96258=AXIS2_PLACEMENT_3D('',#142057,#108991,#108992);
#96259=AXIS2_PLACEMENT_3D('',#142058,#108993,#108994);
#96260=AXIS2_PLACEMENT_3D('',#142059,#108995,#108996);
#96261=AXIS2_PLACEMENT_3D('',#142060,#108997,#108998);
#96262=AXIS2_PLACEMENT_3D('',#142063,#108999,#109000);
#96263=AXIS2_PLACEMENT_3D('',#142066,#109003,#109004);
#96264=AXIS2_PLACEMENT_3D('',#142069,#109005,#109006);
#96265=AXIS2_PLACEMENT_3D('',#142070,#109007,#109008);
#96266=AXIS2_PLACEMENT_3D('',#142071,#109009,#109010);
#96267=AXIS2_PLACEMENT_3D('',#142072,#109011,#109012);
#96268=AXIS2_PLACEMENT_3D('',#142075,#109013,#109014);
#96269=AXIS2_PLACEMENT_3D('',#142095,#109017,#109018);
#96270=AXIS2_PLACEMENT_3D('',#142096,#109019,#109020);
#96271=AXIS2_PLACEMENT_3D('',#142097,#109021,#109022);
#96272=AXIS2_PLACEMENT_3D('',#142098,#109023,#109024);
#96273=AXIS2_PLACEMENT_3D('',#142101,#109025,#109026);
#96274=AXIS2_PLACEMENT_3D('',#142103,#109027,#109028);
#96275=AXIS2_PLACEMENT_3D('',#142105,#109029,#109030);
#96276=AXIS2_PLACEMENT_3D('',#142106,#109031,#109032);
#96277=AXIS2_PLACEMENT_3D('',#142124,#109033,#109034);
#96278=AXIS2_PLACEMENT_3D('',#142125,#109035,#109036);
#96279=AXIS2_PLACEMENT_3D('',#142126,#109037,#109038);
#96280=AXIS2_PLACEMENT_3D('',#142127,#109039,#109040);
#96281=AXIS2_PLACEMENT_3D('',#142130,#109041,#109042);
#96282=AXIS2_PLACEMENT_3D('',#142131,#109043,#109044);
#96283=AXIS2_PLACEMENT_3D('',#142132,#109045,#109046);
#96284=AXIS2_PLACEMENT_3D('',#142133,#109047,#109048);
#96285=AXIS2_PLACEMENT_3D('',#142135,#109049,#109050);
#96286=AXIS2_PLACEMENT_3D('',#142138,#109053,#109054);
#96287=AXIS2_PLACEMENT_3D('',#142139,#109055,#109056);
#96288=AXIS2_PLACEMENT_3D('',#142140,#109057,#109058);
#96289=AXIS2_PLACEMENT_3D('',#142141,#109059,#109060);
#96290=AXIS2_PLACEMENT_3D('',#142142,#109061,#109062);
#96291=AXIS2_PLACEMENT_3D('',#142143,#109063,#109064);
#96292=AXIS2_PLACEMENT_3D('',#142149,#109068,#109069);
#96293=AXIS2_PLACEMENT_3D('',#142152,#109071,#109072);
#96294=AXIS2_PLACEMENT_3D('',#142153,#109073,#109074);
#96295=AXIS2_PLACEMENT_3D('',#142157,#109077,#109078);
#96296=AXIS2_PLACEMENT_3D('',#142160,#109080,#109081);
#96297=AXIS2_PLACEMENT_3D('',#142161,#109082,#109083);
#96298=AXIS2_PLACEMENT_3D('',#142164,#109085,#109086);
#96299=AXIS2_PLACEMENT_3D('',#142165,#109087,#109088);
#96300=AXIS2_PLACEMENT_3D('',#142168,#109090,#109091);
#96301=AXIS2_PLACEMENT_3D('',#142169,#109092,#109093);
#96302=AXIS2_PLACEMENT_3D('',#142170,#109094,#109095);
#96303=AXIS2_PLACEMENT_3D('',#142173,#109096,#109097);
#96304=AXIS2_PLACEMENT_3D('',#142177,#109099,#109100);
#96305=AXIS2_PLACEMENT_3D('',#142190,#109102,#109103);
#96306=AXIS2_PLACEMENT_3D('',#142191,#109104,#109105);
#96307=AXIS2_PLACEMENT_3D('',#142192,#109106,#109107);
#96308=AXIS2_PLACEMENT_3D('',#142193,#109108,#109109);
#96309=AXIS2_PLACEMENT_3D('',#142196,#109110,#109111);
#96310=AXIS2_PLACEMENT_3D('',#142199,#109114,#109115);
#96311=AXIS2_PLACEMENT_3D('',#142202,#109116,#109117);
#96312=AXIS2_PLACEMENT_3D('',#142203,#109118,#109119);
#96313=AXIS2_PLACEMENT_3D('',#142204,#109120,#109121);
#96314=AXIS2_PLACEMENT_3D('',#142222,#109122,#109123);
#96315=AXIS2_PLACEMENT_3D('',#142223,#109124,#109125);
#96316=AXIS2_PLACEMENT_3D('',#142224,#109126,#109127);
#96317=AXIS2_PLACEMENT_3D('',#142225,#109128,#109129);
#96318=AXIS2_PLACEMENT_3D('',#142228,#109130,#109131);
#96319=AXIS2_PLACEMENT_3D('',#142231,#109134,#109135);
#96320=AXIS2_PLACEMENT_3D('',#142234,#109136,#109137);
#96321=AXIS2_PLACEMENT_3D('',#142235,#109138,#109139);
#96322=AXIS2_PLACEMENT_3D('',#142236,#109140,#109141);
#96323=AXIS2_PLACEMENT_3D('',#142254,#109142,#109143);
#96324=AXIS2_PLACEMENT_3D('',#142255,#109144,#109145);
#96325=AXIS2_PLACEMENT_3D('',#142256,#109146,#109147);
#96326=AXIS2_PLACEMENT_3D('',#142257,#109148,#109149);
#96327=AXIS2_PLACEMENT_3D('',#142260,#109150,#109151);
#96328=AXIS2_PLACEMENT_3D('',#142261,#109152,#109153);
#96329=AXIS2_PLACEMENT_3D('',#142262,#109154,#109155);
#96330=AXIS2_PLACEMENT_3D('',#142274,#109156,#109157);
#96331=AXIS2_PLACEMENT_3D('',#142275,#109158,#109159);
#96332=AXIS2_PLACEMENT_3D('',#142276,#109160,#109161);
#96333=AXIS2_PLACEMENT_3D('',#142277,#109162,#109163);
#96334=AXIS2_PLACEMENT_3D('',#142280,#109164,#109165);
#96335=AXIS2_PLACEMENT_3D('',#142292,#109168,#109169);
#96336=AXIS2_PLACEMENT_3D('',#142293,#109170,#109171);
#96337=AXIS2_PLACEMENT_3D('',#142294,#109172,#109173);
#96338=AXIS2_PLACEMENT_3D('',#142298,#109175,#109176);
#96339=AXIS2_PLACEMENT_3D('',#142300,#109178,#109179);
#96340=AXIS2_PLACEMENT_3D('',#142303,#109181,#109182);
#96341=AXIS2_PLACEMENT_3D('',#142304,#109183,#109184);
#96342=AXIS2_PLACEMENT_3D('',#142307,#109186,#109187);
#96343=AXIS2_PLACEMENT_3D('',#142308,#109188,#109189);
#96344=AXIS2_PLACEMENT_3D('',#142312,#109192,#109193);
#96345=AXIS2_PLACEMENT_3D('',#142315,#109195,#109196);
#96346=AXIS2_PLACEMENT_3D('',#142316,#109197,#109198);
#96347=AXIS2_PLACEMENT_3D('',#142320,#109201,#109202);
#96348=AXIS2_PLACEMENT_3D('',#142321,#109203,#109204);
#96349=AXIS2_PLACEMENT_3D('',#142324,#109205,#109206);
#96350=AXIS2_PLACEMENT_3D('',#142328,#109208,#109209);
#96351=AXIS2_PLACEMENT_3D('',#142341,#109211,#109212);
#96352=AXIS2_PLACEMENT_3D('',#142342,#109213,#109214);
#96353=AXIS2_PLACEMENT_3D('',#142343,#109215,#109216);
#96354=AXIS2_PLACEMENT_3D('',#142344,#109217,#109218);
#96355=AXIS2_PLACEMENT_3D('',#142347,#109219,#109220);
#96356=AXIS2_PLACEMENT_3D('',#142361,#109223,#109224);
#96357=AXIS2_PLACEMENT_3D('',#142362,#109225,#109226);
#96358=AXIS2_PLACEMENT_3D('',#142363,#109227,#109228);
#96359=AXIS2_PLACEMENT_3D('',#142364,#109229,#109230);
#96360=AXIS2_PLACEMENT_3D('',#142367,#109231,#109232);
#96361=AXIS2_PLACEMENT_3D('',#142370,#109235,#109236);
#96362=AXIS2_PLACEMENT_3D('',#142373,#109237,#109238);
#96363=AXIS2_PLACEMENT_3D('',#142374,#109239,#109240);
#96364=AXIS2_PLACEMENT_3D('',#142375,#109241,#109242);
#96365=AXIS2_PLACEMENT_3D('',#142376,#109243,#109244);
#96366=AXIS2_PLACEMENT_3D('',#142379,#109245,#109246);
#96367=AXIS2_PLACEMENT_3D('',#142380,#109247,#109248);
#96368=AXIS2_PLACEMENT_3D('',#142381,#109249,#109250);
#96369=AXIS2_PLACEMENT_3D('',#142399,#109251,#109252);
#96370=AXIS2_PLACEMENT_3D('',#142400,#109253,#109254);
#96371=AXIS2_PLACEMENT_3D('',#142401,#109255,#109256);
#96372=AXIS2_PLACEMENT_3D('',#142402,#109257,#109258);
#96373=AXIS2_PLACEMENT_3D('',#142405,#109259,#109260);
#96374=AXIS2_PLACEMENT_3D('',#142406,#109261,#109262);
#96375=AXIS2_PLACEMENT_3D('',#142407,#109263,#109264);
#96376=AXIS2_PLACEMENT_3D('',#142408,#109265,#109266);
#96377=AXIS2_PLACEMENT_3D('',#142411,#109267,#109268);
#96378=AXIS2_PLACEMENT_3D('',#142412,#109269,#109270);
#96379=AXIS2_PLACEMENT_3D('',#142413,#109271,#109272);
#96380=AXIS2_PLACEMENT_3D('',#142423,#109273,#109274);
#96381=AXIS2_PLACEMENT_3D('',#142424,#109275,#109276);
#96382=AXIS2_PLACEMENT_3D('',#142425,#109277,#109278);
#96383=AXIS2_PLACEMENT_3D('',#142429,#109280,#109281);
#96384=AXIS2_PLACEMENT_3D('',#142431,#109283,#109284);
#96385=AXIS2_PLACEMENT_3D('',#142434,#109286,#109287);
#96386=AXIS2_PLACEMENT_3D('',#142435,#109288,#109289);
#96387=AXIS2_PLACEMENT_3D('',#142439,#109291,#109292);
#96388=AXIS2_PLACEMENT_3D('',#142442,#109294,#109295);
#96389=AXIS2_PLACEMENT_3D('',#142443,#109296,#109297);
#96390=AXIS2_PLACEMENT_3D('',#142447,#109299,#109300);
#96391=AXIS2_PLACEMENT_3D('',#142520,#109302,#109303);
#96392=AXIS2_PLACEMENT_3D('',#142523,#109305,#109306);
#96393=AXIS2_PLACEMENT_3D('',#142524,#109307,#109308);
#96394=AXIS2_PLACEMENT_3D('',#142527,#109310,#109311);
#96395=AXIS2_PLACEMENT_3D('',#142528,#109312,#109313);
#96396=AXIS2_PLACEMENT_3D('',#142532,#109316,#109317);
#96397=AXIS2_PLACEMENT_3D('',#142533,#109318,#109319);
#96398=AXIS2_PLACEMENT_3D('',#142536,#109320,#109321);
#96399=AXIS2_PLACEMENT_3D('',#142538,#109322,#109323);
#96400=AXIS2_PLACEMENT_3D('',#142540,#109324,#109325);
#96401=AXIS2_PLACEMENT_3D('',#142572,#109326,#109327);
#96402=AXIS2_PLACEMENT_3D('',#142573,#109328,#109329);
#96403=AXIS2_PLACEMENT_3D('',#142574,#109330,#109331);
#96404=AXIS2_PLACEMENT_3D('',#142575,#109332,#109333);
#96405=AXIS2_PLACEMENT_3D('',#142578,#109334,#109335);
#96406=AXIS2_PLACEMENT_3D('',#142579,#109336,#109337);
#96407=AXIS2_PLACEMENT_3D('',#142580,#109338,#109339);
#96408=AXIS2_PLACEMENT_3D('',#142598,#109340,#109341);
#96409=AXIS2_PLACEMENT_3D('',#142599,#109342,#109343);
#96410=AXIS2_PLACEMENT_3D('',#142600,#109344,#109345);
#96411=AXIS2_PLACEMENT_3D('',#142601,#109346,#109347);
#96412=AXIS2_PLACEMENT_3D('',#142606,#109350,#109351);
#96413=AXIS2_PLACEMENT_3D('',#142607,#109352,#109353);
#96414=AXIS2_PLACEMENT_3D('',#142616,#109356,#109357);
#96415=AXIS2_PLACEMENT_3D('',#142617,#109358,#109359);
#96416=AXIS2_PLACEMENT_3D('',#142621,#109361,#109362);
#96417=AXIS2_PLACEMENT_3D('',#142623,#109364,#109365);
#96418=AXIS2_PLACEMENT_3D('',#142625,#109366,#109367);
#96419=AXIS2_PLACEMENT_3D('',#142629,#109369,#109370);
#96420=AXIS2_PLACEMENT_3D('',#142635,#109373,#109374);
#96421=AXIS2_PLACEMENT_3D('',#142637,#109376,#109377);
#96422=AXIS2_PLACEMENT_3D('',#142657,#109379,#109380);
#96423=AXIS2_PLACEMENT_3D('',#142658,#109381,#109382);
#96424=AXIS2_PLACEMENT_3D('',#142662,#109384,#109385);
#96425=AXIS2_PLACEMENT_3D('',#142709,#109388,#109389);
#96426=AXIS2_PLACEMENT_3D('',#142726,#109392,#109393);
#96427=AXIS2_PLACEMENT_3D('',#142729,#109394,#109395);
#96428=AXIS2_PLACEMENT_3D('',#142733,#109397,#109398);
#96429=AXIS2_PLACEMENT_3D('',#142735,#109400,#109401);
#96430=AXIS2_PLACEMENT_3D('',#142738,#109402,#109403);
#96431=AXIS2_PLACEMENT_3D('',#142739,#109404,#109405);
#96432=AXIS2_PLACEMENT_3D('',#142740,#109406,#109407);
#96433=AXIS2_PLACEMENT_3D('',#142741,#109408,#109409);
#96434=AXIS2_PLACEMENT_3D('',#142744,#109410,#109411);
#96435=AXIS2_PLACEMENT_3D('',#142764,#109414,#109415);
#96436=AXIS2_PLACEMENT_3D('',#142765,#109416,#109417);
#96437=AXIS2_PLACEMENT_3D('',#142766,#109418,#109419);
#96438=AXIS2_PLACEMENT_3D('',#142767,#109420,#109421);
#96439=AXIS2_PLACEMENT_3D('',#142770,#109422,#109423);
#96440=AXIS2_PLACEMENT_3D('',#142771,#109424,#109425);
#96441=AXIS2_PLACEMENT_3D('',#142772,#109426,#109427);
#96442=AXIS2_PLACEMENT_3D('',#142790,#109428,#109429);
#96443=AXIS2_PLACEMENT_3D('',#142791,#109430,#109431);
#96444=AXIS2_PLACEMENT_3D('',#142792,#109432,#109433);
#96445=AXIS2_PLACEMENT_3D('',#142793,#109434,#109435);
#96446=AXIS2_PLACEMENT_3D('',#142796,#109436,#109437);
#96447=AXIS2_PLACEMENT_3D('',#142810,#109440,#109441);
#96448=AXIS2_PLACEMENT_3D('',#142811,#109442,#109443);
#96449=AXIS2_PLACEMENT_3D('',#142812,#109444,#109445);
#96450=AXIS2_PLACEMENT_3D('',#142813,#109446,#109447);
#96451=AXIS2_PLACEMENT_3D('',#142816,#109448,#109449);
#96452=AXIS2_PLACEMENT_3D('',#142818,#109450,#109451);
#96453=AXIS2_PLACEMENT_3D('',#142819,#109452,#109453);
#96454=AXIS2_PLACEMENT_3D('',#142820,#109454,#109455);
#96455=AXIS2_PLACEMENT_3D('',#142832,#109456,#109457);
#96456=AXIS2_PLACEMENT_3D('',#142833,#109458,#109459);
#96457=AXIS2_PLACEMENT_3D('',#142834,#109460,#109461);
#96458=AXIS2_PLACEMENT_3D('',#142835,#109462,#109463);
#96459=AXIS2_PLACEMENT_3D('',#142838,#109464,#109465);
#96460=AXIS2_PLACEMENT_3D('',#142856,#109468,#109469);
#96461=AXIS2_PLACEMENT_3D('',#142857,#109470,#109471);
#96462=AXIS2_PLACEMENT_3D('',#142858,#109472,#109473);
#96463=AXIS2_PLACEMENT_3D('',#142862,#109475,#109476);
#96464=AXIS2_PLACEMENT_3D('',#142864,#109478,#109479);
#96465=AXIS2_PLACEMENT_3D('',#142866,#109480,#109481);
#96466=AXIS2_PLACEMENT_3D('',#142871,#109484,#109485);
#96467=AXIS2_PLACEMENT_3D('',#142875,#109487,#109488);
#96468=AXIS2_PLACEMENT_3D('',#142879,#109490,#109491);
#96469=AXIS2_PLACEMENT_3D('',#142883,#109493,#109494);
#96470=AXIS2_PLACEMENT_3D('',#142886,#109496,#109497);
#96471=AXIS2_PLACEMENT_3D('',#142887,#109498,#109499);
#96472=AXIS2_PLACEMENT_3D('',#142890,#109501,#109502);
#96473=AXIS2_PLACEMENT_3D('',#142891,#109503,#109504);
#96474=AXIS2_PLACEMENT_3D('',#142895,#109507,#109508);
#96475=AXIS2_PLACEMENT_3D('',#142898,#109510,#109511);
#96476=AXIS2_PLACEMENT_3D('',#142899,#109512,#109513);
#96477=AXIS2_PLACEMENT_3D('',#142903,#109516,#109517);
#96478=AXIS2_PLACEMENT_3D('',#142904,#109518,#109519);
#96479=AXIS2_PLACEMENT_3D('',#142907,#109520,#109521);
#96480=AXIS2_PLACEMENT_3D('',#142909,#109522,#109523);
#96481=AXIS2_PLACEMENT_3D('',#142911,#109524,#109525);
#96482=AXIS2_PLACEMENT_3D('',#142937,#109526,#109527);
#96483=AXIS2_PLACEMENT_3D('',#142938,#109528,#109529);
#96484=AXIS2_PLACEMENT_3D('',#142939,#109530,#109531);
#96485=AXIS2_PLACEMENT_3D('',#142940,#109532,#109533);
#96486=AXIS2_PLACEMENT_3D('',#142943,#109534,#109535);
#96487=AXIS2_PLACEMENT_3D('',#142957,#109538,#109539);
#96488=AXIS2_PLACEMENT_3D('',#142958,#109540,#109541);
#96489=AXIS2_PLACEMENT_3D('',#142959,#109542,#109543);
#96490=AXIS2_PLACEMENT_3D('',#142960,#109544,#109545);
#96491=AXIS2_PLACEMENT_3D('',#142963,#109546,#109547);
#96492=AXIS2_PLACEMENT_3D('',#142976,#109550,#109551);
#96493=AXIS2_PLACEMENT_3D('',#142977,#109552,#109553);
#96494=AXIS2_PLACEMENT_3D('',#142978,#109554,#109555);
#96495=AXIS2_PLACEMENT_3D('',#142979,#109556,#109557);
#96496=AXIS2_PLACEMENT_3D('',#142981,#109558,#109559);
#96497=AXIS2_PLACEMENT_3D('',#142982,#109560,#109561);
#96498=AXIS2_PLACEMENT_3D('',#142994,#109562,#109563);
#96499=AXIS2_PLACEMENT_3D('',#142995,#109564,#109565);
#96500=AXIS2_PLACEMENT_3D('',#142996,#109566,#109567);
#96501=AXIS2_PLACEMENT_3D('',#142997,#109568,#109569);
#96502=AXIS2_PLACEMENT_3D('',#143000,#109570,#109571);
#96503=AXIS2_PLACEMENT_3D('',#143020,#109574,#109575);
#96504=AXIS2_PLACEMENT_3D('',#143021,#109576,#109577);
#96505=AXIS2_PLACEMENT_3D('',#143022,#109578,#109579);
#96506=AXIS2_PLACEMENT_3D('',#143023,#109580,#109581);
#96507=AXIS2_PLACEMENT_3D('',#143025,#109582,#109583);
#96508=AXIS2_PLACEMENT_3D('',#143027,#109584,#109585);
#96509=AXIS2_PLACEMENT_3D('',#143042,#109586,#109587);
#96510=AXIS2_PLACEMENT_3D('',#143045,#109588,#109589);
#96511=AXIS2_PLACEMENT_3D('',#143050,#109590,#109591);
#96512=AXIS2_PLACEMENT_3D('',#143057,#109592,#109593);
#96513=AXIS2_PLACEMENT_3D('',#143063,#109597,#109598);
#96514=AXIS2_PLACEMENT_3D('',#143066,#109600,#109601);
#96515=AXIS2_PLACEMENT_3D('',#143067,#109602,#109603);
#96516=AXIS2_PLACEMENT_3D('',#143096,#109604,#109605);
#96517=AXIS2_PLACEMENT_3D('',#143099,#109607,#109608);
#96518=AXIS2_PLACEMENT_3D('',#143103,#109610,#109611);
#96519=AXIS2_PLACEMENT_3D('',#143107,#109613,#109614);
#96520=AXIS2_PLACEMENT_3D('',#143165,#109615,#109616);
#96521=AXIS2_PLACEMENT_3D('',#143167,#109617,#109618);
#96522=AXIS2_PLACEMENT_3D('',#143171,#109620,#109621);
#96523=AXIS2_PLACEMENT_3D('',#143175,#109623,#109624);
#96524=AXIS2_PLACEMENT_3D('',#143177,#109626,#109627);
#96525=AXIS2_PLACEMENT_3D('',#143178,#109628,#109629);
#96526=AXIS2_PLACEMENT_3D('',#143181,#109630,#109631);
#96527=AXIS2_PLACEMENT_3D('',#143183,#109632,#109633);
#96528=AXIS2_PLACEMENT_3D('',#143185,#109634,#109635);
#96529=AXIS2_PLACEMENT_3D('',#143186,#109636,#109637);
#96530=AXIS2_PLACEMENT_3D('',#143204,#109638,#109639);
#96531=AXIS2_PLACEMENT_3D('',#143205,#109640,#109641);
#96532=AXIS2_PLACEMENT_3D('',#143206,#109642,#109643);
#96533=AXIS2_PLACEMENT_3D('',#143207,#109644,#109645);
#96534=AXIS2_PLACEMENT_3D('',#143210,#109646,#109647);
#96535=AXIS2_PLACEMENT_3D('',#143223,#109650,#109651);
#96536=AXIS2_PLACEMENT_3D('',#143224,#109652,#109653);
#96537=AXIS2_PLACEMENT_3D('',#143225,#109654,#109655);
#96538=AXIS2_PLACEMENT_3D('',#143226,#109656,#109657);
#96539=AXIS2_PLACEMENT_3D('',#143228,#109658,#109659);
#96540=AXIS2_PLACEMENT_3D('',#143229,#109660,#109661);
#96541=AXIS2_PLACEMENT_3D('',#143241,#109662,#109663);
#96542=AXIS2_PLACEMENT_3D('',#143242,#109664,#109665);
#96543=AXIS2_PLACEMENT_3D('',#143243,#109666,#109667);
#96544=AXIS2_PLACEMENT_3D('',#143244,#109668,#109669);
#96545=AXIS2_PLACEMENT_3D('',#143247,#109670,#109671);
#96546=AXIS2_PLACEMENT_3D('',#143261,#109674,#109675);
#96547=AXIS2_PLACEMENT_3D('',#143262,#109676,#109677);
#96548=AXIS2_PLACEMENT_3D('',#143263,#109678,#109679);
#96549=AXIS2_PLACEMENT_3D('',#143264,#109680,#109681);
#96550=AXIS2_PLACEMENT_3D('',#143267,#109682,#109683);
#96551=AXIS2_PLACEMENT_3D('',#143279,#109686,#109687);
#96552=AXIS2_PLACEMENT_3D('',#143280,#109688,#109689);
#96553=AXIS2_PLACEMENT_3D('',#143281,#109690,#109691);
#96554=AXIS2_PLACEMENT_3D('',#143287,#109695,#109696);
#96555=AXIS2_PLACEMENT_3D('',#143290,#109698,#109699);
#96556=AXIS2_PLACEMENT_3D('',#143291,#109700,#109701);
#96557=AXIS2_PLACEMENT_3D('',#143295,#109704,#109705);
#96558=AXIS2_PLACEMENT_3D('',#143298,#109707,#109708);
#96559=AXIS2_PLACEMENT_3D('',#143299,#109709,#109710);
#96560=AXIS2_PLACEMENT_3D('',#143303,#109712,#109713);
#96561=AXIS2_PLACEMENT_3D('',#143307,#109715,#109716);
#96562=AXIS2_PLACEMENT_3D('',#143311,#109718,#109719);
#96563=AXIS2_PLACEMENT_3D('',#143355,#109720,#109721);
#96564=AXIS2_PLACEMENT_3D('',#143358,#109723,#109724);
#96565=AXIS2_PLACEMENT_3D('',#143359,#109725,#109726);
#96566=AXIS2_PLACEMENT_3D('',#143360,#109727,#109728);
#96567=AXIS2_PLACEMENT_3D('',#143363,#109730,#109731);
#96568=AXIS2_PLACEMENT_3D('',#143364,#109732,#109733);
#96569=AXIS2_PLACEMENT_3D('',#143368,#109736,#109737);
#96570=AXIS2_PLACEMENT_3D('',#143369,#109738,#109739);
#96571=AXIS2_PLACEMENT_3D('',#143370,#109740,#109741);
#96572=AXIS2_PLACEMENT_3D('',#143373,#109743,#109744);
#96573=AXIS2_PLACEMENT_3D('',#143374,#109745,#109746);
#96574=AXIS2_PLACEMENT_3D('',#143375,#109747,#109748);
#96575=AXIS2_PLACEMENT_3D('',#143376,#109749,#109750);
#96576=AXIS2_PLACEMENT_3D('',#143379,#109751,#109752);
#96577=AXIS2_PLACEMENT_3D('',#143383,#109754,#109755);
#96578=AXIS2_PLACEMENT_3D('',#143385,#109757,#109758);
#96579=AXIS2_PLACEMENT_3D('',#143399,#109766,#109767);
#96580=AXIS2_PLACEMENT_3D('',#143405,#109771,#109772);
#96581=AXIS2_PLACEMENT_3D('',#143406,#109773,#109774);
#96582=AXIS2_PLACEMENT_3D('',#143407,#109775,#109776);
#96583=AXIS2_PLACEMENT_3D('',#143408,#109777,#109778);
#96584=AXIS2_PLACEMENT_3D('',#143411,#109780,#109781);
#96585=AXIS2_PLACEMENT_3D('',#143412,#109782,#109783);
#96586=AXIS2_PLACEMENT_3D('',#143414,#109784,#109785);
#96587=AXIS2_PLACEMENT_3D('',#143417,#109787,#109788);
#96588=AXIS2_PLACEMENT_3D('',#143418,#109789,#109790);
#96589=AXIS2_PLACEMENT_3D('',#143420,#109791,#109792);
#96590=AXIS2_PLACEMENT_3D('',#143423,#109794,#109795);
#96591=AXIS2_PLACEMENT_3D('',#143424,#109796,#109797);
#96592=AXIS2_PLACEMENT_3D('',#143426,#109798,#109799);
#96593=AXIS2_PLACEMENT_3D('',#143429,#109801,#109802);
#96594=AXIS2_PLACEMENT_3D('',#143430,#109803,#109804);
#96595=AXIS2_PLACEMENT_3D('',#143436,#109808,#109809);
#96596=AXIS2_PLACEMENT_3D('',#143438,#109810,#109811);
#96597=AXIS2_PLACEMENT_3D('',#143440,#109812,#109813);
#96598=AXIS2_PLACEMENT_3D('',#143442,#109815,#109816);
#96599=AXIS2_PLACEMENT_3D('',#143444,#109817,#109818);
#96600=AXIS2_PLACEMENT_3D('',#143446,#109819,#109820);
#96601=AXIS2_PLACEMENT_3D('',#143447,#109821,#109822);
#96602=AXIS2_PLACEMENT_3D('',#143449,#109823,#109824);
#96603=AXIS2_PLACEMENT_3D('',#143451,#109826,#109827);
#96604=AXIS2_PLACEMENT_3D('',#143453,#109828,#109829);
#96605=AXIS2_PLACEMENT_3D('',#143455,#109831,#109832);
#96606=AXIS2_PLACEMENT_3D('',#143473,#109842,#109843);
#96607=AXIS2_PLACEMENT_3D('',#143476,#109845,#109846);
#96608=AXIS2_PLACEMENT_3D('',#143477,#109847,#109848);
#96609=AXIS2_PLACEMENT_3D('',#143480,#109850,#109851);
#96610=AXIS2_PLACEMENT_3D('',#143481,#109852,#109853);
#96611=AXIS2_PLACEMENT_3D('',#143482,#109854,#109855);
#96612=AXIS2_PLACEMENT_3D('',#143483,#109856,#109857);
#96613=AXIS2_PLACEMENT_3D('',#143485,#109858,#109859);
#96614=AXIS2_PLACEMENT_3D('',#143488,#109861,#109862);
#96615=AXIS2_PLACEMENT_3D('',#143489,#109863,#109864);
#96616=AXIS2_PLACEMENT_3D('',#143492,#109865,#109866);
#96617=AXIS2_PLACEMENT_3D('',#143496,#109868,#109869);
#96618=AXIS2_PLACEMENT_3D('',#143498,#109871,#109872);
#96619=AXIS2_PLACEMENT_3D('',#143504,#109876,#109877);
#96620=AXIS2_PLACEMENT_3D('',#143507,#109879,#109880);
#96621=AXIS2_PLACEMENT_3D('',#143508,#109881,#109882);
#96622=AXIS2_PLACEMENT_3D('',#143514,#109886,#109887);
#96623=AXIS2_PLACEMENT_3D('',#143516,#109888,#109889);
#96624=AXIS2_PLACEMENT_3D('',#143519,#109891,#109892);
#96625=AXIS2_PLACEMENT_3D('',#143520,#109893,#109894);
#96626=AXIS2_PLACEMENT_3D('',#143523,#109895,#109896);
#96627=AXIS2_PLACEMENT_3D('',#143527,#109898,#109899);
#96628=AXIS2_PLACEMENT_3D('',#143529,#109901,#109902);
#96629=AXIS2_PLACEMENT_3D('',#143530,#109903,#109904);
#96630=AXIS2_PLACEMENT_3D('',#143531,#109905,#109906);
#96631=AXIS2_PLACEMENT_3D('',#143532,#109907,#109908);
#96632=AXIS2_PLACEMENT_3D('',#143534,#109909,#109910);
#96633=AXIS2_PLACEMENT_3D('',#143537,#109912,#109913);
#96634=AXIS2_PLACEMENT_3D('',#143538,#109914,#109915);
#96635=AXIS2_PLACEMENT_3D('',#143540,#109916,#109917);
#96636=AXIS2_PLACEMENT_3D('',#143543,#109919,#109920);
#96637=AXIS2_PLACEMENT_3D('',#143544,#109921,#109922);
#96638=AXIS2_PLACEMENT_3D('',#143549,#109924,#109925);
#96639=AXIS2_PLACEMENT_3D('',#143552,#109927,#109928);
#96640=AXIS2_PLACEMENT_3D('',#143553,#109929,#109930);
#96641=AXIS2_PLACEMENT_3D('',#143596,#109933,#109934);
#96642=AXIS2_PLACEMENT_3D('',#143619,#109937,#109938);
#96643=AXIS2_PLACEMENT_3D('',#143621,#109939,#109940);
#96644=AXIS2_PLACEMENT_3D('',#143624,#109942,#109943);
#96645=AXIS2_PLACEMENT_3D('',#143625,#109944,#109945);
#96646=AXIS2_PLACEMENT_3D('',#143629,#109947,#109948);
#96647=AXIS2_PLACEMENT_3D('',#143631,#109949,#109950);
#96648=AXIS2_PLACEMENT_3D('',#143632,#109951,#109952);
#96649=AXIS2_PLACEMENT_3D('',#143634,#109954,#109955);
#96650=AXIS2_PLACEMENT_3D('',#143636,#109956,#109957);
#96651=AXIS2_PLACEMENT_3D('',#143639,#109959,#109960);
#96652=AXIS2_PLACEMENT_3D('',#143640,#109961,#109962);
#96653=AXIS2_PLACEMENT_3D('',#143644,#109964,#109965);
#96654=AXIS2_PLACEMENT_3D('',#143646,#109966,#109967);
#96655=AXIS2_PLACEMENT_3D('',#143647,#109968,#109969);
#96656=AXIS2_PLACEMENT_3D('',#143649,#109971,#109972);
#96657=AXIS2_PLACEMENT_3D('',#143656,#109973,#109974);
#96658=AXIS2_PLACEMENT_3D('',#143659,#109975,#109976);
#96659=AXIS2_PLACEMENT_3D('',#143665,#109979,#109980);
#96660=AXIS2_PLACEMENT_3D('',#143669,#109983,#109984);
#96661=AXIS2_PLACEMENT_3D('',#143672,#109985,#109986);
#96662=AXIS2_PLACEMENT_3D('',#143678,#109989,#109990);
#96663=AXIS2_PLACEMENT_3D('',#143682,#109993,#109994);
#96664=AXIS2_PLACEMENT_3D('',#143688,#109998,#109999);
#96665=AXIS2_PLACEMENT_3D('',#143690,#110000,#110001);
#96666=AXIS2_PLACEMENT_3D('',#143692,#110002,#110003);
#96667=AXIS2_PLACEMENT_3D('',#143694,#110005,#110006);
#96668=AXIS2_PLACEMENT_3D('',#143698,#110009,#110010);
#96669=AXIS2_PLACEMENT_3D('',#143704,#110014,#110015);
#96670=AXIS2_PLACEMENT_3D('',#143706,#110016,#110017);
#96671=AXIS2_PLACEMENT_3D('',#143708,#110018,#110019);
#96672=AXIS2_PLACEMENT_3D('',#143710,#110021,#110022);
#96673=AXIS2_PLACEMENT_3D('',#143714,#110025,#110026);
#96674=AXIS2_PLACEMENT_3D('',#143715,#110027,#110028);
#96675=AXIS2_PLACEMENT_3D('',#143717,#110029,#110030);
#96676=AXIS2_PLACEMENT_3D('',#143718,#110031,#110032);
#96677=AXIS2_PLACEMENT_3D('',#143719,#110033,#110034);
#96678=AXIS2_PLACEMENT_3D('',#143720,#110035,#110036);
#96679=AXIS2_PLACEMENT_3D('',#143721,#110037,#110038);
#96680=AXIS2_PLACEMENT_3D('',#143723,#110039,#110040);
#96681=AXIS2_PLACEMENT_3D('',#143724,#110041,#110042);
#96682=AXIS2_PLACEMENT_3D('',#143725,#110043,#110044);
#96683=AXIS2_PLACEMENT_3D('',#143726,#110045,#110046);
#96684=AXIS2_PLACEMENT_3D('',#143737,#110050,#110051);
#96685=AXIS2_PLACEMENT_3D('',#143739,#110052,#110053);
#96686=AXIS2_PLACEMENT_3D('',#143741,#110054,#110055);
#96687=AXIS2_PLACEMENT_3D('',#143743,#110057,#110058);
#96688=AXIS2_PLACEMENT_3D('',#143751,#110061,#110062);
#96689=AXIS2_PLACEMENT_3D('',#143758,#110063,#110064);
#96690=AXIS2_PLACEMENT_3D('',#143769,#110068,#110069);
#96691=AXIS2_PLACEMENT_3D('',#143771,#110070,#110071);
#96692=AXIS2_PLACEMENT_3D('',#143773,#110072,#110073);
#96693=AXIS2_PLACEMENT_3D('',#143775,#110075,#110076);
#96694=AXIS2_PLACEMENT_3D('',#143783,#110079,#110080);
#96695=AXIS2_PLACEMENT_3D('',#143790,#110081,#110082);
#96696=AXIS2_PLACEMENT_3D('',#143796,#110086,#110087);
#96697=AXIS2_PLACEMENT_3D('',#143799,#110090,#110091);
#96698=AXIS2_PLACEMENT_3D('',#143828,#110094,#110095);
#96699=AXIS2_PLACEMENT_3D('',#143829,#110096,#110097);
#96700=AXIS2_PLACEMENT_3D('',#143835,#110101,#110102);
#96701=AXIS2_PLACEMENT_3D('',#143838,#110103,#110104);
#96702=AXIS2_PLACEMENT_3D('',#143857,#110107,#110108);
#96703=AXIS2_PLACEMENT_3D('',#143864,#110111,#110112);
#96704=AXIS2_PLACEMENT_3D('',#143866,#110114,#110115);
#96705=AXIS2_PLACEMENT_3D('',#143872,#110119,#110120);
#96706=AXIS2_PLACEMENT_3D('',#143896,#110122,#110123);
#96707=AXIS2_PLACEMENT_3D('',#143897,#110124,#110125);
#96708=AXIS2_PLACEMENT_3D('',#143899,#110126,#110127);
#96709=AXIS2_PLACEMENT_3D('',#143901,#110128,#110129);
#96710=AXIS2_PLACEMENT_3D('',#143902,#110130,#110131);
#96711=AXIS2_PLACEMENT_3D('',#143904,#110132,#110133);
#96712=AXIS2_PLACEMENT_3D('',#143906,#110135,#110136);
#96713=AXIS2_PLACEMENT_3D('',#143933,#110137,#110138);
#96714=AXIS2_PLACEMENT_3D('',#143934,#110139,#110140);
#96715=AXIS2_PLACEMENT_3D('',#143938,#110143,#110144);
#96716=AXIS2_PLACEMENT_3D('',#143941,#110146,#110147);
#96717=AXIS2_PLACEMENT_3D('',#143942,#110148,#110149);
#96718=AXIS2_PLACEMENT_3D('',#143946,#110152,#110153);
#96719=AXIS2_PLACEMENT_3D('',#143947,#110154,#110155);
#96720=AXIS2_PLACEMENT_3D('',#143976,#110157,#110158);
#96721=AXIS2_PLACEMENT_3D('',#143978,#110159,#110160);
#96722=AXIS2_PLACEMENT_3D('',#143981,#110162,#110163);
#96723=AXIS2_PLACEMENT_3D('',#143982,#110164,#110165);
#96724=AXIS2_PLACEMENT_3D('',#143984,#110166,#110167);
#96725=AXIS2_PLACEMENT_3D('',#143985,#110168,#110169);
#96726=AXIS2_PLACEMENT_3D('',#143986,#110170,#110171);
#96727=AXIS2_PLACEMENT_3D('',#143987,#110172,#110173);
#96728=AXIS2_PLACEMENT_3D('',#143988,#110174,#110175);
#96729=AXIS2_PLACEMENT_3D('',#143990,#110176,#110177);
#96730=AXIS2_PLACEMENT_3D('',#143992,#110179,#110180);
#96731=AXIS2_PLACEMENT_3D('',#144003,#110181,#110182);
#96732=AXIS2_PLACEMENT_3D('',#144005,#110184,#110185);
#96733=AXIS2_PLACEMENT_3D('',#144011,#110189,#110190);
#96734=AXIS2_PLACEMENT_3D('',#144032,#110192,#110193);
#96735=AXIS2_PLACEMENT_3D('',#144038,#110197,#110198);
#96736=AXIS2_PLACEMENT_3D('',#144050,#110199,#110200);
#96737=AXIS2_PLACEMENT_3D('',#144051,#110201,#110202);
#96738=AXIS2_PLACEMENT_3D('',#144052,#110203,#110204);
#96739=AXIS2_PLACEMENT_3D('',#144053,#110205,#110206);
#96740=AXIS2_PLACEMENT_3D('',#144057,#110209,#110210);
#96741=AXIS2_PLACEMENT_3D('',#144058,#110211,#110212);
#96742=AXIS2_PLACEMENT_3D('',#144060,#110213,#110214);
#96743=AXIS2_PLACEMENT_3D('',#144084,#110216,#110217);
#96744=AXIS2_PLACEMENT_3D('',#144085,#110218,#110219);
#96745=AXIS2_PLACEMENT_3D('',#144087,#110221,#110222);
#96746=AXIS2_PLACEMENT_3D('',#144099,#110223,#110224);
#96747=AXIS2_PLACEMENT_3D('',#144100,#110225,#110226);
#96748=AXIS2_PLACEMENT_3D('',#144101,#110227,#110228);
#96749=AXIS2_PLACEMENT_3D('',#144102,#110229,#110230);
#96750=AXIS2_PLACEMENT_3D('',#144104,#110232,#110233);
#96751=AXIS2_PLACEMENT_3D('',#144106,#110235,#110236);
#96752=AXIS2_PLACEMENT_3D('',#144108,#110238,#110239);
#96753=AXIS2_PLACEMENT_3D('',#144110,#110241,#110242);
#96754=AXIS2_PLACEMENT_3D('',#144115,#110247,#110248);
#96755=AXIS2_PLACEMENT_3D('',#144134,#110250,#110251);
#96756=AXIS2_PLACEMENT_3D('',#144136,#110253,#110254);
#96757=AXIS2_PLACEMENT_3D('',#144152,#110256,#110257);
#96758=AXIS2_PLACEMENT_3D('',#144153,#110258,#110259);
#96759=AXIS2_PLACEMENT_3D('',#144168,#110260,#110261);
#96760=AXIS2_PLACEMENT_3D('',#144200,#110262,#110263);
#96761=AXIS2_PLACEMENT_3D('',#144201,#110264,#110265);
#96762=AXIS2_PLACEMENT_3D('',#144206,#110267,#110268);
#96763=AXIS2_PLACEMENT_3D('',#144223,#110269,#110270);
#96764=AXIS2_PLACEMENT_3D('',#144224,#110271,#110272);
#96765=AXIS2_PLACEMENT_3D('',#144225,#110273,#110274);
#96766=AXIS2_PLACEMENT_3D('',#144226,#110275,#110276);
#96767=AXIS2_PLACEMENT_3D('',#144227,#110277,#110278);
#96768=AXIS2_PLACEMENT_3D('',#144229,#110280,#110281);
#96769=AXIS2_PLACEMENT_3D('',#144246,#110283,#110284);
#96770=AXIS2_PLACEMENT_3D('',#144268,#110286,#110287);
#96771=AXIS2_PLACEMENT_3D('',#144270,#110289,#110290);
#96772=AXIS2_PLACEMENT_3D('',#144272,#110291,#110292);
#96773=AXIS2_PLACEMENT_3D('',#144306,#110294,#110295);
#96774=AXIS2_PLACEMENT_3D('',#144323,#110296,#110297);
#96775=AXIS2_PLACEMENT_3D('',#144325,#110299,#110300);
#96776=AXIS2_PLACEMENT_3D('',#144344,#110301,#110302);
#96777=AXIS2_PLACEMENT_3D('',#144345,#110303,#110304);
#96778=AXIS2_PLACEMENT_3D('',#144347,#110305,#110306);
#96779=AXIS2_PLACEMENT_3D('',#144350,#110308,#110309);
#96780=AXIS2_PLACEMENT_3D('',#144351,#110310,#110311);
#96781=AXIS2_PLACEMENT_3D('',#144353,#110312,#110313);
#96782=AXIS2_PLACEMENT_3D('',#144354,#110314,#110315);
#96783=AXIS2_PLACEMENT_3D('',#144357,#110317,#110318);
#96784=AXIS2_PLACEMENT_3D('',#144358,#110319,#110320);
#96785=AXIS2_PLACEMENT_3D('',#144361,#110322,#110323);
#96786=AXIS2_PLACEMENT_3D('',#144362,#110324,#110325);
#96787=AXIS2_PLACEMENT_3D('',#144364,#110326,#110327);
#96788=AXIS2_PLACEMENT_3D('',#144367,#110329,#110330);
#96789=AXIS2_PLACEMENT_3D('',#144368,#110331,#110332);
#96790=AXIS2_PLACEMENT_3D('',#144379,#110333,#110334);
#96791=AXIS2_PLACEMENT_3D('',#144381,#110335,#110336);
#96792=AXIS2_PLACEMENT_3D('',#144384,#110338,#110339);
#96793=AXIS2_PLACEMENT_3D('',#144385,#110340,#110341);
#96794=AXIS2_PLACEMENT_3D('',#144401,#110343,#110344);
#96795=AXIS2_PLACEMENT_3D('',#144403,#110345,#110346);
#96796=AXIS2_PLACEMENT_3D('',#144406,#110348,#110349);
#96797=AXIS2_PLACEMENT_3D('',#144407,#110350,#110351);
#96798=AXIS2_PLACEMENT_3D('',#144410,#110353,#110354);
#96799=AXIS2_PLACEMENT_3D('',#144411,#110355,#110356);
#96800=AXIS2_PLACEMENT_3D('',#144414,#110357,#110358);
#96801=AXIS2_PLACEMENT_3D('',#144418,#110360,#110361);
#96802=AXIS2_PLACEMENT_3D('',#144420,#110363,#110364);
#96803=AXIS2_PLACEMENT_3D('',#144425,#110366,#110367);
#96804=AXIS2_PLACEMENT_3D('',#144428,#110369,#110370);
#96805=AXIS2_PLACEMENT_3D('',#144429,#110371,#110372);
#96806=AXIS2_PLACEMENT_3D('',#144433,#110374,#110375);
#96807=AXIS2_PLACEMENT_3D('',#144434,#110376,#110377);
#96808=AXIS2_PLACEMENT_3D('',#144435,#110378,#110379);
#96809=AXIS2_PLACEMENT_3D('',#144438,#110381,#110382);
#96810=AXIS2_PLACEMENT_3D('',#144439,#110383,#110384);
#96811=AXIS2_PLACEMENT_3D('',#144443,#110387,#110388);
#96812=AXIS2_PLACEMENT_3D('',#144445,#110389,#110390);
#96813=AXIS2_PLACEMENT_3D('',#144447,#110392,#110393);
#96814=AXIS2_PLACEMENT_3D('',#144451,#110395,#110396);
#96815=AXIS2_PLACEMENT_3D('',#144471,#110399,#110400);
#96816=AXIS2_PLACEMENT_3D('',#144473,#110401,#110402);
#96817=AXIS2_PLACEMENT_3D('',#144476,#110404,#110405);
#96818=AXIS2_PLACEMENT_3D('',#144477,#110406,#110407);
#96819=AXIS2_PLACEMENT_3D('',#144481,#110410,#110411);
#96820=AXIS2_PLACEMENT_3D('',#144496,#110413,#110414);
#96821=AXIS2_PLACEMENT_3D('',#144497,#110415,#110416);
#96822=AXIS2_PLACEMENT_3D('',#144499,#110417,#110418);
#96823=AXIS2_PLACEMENT_3D('',#144501,#110420,#110421);
#96824=AXIS2_PLACEMENT_3D('',#144503,#110423,#110424);
#96825=AXIS2_PLACEMENT_3D('',#144504,#110425,#110426);
#96826=AXIS2_PLACEMENT_3D('',#144508,#110428,#110429);
#96827=AXIS2_PLACEMENT_3D('',#144513,#110430,#110431);
#96828=AXIS2_PLACEMENT_3D('',#144514,#110432,#110433);
#96829=AXIS2_PLACEMENT_3D('',#144515,#110434,#110435);
#96830=AXIS2_PLACEMENT_3D('',#144517,#110436,#110437);
#96831=AXIS2_PLACEMENT_3D('',#144518,#110438,#110439);
#96832=AXIS2_PLACEMENT_3D('',#144520,#110440,#110441);
#96833=AXIS2_PLACEMENT_3D('',#144522,#110442,#110443);
#96834=AXIS2_PLACEMENT_3D('',#144523,#110444,#110445);
#96835=AXIS2_PLACEMENT_3D('',#144526,#110447,#110448);
#96836=AXIS2_PLACEMENT_3D('',#144527,#110449,#110450);
#96837=AXIS2_PLACEMENT_3D('',#144530,#110452,#110453);
#96838=AXIS2_PLACEMENT_3D('',#144531,#110454,#110455);
#96839=AXIS2_PLACEMENT_3D('',#144532,#110456,#110457);
#96840=AXIS2_PLACEMENT_3D('',#144533,#110458,#110459);
#96841=AXIS2_PLACEMENT_3D('',#144539,#110460,#110461);
#96842=AXIS2_PLACEMENT_3D('',#144540,#110462,#110463);
#96843=AXIS2_PLACEMENT_3D('',#144541,#110464,#110465);
#96844=AXIS2_PLACEMENT_3D('',#144542,#110466,#110467);
#96845=AXIS2_PLACEMENT_3D('',#144543,#110468,#110469);
#96846=AXIS2_PLACEMENT_3D('',#144544,#110470,#110471);
#96847=AXIS2_PLACEMENT_3D('',#144546,#110472,#110473);
#96848=AXIS2_PLACEMENT_3D('',#144548,#110475,#110476);
#96849=AXIS2_PLACEMENT_3D('',#144549,#110477,#110478);
#96850=AXIS2_PLACEMENT_3D('',#144551,#110480,#110481);
#96851=AXIS2_PLACEMENT_3D('',#144553,#110482,#110483);
#96852=AXIS2_PLACEMENT_3D('',#144555,#110484,#110485);
#96853=AXIS2_PLACEMENT_3D('',#144556,#110486,#110487);
#96854=AXIS2_PLACEMENT_3D('',#144559,#110488,#110489);
#96855=AXIS2_PLACEMENT_3D('',#144561,#110491,#110492);
#96856=AXIS2_PLACEMENT_3D('',#144562,#110493,#110494);
#96857=AXIS2_PLACEMENT_3D('',#144564,#110495,#110496);
#96858=AXIS2_PLACEMENT_3D('',#144571,#110497,#110498);
#96859=AXIS2_PLACEMENT_3D('',#144593,#110499,#110500);
#96860=AXIS2_PLACEMENT_3D('',#144594,#110501,#110502);
#96861=AXIS2_PLACEMENT_3D('',#144613,#110503,#110504);
#96862=AXIS2_PLACEMENT_3D('',#144614,#110505,#110506);
#96863=AXIS2_PLACEMENT_3D('',#144616,#110508,#110509);
#96864=AXIS2_PLACEMENT_3D('',#144628,#110510,#110511);
#96865=AXIS2_PLACEMENT_3D('',#144629,#110512,#110513);
#96866=AXIS2_PLACEMENT_3D('',#144630,#110514,#110515);
#96867=AXIS2_PLACEMENT_3D('',#144631,#110516,#110517);
#96868=AXIS2_PLACEMENT_3D('',#144632,#110518,#110519);
#96869=AXIS2_PLACEMENT_3D('',#144633,#110520,#110521);
#96870=AXIS2_PLACEMENT_3D('',#144634,#110522,#110523);
#96871=AXIS2_PLACEMENT_3D('',#144635,#110524,#110525);
#96872=AXIS2_PLACEMENT_3D('',#144639,#110526,#110527);
#96873=AXIS2_PLACEMENT_3D('',#144640,#110528,#110529);
#96874=AXIS2_PLACEMENT_3D('',#144641,#110530,#110531);
#96875=AXIS2_PLACEMENT_3D('',#144642,#110532,#110533);
#96876=AXIS2_PLACEMENT_3D('',#144646,#110535,#110536);
#96877=AXIS2_PLACEMENT_3D('',#144648,#110538,#110539);
#96878=AXIS2_PLACEMENT_3D('',#144684,#110540,#110541);
#96879=AXIS2_PLACEMENT_3D('',#144685,#110542,#110543);
#96880=AXIS2_PLACEMENT_3D('',#144694,#110548,#110549);
#96881=AXIS2_PLACEMENT_3D('',#144702,#110553,#110554);
#96882=AXIS2_PLACEMENT_3D('',#144703,#110555,#110556);
#96883=AXIS2_PLACEMENT_3D('',#144709,#110557,#110558);
#96884=AXIS2_PLACEMENT_3D('',#144710,#110559,#110560);
#96885=AXIS2_PLACEMENT_3D('',#144712,#110561,#110562);
#96886=AXIS2_PLACEMENT_3D('',#144713,#110563,#110564);
#96887=AXIS2_PLACEMENT_3D('',#144714,#110565,#110566);
#96888=AXIS2_PLACEMENT_3D('',#144717,#110567,#110568);
#96889=AXIS2_PLACEMENT_3D('',#144738,#110571,#110572);
#96890=AXIS2_PLACEMENT_3D('',#144739,#110573,#110574);
#96891=AXIS2_PLACEMENT_3D('',#144740,#110575,#110576);
#96892=AXIS2_PLACEMENT_3D('',#144741,#110577,#110578);
#96893=AXIS2_PLACEMENT_3D('',#144742,#110579,#110580);
#96894=AXIS2_PLACEMENT_3D('',#144743,#110581,#110582);
#96895=AXIS2_PLACEMENT_3D('',#144744,#110583,#110584);
#96896=AXIS2_PLACEMENT_3D('',#144745,#110585,#110586);
#96897=AXIS2_PLACEMENT_3D('',#144746,#110587,#110588);
#96898=AXIS2_PLACEMENT_3D('',#144747,#110589,#110590);
#96899=AXIS2_PLACEMENT_3D('',#144748,#110591,#110592);
#96900=AXIS2_PLACEMENT_3D('',#144749,#110593,#110594);
#96901=AXIS2_PLACEMENT_3D('',#144775,#110595,#110596);
#96902=AXIS2_PLACEMENT_3D('',#144776,#110597,#110598);
#96903=AXIS2_PLACEMENT_3D('',#144777,#110599,#110600);
#96904=AXIS2_PLACEMENT_3D('',#144778,#110601,#110602);
#96905=AXIS2_PLACEMENT_3D('',#144779,#110603,#110604);
#96906=AXIS2_PLACEMENT_3D('',#144794,#110606,#110607);
#96907=AXIS2_PLACEMENT_3D('',#144795,#110608,#110609);
#96908=AXIS2_PLACEMENT_3D('',#144809,#110610,#110611);
#96909=AXIS2_PLACEMENT_3D('',#144812,#110613,#110614);
#96910=AXIS2_PLACEMENT_3D('',#144822,#110616,#110617);
#96911=AXIS2_PLACEMENT_3D('',#144836,#110618,#110619);
#96912=AXIS2_PLACEMENT_3D('',#144911,#110620,#110621);
#96913=AXIS2_PLACEMENT_3D('',#144912,#110622,#110623);
#96914=AXIS2_PLACEMENT_3D('',#144913,#110624,#110625);
#96915=AXIS2_PLACEMENT_3D('',#144914,#110626,#110627);
#96916=AXIS2_PLACEMENT_3D('',#144915,#110628,#110629);
#96917=AXIS2_PLACEMENT_3D('',#144921,#110633,#110634);
#96918=AXIS2_PLACEMENT_3D('',#144922,#110635,#110636);
#96919=AXIS2_PLACEMENT_3D('',#144923,#110637,#110638);
#96920=AXIS2_PLACEMENT_3D('',#144926,#110640,#110641);
#96921=AXIS2_PLACEMENT_3D('',#144927,#110642,#110643);
#96922=AXIS2_PLACEMENT_3D('',#144928,#110644,#110645);
#96923=AXIS2_PLACEMENT_3D('',#144929,#110646,#110647);
#96924=AXIS2_PLACEMENT_3D('',#144937,#110652,#110653);
#96925=AXIS2_PLACEMENT_3D('',#144939,#110654,#110655);
#96926=AXIS2_PLACEMENT_3D('',#144942,#110657,#110658);
#96927=AXIS2_PLACEMENT_3D('',#144943,#110659,#110660);
#96928=AXIS2_PLACEMENT_3D('',#144946,#110661,#110662);
#96929=AXIS2_PLACEMENT_3D('',#144950,#110664,#110665);
#96930=AXIS2_PLACEMENT_3D('',#144952,#110667,#110668);
#96931=AXIS2_PLACEMENT_3D('',#144958,#110672,#110673);
#96932=AXIS2_PLACEMENT_3D('',#144960,#110674,#110675);
#96933=AXIS2_PLACEMENT_3D('',#144963,#110677,#110678);
#96934=AXIS2_PLACEMENT_3D('',#144964,#110679,#110680);
#96935=AXIS2_PLACEMENT_3D('',#144970,#110681,#110682);
#96936=AXIS2_PLACEMENT_3D('',#144978,#110683,#110684);
#96937=AXIS2_PLACEMENT_3D('',#144979,#110685,#110686);
#96938=AXIS2_PLACEMENT_3D('',#144980,#110687,#110688);
#96939=AXIS2_PLACEMENT_3D('',#144983,#110690,#110691);
#96940=AXIS2_PLACEMENT_3D('',#144984,#110692,#110693);
#96941=AXIS2_PLACEMENT_3D('',#144987,#110695,#110696);
#96942=AXIS2_PLACEMENT_3D('',#144988,#110697,#110698);
#96943=AXIS2_PLACEMENT_3D('',#144989,#110699,#110700);
#96944=AXIS2_PLACEMENT_3D('',#144990,#110701,#110702);
#96945=AXIS2_PLACEMENT_3D('',#144994,#110705,#110706);
#96946=AXIS2_PLACEMENT_3D('',#144995,#110707,#110708);
#96947=AXIS2_PLACEMENT_3D('',#144996,#110709,#110710);
#96948=AXIS2_PLACEMENT_3D('',#145005,#110715,#110716);
#96949=AXIS2_PLACEMENT_3D('',#145006,#110717,#110718);
#96950=AXIS2_PLACEMENT_3D('',#145007,#110719,#110720);
#96951=AXIS2_PLACEMENT_3D('',#145008,#110721,#110722);
#96952=AXIS2_PLACEMENT_3D('',#145022,#110730,#110731);
#96953=AXIS2_PLACEMENT_3D('',#145024,#110732,#110733);
#96954=AXIS2_PLACEMENT_3D('',#145026,#110735,#110736);
#96955=AXIS2_PLACEMENT_3D('',#145030,#110739,#110740);
#96956=AXIS2_PLACEMENT_3D('',#145031,#110741,#110742);
#96957=AXIS2_PLACEMENT_3D('',#145032,#110743,#110744);
#96958=AXIS2_PLACEMENT_3D('',#145035,#110745,#110746);
#96959=AXIS2_PLACEMENT_3D('',#145037,#110748,#110749);
#96960=AXIS2_PLACEMENT_3D('',#145040,#110752,#110753);
#96961=AXIS2_PLACEMENT_3D('',#145044,#110756,#110757);
#96962=AXIS2_PLACEMENT_3D('',#145046,#110758,#110759);
#96963=AXIS2_PLACEMENT_3D('',#145048,#110761,#110762);
#96964=AXIS2_PLACEMENT_3D('',#145051,#110764,#110765);
#96965=AXIS2_PLACEMENT_3D('',#145052,#110766,#110767);
#96966=AXIS2_PLACEMENT_3D('',#145056,#110769,#110770);
#96967=AXIS2_PLACEMENT_3D('',#145057,#110771,#110772);
#96968=AXIS2_PLACEMENT_3D('',#145058,#110773,#110774);
#96969=AXIS2_PLACEMENT_3D('',#145060,#110775,#110776);
#96970=AXIS2_PLACEMENT_3D('',#145063,#110778,#110779);
#96971=AXIS2_PLACEMENT_3D('',#145064,#110780,#110781);
#96972=AXIS2_PLACEMENT_3D('',#145065,#110782,#110783);
#96973=AXIS2_PLACEMENT_3D('',#145068,#110785,#110786);
#96974=AXIS2_PLACEMENT_3D('',#145069,#110787,#110788);
#96975=AXIS2_PLACEMENT_3D('',#145078,#110789,#110790);
#96976=AXIS2_PLACEMENT_3D('',#145080,#110791,#110792);
#96977=AXIS2_PLACEMENT_3D('',#145083,#110794,#110795);
#96978=AXIS2_PLACEMENT_3D('',#145084,#110796,#110797);
#96979=AXIS2_PLACEMENT_3D('',#145085,#110798,#110799);
#96980=AXIS2_PLACEMENT_3D('',#145086,#110800,#110801);
#96981=AXIS2_PLACEMENT_3D('',#145087,#110802,#110803);
#96982=AXIS2_PLACEMENT_3D('',#145090,#110804,#110805);
#96983=AXIS2_PLACEMENT_3D('',#145091,#110806,#110807);
#96984=AXIS2_PLACEMENT_3D('',#145093,#110809,#110810);
#96985=AXIS2_PLACEMENT_3D('',#145095,#110811,#110812);
#96986=AXIS2_PLACEMENT_3D('',#145096,#110813,#110814);
#96987=AXIS2_PLACEMENT_3D('',#145097,#110815,#110816);
#96988=AXIS2_PLACEMENT_3D('',#145099,#110818,#110819);
#96989=AXIS2_PLACEMENT_3D('',#145105,#110823,#110824);
#96990=AXIS2_PLACEMENT_3D('',#145107,#110825,#110826);
#96991=AXIS2_PLACEMENT_3D('',#145110,#110828,#110829);
#96992=AXIS2_PLACEMENT_3D('',#145112,#110830,#110831);
#96993=AXIS2_PLACEMENT_3D('',#145116,#110833,#110834);
#96994=AXIS2_PLACEMENT_3D('',#145118,#110836,#110837);
#96995=AXIS2_PLACEMENT_3D('',#145120,#110838,#110839);
#96996=AXIS2_PLACEMENT_3D('',#145123,#110841,#110842);
#96997=AXIS2_PLACEMENT_3D('',#145125,#110843,#110844);
#96998=AXIS2_PLACEMENT_3D('',#145129,#110846,#110847);
#96999=AXIS2_PLACEMENT_3D('',#145132,#110849,#110850);
#97000=AXIS2_PLACEMENT_3D('',#145134,#110851,#110852);
#97001=AXIS2_PLACEMENT_3D('',#145135,#110853,#110854);
#97002=AXIS2_PLACEMENT_3D('',#145136,#110855,#110856);
#97003=AXIS2_PLACEMENT_3D('',#145137,#110857,#110858);
#97004=AXIS2_PLACEMENT_3D('',#145138,#110859,#110860);
#97005=AXIS2_PLACEMENT_3D('',#145139,#110861,#110862);
#97006=AXIS2_PLACEMENT_3D('',#145140,#110863,#110864);
#97007=AXIS2_PLACEMENT_3D('',#145141,#110865,#110866);
#97008=AXIS2_PLACEMENT_3D('',#145143,#110868,#110869);
#97009=AXIS2_PLACEMENT_3D('',#145145,#110870,#110871);
#97010=AXIS2_PLACEMENT_3D('',#145147,#110872,#110873);
#97011=AXIS2_PLACEMENT_3D('',#145150,#110875,#110876);
#97012=AXIS2_PLACEMENT_3D('',#145151,#110877,#110878);
#97013=AXIS2_PLACEMENT_3D('',#145160,#110883,#110884);
#97014=AXIS2_PLACEMENT_3D('',#145169,#110889,#110890);
#97015=AXIS2_PLACEMENT_3D('',#145170,#110891,#110892);
#97016=AXIS2_PLACEMENT_3D('',#145171,#110893,#110894);
#97017=AXIS2_PLACEMENT_3D('',#145172,#110895,#110896);
#97018=AXIS2_PLACEMENT_3D('',#145173,#110897,#110898);
#97019=AXIS2_PLACEMENT_3D('',#145176,#110901,#110902);
#97020=AXIS2_PLACEMENT_3D('',#145177,#110903,#110904);
#97021=AXIS2_PLACEMENT_3D('',#145182,#110905,#110906);
#97022=AXIS2_PLACEMENT_3D('',#145183,#110907,#110908);
#97023=AXIS2_PLACEMENT_3D('',#145184,#110909,#110910);
#97024=AXIS2_PLACEMENT_3D('',#145185,#110911,#110912);
#97025=AXIS2_PLACEMENT_3D('',#145186,#110913,#110914);
#97026=AXIS2_PLACEMENT_3D('',#145187,#110915,#110916);
#97027=AXIS2_PLACEMENT_3D('',#145188,#110917,#110918);
#97028=AXIS2_PLACEMENT_3D('',#145189,#110919,#110920);
#97029=AXIS2_PLACEMENT_3D('',#145190,#110921,#110922);
#97030=AXIS2_PLACEMENT_3D('',#145191,#110923,#110924);
#97031=AXIS2_PLACEMENT_3D('',#145192,#110925,#110926);
#97032=AXIS2_PLACEMENT_3D('',#145198,#110930,#110931);
#97033=AXIS2_PLACEMENT_3D('',#145199,#110932,#110933);
#97034=AXIS2_PLACEMENT_3D('',#145200,#110934,#110935);
#97035=AXIS2_PLACEMENT_3D('',#145206,#110936,#110937);
#97036=AXIS2_PLACEMENT_3D('',#145207,#110938,#110939);
#97037=AXIS2_PLACEMENT_3D('',#145208,#110940,#110941);
#97038=AXIS2_PLACEMENT_3D('',#145241,#110942,#110943);
#97039=AXIS2_PLACEMENT_3D('',#145273,#110944,#110945);
#97040=AXIS2_PLACEMENT_3D('',#145294,#110946,#110947);
#97041=AXIS2_PLACEMENT_3D('',#145295,#110948,#110949);
#97042=AXIS2_PLACEMENT_3D('',#145296,#110950,#110951);
#97043=AXIS2_PLACEMENT_3D('',#145317,#110952,#110953);
#97044=AXIS2_PLACEMENT_3D('',#145319,#110954,#110955);
#97045=AXIS2_PLACEMENT_3D('',#145321,#110957,#110958);
#97046=AXIS2_PLACEMENT_3D('',#145323,#110960,#110961);
#97047=AXIS2_PLACEMENT_3D('',#145326,#110964,#110965);
#97048=AXIS2_PLACEMENT_3D('',#145327,#110966,#110967);
#97049=AXIS2_PLACEMENT_3D('',#145328,#110968,#110969);
#97050=AXIS2_PLACEMENT_3D('',#145329,#110970,#110971);
#97051=AXIS2_PLACEMENT_3D('',#145333,#110973,#110974);
#97052=AXIS2_PLACEMENT_3D('',#145335,#110976,#110977);
#97053=AXIS2_PLACEMENT_3D('',#145338,#110979,#110980);
#97054=AXIS2_PLACEMENT_3D('',#145339,#110981,#110982);
#97055=AXIS2_PLACEMENT_3D('',#145340,#110983,#110984);
#97056=AXIS2_PLACEMENT_3D('',#145341,#110985,#110986);
#97057=AXIS2_PLACEMENT_3D('',#145342,#110987,#110988);
#97058=AXIS2_PLACEMENT_3D('',#145344,#110990,#110991);
#97059=AXIS2_PLACEMENT_3D('',#145345,#110992,#110993);
#97060=AXIS2_PLACEMENT_3D('',#145346,#110994,#110995);
#97061=AXIS2_PLACEMENT_3D('',#145347,#110996,#110997);
#97062=AXIS2_PLACEMENT_3D('',#145348,#110998,#110999);
#97063=AXIS2_PLACEMENT_3D('',#145350,#111001,#111002);
#97064=AXIS2_PLACEMENT_3D('',#145352,#111004,#111005);
#97065=AXIS2_PLACEMENT_3D('',#145354,#111007,#111008);
#97066=AXIS2_PLACEMENT_3D('',#145355,#111009,#111010);
#97067=AXIS2_PLACEMENT_3D('',#145356,#111011,#111012);
#97068=AXIS2_PLACEMENT_3D('',#145358,#111014,#111015);
#97069=AXIS2_PLACEMENT_3D('',#145359,#111016,#111017);
#97070=AXIS2_PLACEMENT_3D('',#145361,#111019,#111020);
#97071=AXIS2_PLACEMENT_3D('',#145363,#111022,#111023);
#97072=AXIS2_PLACEMENT_3D('',#145365,#111025,#111026);
#97073=AXIS2_PLACEMENT_3D('',#145366,#111027,#111028);
#97074=AXIS2_PLACEMENT_3D('',#145367,#111029,#111030);
#97075=AXIS2_PLACEMENT_3D('',#145368,#111031,#111032);
#97076=AXIS2_PLACEMENT_3D('',#145369,#111033,#111034);
#97077=AXIS2_PLACEMENT_3D('',#145370,#111035,#111036);
#97078=AXIS2_PLACEMENT_3D('',#145376,#111040,#111041);
#97079=AXIS2_PLACEMENT_3D('',#145378,#111042,#111043);
#97080=AXIS2_PLACEMENT_3D('',#145381,#111045,#111046);
#97081=AXIS2_PLACEMENT_3D('',#145382,#111047,#111048);
#97082=AXIS2_PLACEMENT_3D('',#145385,#111051,#111052);
#97083=AXIS2_PLACEMENT_3D('',#145386,#111053,#111054);
#97084=AXIS2_PLACEMENT_3D('',#145387,#111055,#111056);
#97085=AXIS2_PLACEMENT_3D('',#145389,#111058,#111059);
#97086=AXIS2_PLACEMENT_3D('',#145390,#111060,#111061);
#97087=AXIS2_PLACEMENT_3D('',#145391,#111062,#111063);
#97088=AXIS2_PLACEMENT_3D('',#145392,#111064,#111065);
#97089=AXIS2_PLACEMENT_3D('',#145393,#111066,#111067);
#97090=AXIS2_PLACEMENT_3D('',#145394,#111068,#111069);
#97091=AXIS2_PLACEMENT_3D('',#145396,#111071,#111072);
#97092=AXIS2_PLACEMENT_3D('',#145397,#111073,#111074);
#106742=DIRECTION('axis',(0.,0.,1.));
#106743=DIRECTION('refdir',(1.,0.,0.));
#106744=DIRECTION('center_axis',(0.707106781187368,-1.61919227945235E-16,
0.707106781185727));
#106745=DIRECTION('ref_axis',(-0.499999999999422,0.707106781186549,0.500000000000576));
#106746=DIRECTION('center_axis',(-0.707106781187366,0.,-0.707106781185729));
#106747=DIRECTION('ref_axis',(-0.707106781185729,0.,0.707106781187366));
#106748=DIRECTION('',(0.707106781187368,-1.61919227945235E-16,0.707106781185727));
#106749=DIRECTION('center_axis',(0.707106781187366,0.,0.707106781185729));
#106750=DIRECTION('ref_axis',(0.,1.,0.));
#106751=DIRECTION('',(-0.707106781187368,1.61919227945235E-16,-0.707106781185727));
#106752=DIRECTION('center_axis',(0.0231981048318895,0.,-0.999730887755404));
#106753=DIRECTION('ref_axis',(0.,1.,0.));
#106754=DIRECTION('center_axis',(-6.93889390390725E-18,-1.,-2.22049474265475E-16));
#106755=DIRECTION('ref_axis',(0.37194083714349,-1.73472347597681E-16,0.928256437448726));
#106756=DIRECTION('center_axis',(6.93889390390725E-18,1.,2.22049474265475E-16));
#106757=DIRECTION('ref_axis',(0.37194083714349,-2.08699711926501E-16,0.928256437448726));
#106758=DIRECTION('center_axis',(-6.93889390390725E-18,-1.,-2.22049474265475E-16));
#106759=DIRECTION('ref_axis',(0.,2.03710646720212E-16,-1.));
#106760=DIRECTION('center_axis',(0.978760432413326,0.,-0.205007355824322));
#106761=DIRECTION('ref_axis',(0.,1.,0.));
#106762=DIRECTION('center_axis',(6.93889390390725E-18,1.,2.22049474265475E-16));
#106763=DIRECTION('ref_axis',(-0.768845497716612,1.49223524815209E-16,-0.639434594498058));
#106764=DIRECTION('center_axis',(-6.93889390390725E-18,-1.,-2.22049474265475E-16));
#106765=DIRECTION('ref_axis',(-0.768845497716612,1.47321052872603E-16,-0.639434594498058));
#106766=DIRECTION('center_axis',(-0.474498912689989,0.,-0.880256088792357));
#106767=DIRECTION('ref_axis',(0.,1.,0.));
#106768=DIRECTION('center_axis',(-6.93889390390725E-18,-1.,-2.22049474265475E-16));
#106769=DIRECTION('ref_axis',(0.906884704407261,-8.67361737988403E-17,0.421378847252867));
#106770=DIRECTION('center_axis',(6.93889390390725E-18,1.,2.22049474265475E-16));
#106771=DIRECTION('ref_axis',(0.906884704407261,-9.98597282460494E-17,0.421378847252868));
#106772=DIRECTION('center_axis',(-6.93889390390725E-18,-1.,-2.22049474265475E-16));
#106773=DIRECTION('ref_axis',(0.,2.24081711397792E-16,-1.));
#106774=DIRECTION('center_axis',(0.0394929644100698,0.,-0.99921984856292));
#106775=DIRECTION('ref_axis',(0.,1.,0.));
#106776=DIRECTION('center_axis',(6.93889390390725E-18,1.,2.22049474265475E-16));
#106777=DIRECTION('ref_axis',(-0.974245534865613,-4.12211519055028E-17,
0.225489773148175));
#106778=DIRECTION('center_axis',(-6.93889390390725E-18,-1.,-2.22049474265475E-16));
#106779=DIRECTION('ref_axis',(-0.974245534865613,-4.33096991770057E-17,
0.225489773148175));
#106780=DIRECTION('center_axis',(-0.97649605508074,-1.49557640001864E-16,
0.215535274170498));
#106781=DIRECTION('ref_axis',(0.,1.,6.93889390390723E-16));
#106782=DIRECTION('center_axis',(-6.93889390390725E-18,-1.,-2.22049474265475E-16));
#106783=DIRECTION('ref_axis',(0.641559662047602,1.7347234759768E-16,-0.767073138646744));
#106784=DIRECTION('center_axis',(6.93889390390725E-18,1.,2.22049474265475E-16));
#106785=DIRECTION('ref_axis',(0.641559662047602,1.65876472731702E-16,-0.767073138646744));
#106786=DIRECTION('center_axis',(6.93889390390725E-18,1.,2.22049474265475E-16));
#106787=DIRECTION('ref_axis',(0.,-2.22044604925031E-16,1.));
#106788=DIRECTION('center_axis',(-0.864862503651722,0.,0.502008814441813));
#106789=DIRECTION('ref_axis',(0.,1.,0.));
#106790=DIRECTION('center_axis',(-6.93889390390725E-18,-1.,-2.22049474265475E-16));
#106791=DIRECTION('ref_axis',(-0.363087995156522,2.08166817117217E-16,-0.93175485390376));
#106792=DIRECTION('center_axis',(6.93889390390725E-18,1.,2.22049474265475E-16));
#106793=DIRECTION('ref_axis',(-0.363087995156523,2.09415104529808E-16,-0.93175485390376));
#106794=DIRECTION('center_axis',(1.88217497143483E-12,0.,1.));
#106795=DIRECTION('ref_axis',(0.,1.,0.));
#106796=DIRECTION('center_axis',(-6.93889390390725E-18,-1.,-2.22049474265475E-16));
#106797=DIRECTION('ref_axis',(-0.866605104544004,8.67361737988402E-17,-0.498994581912747));
#106798=DIRECTION('center_axis',(6.93889390390725E-18,1.,2.22049474265475E-16));
#106799=DIRECTION('ref_axis',(-0.866605104544003,1.16814765452061E-16,-0.498994581912747));
#106800=DIRECTION('center_axis',(1.88236169427837E-12,-2.22049474265488E-16,
1.));
#106801=DIRECTION('ref_axis',(-0.707106781186548,0.707106781186548,1.3306533587345E-12));
#106802=DIRECTION('center_axis',(1.88182802673964E-12,0.,1.));
#106803=DIRECTION('ref_axis',(0.,1.,0.));
#106804=DIRECTION('',(-1.88236169427837E-12,2.22049474265488E-16,-1.));
#106805=DIRECTION('',(1.88236169427837E-12,-2.22049474265488E-16,1.));
#106806=DIRECTION('center_axis',(-6.93889390390725E-18,-1.,-2.22049474265475E-16));
#106807=DIRECTION('ref_axis',(-0.923879532510704,-8.67361737988403E-17,
0.382683432366495));
#106808=DIRECTION('center_axis',(6.93889390390725E-18,1.,2.22049474265475E-16));
#106809=DIRECTION('ref_axis',(-0.923879532510704,-7.85639529110045E-17,
0.382683432366495));
#106810=DIRECTION('center_axis',(0.,-1.,-2.22044604925031E-16));
#106811=DIRECTION('ref_axis',(-1.,0.,0.));
#106812=DIRECTION('',(0.,1.,2.22044604925031E-16));
#106813=DIRECTION('center_axis',(-5.19732413453357E-17,1.,2.87905372759356E-16));
#106814=DIRECTION('ref_axis',(-1.,0.,0.));
#106815=DIRECTION('',(0.,1.,2.22044604925031E-16));
#106816=DIRECTION('center_axis',(4.16333634234434E-17,-1.,-2.28983498828938E-16));
#106817=DIRECTION('ref_axis',(-1.,0.,0.));
#106818=DIRECTION('',(0.,-1.,-2.22044604925031E-16));
#106819=DIRECTION('',(0.,-1.,-2.22044604925031E-16));
#106820=DIRECTION('center_axis',(0.,-1.,-2.22044604925031E-16));
#106821=DIRECTION('ref_axis',(-1.,0.,0.));
#106822=DIRECTION('',(0.,-1.,-2.22044604925031E-16));
#106823=DIRECTION('center_axis',(1.04492064682899E-28,-1.,-2.22044604925092E-16));
#106824=DIRECTION('ref_axis',(-0.866605104544003,0.,-0.498994581912747));
#106825=DIRECTION('',(1.04492064682899E-28,-1.,-2.22044604925092E-16));
#106826=DIRECTION('center_axis',(0.,-1.,-2.22044604925031E-16));
#106827=DIRECTION('ref_axis',(-0.866605104544003,0.,-0.498994581912747));
#106828=DIRECTION('center_axis',(1.,5.22460323415068E-28,-1.88236169427837E-12));
#106829=DIRECTION('ref_axis',(1.88236169427837E-12,-2.12407076745007E-16,
1.));
#106830=DIRECTION('',(-2.62675723349586E-44,1.,2.77555756156289E-16));
#106831=DIRECTION('',(1.88236169427837E-12,-2.12407076745007E-16,1.));
#106832=DIRECTION('center_axis',(-6.34155293818297E-44,-1.,-2.77555756156289E-16));
#106833=DIRECTION('ref_axis',(-0.923879532510704,-3.75530232012225E-16,
0.382683432366498));
#106834=DIRECTION('',(-6.34155293818297E-44,-1.,-2.77555756156289E-16));
#106835=DIRECTION('center_axis',(0.,-1.,-2.22044604925031E-16));
#106836=DIRECTION('ref_axis',(-0.923879532510704,-3.75530232012225E-16,
0.382683432366498));
#106837=DIRECTION('center_axis',(0.707106781185727,1.962615573357E-16,-0.707106781187368));
#106838=DIRECTION('ref_axis',(0.707106781187368,-1.66829210022371E-16,0.707106781185727));
#106839=DIRECTION('',(-1.38777878078145E-16,1.,1.38777878078467E-16));
#106840=DIRECTION('',(0.707106781187368,-1.66829210022371E-16,0.707106781185727));
#106841=DIRECTION('center_axis',(-6.93889390390725E-18,-1.,-2.22049474265475E-16));
#106842=DIRECTION('ref_axis',(1.,-6.93889390390725E-18,-1.83750175990301E-19));
#106843=DIRECTION('center_axis',(-0.442887523223796,1.9908012597496E-16,
-0.896577181157702));
#106844=DIRECTION('ref_axis',(0.633975804653729,0.70710678118655,-0.31316877097446));
#106845=DIRECTION('center_axis',(0.442887523223797,0.,0.896577181157702));
#106846=DIRECTION('ref_axis',(0.896577181157702,-1.38777878078145E-15,-0.442887523223797));
#106847=DIRECTION('',(-0.442887523223796,1.9908012597496E-16,-0.896577181157702));
#106848=DIRECTION('center_axis',(-0.442887523223799,0.,-0.896577181157701));
#106849=DIRECTION('ref_axis',(0.,1.,0.));
#106850=DIRECTION('',(0.442887523223796,-1.9908012597496E-16,0.896577181157702));
#106851=DIRECTION('center_axis',(-0.990557901827268,0.,0.137095014962474));
#106852=DIRECTION('ref_axis',(0.,1.,0.));
#106853=DIRECTION('center_axis',(3.42121385298657E-49,-1.,-2.22044604925031E-16));
#106854=DIRECTION('ref_axis',(0.468176250029909,2.31296463463574E-16,-0.883635105067659));
#106855=DIRECTION('center_axis',(-3.42121385298657E-49,1.,2.22044604925031E-16));
#106856=DIRECTION('ref_axis',(0.468176250029909,1.96206407802637E-16,-0.883635105067659));
#106857=DIRECTION('center_axis',(3.42121385298657E-49,-1.,-2.22044604925031E-16));
#106858=DIRECTION('ref_axis',(-0.0834849737561929,-2.22044604925031E-16,
0.996509036164213));
#106859=DIRECTION('center_axis',(-0.953939201414718,0.,-0.300000000007082));
#106860=DIRECTION('ref_axis',(0.,1.,0.));
#106861=DIRECTION('center_axis',(-3.42121385298657E-49,1.,2.22044604925031E-16));
#106862=DIRECTION('ref_axis',(-0.0834849737561933,-2.16840434497101E-16,
0.996509036164212));
#106863=DIRECTION('center_axis',(3.42121385298657E-49,-1.,-2.22044604925031E-16));
#106864=DIRECTION('ref_axis',(-0.0834849737561933,-2.21269455239306E-16,
0.996509036164212));
#106865=DIRECTION('center_axis',(-7.42739203474237E-12,0.,1.));
#106866=DIRECTION('ref_axis',(0.,1.,0.));
#106867=DIRECTION('center_axis',(3.42121385298657E-49,-1.,-2.22044604925031E-16));
#106868=DIRECTION('ref_axis',(-0.591607978303975,1.7347234759768E-16,-0.806225774834248));
#106869=DIRECTION('center_axis',(-3.42121385298657E-49,1.,2.22044604925031E-16));
#106870=DIRECTION('ref_axis',(-0.591607978303975,1.79018083653448E-16,-0.806225774834248));
#106871=DIRECTION('center_axis',(-7.42407262755995E-12,-2.22044604925031E-16,
1.));
#106872=DIRECTION('ref_axis',(-0.707106781186548,0.707106781186548,-5.2441088120038E-12));
#106873=DIRECTION('center_axis',(-7.42184091961917E-12,0.,1.));
#106874=DIRECTION('ref_axis',(0.,1.,0.));
#106875=DIRECTION('',(7.42407262755995E-12,2.22044604925031E-16,-1.));
#106876=DIRECTION('',(-7.42407262755995E-12,-2.22044604925031E-16,1.));
#106877=DIRECTION('center_axis',(0.707106781186548,0.,0.707106781186548));
#106878=DIRECTION('ref_axis',(0.,1.,0.));
#106879=DIRECTION('center_axis',(3.42121385298657E-49,-1.,-2.22044604925031E-16));
#106880=DIRECTION('ref_axis',(-0.923879532512707,-8.67361737988402E-17,
0.38268343236166));
#106881=DIRECTION('center_axis',(-3.42121385298657E-49,1.,2.22044604925031E-16));
#106882=DIRECTION('ref_axis',(-0.923879532512707,-8.49727915500997E-17,
0.38268343236166));
#106883=DIRECTION('center_axis',(0.707106781186547,-1.57009245868378E-16,
0.707106781186548));
#106884=DIRECTION('ref_axis',(-0.500000000000001,0.707106781186546,0.500000000000001));
#106885=DIRECTION('center_axis',(0.707106781186545,0.,0.70710678118655));
#106886=DIRECTION('ref_axis',(0.,1.,0.));
#106887=DIRECTION('',(-0.707106781186547,1.57009245868378E-16,-0.707106781186548));
#106888=DIRECTION('',(0.707106781186547,-1.57009245868378E-16,0.707106781186548));
#106889=DIRECTION('center_axis',(3.42121385298657E-49,-1.,-2.22044604925031E-16));
#106890=DIRECTION('ref_axis',(0.,1.38777878078145E-16,-1.));
#106891=DIRECTION('center_axis',(1.88182802673965E-12,0.,1.));
#106892=DIRECTION('ref_axis',(0.,1.,0.));
#106893=DIRECTION('center_axis',(-3.42121385298657E-49,1.,2.22044604925031E-16));
#106894=DIRECTION('ref_axis',(0.923879532510927,8.67361737988404E-17,-0.382683432365959));
#106895=DIRECTION('center_axis',(3.42121385298657E-49,-1.,-2.22044604925031E-16));
#106896=DIRECTION('ref_axis',(0.923879532510927,8.49727915510542E-17,-0.382683432365959));
#106897=DIRECTION('center_axis',(-1.88236169427837E-12,2.22044604925031E-16,
-1.));
#106898=DIRECTION('ref_axis',(-0.707106781186548,0.707106781186548,1.3306533587345E-12));
#106899=DIRECTION('center_axis',(1.88113413734926E-12,0.,1.));
#106900=DIRECTION('ref_axis',(0.,1.,0.));
#106901=DIRECTION('',(-1.88236169427837E-12,2.22044604925031E-16,-1.));
#106902=DIRECTION('',(1.88236169427837E-12,-2.22044604925031E-16,1.));
#106903=DIRECTION('center_axis',(0.915812085606104,0.,-0.401607051553878));
#106904=DIRECTION('ref_axis',(0.,1.,0.));
#106905=DIRECTION('center_axis',(3.42121385298657E-49,-1.,-2.22044604925031E-16));
#106906=DIRECTION('ref_axis',(-0.546988550357502,-1.73472347597681E-16,
0.837140087307852));
#106907=DIRECTION('center_axis',(-3.42121385298657E-49,1.,2.22044604925031E-16));
#106908=DIRECTION('ref_axis',(-0.546988550357502,-1.85882439953178E-16,
0.837140087307852));
#106909=DIRECTION('center_axis',(3.42121385298657E-49,-1.,-2.22044604925031E-16));
#106910=DIRECTION('ref_axis',(0.,2.22044604925031E-16,-1.));
#106911=DIRECTION('center_axis',(0.943231903981036,0.,-0.332134875182221));
#106912=DIRECTION('ref_axis',(0.,1.,0.));
#106913=DIRECTION('center_axis',(-3.42121385298657E-49,1.,2.22044604925031E-16));
#106914=DIRECTION('ref_axis',(-0.367127042551388,2.05012774433623E-16,-0.930170809382595));
#106915=DIRECTION('center_axis',(3.42121385298657E-49,-1.,-2.22044604925031E-16));
#106916=DIRECTION('ref_axis',(-0.367127042551388,2.06539409882155E-16,-0.930170809382595));
#106917=DIRECTION('center_axis',(-0.143915261386658,0.,-0.989590014874852));
#106918=DIRECTION('ref_axis',(0.,1.,0.));
#106919=DIRECTION('center_axis',(3.42121385298657E-49,-1.,-2.22044604925031E-16));
#106920=DIRECTION('ref_axis',(0.855693526352071,-1.15648231731787E-16,0.517482935911086));
#106921=DIRECTION('center_axis',(-3.42121385298657E-49,1.,2.22044604925031E-16));
#106922=DIRECTION('ref_axis',(0.855693526352071,-1.14904294059822E-16,0.517482935911086));
#106923=DIRECTION('center_axis',(3.42121385298657E-49,-1.,-2.22044604925031E-16));
#106924=DIRECTION('ref_axis',(0.,2.24855296126614E-16,-1.));
#106925=DIRECTION('center_axis',(0.681400754633201,0.,-0.731910521570297));
#106926=DIRECTION('ref_axis',(0.,1.,0.));
#106927=DIRECTION('center_axis',(-3.42121385298657E-49,1.,2.22044604925031E-16));
#106928=DIRECTION('ref_axis',(-0.954556261212484,6.60847038467355E-17,-0.29803077723625));
#106929=DIRECTION('center_axis',(-3.42121385298657E-49,1.,2.22044604925031E-16));
#106930=DIRECTION('ref_axis',(-0.954556261212484,6.60847038467355E-17,-0.29803077723625));
#106931=DIRECTION('center_axis',(3.42121385298657E-49,-1.,-2.22044604925031E-16));
#106932=DIRECTION('ref_axis',(-0.954556261212484,6.61761261869232E-17,-0.29803077723625));
#106933=DIRECTION('center_axis',(3.42121385298657E-49,-1.,-2.22044604925031E-16));
#106934=DIRECTION('ref_axis',(0.989443824790343,0.,0.144916933393781));
#106935=DIRECTION('center_axis',(-3.42121385298657E-49,1.,2.22044604925031E-16));
#106936=DIRECTION('ref_axis',(0.989443824790343,-3.21780232223691E-17,0.144916933393781));
#106937=DIRECTION('center_axis',(1.,-5.1044736764327E-16,-1.88236169427837E-12));
#106938=DIRECTION('ref_axis',(1.88236169427837E-12,-2.12407076745007E-16,
1.));
#106939=DIRECTION('',(5.10447367643583E-16,1.,1.6657509746718E-16));
#106940=DIRECTION('',(-1.88236169427837E-12,2.22044604925031E-16,-1.));
#106941=DIRECTION('',(-5.1044736764375E-16,-1.,-2.55223683821875E-16));
#106942=DIRECTION('center_axis',(0.,1.,1.6657509746814E-16));
#106943=DIRECTION('ref_axis',(-0.546988550357499,0.,0.837140087307854));
#106944=DIRECTION('',(0.,-1.,-1.6657509746814E-16));
#106945=DIRECTION('center_axis',(4.16333634234434E-17,-1.,-2.28983498828938E-16));
#106946=DIRECTION('ref_axis',(-0.546988550357499,0.,0.837140087307854));
#106947=DIRECTION('center_axis',(0.,1.,1.6657509746814E-16));
#106948=DIRECTION('ref_axis',(-0.91120908155642,6.86196423904955E-17,-0.411944182734877));
#106949=DIRECTION('',(0.,1.,1.6657509746814E-16));
#106950=DIRECTION('center_axis',(-4.16333634234434E-17,1.,2.28983498828938E-16));
#106951=DIRECTION('ref_axis',(-0.91120908155642,6.86196423904955E-17,-0.411944182734877));
#106952=DIRECTION('center_axis',(0.,-1.,-1.6657509746814E-16));
#106953=DIRECTION('ref_axis',(0.855693526352075,0.,0.517482935911081));
#106954=DIRECTION('',(0.,-1.,-1.6657509746814E-16));
#106955=DIRECTION('center_axis',(4.16333634234434E-17,-1.,-2.28983498828938E-16));
#106956=DIRECTION('ref_axis',(0.855693526352075,0.,0.517482935911081));
#106957=DIRECTION('center_axis',(0.,1.,1.6657509746814E-16));
#106958=DIRECTION('ref_axis',(1.,0.,1.15584692836443E-33));
#106959=DIRECTION('center_axis',(0.,1.,2.22044604925031E-16));
#106960=DIRECTION('ref_axis',(1.,0.,1.15584692836443E-33));
#106961=DIRECTION('',(0.,1.,1.6657509746814E-16));
#106962=DIRECTION('',(0.,1.,1.6657509746814E-16));
#106963=DIRECTION('center_axis',(4.16333634234434E-17,-1.,-2.28983498828938E-16));
#106964=DIRECTION('ref_axis',(1.,4.16333634234434E-17,6.93889390390723E-17));
#106965=DIRECTION('',(0.,-1.,-2.67523620391604E-16));
#106966=DIRECTION('center_axis',(-3.42121385298657E-49,1.,2.22044604925031E-16));
#106967=DIRECTION('ref_axis',(0.122670494314896,2.20282346155785E-16,-0.992447454440052));
#106968=DIRECTION('',(0.,1.,2.67523620391604E-16));
#106969=DIRECTION('center_axis',(4.16333634234434E-17,-1.,-2.28983498828938E-16));
#106970=DIRECTION('ref_axis',(1.,4.16333634234434E-17,6.93889390390723E-17));
#106971=DIRECTION('',(0.,-1.,-1.6657509746814E-16));
#106972=DIRECTION('center_axis',(-3.32156684755978E-49,1.,2.15577286334982E-16));
#106973=DIRECTION('ref_axis',(1.,0.,3.03664566131718E-33));
#106974=DIRECTION('',(0.,1.,1.6657509746814E-16));
#106975=DIRECTION('center_axis',(4.16333634234434E-17,-1.,-2.28983498828938E-16));
#106976=DIRECTION('ref_axis',(1.,4.16333634234434E-17,6.93889390390723E-17));
#106977=DIRECTION('center_axis',(0.,-1.,-1.6657509746814E-16));
#106978=DIRECTION('ref_axis',(0.989443824790343,0.,0.144916933393781));
#106979=DIRECTION('',(0.,-1.,-1.6657509746814E-16));
#106980=DIRECTION('center_axis',(4.16333634234434E-17,-1.,-2.28983498828938E-16));
#106981=DIRECTION('ref_axis',(0.989443824790343,0.,0.144916933393781));
#106982=DIRECTION('center_axis',(0.896577181157702,7.37740323484271E-17,
-0.442887523223796));
#106983=DIRECTION('ref_axis',(-0.442887523223796,2.02157641249503E-16,-0.896577181157702));
#106984=DIRECTION('',(0.,1.,1.6657509746814E-16));
#106985=DIRECTION('',(0.442887523223796,-1.86862482701593E-16,0.896577181157702));
#106986=DIRECTION('center_axis',(-3.42121385298657E-49,1.,2.22044604925031E-16));
#106987=DIRECTION('ref_axis',(-1.54077774334651E-33,-2.22044604925031E-16,
1.));
#106988=DIRECTION('center_axis',(3.42121385298657E-49,-1.,-2.22044604925031E-16));
#106989=DIRECTION('ref_axis',(0.,2.11471052009443E-16,-1.));
#106990=DIRECTION('center_axis',(-0.634351002555855,0.,0.77304515104642));
#106991=DIRECTION('ref_axis',(0.77304515104642,-1.38777878078145E-15,0.634351002555855));
#106992=DIRECTION('center_axis',(3.42121385298657E-49,-1.,-2.22044604925031E-16));
#106993=DIRECTION('ref_axis',(-0.487986704420985,1.93811869204134E-16,-0.872851061927719));
#106994=DIRECTION('center_axis',(0.990774955112549,0.,-0.135517483454076));
#106995=DIRECTION('ref_axis',(0.,1.,0.));
#106996=DIRECTION('center_axis',(-3.42121385298657E-49,1.,2.22044604925031E-16));
#106997=DIRECTION('ref_axis',(-0.487986704420985,1.93144469193492E-16,-0.872851061927719));
#106998=DIRECTION('center_axis',(0.000408627366271784,0.,-0.999999916511834));
#106999=DIRECTION('ref_axis',(0.,1.,0.));
#107000=DIRECTION('center_axis',(3.42121385298657E-49,-1.,-2.22044604925031E-16));
#107001=DIRECTION('ref_axis',(0.753363330133439,-1.15648231731787E-16,0.657604510941231));
#107002=DIRECTION('center_axis',(-3.42121385298657E-49,1.,2.22044604925031E-16));
#107003=DIRECTION('ref_axis',(0.753363330133439,-1.46017533828864E-16,0.657604510941231));
#107004=DIRECTION('center_axis',(0.000408627366273739,2.22044586386935E-16,
-0.999999916511834));
#107005=DIRECTION('ref_axis',(0.707106722151499,0.707106781186548,0.000288943181669179));
#107006=DIRECTION('center_axis',(0.000408627366277338,0.,-0.999999916511834));
#107007=DIRECTION('ref_axis',(0.,1.,0.));
#107008=DIRECTION('',(-0.000408627366273739,-2.22044586386934E-16,0.999999916511834));
#107009=DIRECTION('',(0.000408627366273739,2.22044586386934E-16,-0.999999916511834));
#107010=DIRECTION('center_axis',(-1.,0.,-1.30451205393456E-12));
#107011=DIRECTION('ref_axis',(0.,1.,0.));
#107012=DIRECTION('center_axis',(3.42121385298657E-49,-1.,-2.22044604925031E-16));
#107013=DIRECTION('ref_axis',(0.707251238022098,1.15648231731787E-16,-0.706962294833473));
#107014=DIRECTION('center_axis',(-3.42121385298657E-49,1.,2.22044604925031E-16));
#107015=DIRECTION('ref_axis',(0.707251238022098,1.56977163453192E-16,-0.706962294833473));
#107016=DIRECTION('center_axis',(-1.,2.89708077091569E-28,-1.30472918803582E-12));
#107017=DIRECTION('ref_axis',(9.22429319476718E-13,0.707106781186547,-0.707106781186548));
#107018=DIRECTION('center_axis',(-1.,0.,-1.30451205393456E-12));
#107019=DIRECTION('ref_axis',(0.,1.,0.));
#107020=DIRECTION('',(1.,-2.89708077091569E-28,1.30472918803582E-12));
#107021=DIRECTION('',(-1.,2.89708077091569E-28,-1.30472918803582E-12));
#107022=DIRECTION('center_axis',(0.368421052642242,0.,0.9296590385566));
#107023=DIRECTION('ref_axis',(0.,1.,0.));
#107024=DIRECTION('center_axis',(3.42121385298657E-49,-1.,-2.22044604925031E-16));
#107025=DIRECTION('ref_axis',(-0.827170191871368,1.15648231731787E-16,-0.561951486944811));
#107026=DIRECTION('center_axis',(-3.42121385298657E-49,1.,2.22044604925031E-16));
#107027=DIRECTION('ref_axis',(-0.827170191871368,1.24778295905694E-16,-0.561951486944811));
#107028=DIRECTION('center_axis',(3.42121385298657E-49,-1.,-2.22044604925031E-16));
#107029=DIRECTION('ref_axis',(0.,2.22044604925031E-16,-1.));
#107030=DIRECTION('center_axis',(-0.710839466106974,0.,0.703354287272603));
#107031=DIRECTION('ref_axis',(0.,1.,0.));
#107032=DIRECTION('center_axis',(-3.42121385298657E-49,1.,2.22044604925031E-16));
#107033=DIRECTION('ref_axis',(0.978715457840861,-4.33680868994202E-17,0.205221959310776));
#107034=DIRECTION('center_axis',(3.42121385298657E-49,-1.,-2.22044604925031E-16));
#107035=DIRECTION('ref_axis',(0.978715457840861,-4.5568428877102E-17,0.205221959310776));
#107036=DIRECTION('center_axis',(0.442887523223795,0.,0.896577181157703));
#107037=DIRECTION('ref_axis',(0.,1.,0.));
#107038=DIRECTION('center_axis',(3.42121385298657E-49,-1.,-2.22044604925031E-16));
#107039=DIRECTION('ref_axis',(-0.986263994778248,0.,-0.165176670883183));
#107040=DIRECTION('center_axis',(-3.42121385298657E-49,1.,2.22044604925031E-16));
#107041=DIRECTION('ref_axis',(-0.986263994778248,3.66765886290883E-17,-0.165176670883183));
#107042=DIRECTION('center_axis',(0.442887523223796,-1.9908012597496E-16,
0.896577181157703));
#107043=DIRECTION('ref_axis',(-0.633975804653731,0.707106781186549,0.313168770974457));
#107044=DIRECTION('center_axis',(0.442887523223795,0.,0.896577181157703));
#107045=DIRECTION('ref_axis',(0.,1.,0.));
#107046=DIRECTION('',(-0.442887523223796,1.9908012597496E-16,-0.896577181157703));
#107047=DIRECTION('',(0.442887523223796,-1.9908012597496E-16,0.896577181157703));
#107048=DIRECTION('center_axis',(0.991156957142872,0.,-0.132694710924297));
#107049=DIRECTION('ref_axis',(0.,1.,0.));
#107050=DIRECTION('center_axis',(3.42121385298657E-49,-1.,-2.22044604925031E-16));
#107051=DIRECTION('ref_axis',(-0.47013716097003,-2.31296463463574E-16,0.882593366095078));
#107052=DIRECTION('center_axis',(-3.42121385298657E-49,1.,2.22044604925031E-16));
#107053=DIRECTION('ref_axis',(-0.47013716097003,-1.95975095284035E-16,0.882593366095078));
#107054=DIRECTION('center_axis',(3.42121385298657E-49,-1.,-2.22044604925031E-16));
#107055=DIRECTION('ref_axis',(0.,2.24855296126614E-16,-1.));
#107056=DIRECTION('center_axis',(0.929017422864237,0.,0.370035982054031));
#107057=DIRECTION('ref_axis',(0.,1.,0.));
#107058=DIRECTION('center_axis',(3.42121385298657E-49,-1.,-2.22044604925031E-16));
#107059=DIRECTION('ref_axis',(0.122670494314896,2.20367602929994E-16,-0.992447454440052));
#107060=DIRECTION('center_axis',(3.42121385298657E-49,-1.,-2.22044604925031E-16));
#107061=DIRECTION('ref_axis',(0.249622059095992,-2.31296463463574E-16,0.968343341802213));
#107062=DIRECTION('center_axis',(-3.42121385298657E-49,1.,2.22044604925031E-16));
#107063=DIRECTION('ref_axis',(0.249622059095992,-2.15015414762257E-16,0.968343341802213));
#107064=DIRECTION('center_axis',(0.,1.,1.6657509746814E-16));
#107065=DIRECTION('ref_axis',(-0.986263994778249,0.,-0.165176670883179));
#107066=DIRECTION('',(4.0084926897219E-17,-1.,-1.86376085453573E-16));
#107067=DIRECTION('center_axis',(4.16333634234434E-17,-1.,-2.28983498828938E-16));
#107068=DIRECTION('ref_axis',(-0.986263994778249,0.,-0.165176670883179));
#107069=DIRECTION('',(0.,-1.,0.));
#107070=DIRECTION('center_axis',(0.,-1.,-2.22044604925031E-16));
#107071=DIRECTION('ref_axis',(-0.986263994778249,0.,-0.165176670883179));
#107072=DIRECTION('',(0.,1.,1.6657509746814E-16));
#107073=DIRECTION('center_axis',(-0.896577181157703,-1.184828736391E-16,
0.442887523223796));
#107074=DIRECTION('ref_axis',(0.442887523223796,-2.02157641249503E-16,0.896577181157703));
#107075=DIRECTION('',(0.,1.,2.67523620391604E-16));
#107076=DIRECTION('',(-0.442887523223796,1.86862482701593E-16,-0.896577181157703));
#107077=DIRECTION('center_axis',(0.,-1.,-2.67523620391604E-16));
#107078=DIRECTION('ref_axis',(-0.47013716097003,0.,0.882593366095077));
#107079=DIRECTION('center_axis',(4.16333634234434E-17,-1.,-2.28983498828938E-16));
#107080=DIRECTION('ref_axis',(-0.47013716097003,0.,0.882593366095077));
#107081=DIRECTION('center_axis',(0.,-1.,-2.67523620391604E-16));
#107082=DIRECTION('ref_axis',(0.24962205909599,0.,0.968343341802213));
#107083=DIRECTION('',(0.,-1.,-2.67523620391604E-16));
#107084=DIRECTION('center_axis',(1.35739377892777E-16,-1.,-3.84762012452445E-17));
#107085=DIRECTION('ref_axis',(0.24962205909599,0.,0.968343341802213));
#107086=DIRECTION('center_axis',(0.,1.,2.67523620391604E-16));
#107087=DIRECTION('ref_axis',(-0.984274724761795,4.72565661779708E-17,-0.176644462678832));
#107088=DIRECTION('',(0.,1.,2.67523620391604E-16));
#107089=DIRECTION('center_axis',(-1.35739377892777E-16,1.,3.84762012452445E-17));
#107090=DIRECTION('ref_axis',(-0.984274724761795,4.72565661779708E-17,-0.176644462678832));
#107091=DIRECTION('center_axis',(-3.42121385298657E-49,1.,2.22044604925031E-16));
#107092=DIRECTION('ref_axis',(-1.54077774334651E-33,-2.22044604925031E-16,
1.));
#107093=DIRECTION('center_axis',(-0.000408627366273673,-2.22046620305031E-16,
0.999999916511834));
#107094=DIRECTION('ref_axis',(-0.707106722151501,0.707106781186546,-0.000288943181673103));
#107095=DIRECTION('center_axis',(0.000408627366271784,0.,-0.999999916511834));
#107096=DIRECTION('ref_axis',(-0.999999916511834,-2.77555756156288E-15,
-0.000408627366271784));
#107097=DIRECTION('',(-0.000408627366273673,-2.22046620305031E-16,0.999999916511834));
#107098=DIRECTION('center_axis',(-0.000408627366277335,0.,0.999999916511834));
#107099=DIRECTION('ref_axis',(0.,1.,0.));
#107100=DIRECTION('',(0.000408627366273673,2.22046620305031E-16,-0.999999916511834));
#107101=DIRECTION('center_axis',(0.990663871945179,0.,0.136327153651006));
#107102=DIRECTION('ref_axis',(0.,1.,0.));
#107103=DIRECTION('center_axis',(-6.93889390390723E-18,-1.,-2.22049474265475E-16));
#107104=DIRECTION('ref_axis',(-0.753900508899602,-1.15648231731787E-16,
0.656988601636985));
#107105=DIRECTION('center_axis',(6.93889390390723E-18,1.,2.22049474265475E-16));
#107106=DIRECTION('ref_axis',(-0.753900508899602,-1.40652737946546E-16,
0.656988601636985));
#107107=DIRECTION('center_axis',(-6.93889390390723E-18,-1.,-2.22049474265475E-16));
#107108=DIRECTION('ref_axis',(0.,2.11471052009443E-16,-1.));
#107109=DIRECTION('center_axis',(0.829730454564779,0.,0.558164288330708));
#107110=DIRECTION('ref_axis',(0.,1.,0.));
#107111=DIRECTION('center_axis',(6.93889390390723E-18,1.,2.22049474265475E-16));
#107112=DIRECTION('ref_axis',(0.356447025452442,2.07451466911529E-16,-0.934315534520382));
#107113=DIRECTION('center_axis',(-6.93889390390723E-18,-1.,-2.22049474265475E-16));
#107114=DIRECTION('ref_axis',(0.356447025452442,2.04990925146339E-16,-0.934315534520382));
#107115=DIRECTION('center_axis',(0.748617784953237,0.,-0.663001819041026));
#107116=DIRECTION('ref_axis',(0.,1.,0.));
#107117=DIRECTION('center_axis',(-6.93889390390723E-18,-1.,-2.22049474265475E-16));
#107118=DIRECTION('ref_axis',(0.0662762646370237,-2.31296463463574E-16,
0.997801311256787));
#107119=DIRECTION('center_axis',(6.93889390390723E-18,1.,2.22049474265475E-16));
#107120=DIRECTION('ref_axis',(0.0662762646370237,-2.22021140554634E-16,
0.997801311256787));
#107121=DIRECTION('center_axis',(-6.93889390390723E-18,-1.,-2.22049474265475E-16));
#107122=DIRECTION('ref_axis',(0.,1.97372982155583E-16,-1.));
#107123=DIRECTION('center_axis',(0.939530312300397,0.,-0.342465753424659));
#107124=DIRECTION('ref_axis',(0.,1.,0.));
#107125=DIRECTION('center_axis',(6.93889390390723E-18,1.,2.22049474265475E-16));
#107126=DIRECTION('ref_axis',(-0.511715895878297,1.87537673078574E-16,-0.859154725241892));
#107127=DIRECTION('center_axis',(-6.93889390390723E-18,-1.,-2.22049474265475E-16));
#107128=DIRECTION('ref_axis',(-0.511715895878297,1.94325597363103E-16,-0.859154725241892));
#107129=DIRECTION('center_axis',(6.93889390390723E-18,1.,2.22049474265475E-16));
#107130=DIRECTION('ref_axis',(0.,-1.85037170770859E-16,1.));
#107131=DIRECTION('center_axis',(0.,0.,-1.));
#107132=DIRECTION('ref_axis',(0.,1.,0.));
#107133=DIRECTION('center_axis',(-6.93889390390723E-18,-1.,-2.22049474265475E-16));
#107134=DIRECTION('ref_axis',(0.819288030372914,-1.34922937020418E-16,0.573382179080996));
#107135=DIRECTION('center_axis',(6.93889390390723E-18,1.,2.22049474265475E-16));
#107136=DIRECTION('ref_axis',(0.819288030372914,-1.33004164137626E-16,0.573382179080996));
#107137=DIRECTION('center_axis',(7.61924092396395E-16,2.22049474265475E-16,
-1.));
#107138=DIRECTION('ref_axis',(0.707106781186548,0.707106781186547,0.));
#107139=DIRECTION('center_axis',(0.,0.,-1.));
#107140=DIRECTION('ref_axis',(0.,1.,0.));
#107141=DIRECTION('',(-7.61924092396395E-16,-2.22049474265475E-16,1.));
#107142=DIRECTION('',(7.61924092396395E-16,2.22049474265475E-16,-1.));
#107143=DIRECTION('center_axis',(-6.93889390390723E-18,-1.,-2.22049474265475E-16));
#107144=DIRECTION('ref_axis',(0.,2.14881875733901E-16,-1.));
#107145=DIRECTION('center_axis',(0.300000000002116,0.,-0.95393920141628));
#107146=DIRECTION('ref_axis',(0.,1.,0.));
#107147=DIRECTION('center_axis',(6.93889390390723E-18,1.,2.22049474265475E-16));
#107148=DIRECTION('ref_axis',(-0.988417725816438,5.13992141030164E-17,-0.151757699283627));
#107149=DIRECTION('center_axis',(-6.93889390390723E-18,-1.,-2.22049474265475E-16));
#107150=DIRECTION('ref_axis',(-0.988417725816438,4.0556243073849E-17,-0.151757699283627));
#107151=DIRECTION('center_axis',(-1.,0.,-1.30451205393454E-12));
#107152=DIRECTION('ref_axis',(0.,1.,0.));
#107153=DIRECTION('center_axis',(-6.93889390390723E-18,-1.,-2.22049474265475E-16));
#107154=DIRECTION('ref_axis',(0.806225774830896,1.15648231731787E-16,-0.591607978308543));
#107155=DIRECTION('center_axis',(6.93889390390723E-18,1.,2.22049474265475E-16));
#107156=DIRECTION('ref_axis',(0.806225774830896,1.25771925440525E-16,-0.591607978308543));
#107157=DIRECTION('center_axis',(-1.,6.93889390419694E-18,-1.30472918803582E-12));
#107158=DIRECTION('ref_axis',(9.22429319476717E-13,0.707106781186547,-0.707106781186548));
#107159=DIRECTION('center_axis',(-1.,0.,-1.30451205393456E-12));
#107160=DIRECTION('ref_axis',(0.,1.,0.));
#107161=DIRECTION('',(1.,-6.93889390419694E-18,1.30472918803582E-12));
#107162=DIRECTION('',(-1.,6.93889390419694E-18,-1.30472918803582E-12));
#107163=DIRECTION('center_axis',(-6.93889390390723E-18,-1.,-2.22049474265475E-16));
#107164=DIRECTION('ref_axis',(-0.706962294833474,1.15648231731787E-16,-0.707251238022097));
#107165=DIRECTION('center_axis',(6.93889390390723E-18,1.,2.22049474265475E-16));
#107166=DIRECTION('ref_axis',(-0.706962294833474,1.61950301934325E-16,-0.707251238022097));
#107167=DIRECTION('center_axis',(1.,-2.03832691661471E-31,7.61924092396395E-16));
#107168=DIRECTION('ref_axis',(7.61924092396395E-16,2.22049474265475E-16,
-1.));
#107169=DIRECTION('',(0.,1.,2.67523620391604E-16));
#107170=DIRECTION('',(7.61924092396395E-16,2.22044604925031E-16,-1.));
#107171=DIRECTION('',(-9.82764763367805E-32,1.,3.96508223080413E-16));
#107172=DIRECTION('',(7.61924092396395E-16,2.22044604925031E-16,-1.));
#107173=DIRECTION('',(0.,1.,2.67523620391604E-16));
#107174=DIRECTION('center_axis',(0.,1.,2.67523620391604E-16));
#107175=DIRECTION('ref_axis',(-1.,4.09094084738805E-31,-1.53134210293125E-15));
#107176=DIRECTION('',(0.,1.,2.67523620391604E-16));
#107177=DIRECTION('center_axis',(0.,-1.,-2.22044604925031E-16));
#107178=DIRECTION('ref_axis',(-1.,4.09094084738805E-31,-1.53134210293125E-15));
#107179=DIRECTION('center_axis',(0.,-1.,-2.67523620391604E-16));
#107180=DIRECTION('ref_axis',(0.806225774830893,0.,-0.591607978308547));
#107181=DIRECTION('',(0.,-1.,-2.67523620391604E-16));
#107182=DIRECTION('center_axis',(0.,-1.,-2.22044604925031E-16));
#107183=DIRECTION('ref_axis',(0.806225774830893,0.,-0.591607978308547));
#107184=DIRECTION('center_axis',(1.30472918803582E-12,2.67523620391604E-16,
-1.));
#107185=DIRECTION('ref_axis',(-1.,6.93889390419694E-18,-1.30472918803582E-12));
#107186=DIRECTION('',(0.,1.,2.67523620391604E-16));
#107187=DIRECTION('',(-1.,2.89708077091569E-28,-1.30472918803582E-12));
#107188=DIRECTION('center_axis',(0.,-1.,-2.67523620391604E-16));
#107189=DIRECTION('ref_axis',(-0.706962294833475,0.,-0.707251238022096));
#107190=DIRECTION('',(0.,-1.,-2.67523620391604E-16));
#107191=DIRECTION('center_axis',(0.,-1.,-2.22044604925031E-16));
#107192=DIRECTION('ref_axis',(-0.706962294833475,0.,-0.707251238022096));
#107193=DIRECTION('center_axis',(-0.999999916511834,1.09317472416619E-19,
-0.000408627366273673));
#107194=DIRECTION('ref_axis',(-0.000408627366273673,-2.22046620305031E-16,
0.999999916511834));
#107195=DIRECTION('',(0.,1.,2.67523620391604E-16));
#107196=DIRECTION('',(-0.000408627366274271,-2.29000492243171E-16,0.999999916511834));
#107197=DIRECTION('',(1.85839687592837E-20,1.,2.2204461251895E-16));
#107198=DIRECTION('',(-0.000408627366273673,-2.22044586386934E-16,0.999999916511834));
#107199=DIRECTION('center_axis',(-6.93889390390723E-18,-1.,-2.22049474265475E-16));
#107200=DIRECTION('ref_axis',(1.,-6.93889390390723E-18,1.54077774334651E-33));
#107201=DIRECTION('center_axis',(-6.93889390390723E-18,-1.,-2.22049474265475E-16));
#107202=DIRECTION('ref_axis',(0.,1.98254111540207E-16,-1.));
#107203=DIRECTION('center_axis',(-5.55111512312578E-15,0.,-1.));
#107204=DIRECTION('ref_axis',(-1.,0.,5.55111512312578E-15));
#107205=DIRECTION('center_axis',(-6.93889390390723E-18,-1.,-2.22049474265475E-16));
#107206=DIRECTION('ref_axis',(0.948334612654778,-7.70304532255269E-17,0.31727190616396));
#107207=DIRECTION('center_axis',(-0.60175986047648,0.,0.798677075118177));
#107208=DIRECTION('ref_axis',(0.,1.,0.));
#107209=DIRECTION('center_axis',(6.93889390390723E-18,1.,2.22049474265475E-16));
#107210=DIRECTION('ref_axis',(0.948334612654778,-7.2280144832367E-17,0.31727190616396));
#107211=DIRECTION('center_axis',(0.981039208710857,0.,0.193809367606358));
#107212=DIRECTION('ref_axis',(0.,1.,0.));
#107213=DIRECTION('center_axis',(-6.93889390390723E-18,-1.,-2.22049474265475E-16));
#107214=DIRECTION('ref_axis',(-0.934114852736577,-1.15648231731787E-16,
0.356972606647796));
#107215=DIRECTION('center_axis',(6.93889390390723E-18,1.,2.22049474265475E-16));
#107216=DIRECTION('ref_axis',(-0.934114852736577,-7.27838557761162E-17,
0.356972606647796));
#107217=DIRECTION('center_axis',(-6.93889390390723E-18,-1.,-2.22049474265475E-16));
#107218=DIRECTION('ref_axis',(0.,2.14881875733901E-16,-1.));
#107219=DIRECTION('center_axis',(0.899591968564469,0.,0.436731370632227));
#107220=DIRECTION('ref_axis',(0.,1.,0.));
#107221=DIRECTION('center_axis',(6.93889390390723E-18,1.,2.22049474265475E-16));
#107222=DIRECTION('ref_axis',(0.317889633169248,2.05596856412066E-16,-0.948127724055953));
#107223=DIRECTION('center_axis',(-6.93889390390723E-18,-1.,-2.22049474265475E-16));
#107224=DIRECTION('ref_axis',(0.317889633169248,2.08325460225432E-16,-0.948127724055953));
#107225=DIRECTION('center_axis',(6.93889390390723E-18,1.,2.22049474265475E-16));
#107226=DIRECTION('ref_axis',(0.,-2.22184532873183E-16,1.));
#107227=DIRECTION('center_axis',(0.990294325605679,0.,0.138986145616005));
#107228=DIRECTION('ref_axis',(0.,1.,0.));
#107229=DIRECTION('center_axis',(-6.93889390390723E-18,-1.,-2.22049474265475E-16));
#107230=DIRECTION('ref_axis',(-0.291409323841853,-2.08297999568609E-16,
0.956598455977237));
#107231=DIRECTION('center_axis',(6.93889390390723E-18,1.,2.22049474265475E-16));
#107232=DIRECTION('ref_axis',(-0.291409323841853,-2.10390125852163E-16,
0.956598455977237));
#107233=DIRECTION('center_axis',(-1.88182802673964E-12,0.,-1.));
#107234=DIRECTION('ref_axis',(0.,1.,0.));
#107235=DIRECTION('center_axis',(-6.93889390390723E-18,-1.,-2.22049474265475E-16));
#107236=DIRECTION('ref_axis',(0.656130266938607,-1.73472347597681E-16,0.754647648116041));
#107237=DIRECTION('center_axis',(6.93889390390723E-18,1.,2.22049474265475E-16));
#107238=DIRECTION('ref_axis',(0.656130266938607,-1.72121931829273E-16,0.754647648116041));
#107239=DIRECTION('center_axis',(-1.88215207428297E-12,2.22049474265488E-16,
-1.));
#107240=DIRECTION('ref_axis',(0.707106781186548,0.707106781186547,-1.3306533587345E-12));
#107241=DIRECTION('center_axis',(-1.88182802673964E-12,0.,-1.));
#107242=DIRECTION('ref_axis',(0.,1.,0.));
#107243=DIRECTION('',(1.88215207428297E-12,-2.22049474265488E-16,1.));
#107244=DIRECTION('',(-1.88215207428297E-12,2.22049474265488E-16,-1.));
#107245=DIRECTION('center_axis',(-6.93889390390723E-18,-1.,-2.22049474265475E-16));
#107246=DIRECTION('ref_axis',(0.,1.38777878078145E-16,-1.));
#107247=DIRECTION('center_axis',(0.707106781186549,0.,-0.707106781186546));
#107248=DIRECTION('ref_axis',(0.,1.,0.));
#107249=DIRECTION('center_axis',(6.93889390390723E-18,1.,2.22049474265475E-16));
#107250=DIRECTION('ref_axis',(-0.923879532511646,8.67361737988404E-17,-0.382683432364222));
#107251=DIRECTION('center_axis',(-6.93889390390723E-18,-1.,-2.22049474265475E-16));
#107252=DIRECTION('ref_axis',(-0.923879532511646,9.13853570226725E-17,-0.382683432364222));
#107253=DIRECTION('center_axis',(0.707106781186548,1.52106150078638E-16,
-0.707106781186547));
#107254=DIRECTION('ref_axis',(0.500000000000002,0.707106781186548,0.499999999999998));
#107255=DIRECTION('center_axis',(0.707106781186548,0.,-0.707106781186548));
#107256=DIRECTION('ref_axis',(0.,1.,0.));
#107257=DIRECTION('',(-0.707106781186548,-1.52106150078638E-16,0.707106781186547));
#107258=DIRECTION('',(0.707106781186548,1.52106150078638E-16,-0.707106781186547));
#107259=DIRECTION('center_axis',(0.,0.,-1.));
#107260=DIRECTION('ref_axis',(0.,1.,0.));
#107261=DIRECTION('center_axis',(-6.93889390390723E-18,-1.,-2.22049474265475E-16));
#107262=DIRECTION('ref_axis',(0.923879532511287,-8.67361737988403E-17,0.382683432365091));
#107263=DIRECTION('center_axis',(6.93889390390723E-18,1.,2.22049474265475E-16));
#107264=DIRECTION('ref_axis',(0.923879532511287,-9.1385357022863E-17,0.382683432365091));
#107265=DIRECTION('center_axis',(-8.32407533012986E-17,2.22049474265475E-16,
-1.));
#107266=DIRECTION('ref_axis',(0.707106781186551,0.707106781186544,0.));
#107267=DIRECTION('center_axis',(0.,0.,-1.));
#107268=DIRECTION('ref_axis',(0.,1.,0.));
#107269=DIRECTION('',(8.32407533012986E-17,-2.22049474265475E-16,1.));
#107270=DIRECTION('',(-8.32407533012986E-17,2.22049474265475E-16,-1.));
#107271=DIRECTION('center_axis',(-0.873688101364575,0.,0.486486486486485));
#107272=DIRECTION('ref_axis',(0.,1.,0.));
#107273=DIRECTION('center_axis',(-6.93889390390723E-18,-1.,-2.22049474265475E-16));
#107274=DIRECTION('ref_axis',(0.506711709709532,2.31296463463574E-16,-0.862115562580356));
#107275=DIRECTION('center_axis',(6.93889390390723E-18,1.,2.22049474265475E-16));
#107276=DIRECTION('ref_axis',(0.506711709709532,1.8791628863351E-16,-0.862115562580356));
#107277=DIRECTION('center_axis',(-6.93889390390723E-18,-1.,-2.22049474265475E-16));
#107278=DIRECTION('ref_axis',(-0.271927396983848,-1.70803542250024E-16,
0.962317770162013));
#107279=DIRECTION('center_axis',(-0.489871107039562,0.,-0.87179487179487));
#107280=DIRECTION('ref_axis',(0.,1.,0.));
#107281=DIRECTION('center_axis',(6.93889390390723E-18,1.,2.22049474265475E-16));
#107282=DIRECTION('ref_axis',(-0.271927396983848,-2.23835287222814E-16,
0.962317770162013));
#107283=DIRECTION('center_axis',(-6.93889390390723E-18,-1.,-2.22049474265475E-16));
#107284=DIRECTION('ref_axis',(-0.271927396983848,-2.11795279583562E-16,
0.962317770162013));
#107285=DIRECTION('center_axis',(0.,0.,1.));
#107286=DIRECTION('ref_axis',(0.,1.,0.));
#107287=DIRECTION('center_axis',(-6.93889390390723E-18,-1.,-2.22049474265475E-16));
#107288=DIRECTION('ref_axis',(-0.253184841770917,1.73472347597681E-16,-0.967417922046845));
#107289=DIRECTION('center_axis',(6.93889390390723E-18,1.,2.22049474265475E-16));
#107290=DIRECTION('ref_axis',(-0.253184841770917,2.16571463740626E-16,-0.967417922046845));
#107291=DIRECTION('center_axis',(0.,-2.22049474265475E-16,1.));
#107292=DIRECTION('ref_axis',(-0.707106781186548,0.707106781186547,0.));
#107293=DIRECTION('',(0.,2.22049474265475E-16,-1.));
#107294=DIRECTION('',(0.,-2.22049474265475E-16,1.));
#107295=DIRECTION('center_axis',(-1.13917782314015E-33,1.,1.88173394004264E-16));
#107296=DIRECTION('ref_axis',(0.923879532511287,0.,0.382683432365089));
#107297=DIRECTION('',(1.13917782314015E-33,-1.,-1.88173394004264E-16));
#107298=DIRECTION('center_axis',(0.,-1.,-2.22044604925031E-16));
#107299=DIRECTION('ref_axis',(0.923879532511287,0.,0.382683432365089));
#107300=DIRECTION('',(1.62923501610703E-32,1.,1.88173394004264E-16));
#107301=DIRECTION('center_axis',(1.,1.68028728913171E-32,-8.32407533012986E-17));
#107302=DIRECTION('ref_axis',(-8.32407533012986E-17,1.80520972702821E-16,
-1.));
#107303=DIRECTION('',(0.,1.,2.01858731750028E-16));
#107304=DIRECTION('',(-8.32407533012986E-17,2.22044604925031E-16,-1.));
#107305=DIRECTION('center_axis',(0.,-1.,-2.01858731750028E-16));
#107306=DIRECTION('ref_axis',(0.506711709709536,0.,-0.862115562580353));
#107307=DIRECTION('',(0.,-1.,-2.01858731750028E-16));
#107308=DIRECTION('center_axis',(0.,-1.,-2.22044604925031E-16));
#107309=DIRECTION('ref_axis',(0.506711709709536,0.,-0.862115562580353));
#107310=DIRECTION('center_axis',(0.,1.,2.01858731750028E-16));
#107311=DIRECTION('ref_axis',(1.,0.,-1.83750175990301E-19));
#107312=DIRECTION('',(0.,1.,0.));
#107313=DIRECTION('center_axis',(0.,-1.,-2.22044604925031E-16));
#107314=DIRECTION('ref_axis',(1.,0.,-1.83750175990301E-19));
#107315=DIRECTION('center_axis',(0.,-1.,0.));
#107316=DIRECTION('ref_axis',(1.,0.,0.));
#107317=DIRECTION('',(0.,-1.,0.));
#107318=DIRECTION('center_axis',(0.,-1.,-2.22044604925031E-16));
#107319=DIRECTION('ref_axis',(1.,0.,0.));
#107320=DIRECTION('center_axis',(-1.,0.,0.));
#107321=DIRECTION('ref_axis',(0.,-2.22044604925031E-16,1.));
#107322=DIRECTION('',(0.,1.,2.22044604925031E-16));
#107323=DIRECTION('',(0.,2.22049474265475E-16,-1.));
#107324=DIRECTION('center_axis',(0.,-1.,-2.22044604925031E-16));
#107325=DIRECTION('ref_axis',(0.707106781186548,-1.57009245868377E-16,0.707106781186548));
#107326=DIRECTION('',(0.,1.,2.22044604925031E-16));
#107327=DIRECTION('center_axis',(6.93889390390725E-18,1.,2.22049474265475E-16));
#107328=DIRECTION('ref_axis',(0.707106781186548,-1.57009245868377E-16,0.707106781186548));
#107329=DIRECTION('center_axis',(-6.93889390390723E-18,-1.,-2.22049474265475E-16));
#107330=DIRECTION('ref_axis',(1.,-6.93889390390723E-18,-1.83750175990301E-19));
#107331=DIRECTION('center_axis',(-6.93889390390721E-18,-1.,-2.22049474265475E-16));
#107332=DIRECTION('ref_axis',(0.,2.1779837001999E-16,-1.));
#107333=DIRECTION('center_axis',(0.995177777995763,0.,0.0980876658067449));
#107334=DIRECTION('ref_axis',(0.0980876658067449,-6.9388939039072E-16,-0.995177777995763));
#107335=DIRECTION('center_axis',(-6.93889390390721E-18,-1.,-2.22049474265475E-16));
#107336=DIRECTION('ref_axis',(-0.271646851952191,-2.11814819455226E-16,
0.962397001151014));
#107337=DIRECTION('center_axis',(-0.89959196856447,0.,-0.436731370632225));
#107338=DIRECTION('ref_axis',(0.,1.,0.));
#107339=DIRECTION('center_axis',(6.93889390390721E-18,1.,2.22049474265475E-16));
#107340=DIRECTION('ref_axis',(-0.271646851952191,-2.14187059826031E-16,
0.962397001151014));
#107341=DIRECTION('center_axis',(6.93889390390721E-18,1.,2.22049474265475E-16));
#107342=DIRECTION('ref_axis',(0.0641559653703721,2.22044604925031E-16,-0.997939884014762));
#107343=DIRECTION('center_axis',(-0.948108950182503,0.,0.317945622054827));
#107344=DIRECTION('ref_axis',(0.,1.,0.));
#107345=DIRECTION('center_axis',(-6.93889390390721E-18,-1.,-2.22049474265475E-16));
#107346=DIRECTION('ref_axis',(0.0641559653703722,2.25514051876985E-16,-0.997939884014762));
#107347=DIRECTION('center_axis',(6.93889390390721E-18,1.,2.22049474265475E-16));
#107348=DIRECTION('ref_axis',(0.0641559653703722,2.21146855157019E-16,-0.997939884014762));
#107349=DIRECTION('center_axis',(0.609084507830823,0.,0.793105328642094));
#107350=DIRECTION('ref_axis',(0.,1.,0.));
#107351=DIRECTION('center_axis',(-6.93889390390721E-18,-1.,-2.22049474265475E-16));
#107352=DIRECTION('ref_axis',(-0.956462973763756,1.15648231731787E-16,-0.291853695914566));
#107353=DIRECTION('center_axis',(6.93889390390721E-18,1.,2.22049474265475E-16));
#107354=DIRECTION('ref_axis',(-0.956462973763756,7.14427548382275E-17,-0.291853695914567));
#107355=DIRECTION('center_axis',(-6.93889390390721E-18,-1.,-2.22049474265475E-16));
#107356=DIRECTION('ref_axis',(0.,2.11471052309554E-16,-1.));
#107357=DIRECTION('center_axis',(-0.0951854606398691,0.,0.995459556226558));
#107358=DIRECTION('ref_axis',(0.,1.,0.));
#107359=DIRECTION('center_axis',(6.93889390390721E-18,1.,2.22049474265475E-16));
#107360=DIRECTION('ref_axis',(0.9611140067488,5.72279909600596E-17,-0.27615188942187));
#107361=DIRECTION('center_axis',(-6.93889390390721E-18,-1.,-2.22049474265475E-16));
#107362=DIRECTION('ref_axis',(0.961114006748799,5.46503137411547E-17,-0.27615188942187));
#107363=DIRECTION('center_axis',(0.957454413658976,-1.00122880701227E-16,
0.288584555659077));
#107364=DIRECTION('ref_axis',(0.,1.,3.46944695195361E-16));
#107365=DIRECTION('center_axis',(-6.93889390390721E-18,-1.,-2.22049474265475E-16));
#107366=DIRECTION('ref_axis',(-0.830183712534771,-1.15648231731787E-16,
0.557489913309635));
#107367=DIRECTION('center_axis',(6.93889390390721E-18,1.,2.22049474265475E-16));
#107368=DIRECTION('ref_axis',(-0.830183712534771,-1.18029785456679E-16,
0.557489913309635));
#107369=DIRECTION('center_axis',(6.93889390390721E-18,1.,2.22049474265475E-16));
#107370=DIRECTION('ref_axis',(0.,-2.17002965587602E-16,1.));
#107371=DIRECTION('center_axis',(0.998182760026068,0.,0.0602592531213423));
#107372=DIRECTION('ref_axis',(0.,1.,0.));
#107373=DIRECTION('center_axis',(-6.93889390390721E-18,-1.,-2.22049474265475E-16));
#107374=DIRECTION('ref_axis',(-0.17560666354258,-2.1939638064923E-16,0.984460410437841));
#107375=DIRECTION('center_axis',(6.93889390390721E-18,1.,2.22049474265475E-16));
#107376=DIRECTION('ref_axis',(-0.17560666354258,-2.17380400565755E-16,0.984460410437841));
#107377=DIRECTION('center_axis',(-1.88182802673964E-12,0.,-1.));
#107378=DIRECTION('ref_axis',(0.,1.,0.));
#107379=DIRECTION('center_axis',(-6.93889390390721E-18,-1.,-2.22049474265475E-16));
#107380=DIRECTION('ref_axis',(0.685470913635486,-1.73472347597681E-16,0.72810001137188));
#107381=DIRECTION('center_axis',(6.93889390390721E-18,1.,2.22049474265475E-16));
#107382=DIRECTION('ref_axis',(0.685470913635486,-1.66430634681743E-16,0.72810001137188));
#107383=DIRECTION('center_axis',(-1.88215207428297E-12,2.22049474265488E-16,
-1.));
#107384=DIRECTION('ref_axis',(0.707106781186544,0.707106781186551,-1.33071469047117E-12));
#107385=DIRECTION('center_axis',(-1.88182802673965E-12,1.38777878078145E-15,
-1.));
#107386=DIRECTION('ref_axis',(0.,1.,1.38777878078145E-15));
#107387=DIRECTION('',(1.88215207428297E-12,-2.22049474265488E-16,1.));
#107388=DIRECTION('',(-1.88215207428297E-12,2.22049474265488E-16,-1.));
#107389=DIRECTION('center_axis',(-6.93889390390721E-18,-1.,-2.22049474265475E-16));
#107390=DIRECTION('ref_axis',(0.740974920562387,1.73472347597681E-16,-0.671532699946595));
#107391=DIRECTION('center_axis',(6.93889390390721E-18,1.,2.22049474265475E-16));
#107392=DIRECTION('ref_axis',(0.740974920562387,1.43971936615978E-16,-0.671532699946595));
#107393=DIRECTION('center_axis',(0.,1.,2.01858731750028E-16));
#107394=DIRECTION('ref_axis',(0.229951641166733,-1.9644933285631E-16,0.973202056473745));
#107395=DIRECTION('',(0.,1.,2.01858731750028E-16));
#107396=DIRECTION('center_axis',(0.,-1.,-2.22044604925031E-16));
#107397=DIRECTION('ref_axis',(0.229951641166733,-1.9644933285631E-16,0.973202056473745));
#107398=DIRECTION('',(0.,-1.,-2.01858731750028E-16));
#107399=DIRECTION('center_axis',(3.79928830675489E-29,-1.,-2.01858731750026E-16));
#107400=DIRECTION('ref_axis',(0.685470913635487,0.,0.728100011371879));
#107401=DIRECTION('',(3.79928830675489E-29,-1.,-2.01858731750026E-16));
#107402=DIRECTION('center_axis',(-6.93889390390721E-18,-1.,-2.22049474265475E-16));
#107403=DIRECTION('ref_axis',(0.685470913635487,0.,0.728100011371879));
#107404=DIRECTION('center_axis',(-1.,-4.1792171374299E-28,1.88215207428297E-12));
#107405=DIRECTION('ref_axis',(-1.88215207428297E-12,2.22049474265488E-16,
-1.));
#107406=DIRECTION('',(-3.79928830675446E-29,1.,2.01858731750028E-16));
#107407=DIRECTION('',(-1.88215207428297E-12,2.22049474265488E-16,-1.));
#107408=DIRECTION('center_axis',(0.,1.,2.01858731750028E-16));
#107409=DIRECTION('ref_axis',(0.740974920562388,0.,-0.671532699946594));
#107410=DIRECTION('',(0.,-1.,-2.01858731750028E-16));
#107411=DIRECTION('center_axis',(-6.93889390390721E-18,-1.,-2.22049474265475E-16));
#107412=DIRECTION('ref_axis',(0.740974920562388,0.,-0.671532699946594));
#107413=DIRECTION('center_axis',(0.,1.,2.01858731750028E-16));
#107414=DIRECTION('ref_axis',(0.425760116003353,-1.82649062652652E-16,0.904836075552258));
#107415=DIRECTION('',(0.,1.,2.01858731750028E-16));
#107416=DIRECTION('center_axis',(0.,-1.,-2.22044604925031E-16));
#107417=DIRECTION('ref_axis',(0.89959196856447,-9.69738446503996E-17,0.436731370632224));
#107418=DIRECTION('center_axis',(-6.93889390390721E-18,-1.,-2.22049474265475E-16));
#107419=DIRECTION('ref_axis',(1.,-6.93889390390721E-18,-1.83750175990301E-19));
#107420=DIRECTION('center_axis',(-6.93889390390721E-18,-1.,-2.22049474265475E-16));
#107421=DIRECTION('ref_axis',(0.,2.01858731750028E-16,-1.));
#107422=DIRECTION('center_axis',(-0.961527331301806,0.,-0.274709284807824));
#107423=DIRECTION('ref_axis',(-0.274709284807824,0.,0.961527331301806));
#107424=DIRECTION('center_axis',(-6.93889390390721E-18,-1.,-2.22049474265475E-16));
#107425=DIRECTION('ref_axis',(0.544438391932684,1.82477483735409E-16,-0.838800832969158));
#107426=DIRECTION('center_axis',(0.642414549106759,0.,0.766357323378566));
#107427=DIRECTION('ref_axis',(0.,1.,0.));
#107428=DIRECTION('center_axis',(6.93889390390721E-18,1.,2.22049474265475E-16));
#107429=DIRECTION('ref_axis',(0.544438391932684,1.92747052886312E-16,-0.838800832969158));
#107430=DIRECTION('center_axis',(0.979447089047538,0.,0.201701263645781));
#107431=DIRECTION('ref_axis',(0.,1.,0.));
#107432=DIRECTION('center_axis',(-6.93889390390721E-18,-1.,-2.22049474265475E-16));
#107433=DIRECTION('ref_axis',(-0.512525209353285,-1.73472347597681E-16,
0.858672178294703));
#107434=DIRECTION('center_axis',(6.93889390390721E-18,1.,2.22049474265475E-16));
#107435=DIRECTION('ref_axis',(-0.512525209353286,-1.87111347705949E-16,
0.858672178294703));
#107436=DIRECTION('center_axis',(6.93889390390721E-18,1.,2.22049474265475E-16));
#107437=DIRECTION('ref_axis',(0.,-2.15078296159505E-16,1.));
#107438=DIRECTION('center_axis',(0.997789534013799,0.,0.0664533356012022));
#107439=DIRECTION('ref_axis',(0.,1.,0.));
#107440=DIRECTION('center_axis',(-6.93889390390721E-18,-1.,-2.22049474265475E-16));
#107441=DIRECTION('ref_axis',(-0.134390600847534,-2.1916945940167E-16,0.990928436570391));
#107442=DIRECTION('center_axis',(6.93889390390721E-18,1.,2.22049474265475E-16));
#107443=DIRECTION('ref_axis',(-0.134390600847534,-2.19102616254201E-16,
0.990928436570391));
#107444=DIRECTION('center_axis',(-6.93889390390721E-18,-1.,-2.22049474265475E-16));
#107445=DIRECTION('ref_axis',(0.,1.8503717077086E-16,-1.));
#107446=DIRECTION('center_axis',(0.0349202536836706,0.,0.999390101953521));
#107447=DIRECTION('ref_axis',(0.,1.,0.));
#107448=DIRECTION('center_axis',(6.93889390390721E-18,1.,2.22049474265475E-16));
#107449=DIRECTION('ref_axis',(0.718181642132044,1.73472347597681E-16,-0.695855681089492));
#107450=DIRECTION('center_axis',(-6.93889390390721E-18,-1.,-2.22049474265475E-16));
#107451=DIRECTION('ref_axis',(0.718181642132044,1.49531001932078E-16,-0.695855681089492));
#107452=DIRECTION('center_axis',(-6.93889390390721E-18,-1.,-2.22049474265475E-16));
#107453=DIRECTION('ref_axis',(0.,2.06553120860494E-16,-1.));
#107454=DIRECTION('center_axis',(0.0174573777538545,0.,0.999847608369375));
#107455=DIRECTION('ref_axis',(0.,1.,0.));
#107456=DIRECTION('center_axis',(6.93889390390721E-18,1.,2.22049474265475E-16));
#107457=DIRECTION('ref_axis',(0.999656987972984,0.,-0.0261898147527144));
#107458=DIRECTION('center_axis',(-6.93889390390721E-18,-1.,-2.22049474265475E-16));
#107459=DIRECTION('ref_axis',(0.999656987972984,-1.12107918289356E-18,-0.0261898147527144));
#107460=DIRECTION('center_axis',(0.999631786816462,0.,0.0271346786627047));
#107461=DIRECTION('ref_axis',(0.,1.,0.));
#107462=DIRECTION('center_axis',(-6.93889390390721E-18,-1.,-2.22049474265475E-16));
#107463=DIRECTION('ref_axis',(-0.71052079274556,-1.73472347597681E-16,0.703676206131926));
#107464=DIRECTION('center_axis',(6.93889390390721E-18,1.,2.22049474265475E-16));
#107465=DIRECTION('ref_axis',(-0.71052079274556,-1.51320703227337E-16,0.703676206131926));
#107466=DIRECTION('center_axis',(0.999631786816462,-1.29615800431083E-17,
0.0271346786627023));
#107467=DIRECTION('ref_axis',(-0.0191871152877203,0.707106781186547,0.706846415147545));
#107468=DIRECTION('center_axis',(0.999631786816462,0.,0.0271346786627047));
#107469=DIRECTION('ref_axis',(0.,1.,0.));
#107470=DIRECTION('',(-0.999631786816462,1.29615800431083E-17,-0.0271346786627023));
#107471=DIRECTION('',(0.999631786816462,-1.29615800431083E-17,0.0271346786627023));
#107472=DIRECTION('center_axis',(0.,0.,-1.));
#107473=DIRECTION('ref_axis',(0.,1.,0.));
#107474=DIRECTION('center_axis',(-6.93889390390721E-18,-1.,-2.22049474265475E-16));
#107475=DIRECTION('ref_axis',(0.697447245796159,-1.15648231731787E-16,0.716636127564995));
#107476=DIRECTION('center_axis',(6.93889390390721E-18,1.,2.22049474265475E-16));
#107477=DIRECTION('ref_axis',(0.69744724579616,-1.63968187807605E-16,0.716636127564995));
#107478=DIRECTION('center_axis',(-8.32407533012986E-17,2.22049474265475E-16,
-1.));
#107479=DIRECTION('ref_axis',(0.707106781186548,0.707106781186547,0.));
#107480=DIRECTION('center_axis',(0.,0.,-1.));
#107481=DIRECTION('ref_axis',(0.,1.,0.));
#107482=DIRECTION('',(8.32407533012986E-17,-2.22049474265475E-16,1.));
#107483=DIRECTION('',(-8.32407533012986E-17,2.22049474265475E-16,-1.));
#107484=DIRECTION('center_axis',(-0.70710678118655,0.,-0.707106781186545));
#107485=DIRECTION('ref_axis',(0.,1.,0.));
#107486=DIRECTION('center_axis',(-6.93889390390721E-18,-1.,-2.22049474265475E-16));
#107487=DIRECTION('ref_axis',(0.923879532511286,8.67361737988402E-17,-0.382683432365091));
#107488=DIRECTION('center_axis',(6.93889390390721E-18,1.,2.22049474265475E-16));
#107489=DIRECTION('ref_axis',(0.923879532511286,7.85639529106886E-17,-0.382683432365091));
#107490=DIRECTION('center_axis',(-0.707106781186547,1.61919227945412E-16,
-0.707106781186548));
#107491=DIRECTION('ref_axis',(0.500000000000001,0.707106781186546,-0.500000000000001));
#107492=DIRECTION('center_axis',(-0.707106781186548,0.,-0.707106781186548));
#107493=DIRECTION('ref_axis',(0.,1.,0.));
#107494=DIRECTION('',(0.707106781186547,-1.61919227945412E-16,0.707106781186548));
#107495=DIRECTION('',(-0.707106781186547,1.61919227945412E-16,-0.707106781186548));
#107496=DIRECTION('center_axis',(-0.999306434017034,0.,0.0372377621797867));
#107497=DIRECTION('ref_axis',(0.,1.,0.));
#107498=DIRECTION('center_axis',(-6.93889390390721E-18,-1.,-2.22049474265475E-16));
#107499=DIRECTION('ref_axis',(0.365412486013864,1.73472347597681E-16,-0.930845698848723));
#107500=DIRECTION('center_axis',(6.93889390390721E-18,1.,2.22049474265475E-16));
#107501=DIRECTION('ref_axis',(0.365412486013864,2.04158239580024E-16,-0.930845698848723));
#107502=DIRECTION('center_axis',(-6.93889390390721E-18,-1.,-2.22049474265475E-16));
#107503=DIRECTION('ref_axis',(-0.123085713533701,-2.13127337608609E-16,
0.992396043484606));
#107504=DIRECTION('center_axis',(-0.959930094890458,0.,-0.280239563451696));
#107505=DIRECTION('ref_axis',(0.,1.,0.));
#107506=DIRECTION('center_axis',(6.93889390390721E-18,1.,2.22049474265475E-16));
#107507=DIRECTION('ref_axis',(-0.1230857135337,-2.19181085988492E-16,0.992396043484606));
#107508=DIRECTION('center_axis',(-6.93889390390721E-18,-1.,-2.22049474265475E-16));
#107509=DIRECTION('ref_axis',(-0.1230857135337,-2.19506941011597E-16,0.992396043484606));
#107510=DIRECTION('center_axis',(-0.360174124451025,0.,0.932885094787101));
#107511=DIRECTION('ref_axis',(0.,1.,0.));
#107512=DIRECTION('center_axis',(-6.93889390390721E-18,-1.,-2.22049474265475E-16));
#107513=DIRECTION('ref_axis',(-0.44318546164383,2.31296463463574E-16,-0.896429945164454));
#107514=DIRECTION('center_axis',(6.93889390390721E-18,1.,2.22049474265475E-16));
#107515=DIRECTION('ref_axis',(-0.44318546164383,2.02127014937696E-16,-0.896429945164454));
#107516=DIRECTION('center_axis',(-6.93889390390721E-18,-1.,-2.22049474265475E-16));
#107517=DIRECTION('ref_axis',(0.,2.11471052309554E-16,-1.));
#107518=DIRECTION('center_axis',(-0.598212156168195,0.,0.801337766620667));
#107519=DIRECTION('ref_axis',(0.,1.,0.));
#107520=DIRECTION('center_axis',(6.93889390390721E-18,1.,2.22049474265475E-16));
#107521=DIRECTION('ref_axis',(0.875241543457166,-1.14455981920119E-16,0.483686097181549));
#107522=DIRECTION('center_axis',(-6.93889390390721E-18,-1.,-2.22049474265475E-16));
#107523=DIRECTION('ref_axis',(0.875241543457166,-1.13475451799024E-16,0.483686097181549));
#107524=DIRECTION('center_axis',(-6.93889390390721E-18,-1.,-2.22049474265475E-16));
#107525=DIRECTION('ref_axis',(-0.947452442825118,-1.15648231731787E-16,
0.319896652975169));
#107526=DIRECTION('center_axis',(6.93889390390721E-18,1.,2.22049474265475E-16));
#107527=DIRECTION('ref_axis',(-0.947452442825118,-6.44586116326602E-17,
0.319896652975169));
#107528=DIRECTION('center_axis',(1.13917782314015E-33,-1.,-1.88173394004264E-16));
#107529=DIRECTION('ref_axis',(0.923879532511287,0.,-0.382683432365089));
#107530=DIRECTION('',(-1.62923501610704E-32,-1.,-1.88173394004264E-16));
#107531=DIRECTION('center_axis',(0.,-1.,-2.22044604925031E-16));
#107532=DIRECTION('ref_axis',(0.923879532511287,0.,-0.382683432365089));
#107533=DIRECTION('',(-1.13917782314014E-33,1.,1.88173394004264E-16));
#107534=DIRECTION('center_axis',(-0.707106781186548,-1.33058682939303E-16,
0.707106781186547));
#107535=DIRECTION('ref_axis',(-0.707106781186547,1.61919227945412E-16,-0.707106781186548));
#107536=DIRECTION('',(0.,1.,1.88173394004264E-16));
#107537=DIRECTION('',(-0.707106781186547,1.61919227945412E-16,-0.707106781186548));
#107538=DIRECTION('center_axis',(0.,1.,1.88173394004264E-16));
#107539=DIRECTION('ref_axis',(0.365412486013864,0.,-0.930845698848723));
#107540=DIRECTION('',(0.,-1.,-1.88173394004264E-16));
#107541=DIRECTION('center_axis',(0.,-1.,-2.22044604925031E-16));
#107542=DIRECTION('ref_axis',(0.365412486013864,0.,-0.930845698848723));
#107543=DIRECTION('center_axis',(0.,1.,1.88173394004264E-16));
#107544=DIRECTION('ref_axis',(0.13797098470004,-1.86373754703504E-16,0.99043627123652));
#107545=DIRECTION('',(0.,1.,1.88173394004264E-16));
#107546=DIRECTION('center_axis',(0.,-1.,-2.22044604925031E-16));
#107547=DIRECTION('ref_axis',(0.13797098470004,-1.86373754703504E-16,0.99043627123652));
#107548=DIRECTION('center_axis',(0.,1.,2.01858731750028E-16));
#107549=DIRECTION('ref_axis',(-0.443185461643831,0.,-0.896429945164453));
#107550=DIRECTION('',(0.,-1.,-2.01858731750028E-16));
#107551=DIRECTION('center_axis',(0.,-1.,-2.22044604925031E-16));
#107552=DIRECTION('ref_axis',(-0.443185461643831,0.,-0.896429945164453));
#107553=DIRECTION('center_axis',(0.,1.,2.01858731750028E-16));
#107554=DIRECTION('ref_axis',(-0.984274724761795,3.56572272070144E-17,-0.176644462678833));
#107555=DIRECTION('',(0.,1.,2.01858731750028E-16));
#107556=DIRECTION('center_axis',(0.,-1.,-2.22044604925031E-16));
#107557=DIRECTION('ref_axis',(-0.984274724761795,3.56572272070144E-17,-0.176644462678833));
#107558=DIRECTION('center_axis',(0.,1.,2.00642715293703E-16));
#107559=DIRECTION('ref_axis',(-0.947452442825118,0.,0.319896652975169));
#107560=DIRECTION('',(0.,-1.,-2.00642715293703E-16));
#107561=DIRECTION('center_axis',(0.,-1.,-2.22044604925031E-16));
#107562=DIRECTION('ref_axis',(-0.947452442825118,0.,0.319896652975169));
#107563=DIRECTION('center_axis',(0.,1.,2.00642715293703E-16));
#107564=DIRECTION('ref_axis',(1.,0.,1.39223851401487E-33));
#107565=DIRECTION('',(0.,1.,2.00642715293703E-16));
#107566=DIRECTION('center_axis',(0.,-1.,-2.22044604925031E-16));
#107567=DIRECTION('ref_axis',(1.,0.,1.39223851401487E-33));
#107568=DIRECTION('',(0.,-1.,-2.00642715293703E-16));
#107569=DIRECTION('center_axis',(-6.93889390390723E-18,-1.,-2.22049474265475E-16));
#107570=DIRECTION('ref_axis',(1.,-6.93889390390723E-18,-1.83750175990302E-19));
#107571=DIRECTION('center_axis',(-6.93889390390721E-18,-1.,-2.22049474265475E-16));
#107572=DIRECTION('ref_axis',(1.,-6.93889390390721E-18,-1.83750175990301E-19));
#107573=DIRECTION('center_axis',(-6.93889390390725E-18,-1.,-2.22049474265475E-16));
#107574=DIRECTION('ref_axis',(0.,2.03710646720212E-16,-1.));
#107575=DIRECTION('center_axis',(-0.00645890109586822,0.,-0.99997914108077));
#107576=DIRECTION('ref_axis',(-0.99997914108077,0.,0.00645890109586822));
#107577=DIRECTION('center_axis',(-6.93889390390725E-18,-1.,-2.22049474265475E-16));
#107578=DIRECTION('ref_axis',(0.813766779597698,-1.34699921502175E-16,0.581191559146545));
#107579=DIRECTION('center_axis',(-0.947984515197821,0.,0.31831644466655));
#107580=DIRECTION('ref_axis',(0.,1.,0.));
#107581=DIRECTION('center_axis',(6.93889390390725E-18,1.,2.22049474265475E-16));
#107582=DIRECTION('ref_axis',(0.813766779597698,-1.34301172333688E-16,0.581191559146545));
#107583=DIRECTION('center_axis',(0.989904612137255,0.,0.141735171603208));
#107584=DIRECTION('ref_axis',(0.,1.,0.));
#107585=DIRECTION('center_axis',(-6.93889390390725E-18,-1.,-2.22049474265475E-16));
#107586=DIRECTION('ref_axis',(-0.995874208858217,0.,0.0907444771378411));
#107587=DIRECTION('center_axis',(6.93889390390725E-18,1.,2.22049474265475E-16));
#107588=DIRECTION('ref_axis',(-0.995874208858217,-1.32394979640483E-17,
0.0907444771378411));
#107589=DIRECTION('center_axis',(6.93889390390725E-18,1.,2.22049474265475E-16));
#107590=DIRECTION('ref_axis',(0.,-2.1541640776309E-16,1.));
#107591=DIRECTION('center_axis',(1.,0.,0.));
#107592=DIRECTION('ref_axis',(0.,1.,0.));
#107593=DIRECTION('center_axis',(-6.93889390390725E-18,-1.,-2.22049474265475E-16));
#107594=DIRECTION('ref_axis',(-0.0710471247227679,-2.22665998408963E-16,
0.997472960068907));
#107595=DIRECTION('center_axis',(6.93889390390725E-18,1.,2.22049474265475E-16));
#107596=DIRECTION('ref_axis',(-0.0710471247227679,-2.20995357916699E-16,
0.997472960068907));
#107597=DIRECTION('center_axis',(1.,-6.93889390390718E-18,-3.2590836004222E-16));
#107598=DIRECTION('ref_axis',(0.,0.707106781186547,0.707106781186548));
#107599=DIRECTION('center_axis',(1.,0.,1.38777878078144E-15));
#107600=DIRECTION('ref_axis',(0.,1.,0.));
#107601=DIRECTION('',(-1.,6.93889390390718E-18,3.2590836004222E-16));
#107602=DIRECTION('',(1.,-6.93889390390718E-18,-3.2590836004222E-16));
#107603=DIRECTION('center_axis',(0.472653347758817,0.,-0.881248439914865));
#107604=DIRECTION('ref_axis',(0.,1.,0.));
#107605=DIRECTION('center_axis',(-6.93889390390725E-18,-1.,-2.22049474265475E-16));
#107606=DIRECTION('ref_axis',(0.51349131065734,-1.73472347597681E-16,0.858094793061587));
#107607=DIRECTION('center_axis',(6.93889390390725E-18,1.,2.22049474265475E-16));
#107608=DIRECTION('ref_axis',(0.51349131065734,-1.94102559394496E-16,0.858094793061587));
#107609=DIRECTION('center_axis',(6.93889390390725E-18,1.,2.22049474265475E-16));
#107610=DIRECTION('ref_axis',(0.,-2.22044604925031E-16,1.));
#107611=DIRECTION('center_axis',(0.00430977270832746,0.,-0.999990712886476));
#107612=DIRECTION('ref_axis',(0.,1.,0.));
#107613=DIRECTION('center_axis',(-6.93889390390725E-18,-1.,-2.22049474265475E-16));
#107614=DIRECTION('ref_axis',(0.969330497601796,-5.78241158658936E-17,0.24576083174309));
#107615=DIRECTION('center_axis',(6.93889390390725E-18,1.,2.22049474265475E-16));
#107616=DIRECTION('ref_axis',(0.969330497601796,-6.12971449642794E-17,0.24576083174309));
#107617=DIRECTION('center_axis',(-0.96830751921471,0.,0.249760982205497));
#107618=DIRECTION('ref_axis',(0.,1.,0.));
#107619=DIRECTION('center_axis',(-6.93889390390725E-18,-1.,-2.22049474265475E-16));
#107620=DIRECTION('ref_axis',(0.614172012824047,1.73472347597681E-16,-0.789172185688053));
#107621=DIRECTION('center_axis',(6.93889390390725E-18,1.,2.22049474265475E-16));
#107622=DIRECTION('ref_axis',(0.614172012824046,1.70973594501233E-16,-0.789172185688053));
#107623=DIRECTION('center_axis',(-6.93889390390725E-18,-1.,-2.22049474265475E-16));
#107624=DIRECTION('ref_axis',(-0.0145150489551482,-2.03710646725265E-16,
0.999894651127722));
#107625=DIRECTION('center_axis',(-0.960649678360777,0.,-0.277762840324864));
#107626=DIRECTION('ref_axis',(0.,1.,0.));
#107627=DIRECTION('center_axis',(6.93889390390725E-18,1.,2.22049474265475E-16));
#107628=DIRECTION('ref_axis',(-0.0145150489551485,-2.19846143496015E-16,
0.999894651127722));
#107629=DIRECTION('center_axis',(-6.93889390390725E-18,-1.,-2.22049474265475E-16));
#107630=DIRECTION('ref_axis',(-0.0145150489551485,-2.21925363219061E-16,
0.999894651127722));
#107631=DIRECTION('center_axis',(-6.93889390390725E-18,-1.,-2.22049474265475E-16));
#107632=DIRECTION('ref_axis',(-0.603509608361002,1.73472347597681E-16,-0.797355725266929));
#107633=DIRECTION('center_axis',(6.93889390390725E-18,1.,2.22049474265475E-16));
#107634=DIRECTION('ref_axis',(-0.603509608361002,1.81240108740494E-16,-0.797355725266929));
#107635=DIRECTION('center_axis',(0.,-1.,-2.22044604925031E-16));
#107636=DIRECTION('ref_axis',(0.957056520812277,-6.43710396276775E-17,0.28990139008066));
#107637=DIRECTION('',(0.,1.,2.22044604925031E-16));
#107638=DIRECTION('center_axis',(0.,-1.,-2.22044604925031E-16));
#107639=DIRECTION('ref_axis',(-1.,0.,0.));
#107640=DIRECTION('',(0.,1.,2.22044604925031E-16));
#107641=DIRECTION('center_axis',(0.,1.,2.22044604925031E-16));
#107642=DIRECTION('ref_axis',(-1.,0.,0.));
#107643=DIRECTION('',(0.,-1.,-2.22044604925031E-16));
#107644=DIRECTION('center_axis',(0.,-1.,-2.22044604925031E-16));
#107645=DIRECTION('ref_axis',(-1.,0.,0.));
#107646=DIRECTION('',(0.,-1.,-2.22044604925031E-16));
#107647=DIRECTION('center_axis',(0.,1.,0.));
#107648=DIRECTION('ref_axis',(0.614172012824043,0.,-0.789172185688056));
#107649=DIRECTION('',(0.,-1.,0.));
#107650=DIRECTION('center_axis',(0.,-1.,-2.22044604925031E-16));
#107651=DIRECTION('ref_axis',(0.614172012824043,0.,-0.789172185688056));
#107652=DIRECTION('center_axis',(0.,1.,0.));
#107653=DIRECTION('ref_axis',(0.414254853160806,0.,0.910160928975046));
#107654=DIRECTION('',(0.,1.,0.));
#107655=DIRECTION('center_axis',(0.,-1.,-2.22044604925031E-16));
#107656=DIRECTION('ref_axis',(0.414254853160806,0.,0.910160928975046));
#107657=DIRECTION('center_axis',(0.,1.,0.));
#107658=DIRECTION('ref_axis',(-0.603509608361001,0.,-0.79735572526693));
#107659=DIRECTION('',(0.,-1.,0.));
#107660=DIRECTION('center_axis',(0.,-1.,-2.22044604925031E-16));
#107661=DIRECTION('ref_axis',(-0.603509608361001,0.,-0.79735572526693));
#107662=DIRECTION('center_axis',(0.,1.,0.));
#107663=DIRECTION('ref_axis',(1.,0.,-1.83750175990302E-19));
#107664=DIRECTION('',(0.,1.,0.));
#107665=DIRECTION('center_axis',(0.,-1.,-2.22044604925031E-16));
#107666=DIRECTION('ref_axis',(1.,0.,-1.83750175990302E-19));
#107667=DIRECTION('center_axis',(-6.93889390390725E-18,-1.,-2.22049474265475E-16));
#107668=DIRECTION('ref_axis',(1.,-6.93889390390725E-18,-1.83750175990301E-19));
#107669=DIRECTION('center_axis',(1.,-6.93889390390718E-18,-2.46926126761481E-16));
#107670=DIRECTION('ref_axis',(0.,0.707106781186548,0.707106781186548));
#107671=DIRECTION('center_axis',(-1.,0.,0.));
#107672=DIRECTION('ref_axis',(0.,0.,1.));
#107673=DIRECTION('',(1.,-6.93889390390718E-18,-2.46926126761481E-16));
#107674=DIRECTION('center_axis',(1.,0.,0.));
#107675=DIRECTION('ref_axis',(0.,1.,0.));
#107676=DIRECTION('',(-1.,6.93889390390718E-18,2.46926126761481E-16));
#107677=DIRECTION('center_axis',(0.,0.,-1.));
#107678=DIRECTION('ref_axis',(0.,1.,0.));
#107679=DIRECTION('center_axis',(-6.93889390390723E-18,-1.,-2.22049474265475E-16));
#107680=DIRECTION('ref_axis',(0.707106781186548,-1.15648231731787E-16,0.707106781186547));
#107681=DIRECTION('center_axis',(6.93889390390723E-18,1.,2.22049474265475E-16));
#107682=DIRECTION('ref_axis',(0.707106781186548,-1.61919227945412E-16,0.707106781186547));
#107683=DIRECTION('center_axis',(1.54077774334651E-33,2.22049474265475E-16,
-1.));
#107684=DIRECTION('ref_axis',(0.707106781186548,0.707106781186547,0.));
#107685=DIRECTION('center_axis',(0.,0.,-1.));
#107686=DIRECTION('ref_axis',(0.,1.,0.));
#107687=DIRECTION('',(-1.54077774334651E-33,-2.22049474265475E-16,1.));
#107688=DIRECTION('',(1.54077774334651E-33,2.22049474265475E-16,-1.));
#107689=DIRECTION('center_axis',(-0.845470457966937,0.,0.534022194955582));
#107690=DIRECTION('ref_axis',(0.,1.,0.));
#107691=DIRECTION('center_axis',(-6.93889390390723E-18,-1.,-2.22049474265475E-16));
#107692=DIRECTION('ref_axis',(0.482689240114392,2.31296463463574E-16,-0.875791697538741));
#107693=DIRECTION('center_axis',(6.93889390390723E-18,1.,2.22049474265475E-16));
#107694=DIRECTION('ref_axis',(0.482689240114392,1.91119756578834E-16,-0.875791697538742));
#107695=DIRECTION('center_axis',(-6.93889390390723E-18,-1.,-2.22049474265475E-16));
#107696=DIRECTION('ref_axis',(0.00955154174511641,-2.01858731750028E-16,
0.99995438298469));
#107697=DIRECTION('center_axis',(-0.855517195345567,0.,-0.517774399201095));
#107698=DIRECTION('ref_axis',(0.,1.,0.));
#107699=DIRECTION('center_axis',(6.93889390390723E-18,1.,2.22049474265475E-16));
#107700=DIRECTION('ref_axis',(0.00955154174511598,-2.31296463463574E-16,
0.99995438298469));
#107701=DIRECTION('center_axis',(-6.93889390390723E-18,-1.,-2.22049474265475E-16));
#107702=DIRECTION('ref_axis',(0.00955154174511598,-2.22105622165996E-16,
0.99995438298469));
#107703=DIRECTION('center_axis',(-0.238180414155802,0.,0.971220927653729));
#107704=DIRECTION('ref_axis',(0.,1.,0.));
#107705=DIRECTION('center_axis',(-6.93889390390723E-18,-1.,-2.22049474265475E-16));
#107706=DIRECTION('ref_axis',(-0.382987746401723,2.31296463463574E-16,-0.923753422784527));
#107707=DIRECTION('center_axis',(6.93889390390723E-18,1.,2.22049474265475E-16));
#107708=DIRECTION('ref_axis',(-0.382987746401723,2.07776473219015E-16,-0.923753422784527));
#107709=DIRECTION('center_axis',(-6.93889390390723E-18,-1.,-2.22049474265475E-16));
#107710=DIRECTION('ref_axis',(0.,2.22044604925031E-16,-1.));
#107711=DIRECTION('center_axis',(-0.369109963398455,0.,0.929385729888291));
#107712=DIRECTION('ref_axis',(0.,1.,0.));
#107713=DIRECTION('center_axis',(6.93889390390723E-18,1.,2.22049474265475E-16));
#107714=DIRECTION('ref_axis',(0.952555538217842,-7.35943292838645E-17,0.304364824857469));
#107715=DIRECTION('center_axis',(-6.93889390390723E-18,-1.,-2.22049474265475E-16));
#107716=DIRECTION('ref_axis',(0.952555538217842,-7.41937311617772E-17,0.304364824857469));
#107717=DIRECTION('center_axis',(-6.93889390390723E-18,-1.,-2.22049474265475E-16));
#107718=DIRECTION('ref_axis',(-0.82737837879608,-1.15648231731787E-16,0.561644921904196));
#107719=DIRECTION('center_axis',(6.93889390390723E-18,1.,2.22049474265475E-16));
#107720=DIRECTION('ref_axis',(-0.82737837879608,-1.18971868843848E-16,0.561644921904196));
#107721=DIRECTION('center_axis',(0.,-1.,-2.67523620391604E-16));
#107722=DIRECTION('ref_axis',(-0.382987746401723,0.,-0.923753422784527));
#107723=DIRECTION('',(0.,-1.,-2.67523620391604E-16));
#107724=DIRECTION('center_axis',(0.,-1.,-2.22044604925031E-16));
#107725=DIRECTION('ref_axis',(-0.382987746401723,0.,-0.923753422784527));
#107726=DIRECTION('',(0.,1.,2.67523620391604E-16));
#107727=DIRECTION('center_axis',(0.,1.,2.67523620391604E-16));
#107728=DIRECTION('ref_axis',(0.846680472137446,1.42349762883284E-16,-0.532101661434271));
#107729=DIRECTION('',(0.,1.,2.67523620391604E-16));
#107730=DIRECTION('center_axis',(0.,-1.,-2.22044604925031E-16));
#107731=DIRECTION('ref_axis',(0.846680472137446,1.42349762883284E-16,-0.532101661434271));
#107732=DIRECTION('center_axis',(0.,-1.,-2.67523620391604E-16));
#107733=DIRECTION('ref_axis',(-0.827378378796083,0.,0.561644921904192));
#107734=DIRECTION('',(0.,-1.,-2.67523620391604E-16));
#107735=DIRECTION('center_axis',(0.,-1.,-2.22044604925031E-16));
#107736=DIRECTION('ref_axis',(-0.827378378796083,0.,0.561644921904192));
#107737=DIRECTION('center_axis',(2.46926126761481E-16,-2.67523620391604E-16,
1.));
#107738=DIRECTION('ref_axis',(1.,-6.93889390390717E-18,-2.46926126761481E-16));
#107739=DIRECTION('',(0.,1.,2.67523620391604E-16));
#107740=DIRECTION('',(1.,5.48286142624213E-32,-2.46926126761481E-16));
#107741=DIRECTION('center_axis',(-6.93889390390723E-18,-1.,-2.22049474265475E-16));
#107742=DIRECTION('ref_axis',(1.,-6.93889390390723E-18,1.54077774334651E-33));
#107743=DIRECTION('center_axis',(-0.185783118407687,-0.485875683947296,
0.854054712921521));
#107744=DIRECTION('ref_axis',(-0.97714808085684,5.55111512312577E-15,-0.212559704736796));
#107745=DIRECTION('center_axis',(-0.947567167180116,0.319117547005372,0.0167467870209411));
#107746=DIRECTION('ref_axis',(-0.0176706968910312,0.,-0.999843861046006));
#107747=DIRECTION('center_axis',(0.,-1.,-2.22044604925031E-16));
#107748=DIRECTION('ref_axis',(0.634326560888794,-1.71654958451944E-16,0.773065206920474));
#107749=DIRECTION('',(0.,1.,2.22044604925031E-16));
#107750=DIRECTION('center_axis',(0.,1.,2.22044604925031E-16));
#107751=DIRECTION('ref_axis',(0.634326560888794,-1.71654958451944E-16,0.773065206920474));
#107752=DIRECTION('center_axis',(0.,-1.,-2.22044604925031E-16));
#107753=DIRECTION('ref_axis',(1.,0.,0.));
#107754=DIRECTION('',(0.,1.,2.22044604925031E-16));
#107755=DIRECTION('center_axis',(4.16333634234434E-17,-1.,-2.28983498828938E-16));
#107756=DIRECTION('ref_axis',(1.,0.,0.));
#107757=DIRECTION('',(0.,-1.,-2.22044604925031E-16));
#107758=DIRECTION('center_axis',(-6.93889390390725E-18,-1.,-2.22049474265475E-16));
#107759=DIRECTION('ref_axis',(1.,0.,0.));
#107760=DIRECTION('center_axis',(0.,1.,2.22044604925031E-16));
#107761=DIRECTION('ref_axis',(1.,0.,1.49586791797067E-33));
#107762=DIRECTION('center_axis',(0.,1.,2.22044604925031E-16));
#107763=DIRECTION('ref_axis',(1.,0.,0.));
#107764=DIRECTION('',(0.,1.,2.22044604925031E-16));
#107765=DIRECTION('center_axis',(0.,1.,2.22044604925031E-16));
#107766=DIRECTION('ref_axis',(1.,0.,1.49586791797067E-33));
#107767=DIRECTION('',(0.,-1.,-2.22044604925031E-16));
#107768=DIRECTION('center_axis',(0.,-1.,-2.22044604925031E-16));
#107769=DIRECTION('ref_axis',(1.,0.,0.));
#107770=DIRECTION('',(0.,1.,2.22044604925031E-16));
#107771=DIRECTION('center_axis',(0.,-1.,-2.22044604925031E-16));
#107772=DIRECTION('ref_axis',(1.,0.,0.));
#107773=DIRECTION('center_axis',(0.,-1.,-2.22044604925031E-16));
#107774=DIRECTION('ref_axis',(1.,0.,0.));
#107775=DIRECTION('center_axis',(3.42121385298657E-49,-1.,-2.22044604925031E-16));
#107776=DIRECTION('ref_axis',(1.,0.,1.54077774334651E-33));
#107777=DIRECTION('center_axis',(0.,-1.,-2.22044604925031E-16));
#107778=DIRECTION('ref_axis',(-0.438909080076843,0.,0.898531479374039));
#107779=DIRECTION('center_axis',(-4.16333634234434E-17,1.,2.28983498828938E-16));
#107780=DIRECTION('ref_axis',(-0.438909080076843,0.,0.898531479374039));
#107781=DIRECTION('center_axis',(0.,1.,2.22044604925031E-16));
#107782=DIRECTION('ref_axis',(-0.438909080076843,0.,0.898531479374039));
#107783=DIRECTION('',(1.02786322857718E-29,-1.,-2.22044604925031E-16));
#107784=DIRECTION('center_axis',(4.16333634234434E-17,-1.,-2.28983498828938E-16));
#107785=DIRECTION('ref_axis',(1.,4.16333634234434E-17,6.93889390390723E-17));
#107786=DIRECTION('',(-1.88249434430459E-12,2.2898349882886E-16,-1.));
#107787=DIRECTION('center_axis',(4.16333634234434E-17,-1.,-2.28983498828938E-16));
#107788=DIRECTION('ref_axis',(0.923879532510927,0.,-0.382683432365958));
#107789=DIRECTION('',(0.707106781186548,-1.57009245868377E-16,0.707106781186548));
#107790=DIRECTION('',(-0.707106781186548,-1.57009245868377E-16,0.707106781186547));
#107791=DIRECTION('',(-0.707106781186547,1.57009245868378E-16,-0.707106781186548));
#107792=DIRECTION('center_axis',(9.62964972189322E-33,1.,2.22044604925031E-16));
#107793=DIRECTION('ref_axis',(0.923879532510927,-3.75530232012134E-16,-0.382683432365958));
#107794=DIRECTION('center_axis',(4.16333634234434E-17,-1.,-2.28983498828938E-16));
#107795=DIRECTION('ref_axis',(0.226765259529559,0.,-0.973949442769229));
#107796=DIRECTION('center_axis',(1.,4.28276345240491E-28,-1.88249434430459E-12));
#107797=DIRECTION('ref_axis',(-1.88249434430459E-12,2.22049474265623E-16,
-1.));
#107798=DIRECTION('',(-1.8825923899717E-12,2.22054343606079E-16,-1.));
#107799=DIRECTION('',(8.56552690482593E-29,-1.,-1.82003774528629E-16));
#107800=DIRECTION('',(1.88250052083182E-12,-2.22044604925031E-16,1.));
#107801=DIRECTION('',(0.,1.,2.27504718160893E-16));
#107802=DIRECTION('center_axis',(0.,-1.,-2.22044604925031E-16));
#107803=DIRECTION('ref_axis',(0.905538513813742,0.,-0.424264068711928));
#107804=DIRECTION('center_axis',(0.,1.,2.22044604925031E-16));
#107805=DIRECTION('ref_axis',(0.905538513813742,0.,-0.424264068711928));
#107806=DIRECTION('',(0.,1.,2.22044604925031E-16));
#107807=DIRECTION('center_axis',(0.,1.,2.22044604925031E-16));
#107808=DIRECTION('ref_axis',(0.905538513813742,0.,-0.424264068711928));
#107809=DIRECTION('',(0.,-1.,-2.22044604925031E-16));
#107810=DIRECTION('center_axis',(0.,-1.,-2.22044604925031E-16));
#107811=DIRECTION('ref_axis',(-1.,0.,0.));
#107812=DIRECTION('center_axis',(0.,1.,2.22044604925031E-16));
#107813=DIRECTION('ref_axis',(-1.,0.,0.));
#107814=DIRECTION('',(0.,-2.22044604925031E-16,1.));
#107815=DIRECTION('center_axis',(0.,-1.,-2.22044604925031E-16));
#107816=DIRECTION('ref_axis',(1.,0.,-1.837501759903E-19));
#107817=DIRECTION('',(-1.,-4.08007352326711E-35,1.837501759903E-19));
#107818=DIRECTION('center_axis',(0.,-1.,-2.22044604925031E-16));
#107819=DIRECTION('ref_axis',(1.,0.,6.93889390390723E-17));
#107820=DIRECTION('',(0.000408627366273739,2.22044586386934E-16,-0.999999916511834));
#107821=DIRECTION('center_axis',(0.,-1.,-2.22044604925031E-16));
#107822=DIRECTION('ref_axis',(0.707251238022098,0.,-0.706962294833472));
#107823=DIRECTION('',(-1.,2.89708077091569E-28,-1.30472918803582E-12));
#107824=DIRECTION('center_axis',(0.,-1.,-2.22044604925031E-16));
#107825=DIRECTION('ref_axis',(-0.827170191871368,0.,-0.561951486944811));
#107826=DIRECTION('center_axis',(0.,-1.,-2.22044604925031E-16));
#107827=DIRECTION('ref_axis',(1.,0.,1.85631801868649E-33));
#107828=DIRECTION('center_axis',(0.,1.,2.22044604925031E-16));
#107829=DIRECTION('ref_axis',(-0.442887523223796,0.,-0.896577181157702));
#107830=DIRECTION('center_axis',(0.,-1.,-2.22044604925031E-16));
#107831=DIRECTION('ref_axis',(0.442887523223796,0.,0.896577181157703));
#107832=DIRECTION('center_axis',(0.,-1.,-2.22044604925031E-16));
#107833=DIRECTION('ref_axis',(0.468176250029908,0.,-0.883635105067659));
#107834=DIRECTION('center_axis',(0.,-1.,-2.22044604925031E-16));
#107835=DIRECTION('ref_axis',(1.,0.,1.15584692836443E-33));
#107836=DIRECTION('center_axis',(0.,-1.,-2.22044604925031E-16));
#107837=DIRECTION('ref_axis',(-0.591607978303977,0.,-0.806225774834246));
#107838=DIRECTION('',(-7.42407262755995E-12,-1.64826352645555E-16,1.));
#107839=DIRECTION('center_axis',(0.,-1.,-2.22044604925031E-16));
#107840=DIRECTION('ref_axis',(-0.923879532512709,3.75530232012858E-16,0.382683432361657));
#107841=DIRECTION('',(0.707106781186547,-2.82505968889577E-16,0.707106781186548));
#107842=DIRECTION('',(-0.707106781186548,-1.57009245868377E-16,0.707106781186547));
#107843=DIRECTION('',(-0.707106781186548,1.66829210022541E-16,-0.707106781186548));
#107844=DIRECTION('center_axis',(0.,1.,2.22044604925031E-16));
#107845=DIRECTION('ref_axis',(-0.923879532511288,0.,0.382683432365088));
#107846=DIRECTION('',(-4.61226199516842E-16,2.22044604925031E-16,-1.));
#107847=DIRECTION('center_axis',(0.,-1.,-2.22044604925031E-16));
#107848=DIRECTION('ref_axis',(-0.939690906904483,-7.59447731678524E-17,
0.342024852139477));
#107849=DIRECTION('',(1.,-2.8970973742862E-28,1.30473666552914E-12));
#107850=DIRECTION('center_axis',(0.,1.,2.22044604925031E-16));
#107851=DIRECTION('ref_axis',(-1.,0.,0.));
#107852=DIRECTION('center_axis',(0.,1.,2.22044604925031E-16));
#107853=DIRECTION('ref_axis',(-1.,0.,0.));
#107854=DIRECTION('center_axis',(0.,1.,2.22044604925031E-16));
#107855=DIRECTION('ref_axis',(-1.,0.,0.));
#107856=DIRECTION('',(0.,1.,2.22044604925031E-16));
#107857=DIRECTION('center_axis',(0.,-1.,-2.22044604925031E-16));
#107858=DIRECTION('ref_axis',(-1.,0.,0.));
#107859=DIRECTION('',(-1.,0.,0.));
#107860=DIRECTION('center_axis',(0.,1.,2.22044604925031E-16));
#107861=DIRECTION('ref_axis',(0.707106781186548,1.57009245868377E-16,-0.707106781186548));
#107862=DIRECTION('',(-1.190587693968E-16,2.22044604925031E-16,-1.));
#107863=DIRECTION('center_axis',(0.,1.,2.22044604925031E-16));
#107864=DIRECTION('ref_axis',(0.923879532511288,0.,0.382683432365088));
#107865=DIRECTION('',(-0.707106781186548,-1.52106150078638E-16,0.707106781186547));
#107866=DIRECTION('center_axis',(0.,-1.,-2.22044604925031E-16));
#107867=DIRECTION('ref_axis',(-0.923879532511647,0.,-0.382683432364221));
#107868=DIRECTION('',(1.88205007134457E-12,-2.22049474265488E-16,1.));
#107869=DIRECTION('center_axis',(0.,1.,2.22044604925031E-16));
#107870=DIRECTION('ref_axis',(0.89959196856447,-9.69738446503996E-17,0.436731370632224));
#107871=DIRECTION('center_axis',(0.,-1.,-2.22044604925031E-16));
#107872=DIRECTION('ref_axis',(-1.,0.,0.));
#107873=DIRECTION('center_axis',(0.,1.,2.22044604925031E-16));
#107874=DIRECTION('ref_axis',(0.706817778969831,-1.57073391034583E-16,0.707395665333168));
#107875=DIRECTION('center_axis',(0.,-1.,-2.22044604925031E-16));
#107876=DIRECTION('ref_axis',(-0.753900508899602,0.,0.656988601636985));
#107877=DIRECTION('center_axis',(-4.16333634234434E-17,1.,2.28983498828938E-16));
#107878=DIRECTION('ref_axis',(-0.984274724761795,4.72565661779708E-17,-0.176644462678832));
#107879=DIRECTION('center_axis',(0.,-1.,-2.22044604925031E-16));
#107880=DIRECTION('ref_axis',(0.0662762646370231,0.,0.997801311256787));
#107881=DIRECTION('center_axis',(0.,-1.,-2.22044604925031E-16));
#107882=DIRECTION('ref_axis',(-1.,0.,-1.85631801868649E-33));
#107883=DIRECTION('center_axis',(0.,1.,2.22044604925031E-16));
#107884=DIRECTION('ref_axis',(1.,1.85370757147271E-31,-6.93889390390722E-16));
#107885=DIRECTION('',(-1.,6.93889390390712E-18,1.83750175990302E-19));
#107886=DIRECTION('center_axis',(-6.93889390390723E-18,-1.,-2.22049474265475E-16));
#107887=DIRECTION('ref_axis',(1.,-6.93889390390723E-18,-1.83750175990302E-19));
#107888=DIRECTION('',(0.,-2.22044604925031E-16,1.));
#107889=DIRECTION('center_axis',(0.,1.,2.22044604925031E-16));
#107890=DIRECTION('ref_axis',(-0.923879532511647,0.,-0.382683432364221));
#107891=DIRECTION('',(0.707106781186548,1.52106150078638E-16,-0.707106781186547));
#107892=DIRECTION('center_axis',(0.,-1.,-2.22044604925031E-16));
#107893=DIRECTION('ref_axis',(-0.934114852736578,0.,0.356972606647795));
#107894=DIRECTION('center_axis',(0.,-1.,-2.22044604925031E-16));
#107895=DIRECTION('ref_axis',(-0.243728531198527,1.95771377718342E-16,-0.969843494116349));
#107896=DIRECTION('center_axis',(0.,1.,2.22044604925031E-16));
#107897=DIRECTION('ref_axis',(0.470867335571779,-1.78080586840007E-16,0.882204030988032));
#107898=DIRECTION('center_axis',(0.,-1.,-2.22044604925031E-16));
#107899=DIRECTION('ref_axis',(0.656130266938609,0.,0.754647648116039));
#107900=DIRECTION('',(-1.88215207428297E-12,2.22049474265488E-16,-1.));
#107901=DIRECTION('center_axis',(0.,-1.,-2.22044604925031E-16));
#107902=DIRECTION('ref_axis',(1.,0.,0.));
#107903=DIRECTION('center_axis',(0.,2.22044604925031E-16,-1.));
#107904=DIRECTION('ref_axis',(1.,0.,0.));
#107905=DIRECTION('',(0.,-1.,-2.22044604925031E-16));
#107906=DIRECTION('',(1.,0.,0.));
#107907=DIRECTION('',(0.,1.,2.22044604925031E-16));
#107908=DIRECTION('center_axis',(-6.50074362628841E-34,-1.,-2.27504718160893E-16));
#107909=DIRECTION('ref_axis',(0.923879532511288,0.,0.382683432365088));
#107910=DIRECTION('',(6.50074362628841E-34,1.,2.27504718160893E-16));
#107911=DIRECTION('center_axis',(0.,-1.,-2.22044604925031E-16));
#107912=DIRECTION('ref_axis',(0.923879532511288,0.,0.382683432365088));
#107913=DIRECTION('',(-6.50074362628841E-34,-1.,-2.27504718160893E-16));
#107914=DIRECTION('center_axis',(-0.707106781186547,1.60870128963502E-16,
-0.707106781186548));
#107915=DIRECTION('ref_axis',(-0.707106781186548,-1.52106150078733E-16,
0.707106781186547));
#107916=DIRECTION('',(0.707106781186548,1.57009245868377E-16,-0.707106781186547));
#107917=DIRECTION('',(0.,1.,2.27504718160893E-16));
#107918=DIRECTION('center_axis',(0.,-1.,-2.22044604925031E-16));
#107919=DIRECTION('ref_axis',(1.,0.,0.));
#107920=DIRECTION('',(1.190587693968E-16,-2.22044604925031E-16,1.));
#107921=DIRECTION('center_axis',(0.,-1.,-2.22044604925031E-16));
#107922=DIRECTION('ref_axis',(0.707106781186548,1.57009245868377E-16,-0.707106781186548));
#107923=DIRECTION('center_axis',(0.,-1.,-2.22044604925031E-16));
#107924=DIRECTION('ref_axis',(-0.939690906904483,-7.59447731678524E-17,
0.342024852139477));
#107925=DIRECTION('',(4.61226199516842E-16,-2.22044604925031E-16,1.));
#107926=DIRECTION('center_axis',(0.,-1.,-2.22044604925031E-16));
#107927=DIRECTION('ref_axis',(-0.923879532511288,0.,0.382683432365088));
#107928=DIRECTION('',(0.707106781186548,-1.57009245868377E-16,0.707106781186548));
#107929=DIRECTION('center_axis',(0.,1.,2.22044604925031E-16));
#107930=DIRECTION('ref_axis',(0.923879532510927,0.,-0.382683432365958));
#107931=DIRECTION('center_axis',(0.,-1.,-2.22044604925031E-16));
#107932=DIRECTION('ref_axis',(-0.923879532510705,0.,0.382683432366494));
#107933=DIRECTION('',(0.707106781187368,-1.57009245868195E-16,0.707106781185727));
#107934=DIRECTION('center_axis',(0.,-1.,-2.22044604925031E-16));
#107935=DIRECTION('ref_axis',(-0.382683432364552,0.,0.92387953251151));
#107936=DIRECTION('',(-1.,1.35429601616597E-31,-6.09920703375441E-16));
#107937=DIRECTION('center_axis',(0.,1.,2.22044604925031E-16));
#107938=DIRECTION('ref_axis',(0.360742674985292,2.07093317185659E-16,-0.932665386108253));
#107939=DIRECTION('center_axis',(0.,1.,2.22044604925031E-16));
#107940=DIRECTION('ref_axis',(0.707106781186547,-1.57009245868377E-16,0.707106781186547));
#107941=DIRECTION('',(0.707106781186548,1.57009245868377E-16,-0.707106781186548));
#107942=DIRECTION('center_axis',(0.,1.,2.22044604925031E-16));
#107943=DIRECTION('ref_axis',(-0.707106781186547,1.57009245868377E-16,-0.707106781186547));
#107944=DIRECTION('center_axis',(0.,1.,2.22044604925031E-16));
#107945=DIRECTION('ref_axis',(-0.993670662656293,-2.49428489271903E-17,
0.112332605134053));
#107946=DIRECTION('',(1.190587693968E-16,-2.22044604925031E-16,1.));
#107947=DIRECTION('center_axis',(0.,-1.,-2.22044604925031E-16));
#107948=DIRECTION('ref_axis',(0.923879532511287,0.,-0.38268343236509));
#107949=DIRECTION('',(-0.707106781186547,1.57009245868378E-16,-0.707106781186548));
#107950=DIRECTION('center_axis',(0.,1.,2.22044604925031E-16));
#107951=DIRECTION('ref_axis',(-0.923879532510926,0.,0.38268343236596));
#107952=DIRECTION('',(-1.88205025509474E-12,2.22044604925031E-16,-1.));
#107953=DIRECTION('center_axis',(0.,1.,2.22044604925031E-16));
#107954=DIRECTION('ref_axis',(-0.923879532511647,0.,-0.382683432364221));
#107955=DIRECTION('',(-0.707106781186548,-1.57009245868377E-16,0.707106781186548));
#107956=DIRECTION('center_axis',(0.,-1.,-2.22044604925031E-16));
#107957=DIRECTION('ref_axis',(0.707106781186548,-1.57009245868377E-16,0.707106781186548));
#107958=DIRECTION('',(0.707106781186548,1.57009245868377E-16,-0.707106781186548));
#107959=DIRECTION('center_axis',(0.,-1.,-2.22044604925031E-16));
#107960=DIRECTION('ref_axis',(-0.707106781186548,1.57009245868377E-16,-0.707106781186548));
#107961=DIRECTION('center_axis',(0.,1.,2.22044604925031E-16));
#107962=DIRECTION('ref_axis',(1.,0.,0.));
#107963=DIRECTION('center_axis',(0.,-1.,-2.22044604925031E-16));
#107964=DIRECTION('ref_axis',(1.,0.,0.));
#107965=DIRECTION('center_axis',(0.,1.,2.22044604925031E-16));
#107966=DIRECTION('ref_axis',(1.,0.,0.));
#107967=DIRECTION('center_axis',(0.,-1.,-2.27504718160893E-16));
#107968=DIRECTION('ref_axis',(-0.923879532511647,0.,-0.382683432364221));
#107969=DIRECTION('',(0.,-1.,-2.27504718160893E-16));
#107970=DIRECTION('center_axis',(-1.,-4.28175312849965E-28,1.88205025509474E-12));
#107971=DIRECTION('ref_axis',(1.88205025509474E-12,-2.22049474265623E-16,
1.));
#107972=DIRECTION('',(-2.6267572334885E-44,1.,2.27504718160893E-16));
#107973=DIRECTION('',(1.88205007134457E-12,-2.22049474265488E-16,1.));
#107974=DIRECTION('center_axis',(6.34155293819033E-44,1.,2.27504718160893E-16));
#107975=DIRECTION('ref_axis',(-0.923879532510926,0.,0.38268343236596));
#107976=DIRECTION('center_axis',(-6.93889390390721E-18,-1.,-2.22049474265475E-16));
#107977=DIRECTION('ref_axis',(-0.923879532510926,0.,0.38268343236596));
#107978=DIRECTION('',(-6.34155293819033E-44,-1.,-2.27504718160893E-16));
#107979=DIRECTION('center_axis',(6.50074362628842E-34,1.,2.27504718160893E-16));
#107980=DIRECTION('ref_axis',(0.923879532511287,0.,-0.38268343236509));
#107981=DIRECTION('',(-6.50074362628842E-34,-1.,-2.27504718160893E-16));
#107982=DIRECTION('center_axis',(0.,1.,2.22044604925031E-16));
#107983=DIRECTION('ref_axis',(0.923879532511287,0.,-0.38268343236509));
#107984=DIRECTION('',(6.50074362628842E-34,1.,2.27504718160893E-16));
#107985=DIRECTION('center_axis',(-0.707106781186548,-1.60870128963501E-16,
0.707106781186547));
#107986=DIRECTION('ref_axis',(0.707106781186547,-1.61919227945507E-16,0.707106781186548));
#107987=DIRECTION('',(0.707106781186547,-1.57009245868378E-16,0.707106781186548));
#107988=DIRECTION('',(0.707106781186547,-1.61919227945412E-16,0.707106781186548));
#107989=DIRECTION('center_axis',(0.,-1.,-2.22044604925031E-16));
#107990=DIRECTION('ref_axis',(-1.,0.,0.));
#107991=DIRECTION('',(-1.190587693968E-16,2.22044604925031E-16,-1.));
#107992=DIRECTION('center_axis',(0.,1.,2.22044604925031E-16));
#107993=DIRECTION('ref_axis',(0.69744724579616,-1.59125185820173E-16,0.716636127564994));
#107994=DIRECTION('',(-0.999631786816462,6.02510900342743E-18,-0.0271346786627024));
#107995=DIRECTION('center_axis',(0.,-1.,-2.22044604925031E-16));
#107996=DIRECTION('ref_axis',(-0.370112462344042,0.,-0.928986956430299));
#107997=DIRECTION('',(-0.707106781186548,-1.57009245868378E-16,0.707106781186548));
#107998=DIRECTION('',(-1.85435565520038E-14,-2.22044604925031E-16,1.));
#107999=DIRECTION('center_axis',(0.,-1.,-2.22044604925031E-16));
#108000=DIRECTION('ref_axis',(0.707106781186561,1.57009245868375E-16,-0.707106781186534));
#108001=DIRECTION('center_axis',(0.,-1.,-2.22044604925031E-16));
#108002=DIRECTION('ref_axis',(0.0271346786627019,0.,-0.999631786816462));
#108003=DIRECTION('',(0.999631786816462,-6.02510900342741E-18,0.0271346786627023));
#108004=DIRECTION('center_axis',(0.,-1.,-2.22044604925031E-16));
#108005=DIRECTION('ref_axis',(0.697447245796159,0.,0.716636127564995));
#108006=DIRECTION('',(-8.32407533012986E-17,2.22044604925031E-16,-1.));
#108007=DIRECTION('center_axis',(0.,-1.,-2.22044604925031E-16));
#108008=DIRECTION('ref_axis',(0.0595262816618969,-2.21650861813111E-16,
0.998226738667878));
#108009=DIRECTION('center_axis',(0.,1.,2.22044604925031E-16));
#108010=DIRECTION('ref_axis',(-0.157390971609958,2.19277123123827E-16,-0.98753636999134));
#108011=DIRECTION('center_axis',(0.,-1.,-2.22044604925031E-16));
#108012=DIRECTION('ref_axis',(0.89959196856447,-9.69738446503996E-17,0.436731370632224));
#108013=DIRECTION('center_axis',(4.004083039641E-17,1.,2.22044604925031E-16));
#108014=DIRECTION('ref_axis',(-0.382683432364552,0.,0.92387953251151));
#108015=DIRECTION('',(-4.004083039641E-17,-1.,-2.22044604925031E-16));
#108016=DIRECTION('center_axis',(0.,1.,2.22044604925031E-16));
#108017=DIRECTION('ref_axis',(-0.382683432364552,0.,0.92387953251151));
#108018=DIRECTION('',(4.004083039641E-17,1.,2.22044604925031E-16));
#108019=DIRECTION('center_axis',(0.707106781185727,1.28696103170951E-16,
-0.707106781187368));
#108020=DIRECTION('ref_axis',(-0.707106781187368,1.6191922794533E-16,-0.707106781185727));
#108021=DIRECTION('',(-8.56552690482593E-29,1.,1.82003774528629E-16));
#108022=DIRECTION('',(-0.707106781187368,1.57009245868195E-16,-0.707106781185727));
#108023=DIRECTION('center_axis',(-8.56552690482593E-29,1.,1.82003774528629E-16));
#108024=DIRECTION('ref_axis',(-0.923879532510705,0.,0.382683432366494));
#108025=DIRECTION('center_axis',(0.,1.,2.22044604925031E-16));
#108026=DIRECTION('ref_axis',(-0.923879532510705,0.,0.382683432366494));
#108027=DIRECTION('center_axis',(0.,-1.,-2.22044604925031E-16));
#108028=DIRECTION('ref_axis',(1.,0.,0.));
#108029=DIRECTION('center_axis',(0.,-1.,-2.22044604925031E-16));
#108030=DIRECTION('ref_axis',(0.371940837143492,0.,0.928256437448725));
#108031=DIRECTION('center_axis',(0.,-1.,-2.22044604925031E-16));
#108032=DIRECTION('ref_axis',(1.,0.,-1.83750175990302E-19));
#108033=DIRECTION('center_axis',(0.,-1.,-2.22044604925031E-16));
#108034=DIRECTION('ref_axis',(0.906884704407261,0.,0.421378847252866));
#108035=DIRECTION('center_axis',(0.,-1.,-2.22044604925031E-16));
#108036=DIRECTION('ref_axis',(0.414254853160806,0.,0.910160928975046));
#108037=DIRECTION('center_axis',(0.,-1.,-2.22044604925031E-16));
#108038=DIRECTION('ref_axis',(0.641559662047602,0.,-0.767073138646744));
#108039=DIRECTION('center_axis',(0.,1.,2.22044604925031E-16));
#108040=DIRECTION('ref_axis',(-0.901335144845703,0.,-0.433122334526835));
#108041=DIRECTION('center_axis',(0.,-1.,-2.22044604925031E-16));
#108042=DIRECTION('ref_axis',(0.141735171603208,0.,-0.989904612137255));
#108043=DIRECTION('center_axis',(0.,1.,2.22044604925031E-16));
#108044=DIRECTION('ref_axis',(2.48741143748787E-16,0.,1.));
#108045=DIRECTION('',(1.,7.23661930473396E-32,-3.2590836004222E-16));
#108046=DIRECTION('center_axis',(0.,-1.,-2.22044604925031E-16));
#108047=DIRECTION('ref_axis',(0.51349131065734,0.,0.858094793061586));
#108048=DIRECTION('center_axis',(0.,1.,2.22044604925031E-16));
#108049=DIRECTION('ref_axis',(-0.891123735454889,-1.00755045690416E-16,
0.453760386227053));
#108050=DIRECTION('',(-1.,-2.58135112964991E-32,1.16253719856037E-16));
#108051=DIRECTION('center_axis',(0.,1.,2.22044604925031E-16));
#108052=DIRECTION('ref_axis',(1.,0.,0.));
#108053=DIRECTION('center_axis',(0.,1.,2.27504718160893E-16));
#108054=DIRECTION('ref_axis',(0.923879532510927,0.,-0.382683432365958));
#108055=DIRECTION('',(0.,-1.,-2.27504718160893E-16));
#108056=DIRECTION('center_axis',(2.09862273058998E-32,1.,2.27504718160893E-16));
#108057=DIRECTION('ref_axis',(-0.923879532511288,0.,0.382683432365088));
#108058=DIRECTION('',(-2.09862273058998E-32,-1.,-2.27504718160893E-16));
#108059=DIRECTION('',(2.09862273058998E-32,1.,2.27504718160893E-16));
#108060=DIRECTION('center_axis',(0.707106781186548,1.60870128963502E-16,
-0.707106781186548));
#108061=DIRECTION('ref_axis',(-0.707106781186548,1.61919227945507E-16,-0.707106781186548));
#108062=DIRECTION('',(-5.33214183189602E-18,1.,2.22172576328997E-16));
#108063=DIRECTION('center_axis',(-0.707106781186547,1.53329341668337E-16,
-0.707106781186548));
#108064=DIRECTION('ref_axis',(-0.707106781186548,-1.57009245868377E-16,
0.707106781186547));
#108065=DIRECTION('',(-2.36032059159488E-16,-1.,1.91916246623874E-17));
#108066=DIRECTION('center_axis',(0.,1.,2.01858731750028E-16));
#108067=DIRECTION('ref_axis',(-0.243728531198527,1.95771377718342E-16,-0.969843494116349));
#108068=DIRECTION('',(0.,1.,2.01858731750028E-16));
#108069=DIRECTION('',(0.,-1.,-2.01858731750028E-16));
#108070=DIRECTION('center_axis',(0.,1.,2.01858731750028E-16));
#108071=DIRECTION('ref_axis',(0.470867335571779,-1.78080586840007E-16,0.882204030988032));
#108072=DIRECTION('',(0.,1.,2.01858731750028E-16));
#108073=DIRECTION('center_axis',(-2.57578868254608E-29,-1.,-2.01858731750032E-16));
#108074=DIRECTION('ref_axis',(0.656130266938609,0.,0.754647648116039));
#108075=DIRECTION('',(-2.57578868254608E-29,-1.,-2.01858731750032E-16));
#108076=DIRECTION('center_axis',(-1.,-3.54170943849992E-28,1.88215207428297E-12));
#108077=DIRECTION('ref_axis',(-1.88215207428297E-12,2.22049474265488E-16,
-1.));
#108078=DIRECTION('',(-4.48415508583941E-44,1.,1.88173394004264E-16));
#108079=DIRECTION('center_axis',(0.,-1.,-1.88173394004264E-16));
#108080=DIRECTION('ref_axis',(-0.923879532511647,0.,-0.382683432364221));
#108081=DIRECTION('',(0.,-1.,-1.88173394004264E-16));
#108082=DIRECTION('center_axis',(-0.707106781186547,1.33058682939303E-16,
-0.707106781186548));
#108083=DIRECTION('ref_axis',(0.707106781186548,1.52106150078638E-16,-0.707106781186547));
#108084=DIRECTION('center_axis',(0.,-1.,-2.01858731750028E-16));
#108085=DIRECTION('ref_axis',(-0.956462973763756,0.,-0.291853695914568));
#108086=DIRECTION('',(0.,-1.,-2.01858731750028E-16));
#108087=DIRECTION('center_axis',(0.,-1.,-2.22044604925031E-16));
#108088=DIRECTION('ref_axis',(-0.956462973763756,0.,-0.291853695914568));
#108089=DIRECTION('',(0.,1.,2.01858731750028E-16));
#108090=DIRECTION('center_axis',(0.,1.,2.01858731750028E-16));
#108091=DIRECTION('ref_axis',(-0.984274724761795,3.56572272070144E-17,-0.176644462678833));
#108092=DIRECTION('',(0.,1.,2.01858731750028E-16));
#108093=DIRECTION('center_axis',(0.,-1.,-2.22044604925031E-16));
#108094=DIRECTION('ref_axis',(-0.984274724761795,3.56572272070144E-17,-0.176644462678833));
#108095=DIRECTION('center_axis',(-3.14252774266953E-33,-1.,-2.01858731750028E-16));
#108096=DIRECTION('ref_axis',(-0.83018371253477,0.,0.557489913309636));
#108097=DIRECTION('center_axis',(0.,-1.,-2.22044604925031E-16));
#108098=DIRECTION('ref_axis',(-0.83018371253477,0.,0.557489913309636));
#108099=DIRECTION('center_axis',(0.,1.,3.96508223080413E-16));
#108100=DIRECTION('ref_axis',(-0.0664533356011988,-3.95631755140045E-16,
0.997789534013799));
#108101=DIRECTION('',(0.,1.,3.96508223080413E-16));
#108102=DIRECTION('center_axis',(0.,1.,2.22044604925031E-16));
#108103=DIRECTION('ref_axis',(-0.0664533356011988,-3.95631755140045E-16,
0.997789534013799));
#108104=DIRECTION('',(0.,-1.,-3.96508223080413E-16));
#108105=DIRECTION('center_axis',(0.,1.,3.96508223080413E-16));
#108106=DIRECTION('ref_axis',(0.0664533356011965,3.95631755140045E-16,-0.997789534013799));
#108107=DIRECTION('',(0.,1.,3.96508223080413E-16));
#108108=DIRECTION('center_axis',(0.,-1.,-2.22044604925031E-16));
#108109=DIRECTION('ref_axis',(0.0664533356011965,3.95631755140045E-16,-0.997789534013799));
#108110=DIRECTION('center_axis',(0.,-1.,-2.22044604925031E-16));
#108111=DIRECTION('ref_axis',(0.707106781186561,1.57009245868375E-16,-0.707106781186534));
#108112=DIRECTION('',(0.,1.,0.));
#108113=DIRECTION('',(0.,-1.,-2.22044604925031E-16));
#108114=DIRECTION('center_axis',(0.,1.,2.22044604925031E-16));
#108115=DIRECTION('ref_axis',(0.707106781186561,1.57009245868375E-16,-0.707106781186534));
#108116=DIRECTION('center_axis',(0.,-1.,0.));
#108117=DIRECTION('ref_axis',(0.0271346786627019,0.,-0.999631786816462));
#108118=DIRECTION('',(0.,-1.,0.));
#108119=DIRECTION('center_axis',(-0.0271346786627023,-2.01784404703786E-16,
0.999631786816462));
#108120=DIRECTION('ref_axis',(0.999631786816462,6.13206694458201E-17,0.0271346786627023));
#108121=DIRECTION('',(2.73791920107971E-48,1.,2.01858731750028E-16));
#108122=DIRECTION('center_axis',(-2.73791920107971E-48,-1.,-2.01858731750028E-16));
#108123=DIRECTION('ref_axis',(0.697447245796159,0.,0.716636127564995));
#108124=DIRECTION('',(-1.00813794530025E-51,-1.,-2.01858731750028E-16));
#108125=DIRECTION('center_axis',(1.,1.68028728913171E-32,-8.32407533012986E-17));
#108126=DIRECTION('ref_axis',(-8.32407533012986E-17,1.80520972702821E-16,
-1.));
#108127=DIRECTION('center_axis',(-6.93889390390721E-18,-1.,-2.22049474265475E-16));
#108128=DIRECTION('ref_axis',(1.,-6.93889390390721E-18,0.));
#108129=DIRECTION('center_axis',(0.,-1.,-2.22044604925031E-16));
#108130=DIRECTION('ref_axis',(0.229951641166733,-1.9644933285631E-16,0.973202056473745));
#108131=DIRECTION('center_axis',(0.,-1.,-2.22044604925031E-16));
#108132=DIRECTION('ref_axis',(0.89959196856447,-9.69738446503996E-17,0.436731370632224));
#108133=DIRECTION('center_axis',(0.,1.,1.6657509746814E-16));
#108134=DIRECTION('ref_axis',(1.,0.,1.15584692836443E-33));
#108135=DIRECTION('',(0.,1.,1.6657509746814E-16));
#108136=DIRECTION('',(0.,-1.,-1.6657509746814E-16));
#108137=DIRECTION('center_axis',(0.,-1.,-1.6657509746814E-16));
#108138=DIRECTION('ref_axis',(-0.591607978303977,0.,-0.806225774834246));
#108139=DIRECTION('',(-5.10447367644408E-16,-1.,-1.6657509747193E-16));
#108140=DIRECTION('center_axis',(1.,-5.10447367645645E-16,7.42407262755995E-12));
#108141=DIRECTION('ref_axis',(-7.42407262755995E-12,-1.64826352645555E-16,
1.));
#108142=DIRECTION('',(5.1044736764375E-16,1.,2.55223683821875E-16));
#108143=DIRECTION('center_axis',(-5.1044736764375E-16,-1.,-2.55223683821875E-16));
#108144=DIRECTION('ref_axis',(-0.923879532512709,3.75530232012858E-16,0.382683432361657));
#108145=DIRECTION('',(-5.1044736764375E-16,-1.,-2.55223683821875E-16));
#108146=DIRECTION('center_axis',(0.707106781186548,-1.8047039754986E-16,
-0.707106781186547));
#108147=DIRECTION('ref_axis',(0.707106781186547,-2.82505968889577E-16,0.707106781186548));
#108148=DIRECTION('',(5.1044736764375E-16,1.,2.55223683821875E-16));
#108149=DIRECTION('center_axis',(-5.1044736764375E-16,-1.,-2.55223683821875E-16));
#108150=DIRECTION('ref_axis',(0.923879532510927,-3.75530232012134E-16,-0.382683432365958));
#108151=DIRECTION('center_axis',(0.,1.,0.));
#108152=DIRECTION('ref_axis',(0.906884704407261,0.,0.421378847252866));
#108153=DIRECTION('',(0.,-1.,0.));
#108154=DIRECTION('',(0.,1.,0.));
#108155=DIRECTION('center_axis',(0.,1.,0.));
#108156=DIRECTION('ref_axis',(0.414254853160806,0.,0.910160928975046));
#108157=DIRECTION('',(0.,1.,0.));
#108158=DIRECTION('center_axis',(0.,1.,2.22044604925031E-16));
#108159=DIRECTION('ref_axis',(0.641559662047602,0.,-0.767073138646744));
#108160=DIRECTION('center_axis',(0.,1.,0.));
#108161=DIRECTION('ref_axis',(0.371940837143492,0.,0.928256437448725));
#108162=DIRECTION('',(0.,-1.,0.));
#108163=DIRECTION('center_axis',(0.,1.,0.));
#108164=DIRECTION('ref_axis',(1.,0.,-1.83750175990302E-19));
#108165=DIRECTION('center_axis',(1.,8.3944909223599E-32,-4.61226199516842E-16));
#108166=DIRECTION('ref_axis',(-4.61226199516842E-16,2.22049474265475E-16,
-1.));
#108167=DIRECTION('',(0.,-1.,-2.22044604925031E-16));
#108168=DIRECTION('center_axis',(0.,-1.,-2.22044604925031E-16));
#108169=DIRECTION('ref_axis',(0.89959196856447,-9.69738446503996E-17,0.436731370632224));
#108170=DIRECTION('center_axis',(0.,1.,2.22044604925031E-16));
#108171=DIRECTION('ref_axis',(0.89959196856447,-9.69738446503996E-17,0.436731370632224));
#108172=DIRECTION('center_axis',(1.,2.64363574135728E-32,-1.190587693968E-16));
#108173=DIRECTION('ref_axis',(1.190587693968E-16,-2.22044604925031E-16,
1.));
#108174=DIRECTION('',(0.,-1.,-2.22044604925031E-16));
#108175=DIRECTION('center_axis',(1.,2.64363574135728E-32,-1.190587693968E-16));
#108176=DIRECTION('ref_axis',(1.190587693968E-16,-2.22044604925031E-16,
1.));
#108177=DIRECTION('',(0.,1.,2.22044604925031E-16));
#108178=DIRECTION('',(1.190587693968E-16,-2.22044604925031E-16,1.));
#108179=DIRECTION('',(0.,1.,2.22044604925031E-16));
#108180=DIRECTION('center_axis',(0.,-1.,-2.22044604925031E-16));
#108181=DIRECTION('ref_axis',(-0.939690906904483,-7.59447731678524E-17,
0.342024852139477));
#108182=DIRECTION('center_axis',(1.35739377892777E-16,-1.,-3.84762012452445E-17));
#108183=DIRECTION('ref_axis',(1.,1.35739377892777E-16,6.93889390390723E-17));
#108184=DIRECTION('center_axis',(4.16333634234434E-17,-1.,-2.28983498828938E-16));
#108185=DIRECTION('ref_axis',(1.,4.16333634234434E-17,6.93889390390723E-17));
#108186=DIRECTION('center_axis',(1.35739377892777E-16,-1.,-3.84762012452445E-17));
#108187=DIRECTION('ref_axis',(-0.997493114923262,0.,-0.0707635900777229));
#108188=DIRECTION('center_axis',(4.16333634234434E-17,-1.,-2.28983498828939E-16));
#108189=DIRECTION('ref_axis',(0.753363330133441,0.,0.657604510941228));
#108190=DIRECTION('',(0.000408627363453739,2.29000492243054E-16,-0.999999916511835));
#108191=DIRECTION('center_axis',(0.,-1.,-2.67523620391604E-16));
#108192=DIRECTION('ref_axis',(0.753363330133441,0.,0.657604510941228));
#108193=DIRECTION('',(0.,-1.,-2.67523620391604E-16));
#108194=DIRECTION('center_axis',(0.,1.,1.6657509746814E-16));
#108195=DIRECTION('ref_axis',(-0.997493114923262,0.,-0.0707635900777229));
#108196=DIRECTION('center_axis',(0.,1.,2.22044604925031E-16));
#108197=DIRECTION('ref_axis',(0.226765259529559,0.,-0.973949442769229));
#108198=DIRECTION('center_axis',(0.,-1.,-2.22044604925031E-16));
#108199=DIRECTION('ref_axis',(-1.,0.,0.));
#108200=DIRECTION('center_axis',(0.,-1.,-2.22044604925031E-16));
#108201=DIRECTION('ref_axis',(-1.,0.,0.));
#108202=DIRECTION('center_axis',(0.,1.,0.));
#108203=DIRECTION('ref_axis',(0.442887523223796,0.,0.896577181157703));
#108204=DIRECTION('',(0.,1.,0.));
#108205=DIRECTION('center_axis',(4.16333634234434E-17,-1.,-2.28983498828938E-16));
#108206=DIRECTION('ref_axis',(0.442887523223796,-1.86862482701593E-16,0.896577181157703));
#108207=DIRECTION('',(0.,1.,0.));
#108208=DIRECTION('center_axis',(0.,1.,0.));
#108209=DIRECTION('ref_axis',(-0.442887523223796,0.,-0.896577181157702));
#108210=DIRECTION('center_axis',(-1.35739377892777E-16,1.,3.84762012452444E-17));
#108211=DIRECTION('ref_axis',(-0.442887523223796,-2.56203928247531E-17,
-0.896577181157702));
#108212=DIRECTION('center_axis',(4.16333634234434E-17,-1.,-2.28983498828938E-16));
#108213=DIRECTION('ref_axis',(1.,4.16333634234434E-17,6.93889390390723E-17));
#108214=DIRECTION('center_axis',(4.16333634234434E-17,-1.,-2.28983498828938E-16));
#108215=DIRECTION('ref_axis',(0.468176250029908,0.,-0.883635105067659));
#108216=DIRECTION('center_axis',(0.,-1.,-1.6657509746814E-16));
#108217=DIRECTION('ref_axis',(0.468176250029908,0.,-0.883635105067659));
#108218=DIRECTION('center_axis',(0.,-1.,-2.22044604925031E-16));
#108219=DIRECTION('ref_axis',(0.0595262816618969,-2.21650861813111E-16,
0.998226738667878));
#108220=DIRECTION('center_axis',(0.,-1.,-2.22044604925031E-16));
#108221=DIRECTION('ref_axis',(0.0595262816618969,-2.21650861813111E-16,
0.998226738667878));
#108222=DIRECTION('',(0.,1.,2.22044604925031E-16));
#108223=DIRECTION('center_axis',(0.,-1.,-2.22044604925031E-16));
#108224=DIRECTION('ref_axis',(-0.157390971609958,2.19277123123827E-16,-0.98753636999134));
#108225=DIRECTION('center_axis',(0.,1.,2.22044604925031E-16));
#108226=DIRECTION('ref_axis',(-0.157390971609958,2.19277123123827E-16,-0.98753636999134));
#108227=DIRECTION('center_axis',(1.,-4.12194440118864E-49,1.54077774334651E-33));
#108228=DIRECTION('ref_axis',(1.54077774334651E-33,2.22049474265475E-16,
-1.));
#108229=DIRECTION('',(0.,1.,2.67523620391604E-16));
#108230=DIRECTION('',(1.54077774334651E-33,2.22044604925031E-16,-1.));
#108231=DIRECTION('',(0.,-1.,-2.67523620391604E-16));
#108232=DIRECTION('center_axis',(0.,-1.,-2.67523620391604E-16));
#108233=DIRECTION('ref_axis',(0.482689240114392,0.,-0.875791697538742));
#108234=DIRECTION('',(0.,-1.,-2.67523620391604E-16));
#108235=DIRECTION('center_axis',(0.,-1.,-2.22044604925031E-16));
#108236=DIRECTION('ref_axis',(0.482689240114392,0.,-0.875791697538742));
#108237=DIRECTION('center_axis',(0.,1.,2.67523620391604E-16));
#108238=DIRECTION('ref_axis',(1.,0.,1.85631801868649E-33));
#108239=DIRECTION('center_axis',(0.,-1.,-2.22044604925031E-16));
#108240=DIRECTION('ref_axis',(1.,0.,1.85631801868649E-33));
#108241=DIRECTION('center_axis',(0.,1.,2.67523620391604E-16));
#108242=DIRECTION('ref_axis',(0.0662762646370231,0.,0.997801311256787));
#108243=DIRECTION('',(0.,-1.,-2.67523620391604E-16));
#108244=DIRECTION('',(0.,1.,2.67523620391604E-16));
#108245=DIRECTION('center_axis',(0.,1.,2.67523620391604E-16));
#108246=DIRECTION('ref_axis',(-1.,0.,-1.85631801868649E-33));
#108247=DIRECTION('',(0.,1.,2.67523620391604E-16));
#108248=DIRECTION('center_axis',(0.,1.,2.67523620391604E-16));
#108249=DIRECTION('ref_axis',(1.,1.85370757147271E-31,-6.93889390390722E-16));
#108250=DIRECTION('center_axis',(0.999999916511834,-1.09317472416637E-19,
0.000408627366273739));
#108251=DIRECTION('ref_axis',(0.000408627366273739,2.22046620305031E-16,
-0.999999916511834));
#108252=DIRECTION('',(0.,1.,2.67523620391604E-16));
#108253=DIRECTION('',(0.,1.,0.));
#108254=DIRECTION('center_axis',(0.,-1.,-2.67523620391604E-16));
#108255=DIRECTION('ref_axis',(0.707251238022098,0.,-0.706962294833472));
#108256=DIRECTION('',(0.,-1.,-2.67523620391604E-16));
#108257=DIRECTION('center_axis',(1.30472918803582E-12,2.67523620391604E-16,
-1.));
#108258=DIRECTION('ref_axis',(-1.,6.93889390419694E-18,-1.30472918803582E-12));
#108259=DIRECTION('',(-1.31710484347345E-28,1.,2.67523620391604E-16));
#108260=DIRECTION('center_axis',(0.,-1.,-1.6657509746814E-16));
#108261=DIRECTION('ref_axis',(-0.827170191871368,0.,-0.561951486944811));
#108262=DIRECTION('',(0.,-1.,-1.6657509746814E-16));
#108263=DIRECTION('center_axis',(0.,1.,1.6657509746814E-16));
#108264=DIRECTION('ref_axis',(1.,0.,1.15584692836443E-33));
#108265=DIRECTION('center_axis',(0.,-1.,0.));
#108266=DIRECTION('ref_axis',(0.141735171603208,0.,-0.989904612137255));
#108267=DIRECTION('',(0.,-1.,0.));
#108268=DIRECTION('center_axis',(0.,1.,0.));
#108269=DIRECTION('ref_axis',(2.48741143748787E-16,0.,1.));
#108270=DIRECTION('',(0.,1.,0.));
#108271=DIRECTION('center_axis',(3.2590836004222E-16,0.,1.));
#108272=DIRECTION('ref_axis',(1.,-6.93889390390704E-18,-3.2590836004222E-16));
#108273=DIRECTION('',(1.19092552242972E-16,1.,-3.88132583947496E-32));
#108274=DIRECTION('center_axis',(1.19092552242972E-16,1.,-3.88132583947496E-32));
#108275=DIRECTION('ref_axis',(0.51349131065734,0.,0.858094793061586));
#108276=DIRECTION('center_axis',(0.,1.,2.67523620391604E-16));
#108277=DIRECTION('ref_axis',(0.707106781186547,0.,0.707106781186547));
#108278=DIRECTION('center_axis',(0.,-1.,-2.22044604925031E-16));
#108279=DIRECTION('ref_axis',(0.707106781186547,0.,0.707106781186547));
#108280=DIRECTION('center_axis',(0.,-1.,-2.22044604925031E-16));
#108281=DIRECTION('ref_axis',(-0.934114852736578,0.,0.356972606647795));
#108282=DIRECTION('center_axis',(0.,1.,2.67523620391604E-16));
#108283=DIRECTION('ref_axis',(-0.984274724761795,4.72565661779708E-17,-0.176644462678832));
#108284=DIRECTION('',(0.,-1.,-2.67523620391604E-16));
#108285=DIRECTION('center_axis',(0.,-1.,-2.67523620391604E-16));
#108286=DIRECTION('ref_axis',(-0.753900508899602,0.,0.656988601636985));
#108287=DIRECTION('center_axis',(0.,1.,0.));
#108288=DIRECTION('ref_axis',(-0.000408627364868437,0.,0.999999916511835));
#108289=DIRECTION('center_axis',(0.,-1.,-2.22044604925031E-16));
#108290=DIRECTION('ref_axis',(-1.,0.,0.));
#108291=DIRECTION('center_axis',(0.,-1.,-2.22044604925031E-16));
#108292=DIRECTION('ref_axis',(-0.512525209353282,0.,0.858672178294705));
#108293=DIRECTION('',(-1.85435565520038E-14,-2.22044604925031E-16,1.));
#108294=DIRECTION('',(-0.707106781186548,-1.57009245868378E-16,0.707106781186548));
#108295=DIRECTION('center_axis',(0.,-1.,-2.22044604925031E-16));
#108296=DIRECTION('ref_axis',(-0.923879532511287,0.,-0.38268343236509));
#108297=DIRECTION('',(0.,-2.22044604925031E-16,1.));
#108298=DIRECTION('center_axis',(0.,1.,2.22044604925031E-16));
#108299=DIRECTION('ref_axis',(0.707106781186548,-1.57009245868377E-16,0.707106781186548));
#108300=DIRECTION('',(-1.,-2.58135112964991E-32,1.16253719856037E-16));
#108301=DIRECTION('center_axis',(0.,1.,2.22044604925031E-16));
#108302=DIRECTION('ref_axis',(-0.891123735454889,-1.00755045690416E-16,
0.453760386227053));
#108303=DIRECTION('center_axis',(0.,1.,2.22044604925031E-16));
#108304=DIRECTION('ref_axis',(-0.901335144845703,0.,-0.433122334526835));
#108305=DIRECTION('center_axis',(0.,-1.,-2.22044604925031E-16));
#108306=DIRECTION('ref_axis',(-1.,0.,0.));
#108307=DIRECTION('center_axis',(0.,-1.,-2.22044604925031E-16));
#108308=DIRECTION('ref_axis',(-1.,0.,0.));
#108309=DIRECTION('center_axis',(0.,1.,2.22044604925031E-16));
#108310=DIRECTION('ref_axis',(-0.785534661760763,1.24913747843662E-16,-0.618817659066387));
#108311=DIRECTION('center_axis',(0.,1.,2.22044604925031E-16));
#108312=DIRECTION('ref_axis',(-1.,0.,0.));
#108313=DIRECTION('',(0.308815713730941,-0.707106781186547,-0.636107581272893));
#108314=DIRECTION('center_axis',(0.,1.,2.01858731750028E-16));
#108315=DIRECTION('ref_axis',(-0.785534661760763,1.24913747843662E-16,-0.618817659066387));
#108316=DIRECTION('center_axis',(0.,-1.,-2.22044604925031E-16));
#108317=DIRECTION('ref_axis',(-0.901335144845703,0.,-0.433122334526835));
#108318=DIRECTION('center_axis',(-1.837501759903E-19,3.96508223080413E-16,
-1.));
#108319=DIRECTION('ref_axis',(-1.,6.93889390390712E-18,1.83750175990302E-19));
#108320=DIRECTION('',(0.,1.,3.96508223080413E-16));
#108321=DIRECTION('center_axis',(0.,1.,3.96508223080413E-16));
#108322=DIRECTION('ref_axis',(1.,0.,-1.837501759903E-19));
#108323=DIRECTION('',(0.,-1.,-3.96508223080413E-16));
#108324=DIRECTION('center_axis',(-1.,0.,0.));
#108325=DIRECTION('ref_axis',(0.,-2.22044604925031E-16,1.));
#108326=DIRECTION('center_axis',(-1.98445518114089E-16,-1.,-4.37374863265516E-16));
#108327=DIRECTION('ref_axis',(-0.512525209353282,0.,0.858672178294705));
#108328=DIRECTION('center_axis',(0.,-1.,-2.22044604925031E-16));
#108329=DIRECTION('ref_axis',(-1.,0.,0.));
#108330=DIRECTION('center_axis',(3.42121385298657E-49,-1.,-2.22044604925031E-16));
#108331=DIRECTION('ref_axis',(-1.,0.,-1.54077774334651E-33));
#108332=DIRECTION('center_axis',(3.42121385298657E-49,-1.,-2.22044604925031E-16));
#108333=DIRECTION('ref_axis',(-1.,0.,-1.54077774334651E-33));
#108334=DIRECTION('center_axis',(0.,1.,2.22044604925031E-16));
#108335=DIRECTION('ref_axis',(-1.,0.,0.));
#108336=DIRECTION('center_axis',(0.,-1.,-2.22044604925031E-16));
#108337=DIRECTION('ref_axis',(-1.,0.,0.));
#108338=DIRECTION('',(0.,1.,2.22044604925031E-16));
#108339=DIRECTION('center_axis',(0.,-1.,-2.22044604925031E-16));
#108340=DIRECTION('ref_axis',(1.,0.,0.));
#108341=DIRECTION('center_axis',(0.,1.,2.22044604925031E-16));
#108342=DIRECTION('ref_axis',(-1.,0.,0.));
#108343=DIRECTION('center_axis',(0.,-1.,-2.22044604925031E-16));
#108344=DIRECTION('ref_axis',(1.,0.,0.));
#108345=DIRECTION('',(0.,1.,2.22044604925031E-16));
#108346=DIRECTION('center_axis',(0.,1.,2.22044604925031E-16));
#108347=DIRECTION('ref_axis',(0.707106781186547,-1.57009245868377E-16,0.707106781186547));
#108348=DIRECTION('',(0.,1.,2.22044604925031E-16));
#108349=DIRECTION('center_axis',(0.,-1.,-2.22044604925031E-16));
#108350=DIRECTION('ref_axis',(0.707106781186547,-1.57009245868377E-16,0.707106781186547));
#108351=DIRECTION('',(0.,1.,2.22044604925031E-16));
#108352=DIRECTION('center_axis',(0.707106781186548,-1.57009245868377E-16,
0.707106781186548));
#108353=DIRECTION('ref_axis',(0.707106781186548,1.57009245868377E-16,-0.707106781186548));
#108354=DIRECTION('',(0.,1.,2.22044604925031E-16));
#108355=DIRECTION('',(-0.707106781186548,-1.57009245868377E-16,0.707106781186548));
#108356=DIRECTION('center_axis',(0.,1.,2.22044604925031E-16));
#108357=DIRECTION('ref_axis',(-0.707106781186547,1.57009245868377E-16,-0.707106781186547));
#108358=DIRECTION('',(0.,-1.,-2.22044604925031E-16));
#108359=DIRECTION('center_axis',(0.,-1.,-2.22044604925031E-16));
#108360=DIRECTION('ref_axis',(-0.707106781186547,1.57009245868377E-16,-0.707106781186547));
#108361=DIRECTION('center_axis',(0.,1.,2.22044604925031E-16));
#108362=DIRECTION('ref_axis',(0.707106781186548,-1.57009245868377E-16,0.707106781186548));
#108363=DIRECTION('center_axis',(0.,-1.,-2.22044604925031E-16));
#108364=DIRECTION('ref_axis',(0.707106781186548,-1.57009245868377E-16,0.707106781186548));
#108365=DIRECTION('',(0.,1.,2.22044604925031E-16));
#108366=DIRECTION('',(0.,1.,2.22044604925031E-16));
#108367=DIRECTION('center_axis',(-0.707106781186548,1.57009245868377E-16,
-0.707106781186548));
#108368=DIRECTION('ref_axis',(-0.707106781186548,-1.57009245868377E-16,
0.707106781186548));
#108369=DIRECTION('',(0.707106781186548,1.57009245868377E-16,-0.707106781186548));
#108370=DIRECTION('',(0.,1.,2.22044604925031E-16));
#108371=DIRECTION('center_axis',(0.,1.,2.22044604925031E-16));
#108372=DIRECTION('ref_axis',(-0.707106781186548,1.57009245868377E-16,-0.707106781186548));
#108373=DIRECTION('center_axis',(0.,-1.,-2.22044604925031E-16));
#108374=DIRECTION('ref_axis',(-0.707106781186548,1.57009245868377E-16,-0.707106781186548));
#108375=DIRECTION('',(0.,1.,2.22044604925031E-16));
#108376=DIRECTION('center_axis',(0.707106781186548,-1.57009245868377E-16,
0.707106781186548));
#108377=DIRECTION('ref_axis',(0.707106781186548,1.57009245868377E-16,-0.707106781186548));
#108378=DIRECTION('',(-0.707106781186548,-1.57009245868377E-16,0.707106781186548));
#108379=DIRECTION('center_axis',(3.42121385298657E-49,-1.,-2.22044604925031E-16));
#108380=DIRECTION('ref_axis',(-1.,0.,-1.54077774334651E-33));
#108381=DIRECTION('center_axis',(-3.42121385298657E-49,1.,2.22044604925031E-16));
#108382=DIRECTION('ref_axis',(-1.,0.,-1.54077774334651E-33));
#108383=DIRECTION('center_axis',(0.,-1.,-2.22044604925031E-16));
#108384=DIRECTION('ref_axis',(1.,0.,0.));
#108385=DIRECTION('',(0.,1.,2.22044604925031E-16));
#108386=DIRECTION('center_axis',(0.,1.,2.22044604925031E-16));
#108387=DIRECTION('ref_axis',(-1.,0.,0.));
#108388=DIRECTION('center_axis',(0.,1.,2.22044604925031E-16));
#108389=DIRECTION('ref_axis',(-1.,0.,0.));
#108390=DIRECTION('',(0.,1.,2.22044604925031E-16));
#108391=DIRECTION('center_axis',(0.,1.,2.22044604925031E-16));
#108392=DIRECTION('ref_axis',(0.360742674985292,2.07093317185659E-16,-0.932665386108253));
#108393=DIRECTION('center_axis',(0.,1.,2.22044604925031E-16));
#108394=DIRECTION('ref_axis',(0.360742674985292,2.07093317185659E-16,-0.932665386108253));
#108395=DIRECTION('',(0.,-1.,-2.22044604925031E-16));
#108396=DIRECTION('center_axis',(1.01862664414594E-31,1.,2.22044604925031E-16));
#108397=DIRECTION('ref_axis',(-0.370112462344042,0.,-0.928986956430299));
#108398=DIRECTION('center_axis',(0.,1.,2.22044604925031E-16));
#108399=DIRECTION('ref_axis',(-0.370112462344042,0.,-0.928986956430299));
#108400=DIRECTION('',(-1.01862664414594E-31,-1.,-2.22044604925031E-16));
#108401=DIRECTION('',(1.02531585888742E-31,1.,2.22044604925031E-16));
#108402=DIRECTION('center_axis',(0.0271346786627024,2.21962845174164E-16,
-0.999631786816462));
#108403=DIRECTION('ref_axis',(0.999631786816462,-6.02510900342743E-18,0.0271346786627024));
#108404=DIRECTION('',(0.,-1.,-2.22044604925031E-16));
#108405=DIRECTION('',(0.999631786816462,-6.02510900342743E-18,0.0271346786627024));
#108406=DIRECTION('center_axis',(0.,-1.,-2.22044604925031E-16));
#108407=DIRECTION('ref_axis',(-0.993670662656293,-2.49428489271903E-17,
0.112332605134053));
#108408=DIRECTION('center_axis',(0.,1.,2.22044604925031E-16));
#108409=DIRECTION('ref_axis',(-0.993670662656293,-2.49428489271903E-17,
0.112332605134053));
#108410=DIRECTION('center_axis',(0.,-1.,-2.22044604925031E-16));
#108411=DIRECTION('ref_axis',(0.707106781186548,1.57009245868377E-16,-0.707106781186548));
#108412=DIRECTION('center_axis',(0.,-1.,-2.22044604925031E-16));
#108413=DIRECTION('ref_axis',(0.69744724579616,-1.59125185820173E-16,0.716636127564994));
#108414=DIRECTION('center_axis',(0.,-1.,-2.22044604925031E-16));
#108415=DIRECTION('ref_axis',(0.69744724579616,-1.59125185820173E-16,0.716636127564994));
#108416=DIRECTION('center_axis',(0.,-1.,-2.22044604925031E-16));
#108417=DIRECTION('ref_axis',(-1.,0.,0.));
#108418=DIRECTION('center_axis',(0.,1.,2.22044604925031E-16));
#108419=DIRECTION('ref_axis',(-0.923879532511287,0.,-0.38268343236509));
#108420=DIRECTION('',(0.707106781186548,1.57009245868377E-16,-0.707106781186548));
#108421=DIRECTION('',(-1.,-2.58135112964991E-32,1.16253719856037E-16));
#108422=DIRECTION('center_axis',(0.,-1.,-2.22044604925031E-16));
#108423=DIRECTION('ref_axis',(0.707106781186548,-1.57009245868377E-16,0.707106781186548));
#108424=DIRECTION('',(0.,2.22044604925031E-16,-1.));
#108425=DIRECTION('center_axis',(0.,1.,2.22044604925031E-16));
#108426=DIRECTION('ref_axis',(0.89959196856447,-9.69738446503996E-17,0.436731370632224));
#108427=DIRECTION('center_axis',(0.,-1.,-2.22044604925031E-16));
#108428=DIRECTION('ref_axis',(1.,0.,0.));
#108429=DIRECTION('',(0.,1.,2.22044604925031E-16));
#108430=DIRECTION('center_axis',(0.,1.,2.22044604925031E-16));
#108431=DIRECTION('ref_axis',(-1.,0.,0.));
#108432=DIRECTION('',(0.,1.,2.22044604925031E-16));
#108433=DIRECTION('center_axis',(0.,-1.,-2.22044604925031E-16));
#108434=DIRECTION('ref_axis',(-1.,0.,0.));
#108435=DIRECTION('',(-0.707106781186547,0.707106781186547,7.04136402448281E-17));
#108436=DIRECTION('center_axis',(0.,-1.,-2.22044604925031E-16));
#108437=DIRECTION('ref_axis',(-0.891123735454889,-1.00755045690416E-16,
0.453760386227053));
#108438=DIRECTION('',(0.,1.,2.22044604925031E-16));
#108439=DIRECTION('center_axis',(1.16253719856037E-16,-2.22044604925031E-16,
1.));
#108440=DIRECTION('ref_axis',(-1.,-2.58135112964991E-32,1.16253719856037E-16));
#108441=DIRECTION('',(0.,-1.,-2.22044604925031E-16));
#108442=DIRECTION('center_axis',(0.,1.,2.22044604925031E-16));
#108443=DIRECTION('ref_axis',(0.707106781186548,-1.57009245868377E-16,0.707106781186548));
#108444=DIRECTION('',(0.,1.,2.22044604925031E-16));
#108445=DIRECTION('center_axis',(-1.,0.,0.));
#108446=DIRECTION('ref_axis',(0.,2.22044604925031E-16,-1.));
#108447=DIRECTION('',(0.,-1.,-2.22044604925031E-16));
#108448=DIRECTION('center_axis',(0.,-1.,-2.22044604925031E-16));
#108449=DIRECTION('ref_axis',(-0.923879532511287,0.,-0.38268343236509));
#108450=DIRECTION('',(1.74315279842105E-32,1.,2.22044604925031E-16));
#108451=DIRECTION('center_axis',(-0.707106781186548,1.57009245868378E-16,
-0.707106781186548));
#108452=DIRECTION('ref_axis',(0.707106781186548,1.57009245868378E-16,-0.707106781186548));
#108453=DIRECTION('',(-1.98173529318078E-45,1.,2.22044604925031E-16));
#108454=DIRECTION('center_axis',(-1.,4.11749668849466E-30,-1.85435565520038E-14));
#108455=DIRECTION('ref_axis',(1.85435565520038E-14,2.22044604925031E-16,
-1.));
#108456=DIRECTION('center_axis',(-1.11022302462516E-16,2.22044604925031E-16,
-1.));
#108457=DIRECTION('ref_axis',(-1.,-1.83750175990327E-19,1.11022302462516E-16));
#108458=DIRECTION('',(1.11022302462516E-16,-2.22044604925031E-16,1.));
#108459=DIRECTION('center_axis',(-1.,0.,-6.93889390390723E-17));
#108460=DIRECTION('ref_axis',(-6.93889390390723E-17,-6.93889390390724E-18,
1.));
#108461=DIRECTION('',(0.,-1.,0.));
#108462=DIRECTION('',(0.,1.,0.));
#108463=DIRECTION('',(6.93889390390723E-17,2.22049474265475E-16,-1.));
#108464=DIRECTION('center_axis',(6.93889390390722E-18,1.,2.22049474265475E-16));
#108465=DIRECTION('ref_axis',(-1.,6.93889390390721E-18,1.83750175990302E-19));
#108466=DIRECTION('center_axis',(-4.16333634234434E-17,1.,2.28983498828938E-16));
#108467=DIRECTION('ref_axis',(0.529831364669109,-1.72142934113367E-16,0.848103015566428));
#108468=DIRECTION('center_axis',(6.93889390390719E-18,1.,2.22049474265475E-16));
#108469=DIRECTION('ref_axis',(-0.805424049353576,1.37197252647342E-16,-0.59269899672843));
#108470=DIRECTION('center_axis',(0.,-1.,0.));
#108471=DIRECTION('ref_axis',(-0.805424049353576,0.,-0.59269899672843));
#108472=DIRECTION('',(0.,1.,0.));
#108473=DIRECTION('center_axis',(0.,-1.,0.));
#108474=DIRECTION('ref_axis',(0.456803537809492,0.,0.889567607236646));
#108475=DIRECTION('center_axis',(0.,1.,2.69144975666705E-16));
#108476=DIRECTION('ref_axis',(0.556470257418726,0.,-0.830867530120378));
#108477=DIRECTION('center_axis',(1.83750175990295E-19,-1.,-2.35922392732845E-16));
#108478=DIRECTION('ref_axis',(0.556470257418726,0.,-0.830867530120378));
#108479=DIRECTION('',(2.6329399793482E-17,-1.,-2.95474375460248E-16));
#108480=DIRECTION('center_axis',(0.,-1.,-2.22044604925031E-16));
#108481=DIRECTION('ref_axis',(0.556470257418726,0.,-0.830867530120378));
#108482=DIRECTION('',(0.,1.,2.69144975666705E-16));
#108483=DIRECTION('center_axis',(-1.83750175990295E-19,1.,2.35922392732845E-16));
#108484=DIRECTION('ref_axis',(1.,1.83750175990295E-19,4.08007322284045E-35));
#108485=DIRECTION('center_axis',(-1.83750175990295E-19,1.,2.35922392732845E-16));
#108486=DIRECTION('ref_axis',(-1.,0.,-1.86756843092096E-33));
#108487=DIRECTION('center_axis',(1.83750175990295E-19,-1.,-2.35922392732845E-16));
#108488=DIRECTION('ref_axis',(0.830867530119088,0.,-0.556470257420652));
#108489=DIRECTION('',(-0.707106781187368,1.6669239273947E-16,-0.707106781185727));
#108490=DIRECTION('center_axis',(1.83750175990295E-19,-1.,-2.35922392732845E-16));
#108491=DIRECTION('ref_axis',(-0.923879532510705,0.,0.382683432366495));
#108492=DIRECTION('',(-1.88260317010131E-12,2.35922392732845E-16,-1.));
#108493=DIRECTION('center_axis',(-1.83750175990295E-19,1.,2.35922392732845E-16));
#108494=DIRECTION('ref_axis',(0.877755401836952,0.,-0.479109021566127));
#108495=DIRECTION('center_axis',(1.83750175990295E-19,-1.,-2.35922392732845E-16));
#108496=DIRECTION('ref_axis',(-0.674528301887451,-1.98696006215612E-16,
0.738248989130924));
#108497=DIRECTION('center_axis',(-1.83750175990295E-19,1.,2.35922392732845E-16));
#108498=DIRECTION('ref_axis',(-0.439524536496337,0.,-0.898230583880153));
#108499=DIRECTION('',(-1.88249434430459E-12,2.35922392732845E-16,-1.));
#108500=DIRECTION('center_axis',(-1.83750175990295E-19,1.,2.35922392732845E-16));
#108501=DIRECTION('ref_axis',(-0.923879532510705,0.,0.382683432366494));
#108502=DIRECTION('',(-0.707106781187368,1.6669239273947E-16,-0.707106781185727));
#108503=DIRECTION('center_axis',(-1.83750175990295E-19,1.,2.35922392732845E-16));
#108504=DIRECTION('ref_axis',(-0.382683432364554,0.,0.923879532511509));
#108505=DIRECTION('',(1.,1.83750175990323E-19,-1.16253719856037E-16));
#108506=DIRECTION('center_axis',(-1.83750175990295E-19,1.,2.35922392732845E-16));
#108507=DIRECTION('ref_axis',(2.55004895630733E-36,-2.22044604925031E-16,
1.));
#108508=DIRECTION('',(-0.868387762761633,1.16830990166913E-16,-0.495885766569122));
#108509=DIRECTION('center_axis',(-1.83750175990295E-19,1.,2.35922392732845E-16));
#108510=DIRECTION('ref_axis',(0.157787733663648,2.19263064006667E-16,-0.987473053356541));
#108511=DIRECTION('',(1.,1.83750175990065E-19,9.76990079422698E-16));
#108512=DIRECTION('center_axis',(1.83750175990295E-19,-1.,-2.35922392732845E-16));
#108513=DIRECTION('ref_axis',(-0.382683432364555,0.,0.923879532511508));
#108514=DIRECTION('',(-0.707106781187368,1.6669239273947E-16,-0.707106781185727));
#108515=DIRECTION('center_axis',(0.,1.,2.69144975666705E-16));
#108516=DIRECTION('ref_axis',(-1.,0.,-1.86756843092096E-33));
#108517=DIRECTION('center_axis',(0.,1.,2.22044604925031E-16));
#108518=DIRECTION('ref_axis',(-1.,0.,-1.86756843092096E-33));
#108519=DIRECTION('',(0.,-1.,-2.69144975666705E-16));
#108520=DIRECTION('center_axis',(0.,-1.,-2.69144975666705E-16));
#108521=DIRECTION('ref_axis',(0.830867530119088,0.,-0.556470257420652));
#108522=DIRECTION('center_axis',(0.,-1.,-2.22044604925031E-16));
#108523=DIRECTION('ref_axis',(0.830867530119088,0.,-0.556470257420652));
#108524=DIRECTION('',(-2.6329399793482E-17,1.,2.95474375460248E-16));
#108525=DIRECTION('center_axis',(0.707106781185727,2.27549631693565E-16,
-0.707106781187368));
#108526=DIRECTION('ref_axis',(-0.707106781187368,1.61919227945235E-16,-0.707106781185727));
#108527=DIRECTION('',(0.707106781187368,-1.57009245868195E-16,0.707106781185727));
#108528=DIRECTION('',(0.,1.,0.));
#108529=DIRECTION('',(0.707106781187368,-1.61919227945235E-16,0.707106781185727));
#108530=DIRECTION('',(3.48630559683805E-32,-1.,-3.21803775253669E-16));
#108531=DIRECTION('center_axis',(6.93889390390724E-18,1.,2.22049474265475E-16));
#108532=DIRECTION('ref_axis',(0.,0.,1.));
#108533=DIRECTION('center_axis',(0.55526819475842,0.,-0.831671348484319));
#108534=DIRECTION('ref_axis',(0.831671348484319,0.,0.55526819475842));
#108535=DIRECTION('center_axis',(6.93889390390724E-18,1.,2.22049474265475E-16));
#108536=DIRECTION('ref_axis',(-0.953563413137572,7.34962729527946E-17,-0.301192325807655));
#108537=DIRECTION('center_axis',(-0.023198104831873,0.,0.999730887755405));
#108538=DIRECTION('ref_axis',(0.,-1.,0.));
#108539=DIRECTION('center_axis',(-6.93889390390724E-18,-1.,-2.22049474265475E-16));
#108540=DIRECTION('ref_axis',(-0.953563413137572,5.96894099260837E-17,-0.301192325807655));
#108541=DIRECTION('center_axis',(-0.707106781187369,0.,-0.707106781185726));
#108542=DIRECTION('ref_axis',(0.,-1.,0.));
#108543=DIRECTION('center_axis',(6.93889390390724E-18,1.,2.22049474265475E-16));
#108544=DIRECTION('ref_axis',(0.371940837143499,-1.7347234759768E-16,0.928256437448722));
#108545=DIRECTION('center_axis',(-6.93889390390724E-18,-1.,-2.22049474265475E-16));
#108546=DIRECTION('ref_axis',(0.371940837143499,-2.08699711926501E-16,0.928256437448722));
#108547=DIRECTION('center_axis',(-0.707106781187368,1.61919227945235E-16,
-0.707106781185727));
#108548=DIRECTION('ref_axis',(-0.499999999999422,-0.707106781186549,0.500000000000576));
#108549=DIRECTION('center_axis',(-0.707106781187366,0.,-0.707106781185729));
#108550=DIRECTION('ref_axis',(0.,-1.,0.));
#108551=DIRECTION('',(-0.707106781187368,1.61919227945235E-16,-0.707106781185727));
#108552=DIRECTION('center_axis',(-1.88182802673964E-12,0.,-1.));
#108553=DIRECTION('ref_axis',(0.,-1.,0.));
#108554=DIRECTION('center_axis',(6.93889390390724E-18,1.,2.22049474265475E-16));
#108555=DIRECTION('ref_axis',(-0.923879532510704,-8.67361737988403E-17,
0.382683432366496));
#108556=DIRECTION('center_axis',(-6.93889390390724E-18,-1.,-2.22049474265475E-16));
#108557=DIRECTION('ref_axis',(-0.923879532510704,-7.85639529110046E-17,
0.382683432366496));
#108558=DIRECTION('center_axis',(-1.88260317010131E-12,2.22049474265488E-16,
-1.));
#108559=DIRECTION('ref_axis',(-0.707106781186548,-0.707106781186548,1.3306533587345E-12));
#108560=DIRECTION('center_axis',(-1.88182802673964E-12,0.,-1.));
#108561=DIRECTION('ref_axis',(0.,-1.,0.));
#108562=DIRECTION('',(1.88260317010131E-12,-2.22049474265488E-16,1.));
#108563=DIRECTION('',(-1.88260317010131E-12,2.22049474265488E-16,-1.));
#108564=DIRECTION('center_axis',(0.909059342886221,0.,0.41666666666686));
#108565=DIRECTION('ref_axis',(0.,-1.,0.));
#108566=DIRECTION('center_axis',(6.93889390390724E-18,1.,2.22049474265475E-16));
#108567=DIRECTION('ref_axis',(-0.540061724868026,1.7347234759768E-16,-0.841625411529721));
#108568=DIRECTION('center_axis',(-6.93889390390724E-18,-1.,-2.22049474265475E-16));
#108569=DIRECTION('ref_axis',(-0.540061724868026,1.90629911169059E-16,-0.841625411529721));
#108570=DIRECTION('center_axis',(6.93889390390724E-18,1.,2.22049474265475E-16));
#108571=DIRECTION('ref_axis',(0.,-3.11641550771974E-16,1.));
#108572=DIRECTION('center_axis',(0.950100400237196,0.,0.311944273018627));
#108573=DIRECTION('ref_axis',(0.,-1.,0.));
#108574=DIRECTION('center_axis',(-6.93889390390724E-18,-1.,-2.22049474265475E-16));
#108575=DIRECTION('ref_axis',(-0.364882950347729,-2.09476042382105E-16,
0.931053399406036));
#108576=DIRECTION('center_axis',(6.93889390390724E-18,1.,2.22049474265475E-16));
#108577=DIRECTION('ref_axis',(-0.364882950347729,-2.04208033771386E-16,
0.931053399406036));
#108578=DIRECTION('center_axis',(6.93889390390724E-18,1.,2.22049474265475E-16));
#108579=DIRECTION('ref_axis',(0.945250138395208,1.15648231731787E-16,-0.326346711127658));
#108580=DIRECTION('center_axis',(-6.93889390390724E-18,-1.,-2.22049474265475E-16));
#108581=DIRECTION('ref_axis',(0.945250138395208,6.59061252111853E-17,-0.326346711127658));
#108582=DIRECTION('center_axis',(0.,-1.,-2.41352831440251E-16));
#108583=DIRECTION('ref_axis',(-0.540061724868023,0.,-0.841625411529723));
#108584=DIRECTION('',(0.,1.,2.41352831440251E-16));
#108585=DIRECTION('center_axis',(0.,1.,2.22044604925031E-16));
#108586=DIRECTION('ref_axis',(-0.540061724868023,0.,-0.841625411529723));
#108587=DIRECTION('',(1.51457201860782E-28,-1.,-2.41352831440251E-16));
#108588=DIRECTION('center_axis',(0.,-1.,-2.41352831440251E-16));
#108589=DIRECTION('ref_axis',(-1.,1.74423844019976E-32,-6.93889390390723E-17));
#108590=DIRECTION('',(0.,-1.,-2.41352831440251E-16));
#108591=DIRECTION('center_axis',(0.,1.,2.22044604925031E-16));
#108592=DIRECTION('ref_axis',(-1.,1.74423844019976E-32,-6.93889390390723E-17));
#108593=DIRECTION('center_axis',(0.,-1.,-1.60901887626834E-16));
#108594=DIRECTION('ref_axis',(0.945250138395209,0.,-0.326346711127656));
#108595=DIRECTION('',(0.,1.,1.60901887626834E-16));
#108596=DIRECTION('center_axis',(0.,1.,2.22044604925031E-16));
#108597=DIRECTION('ref_axis',(0.945250138395209,0.,-0.326346711127656));
#108598=DIRECTION('center_axis',(0.,-1.,-1.60901887626834E-16));
#108599=DIRECTION('ref_axis',(-1.,1.32537114452455E-32,-6.93889390390723E-17));
#108600=DIRECTION('',(0.,-1.,-1.60901887626834E-16));
#108601=DIRECTION('center_axis',(0.,1.,2.22044604925031E-16));
#108602=DIRECTION('ref_axis',(-1.,0.,0.));
#108603=DIRECTION('',(0.,1.,1.60901887626834E-16));
#108604=DIRECTION('center_axis',(0.,1.,2.22044604925031E-16));
#108605=DIRECTION('ref_axis',(-1.,0.,0.));
#108606=DIRECTION('center_axis',(6.93889390390724E-18,1.,2.22049474265475E-16));
#108607=DIRECTION('ref_axis',(-1.,6.93889390390724E-18,1.83750175990302E-19));
#108608=DIRECTION('center_axis',(0.,-1.,-2.22044604925031E-16));
#108609=DIRECTION('ref_axis',(0.,0.,-1.));
#108610=DIRECTION('center_axis',(0.,-1.,-2.22044604925031E-16));
#108611=DIRECTION('ref_axis',(-0.223884986531161,2.16408129595356E-16,-0.974615571805592));
#108612=DIRECTION('center_axis',(0.89959196856447,0.,0.436731370632225));
#108613=DIRECTION('ref_axis',(0.,-1.,0.));
#108614=DIRECTION('center_axis',(0.,1.,2.22044604925031E-16));
#108615=DIRECTION('ref_axis',(-0.223884986531161,2.08166817117217E-16,-0.974615571805592));
#108616=DIRECTION('center_axis',(0.,-1.,-2.22044604925031E-16));
#108617=DIRECTION('ref_axis',(0.,0.,-1.));
#108618=DIRECTION('center_axis',(0.,-1.,-2.22044604925031E-16));
#108619=DIRECTION('ref_axis',(-0.999460488335693,-7.29284625413709E-18,
0.0328440596726021));
#108620=DIRECTION('center_axis',(3.46944695195253E-16,3.46944695195361E-16,
-1.));
#108621=DIRECTION('ref_axis',(0.,-1.,-3.46944695195361E-16));
#108622=DIRECTION('center_axis',(0.,1.,2.22044604925031E-16));
#108623=DIRECTION('ref_axis',(-0.999460488335693,0.,0.0328440596726021));
#108624=DIRECTION('center_axis',(2.22628932034678E-16,2.22044604925031E-16,
-1.));
#108625=DIRECTION('ref_axis',(-0.707106781186549,-0.707106781186546,-4.90653893338678E-16));
#108626=DIRECTION('center_axis',(0.,0.,-1.));
#108627=DIRECTION('ref_axis',(0.,-1.,0.));
#108628=DIRECTION('',(-2.22628932034678E-16,-2.22044604925031E-16,1.));
#108629=DIRECTION('',(2.22628932034678E-16,2.22044604925031E-16,-1.));
#108630=DIRECTION('center_axis',(0.,-1.,-2.22044604925031E-16));
#108631=DIRECTION('ref_axis',(0.,0.,-1.));
#108632=DIRECTION('center_axis',(0.,1.,2.22044604925031E-16));
#108633=DIRECTION('ref_axis',(-0.999213555456797,0.,-0.0396518674388288));
#108634=DIRECTION('center_axis',(0.,-1.,-2.22044604925031E-16));
#108635=DIRECTION('ref_axis',(-0.999213555456797,8.80448323999446E-18,-0.0396518674388288));
#108636=DIRECTION('center_axis',(0.,-1.,-2.22044604925031E-16));
#108637=DIRECTION('ref_axis',(0.,2.04238085258919E-16,-1.));
#108638=DIRECTION('center_axis',(0.,-1.,-2.22044604925031E-16));
#108639=DIRECTION('ref_axis',(-0.229661543013825,-2.16109476147391E-16,
0.973270556248625));
#108640=DIRECTION('center_axis',(-0.899591968564469,0.,-0.436731370632226));
#108641=DIRECTION('ref_axis',(0.,-1.,0.));
#108642=DIRECTION('center_axis',(0.,1.,2.22044604925031E-16));
#108643=DIRECTION('ref_axis',(-0.229661543013825,-2.15407355546517E-16,
0.973270556248625));
#108644=DIRECTION('center_axis',(0.,-1.,-2.22044604925031E-16));
#108645=DIRECTION('ref_axis',(0.,0.,-1.));
#108646=DIRECTION('center_axis',(0.,1.,2.22044604925031E-16));
#108647=DIRECTION('ref_axis',(-0.627438795144384,-1.73472347597681E-16,
0.778665883641863));
#108648=DIRECTION('center_axis',(0.,-1.,-2.22044604925031E-16));
#108649=DIRECTION('ref_axis',(-0.627438795144384,-1.72898558501858E-16,
0.778665883641863));
#108650=DIRECTION('center_axis',(0.,1.,2.22044604925031E-16));
#108651=DIRECTION('ref_axis',(0.,-3.48477392031983E-16,1.));
#108652=DIRECTION('center_axis',(0.,-1.,-2.22044604925031E-16));
#108653=DIRECTION('ref_axis',(-0.234423796430946,-2.14187059826031E-16,
0.972134498753595));
#108654=DIRECTION('center_axis',(0.,1.,2.22044604925031E-16));
#108655=DIRECTION('ref_axis',(-0.234423796430946,-2.15857220709735E-16,
0.972134498753594));
#108656=DIRECTION('center_axis',(1.88212241265405E-12,-2.22044604925031E-16,
1.));
#108657=DIRECTION('ref_axis',(0.707106781186548,-0.707106781186548,-1.3306533587345E-12));
#108658=DIRECTION('',(-1.88212241265405E-12,2.22044604925031E-16,-1.));
#108659=DIRECTION('',(1.88212241265405E-12,-2.22044604925031E-16,1.));
#108660=DIRECTION('center_axis',(0.,-1.,-2.77555756156289E-16));
#108661=DIRECTION('ref_axis',(-1.,0.,0.));
#108662=DIRECTION('',(0.,-1.,-2.77555756156289E-16));
#108663=DIRECTION('center_axis',(0.,-1.,-2.22044604925031E-16));
#108664=DIRECTION('ref_axis',(-1.,0.,0.));
#108665=DIRECTION('',(0.,1.,2.77555756156289E-16));
#108666=DIRECTION('center_axis',(0.,-1.,-2.77555756156289E-16));
#108667=DIRECTION('ref_axis',(0.89959196856447,-1.21217305812999E-16,0.436731370632224));
#108668=DIRECTION('',(0.,1.,2.77555756156289E-16));
#108669=DIRECTION('center_axis',(0.,1.,2.22044604925031E-16));
#108670=DIRECTION('ref_axis',(0.89959196856447,-9.69738446503996E-17,0.436731370632224));
#108671=DIRECTION('center_axis',(-1.,-5.22393909422894E-28,1.88212241265405E-12));
#108672=DIRECTION('ref_axis',(1.88212241265405E-12,-2.22044604925031E-16,
1.));
#108673=DIRECTION('',(0.,-1.,-2.77555756156289E-16));
#108674=DIRECTION('',(1.88212241265405E-12,-2.22044604925031E-16,1.));
#108675=DIRECTION('center_axis',(0.,-1.,-2.77555756156289E-16));
#108676=DIRECTION('ref_axis',(0.89959196856447,-1.21217305812999E-16,0.436731370632224));
#108677=DIRECTION('',(0.,-1.,-2.77555756156289E-16));
#108678=DIRECTION('center_axis',(0.,-1.,-2.22044604925031E-16));
#108679=DIRECTION('ref_axis',(0.89959196856447,-9.69738446503996E-17,0.436731370632224));
#108680=DIRECTION('center_axis',(0.,1.,2.22044604925031E-16));
#108681=DIRECTION('ref_axis',(-1.,0.,0.));
#108682=DIRECTION('center_axis',(6.93889390390722E-18,1.,2.22049474265475E-16));
#108683=DIRECTION('ref_axis',(0.,-2.87669123789514E-16,1.));
#108684=DIRECTION('center_axis',(6.93889390390722E-18,1.,2.22049474265475E-16));
#108685=DIRECTION('ref_axis',(-0.540572225751839,-1.83058718699731E-16,
0.84129761009152));
#108686=DIRECTION('center_axis',(0.881309715225975,0.,0.472539083937308));
#108687=DIRECTION('ref_axis',(0.,-1.,0.));
#108688=DIRECTION('center_axis',(-6.93889390390722E-18,-1.,-2.22049474265475E-16));
#108689=DIRECTION('ref_axis',(-0.540572225751839,-1.80231010491097E-16,
0.84129761009152));
#108690=DIRECTION('center_axis',(-0.577747036373043,0.,0.816215879508703));
#108691=DIRECTION('ref_axis',(0.,-1.,0.));
#108692=DIRECTION('center_axis',(6.93889390390722E-18,1.,2.22049474265475E-16));
#108693=DIRECTION('ref_axis',(0.973362209071398,0.,-0.229272785021789));
#108694=DIRECTION('center_axis',(-6.93889390390722E-18,-1.,-2.22049474265475E-16));
#108695=DIRECTION('ref_axis',(0.973362209071398,4.41558442786504E-17,-0.229272785021789));
#108696=DIRECTION('center_axis',(6.93889390390722E-18,1.,2.22049474265475E-16));
#108697=DIRECTION('ref_axis',(0.,0.,1.));
#108698=DIRECTION('center_axis',(6.93889390390722E-18,1.,2.22049474265475E-16));
#108699=DIRECTION('ref_axis',(-0.98001004047213,-3.73761208507432E-17,0.198948034857887));
#108700=DIRECTION('center_axis',(-6.93889390390722E-18,-1.,-2.22049474265475E-16));
#108701=DIRECTION('ref_axis',(-0.98001004047213,-3.65204942310907E-17,0.198948034857887));
#108702=DIRECTION('center_axis',(6.93889390390722E-18,1.,2.22049474265475E-16));
#108703=DIRECTION('ref_axis',(-0.98001004047213,-3.73761208507432E-17,0.198948034857887));
#108704=DIRECTION('center_axis',(0.,-1.,0.));
#108705=DIRECTION('ref_axis',(-0.832437275985664,0.,0.55411928458552));
#108706=DIRECTION('',(0.,-1.,0.));
#108707=DIRECTION('',(4.44089209850063E-17,-1.,-2.66453525910038E-16));
#108708=DIRECTION('',(0.,-1.,0.));
#108709=DIRECTION('center_axis',(0.,1.,2.22044604925031E-16));
#108710=DIRECTION('ref_axis',(-0.832437275985664,0.,0.55411928458552));
#108711=DIRECTION('',(0.,1.,0.));
#108712=DIRECTION('',(0.,-1.,0.));
#108713=DIRECTION('center_axis',(0.,-1.,0.));
#108714=DIRECTION('ref_axis',(-0.472539083937309,0.,0.881309715225975));
#108715=DIRECTION('',(0.,1.,0.));
#108716=DIRECTION('center_axis',(0.,1.,2.22044604925031E-16));
#108717=DIRECTION('ref_axis',(-1.,0.,0.));
#108718=DIRECTION('',(0.,1.,2.22044604925031E-16));
#108719=DIRECTION('center_axis',(0.,1.,2.22044604925031E-16));
#108720=DIRECTION('ref_axis',(-1.,0.,0.));
#108721=DIRECTION('center_axis',(0.,1.,2.22044604925031E-16));
#108722=DIRECTION('ref_axis',(-1.,0.,0.));
#108723=DIRECTION('center_axis',(-1.88016196282748E-14,-2.22049474265475E-16,
1.));
#108724=DIRECTION('ref_axis',(0.707106781186548,-0.707106781186548,1.57009245868377E-14));
#108725=DIRECTION('',(-1.88016196282748E-14,-2.22049474265475E-16,1.));
#108726=DIRECTION('center_axis',(-1.66533453693773E-14,0.,1.));
#108727=DIRECTION('ref_axis',(0.,-1.,0.));
#108728=DIRECTION('',(1.88016196282748E-14,2.22049474265475E-16,-1.));
#108729=DIRECTION('center_axis',(6.93889390390722E-18,1.,2.22049474265475E-16));
#108730=DIRECTION('ref_axis',(-1.,6.93889390390721E-18,1.83750175990302E-19));
#108731=DIRECTION('',(0.,2.22049474265475E-16,-1.));
#108732=DIRECTION('',(-1.,6.93889390390743E-18,-9.76990079422698E-16));
#108733=DIRECTION('center_axis',(-6.93889390390722E-18,-1.,-2.22049474265475E-16));
#108734=DIRECTION('ref_axis',(0.70710678118654,-1.61919227945413E-16,0.707106781186555));
#108735=DIRECTION('center_axis',(1.,0.,0.));
#108736=DIRECTION('ref_axis',(0.,3.08148791101958E-33,-1.));
#108737=DIRECTION('center_axis',(1.,0.,0.));
#108738=DIRECTION('ref_axis',(1.9854940640545E-17,-2.52712137005744E-16,
1.));
#108739=DIRECTION('',(0.,1.,0.));
#108740=DIRECTION('',(2.22044604925031E-16,-2.22044604925031E-16,1.));
#108741=DIRECTION('',(0.,1.,2.77555756156289E-16));
#108742=DIRECTION('center_axis',(1.,0.,0.));
#108743=DIRECTION('ref_axis',(-4.90653893338679E-16,-0.707106781186548,
0.707106781186548));
#108744=DIRECTION('center_axis',(-1.,0.,-1.38777878078144E-15));
#108745=DIRECTION('ref_axis',(0.,-1.,0.));
#108746=DIRECTION('center_axis',(6.93889390390722E-18,1.,2.22049474265475E-16));
#108747=DIRECTION('ref_axis',(0.70710678118654,-1.15648231731787E-16,0.707106781186555));
#108748=DIRECTION('center_axis',(-1.,6.93889390390743E-18,-9.76990079422698E-16));
#108749=DIRECTION('ref_axis',(-4.90653893338679E-16,-0.707106781186548,
0.707106781186548));
#108750=DIRECTION('',(1.,-6.93889390390743E-18,9.76990079422698E-16));
#108751=DIRECTION('center_axis',(1.,-4.17479820231099E-30,1.88016196282748E-14));
#108752=DIRECTION('ref_axis',(1.88016196282748E-14,0.,-1.));
#108753=DIRECTION('',(1.04369955057775E-30,-1.,-2.77555756156289E-16));
#108754=DIRECTION('center_axis',(-1.,4.17479820231099E-30,-1.88016196282748E-14));
#108755=DIRECTION('ref_axis',(-1.26584900907556E-14,-0.898717034276078,
0.438529009647037));
#108756=DIRECTION('center_axis',(-1.,4.17479820231099E-30,-1.88016196282748E-14));
#108757=DIRECTION('ref_axis',(-1.85037170770859E-14,-2.22044604925031E-16,
1.));
#108758=DIRECTION('',(0.,1.,2.22044604925031E-16));
#108759=DIRECTION('center_axis',(1.,-4.17479820231099E-30,1.88016196282748E-14));
#108760=DIRECTION('ref_axis',(-1.85037170770859E-14,-2.22044604925031E-16,
1.));
#108761=DIRECTION('center_axis',(1.04369955057775E-30,-1.,-2.77555756156289E-16));
#108762=DIRECTION('ref_axis',(0.707106781186538,0.,0.707106781186557));
#108763=DIRECTION('',(-1.04369955057775E-30,1.,2.77555756156289E-16));
#108764=DIRECTION('center_axis',(-9.76990079422698E-16,-2.77555756156289E-16,
1.));
#108765=DIRECTION('ref_axis',(1.,-6.93889390390734E-18,9.76990079422698E-16));
#108766=DIRECTION('center_axis',(-1.26161707343768E-16,2.22044604925031E-16,
-1.));
#108767=DIRECTION('ref_axis',(-0.674310247716091,-0.738448163262029,-7.46314788228609E-17));
#108768=DIRECTION('',(2.53017617534078E-17,-1.,-2.77555756156289E-16));
#108769=DIRECTION('',(-1.,2.16935376201088E-31,-9.76990079422698E-16));
#108770=DIRECTION('',(1.27117486340087E-16,1.,2.77555756156289E-16));
#108771=DIRECTION('',(1.,-1.13108869885842E-30,5.02293560613052E-15));
#108772=DIRECTION('',(-8.41078048960409E-18,-1.,-2.77555756156289E-16));
#108773=DIRECTION('',(0.,1.,2.22044604925031E-16));
#108774=DIRECTION('',(-1.,4.69398999576592E-31,-2.11398515958123E-15));
#108775=DIRECTION('',(2.63976927864639E-32,1.,2.77555756156289E-16));
#108776=DIRECTION('',(1.,-2.7116922025136E-31,9.76990079422698E-16));
#108777=DIRECTION('',(1.,7.55993416755167E-31,9.76990079422697E-16));
#108778=DIRECTION('center_axis',(-0.323730285810082,2.12338308705133E-16,
-0.946149407889326));
#108779=DIRECTION('ref_axis',(-0.669028662334179,-0.707106781186547,0.228911880371771));
#108780=DIRECTION('',(-0.323730285810082,2.12338308705133E-16,-0.946149407889326));
#108781=DIRECTION('center_axis',(-0.164089292933262,0.,-0.986445489596188));
#108782=DIRECTION('ref_axis',(0.986445489596187,-1.2940412193226E-15,-0.164089292933262));
#108783=DIRECTION('',(0.323730285810082,-2.12338308705133E-16,0.946149407889326));
#108784=DIRECTION('center_axis',(6.93889390390723E-17,2.22049474265475E-16,
-1.));
#108785=DIRECTION('ref_axis',(-0.707106781186548,-0.707106781186548,0.));
#108786=DIRECTION('center_axis',(0.808736084303188,0.,-0.588171697675047));
#108787=DIRECTION('ref_axis',(-0.588171697675047,2.04063050372407E-16,-0.808736084303188));
#108788=DIRECTION('',(-6.93889390390723E-17,-2.22049474265475E-16,1.));
#108789=DIRECTION('',(6.93889390390723E-17,2.22049474265475E-16,-1.));
#108790=DIRECTION('center_axis',(0.946149407889326,0.,-0.323730285810082));
#108791=DIRECTION('ref_axis',(-0.323730285810082,5.66263013082985E-17,-0.946149407889326));
#108792=DIRECTION('',(0.,1.,0.));
#108793=DIRECTION('center_axis',(1.,0.,6.93889390390723E-17));
#108794=DIRECTION('ref_axis',(6.93889390390723E-17,6.93889390390724E-18,
-1.));
#108795=DIRECTION('',(0.,1.,0.));
#108796=DIRECTION('',(-1.11022302462516E-16,2.22044604925031E-16,-1.));
#108797=DIRECTION('center_axis',(6.93889390390722E-18,1.,2.22049474265475E-16));
#108798=DIRECTION('ref_axis',(0.,0.,1.));
#108799=DIRECTION('center_axis',(6.93889390390722E-18,1.,2.22049474265475E-16));
#108800=DIRECTION('ref_axis',(0.973489193493256,-5.75449829877939E-17,0.22873301062997));
#108801=DIRECTION('center_axis',(-0.00226873389465586,0.,-0.999997426419946));
#108802=DIRECTION('ref_axis',(0.,-1.,0.));
#108803=DIRECTION('center_axis',(-6.93889390390722E-18,-1.,-2.22049474265475E-16));
#108804=DIRECTION('ref_axis',(0.973489193493256,-5.4780741346636E-17,0.22873301062997));
#108805=DIRECTION('center_axis',(0.990019786637194,0.,0.140928428880923));
#108806=DIRECTION('ref_axis',(0.,-1.,0.));
#108807=DIRECTION('center_axis',(6.93889390390722E-18,1.,2.22049474265475E-16));
#108808=DIRECTION('ref_axis',(-0.656246152467199,1.15648231731787E-16,-0.754546875529942));
#108809=DIRECTION('center_axis',(-6.93889390390722E-18,-1.,-2.22049474265475E-16));
#108810=DIRECTION('ref_axis',(-0.656246152467199,1.72100359446898E-16,-0.754546875529942));
#108811=DIRECTION('center_axis',(6.93889390390722E-18,1.,2.22049474265475E-16));
#108812=DIRECTION('ref_axis',(0.,-2.75992927452516E-16,1.));
#108813=DIRECTION('center_axis',(0.991102794140644,0.,0.133098653060836));
#108814=DIRECTION('ref_axis',(0.,-1.,0.));
#108815=DIRECTION('center_axis',(-6.93889390390722E-18,-1.,-2.22049474265475E-16));
#108816=DIRECTION('ref_axis',(-0.137014611029961,-2.19752839926614E-16,
0.990569026552066));
#108817=DIRECTION('center_axis',(6.93889390390722E-18,1.,2.22049474265475E-16));
#108818=DIRECTION('ref_axis',(-0.137014611029961,-2.19004601720328E-16,
0.990569026552066));
#108819=DIRECTION('center_axis',(-2.22044604925031E-14,0.,1.));
#108820=DIRECTION('ref_axis',(0.,-1.,0.));
#108821=DIRECTION('center_axis',(6.93889390390722E-18,1.,2.22049474265475E-16));
#108822=DIRECTION('ref_axis',(0.752694710045468,1.15648231731787E-16,-0.658369708803168));
#108823=DIRECTION('center_axis',(-6.93889390390722E-18,-1.,-2.22049474265475E-16));
#108824=DIRECTION('ref_axis',(0.752694710045468,1.4096777897702E-16,-0.658369708803168));
#108825=DIRECTION('center_axis',(-2.57651168044591E-14,-2.22049474265475E-16,
1.));
#108826=DIRECTION('ref_axis',(0.707106781186548,-0.707106781186548,1.57009245868377E-14));
#108827=DIRECTION('',(2.57651168044591E-14,2.22049474265475E-16,-1.));
#108828=DIRECTION('',(-2.57651168044591E-14,-2.22049474265475E-16,1.));
#108829=DIRECTION('center_axis',(-0.707106781186563,0.,0.707106781186532));
#108830=DIRECTION('ref_axis',(-0.707106781186532,3.14025378024051E-16,-0.707106781186563));
#108831=DIRECTION('center_axis',(-1.,6.9388939039087E-18,-6.67785932371251E-15));
#108832=DIRECTION('ref_axis',(-3.92523114670943E-15,-0.707106781186548,
0.707106781186548));
#108833=DIRECTION('',(1.,-6.9388939039087E-18,6.67785932371251E-15));
#108834=DIRECTION('',(-1.,6.9388939039087E-18,-6.67785932371251E-15));
#108835=DIRECTION('center_axis',(1.,-6.86520621803209E-30,2.57651168044591E-14));
#108836=DIRECTION('ref_axis',(-2.57651168044591E-14,-2.2898349882894E-16,
1.));
#108837=DIRECTION('',(6.86520621803209E-30,1.,4.58448813522947E-44));
#108838=DIRECTION('center_axis',(-1.,6.86520621803209E-30,-2.57651168044591E-14));
#108839=DIRECTION('ref_axis',(1.97111506292388E-14,0.643991722633251,-0.765032457598929));
#108840=DIRECTION('',(8.62629387613302E-31,-1.,-2.99934041219171E-16));
#108841=DIRECTION('',(-2.57651168044591E-14,-2.22044604925031E-16,1.));
#108842=DIRECTION('',(0.,1.,2.66453525910038E-16));
#108843=DIRECTION('center_axis',(6.67785932371251E-15,0.,-1.));
#108844=DIRECTION('ref_axis',(-1.,-3.76269782527349E-17,-6.67785932371251E-15));
#108845=DIRECTION('',(0.,1.,2.22044604925031E-16));
#108846=DIRECTION('',(0.,-1.,-2.22044604925031E-16));
#108847=DIRECTION('',(-1.,0.,0.));
#108848=DIRECTION('center_axis',(0.,1.,2.22044604925031E-16));
#108849=DIRECTION('ref_axis',(0.973489193493256,-5.07889309786447E-17,0.22873301062997));
#108850=DIRECTION('',(0.,-1.,-2.22044604925031E-16));
#108851=DIRECTION('center_axis',(0.,1.,2.22044604925031E-16));
#108852=DIRECTION('ref_axis',(-1.,0.,0.));
#108853=DIRECTION('center_axis',(6.93889390390722E-18,1.,2.22049474265475E-16));
#108854=DIRECTION('ref_axis',(-1.,6.93889390390721E-18,1.83750175990302E-19));
#108855=DIRECTION('center_axis',(6.93889390390723E-18,1.,2.22049474265475E-16));
#108856=DIRECTION('ref_axis',(0.,0.,1.));
#108857=DIRECTION('center_axis',(-6.93889390390723E-18,-1.,-2.22049474265475E-16));
#108858=DIRECTION('ref_axis',(0.33866857591881,-2.08550719155025E-16,0.940905731561417));
#108859=DIRECTION('center_axis',(6.93889390390723E-18,1.,2.22049474265475E-16));
#108860=DIRECTION('ref_axis',(0.33866857591881,-2.11277608343473E-16,0.940905731561417));
#108861=DIRECTION('center_axis',(-0.17934429547033,0.,0.983786370957766));
#108862=DIRECTION('ref_axis',(0.,-1.,0.));
#108863=DIRECTION('center_axis',(6.93889390390723E-18,1.,2.22049474265475E-16));
#108864=DIRECTION('ref_axis',(0.865342368165252,1.15648231731787E-16,-0.50118119064681));
#108865=DIRECTION('center_axis',(-6.93889390390723E-18,-1.,-2.22049474265475E-16));
#108866=DIRECTION('ref_axis',(0.,0.,-1.));
#108867=DIRECTION('center_axis',(-0.939530312300397,0.,0.342465753424658));
#108868=DIRECTION('ref_axis',(0.,-1.,0.));
#108869=DIRECTION('center_axis',(6.93889390390723E-18,1.,2.22049474265475E-16));
#108870=DIRECTION('ref_axis',(0.764334265490702,-1.34922937020418E-16,0.644820231224787));
#108871=DIRECTION('center_axis',(6.93889390390723E-18,1.,2.22049474265475E-16));
#108872=DIRECTION('ref_axis',(0.,0.,1.));
#108873=DIRECTION('center_axis',(6.93889390390723E-18,1.,2.22049474265475E-16));
#108874=DIRECTION('ref_axis',(-0.819288030372914,1.33004164137626E-16,-0.573382179080996));
#108875=DIRECTION('center_axis',(0.,0.,1.));
#108876=DIRECTION('ref_axis',(0.,-1.,0.));
#108877=DIRECTION('center_axis',(-6.93889390390723E-18,-1.,-2.22049474265475E-16));
#108878=DIRECTION('ref_axis',(-0.819288030372914,1.31276371155002E-16,-0.573382179080996));
#108879=DIRECTION('center_axis',(6.93889390390723E-18,1.,2.22049474265475E-16));
#108880=DIRECTION('ref_axis',(-1.,6.93889390390723E-18,1.83750175990302E-19));
#108881=DIRECTION('center_axis',(-6.93889390390723E-18,-1.,-2.22049474265475E-16));
#108882=DIRECTION('ref_axis',(-0.816812386473668,1.33768869693028E-16,-0.576903393388521));
#108883=DIRECTION('center_axis',(-6.93889390390723E-18,-1.,-2.22049474265475E-16));
#108884=DIRECTION('ref_axis',(-0.983881728593356,4.65340321282978E-17,-0.178820424281317));
#108885=DIRECTION('',(-2.04853783127104E-16,2.22049474265475E-16,-1.));
#108886=DIRECTION('center_axis',(-6.93889390390723E-18,-1.,-2.22049474265475E-16));
#108887=DIRECTION('ref_axis',(-0.707106781186547,-1.52106150078638E-16,
0.707106781186548));
#108888=DIRECTION('',(-1.,6.93889390390728E-18,-2.40389762145677E-16));
#108889=DIRECTION('center_axis',(-6.93889390390723E-18,-1.,-2.22049474265475E-16));
#108890=DIRECTION('ref_axis',(0.707106781186547,-1.61919227945412E-16,0.707106781186548));
#108891=DIRECTION('',(-2.41949676183277E-16,-2.22049474265475E-16,1.));
#108892=DIRECTION('center_axis',(-2.41949676183277E-16,-2.22049474265475E-16,
1.));
#108893=DIRECTION('ref_axis',(0.707106781186548,-0.707106781186548,0.));
#108894=DIRECTION('center_axis',(0.,0.,1.));
#108895=DIRECTION('ref_axis',(0.,-1.,0.));
#108896=DIRECTION('',(2.41949676183277E-16,2.22049474265475E-16,-1.));
#108897=DIRECTION('center_axis',(-1.,0.,0.));
#108898=DIRECTION('ref_axis',(0.,-1.,0.));
#108899=DIRECTION('center_axis',(6.93889390390723E-18,1.,2.22049474265475E-16));
#108900=DIRECTION('ref_axis',(0.707106781186547,-1.15648231731787E-16,0.707106781186548));
#108901=DIRECTION('center_axis',(-1.,6.93889390390728E-18,-2.40389762145677E-16));
#108902=DIRECTION('ref_axis',(0.,-0.707106781186548,0.707106781186548));
#108903=DIRECTION('center_axis',(-1.,0.,0.));
#108904=DIRECTION('ref_axis',(0.,-1.,0.));
#108905=DIRECTION('',(1.,-6.93889390390728E-18,2.40389762145677E-16));
#108906=DIRECTION('center_axis',(0.,0.,-1.));
#108907=DIRECTION('ref_axis',(0.,-1.,0.));
#108908=DIRECTION('center_axis',(6.93889390390723E-18,1.,2.22049474265475E-16));
#108909=DIRECTION('ref_axis',(-0.707106781186547,-1.15648231731787E-16,
0.707106781186548));
#108910=DIRECTION('center_axis',(-2.04853783127104E-16,2.22049474265475E-16,
-1.));
#108911=DIRECTION('ref_axis',(-0.707106781186547,-0.707106781186548,0.));
#108912=DIRECTION('center_axis',(0.,0.,-1.));
#108913=DIRECTION('ref_axis',(0.,-1.,0.));
#108914=DIRECTION('',(2.04853783127104E-16,-2.22049474265475E-16,1.));
#108915=DIRECTION('center_axis',(0.351876296299398,0.,-0.9360465117197));
#108916=DIRECTION('ref_axis',(0.,-1.,0.));
#108917=DIRECTION('center_axis',(6.93889390390723E-18,1.,2.22049474265475E-16));
#108918=DIRECTION('ref_axis',(-0.983881728593356,0.,-0.178820424281317));
#108919=DIRECTION('center_axis',(6.93889390390723E-18,1.,2.22049474265475E-16));
#108920=DIRECTION('ref_axis',(0.,-3.86164530304402E-16,1.));
#108921=DIRECTION('center_axis',(6.93889390390723E-18,1.,2.22049474265475E-16));
#108922=DIRECTION('ref_axis',(-0.816812386473668,1.35760967685141E-16,-0.576903393388521));
#108923=DIRECTION('center_axis',(0.,1.,0.));
#108924=DIRECTION('ref_axis',(-0.983786370957765,0.,-0.179344295470333));
#108925=DIRECTION('',(0.,1.,0.));
#108926=DIRECTION('center_axis',(0.,1.,2.22044604925031E-16));
#108927=DIRECTION('ref_axis',(-0.983786370957765,0.,-0.179344295470333));
#108928=DIRECTION('',(0.,-1.,0.));
#108929=DIRECTION('center_axis',(0.,-1.,-2.39272203583008E-16));
#108930=DIRECTION('ref_axis',(0.342465753424657,-2.24803488157148E-16,0.939530312300397));
#108931=DIRECTION('',(0.,-1.,-2.39272203583008E-16));
#108932=DIRECTION('center_axis',(0.,1.,2.22044604925031E-16));
#108933=DIRECTION('ref_axis',(0.342465753424657,-2.24803488157148E-16,0.939530312300397));
#108934=DIRECTION('center_axis',(0.,-1.,-2.39272203583008E-16));
#108935=DIRECTION('ref_axis',(-0.342465753424657,2.24803488157148E-16,-0.939530312300397));
#108936=DIRECTION('',(0.,-1.,-2.39272203583008E-16));
#108937=DIRECTION('center_axis',(0.,-1.,-2.22044604925031E-16));
#108938=DIRECTION('ref_axis',(-0.342465753424657,2.24803488157148E-16,-0.939530312300397));
#108939=DIRECTION('center_axis',(1.,-5.78918321765678E-32,2.41949676183277E-16));
#108940=DIRECTION('ref_axis',(-2.41949676183277E-16,-2.22049474265475E-16,
1.));
#108941=DIRECTION('',(3.24194260188779E-33,-1.,-2.52671446983656E-16));
#108942=DIRECTION('',(2.41949676183277E-16,2.22044604925031E-16,-1.));
#108943=DIRECTION('center_axis',(-3.24194260188779E-33,1.,2.52671446983656E-16));
#108944=DIRECTION('ref_axis',(0.707106781186548,0.,0.707106781186548));
#108945=DIRECTION('',(-3.24194260188779E-33,1.,2.52671446983656E-16));
#108946=DIRECTION('center_axis',(0.,-1.,-2.22044604925031E-16));
#108947=DIRECTION('ref_axis',(0.707106781186548,0.,0.707106781186548));
#108948=DIRECTION('center_axis',(-2.40389762145677E-16,-2.52671446983656E-16,
1.));
#108949=DIRECTION('ref_axis',(-1.,-6.93889390390718E-18,-2.40389762145677E-16));
#108950=DIRECTION('',(4.78544407166016E-17,-1.,-2.52671446983656E-16));
#108951=DIRECTION('',(1.,-5.3377249763659E-32,2.40389762145677E-16));
#108952=DIRECTION('center_axis',(-4.78544407166016E-17,1.,2.52671446983656E-16));
#108953=DIRECTION('ref_axis',(-0.707106781186548,0.,0.707106781186547));
#108954=DIRECTION('',(-4.78544407166016E-17,1.,2.52671446983656E-16));
#108955=DIRECTION('center_axis',(0.,1.,2.22044604925031E-16));
#108956=DIRECTION('ref_axis',(-0.707106781186548,0.,0.707106781186547));
#108957=DIRECTION('center_axis',(1.,4.78544407166016E-17,-2.04853783127104E-16));
#108958=DIRECTION('ref_axis',(2.04853783127104E-16,-2.28983498828938E-16,
1.));
#108959=DIRECTION('',(4.78544407166015E-17,-1.,-3.49344973759647E-16));
#108960=DIRECTION('',(-2.04853783127104E-16,2.22044604925031E-16,-1.));
#108961=DIRECTION('center_axis',(-4.78544407166016E-17,1.,3.49344973759647E-16));
#108962=DIRECTION('ref_axis',(-0.983881728593356,0.,-0.178820424281317));
#108963=DIRECTION('',(0.,1.,2.22044604925031E-16));
#108964=DIRECTION('center_axis',(0.,1.,2.22044604925031E-16));
#108965=DIRECTION('ref_axis',(-0.983881728593356,0.,-0.178820424281317));
#108966=DIRECTION('center_axis',(0.,1.,2.22044604925031E-16));
#108967=DIRECTION('ref_axis',(0.17741935483871,2.18521943337466E-16,-0.98413534258689));
#108968=DIRECTION('center_axis',(0.,-1.,-2.22044604925031E-16));
#108969=DIRECTION('ref_axis',(-0.994623655913978,-2.29939845948218E-17,
0.103555700453002));
#108970=DIRECTION('',(0.,1.,2.22044604925031E-16));
#108971=DIRECTION('center_axis',(0.,1.,2.22044604925031E-16));
#108972=DIRECTION('ref_axis',(0.17741935483871,2.18521943337466E-16,-0.98413534258689));
#108973=DIRECTION('',(0.,1.,2.22044604925031E-16));
#108974=DIRECTION('center_axis',(1.51594548245566E-16,-0.819152044288998,
0.573576436351038));
#108975=DIRECTION('ref_axis',(-1.9770466526922E-16,-0.573576436351038,-0.819152044288998));
#108976=DIRECTION('',(0.,1.,2.22044604925031E-16));
#108977=DIRECTION('center_axis',(0.,-1.,-2.22044604925031E-16));
#108978=DIRECTION('ref_axis',(0.17741935483871,2.18521943337466E-16,-0.98413534258689));
#108979=DIRECTION('center_axis',(1.,0.,0.));
#108980=DIRECTION('ref_axis',(0.,-1.,0.));
#108981=DIRECTION('center_axis',(6.93889390390723E-18,1.,2.22049474265475E-16));
#108982=DIRECTION('ref_axis',(0.,0.,1.));
#108983=DIRECTION('center_axis',(-0.563542669426771,0.,-0.826086956521739));
#108984=DIRECTION('ref_axis',(0.826086956521739,0.,-0.563542669426771));
#108985=DIRECTION('center_axis',(6.93889390390723E-18,1.,2.22049474265475E-16));
#108986=DIRECTION('ref_axis',(-0.462172675917159,-1.93704275295193E-16,
0.886789951248644));
#108987=DIRECTION('center_axis',(0.999936821691632,0.,-0.0112406683625832));
#108988=DIRECTION('ref_axis',(0.,-1.,0.));
#108989=DIRECTION('center_axis',(-6.93889390390723E-18,-1.,-2.22049474265475E-16));
#108990=DIRECTION('ref_axis',(-0.462172675917159,-1.98254111540207E-16,
0.886789951248644));
#108991=DIRECTION('center_axis',(-0.707106781186548,0.,0.707106781186548));
#108992=DIRECTION('ref_axis',(0.,-1.,0.));
#108993=DIRECTION('center_axis',(6.93889390390723E-18,1.,2.22049474265475E-16));
#108994=DIRECTION('ref_axis',(0.921714097362088,8.67361737988403E-17,-0.387869981725824));
#108995=DIRECTION('center_axis',(-6.93889390390723E-18,-1.,-2.22049474265475E-16));
#108996=DIRECTION('ref_axis',(0.921714097362088,7.97306491942474E-17,-0.387869981725824));
#108997=DIRECTION('center_axis',(-0.707106781186548,-1.52106150078638E-16,
0.707106781186547));
#108998=DIRECTION('ref_axis',(0.500000000000002,-0.707106781186548,0.499999999999998));
#108999=DIRECTION('center_axis',(-0.707106781186549,0.,0.707106781186546));
#109000=DIRECTION('ref_axis',(0.,-1.,0.));
#109001=DIRECTION('',(0.707106781186548,1.52106150078638E-16,-0.707106781186547));
#109002=DIRECTION('',(-0.707106781186548,-1.52106150078638E-16,0.707106781186547));
#109003=DIRECTION('center_axis',(6.93889390390723E-18,1.,2.22049474265475E-16));
#109004=DIRECTION('ref_axis',(0.,0.,1.));
#109005=DIRECTION('center_axis',(1.88182802673964E-12,0.,1.));
#109006=DIRECTION('ref_axis',(0.,-1.,0.));
#109007=DIRECTION('center_axis',(-6.93889390390723E-18,-1.,-2.22049474265475E-16));
#109008=DIRECTION('ref_axis',(-0.923879532511647,8.67361737988402E-17,-0.38268343236422));
#109009=DIRECTION('center_axis',(6.93889390390723E-18,1.,2.22049474265475E-16));
#109010=DIRECTION('ref_axis',(-0.923879532511647,9.13853570226723E-17,-0.38268343236422));
#109011=DIRECTION('center_axis',(1.88212241265405E-12,-2.22049474265488E-16,
1.));
#109012=DIRECTION('ref_axis',(0.707106781186548,-0.707106781186548,-1.3306533587345E-12));
#109013=DIRECTION('center_axis',(1.88182802673964E-12,0.,1.));
#109014=DIRECTION('ref_axis',(0.,-1.,0.));
#109015=DIRECTION('',(-1.88212241265405E-12,2.22049474265488E-16,-1.));
#109016=DIRECTION('',(1.88212241265405E-12,-2.22049474265488E-16,1.));
#109017=DIRECTION('center_axis',(-0.989426754293278,0.,-0.14503343714009));
#109018=DIRECTION('ref_axis',(0.,-1.,0.));
#109019=DIRECTION('center_axis',(6.93889390390723E-18,1.,2.22049474265475E-16));
#109020=DIRECTION('ref_axis',(0.653822056396758,-1.73472347597681E-16,0.756648345381865));
#109021=DIRECTION('center_axis',(-6.93889390390723E-18,-1.,-2.22049474265475E-16));
#109022=DIRECTION('ref_axis',(0.653822056396758,-1.72550169177256E-16,0.756648345381865));
#109023=DIRECTION('center_axis',(6.93889390390723E-18,1.,2.22049474265475E-16));
#109024=DIRECTION('ref_axis',(0.,0.,1.));
#109025=DIRECTION('center_axis',(0.89959196856447,0.,0.436731370632225));
#109026=DIRECTION('ref_axis',(-0.436731370632225,0.,0.89959196856447));
#109027=DIRECTION('center_axis',(6.93889390390723E-18,1.,2.22049474265475E-16));
#109028=DIRECTION('ref_axis',(0.327915980784702,2.07496294239519E-16,-0.944706890811116));
#109029=DIRECTION('center_axis',(-0.976712922996695,0.,-0.214550381149164));
#109030=DIRECTION('ref_axis',(0.,-1.,0.));
#109031=DIRECTION('center_axis',(-6.93889390390723E-18,-1.,-2.22049474265475E-16));
#109032=DIRECTION('ref_axis',(0.327915980784702,2.06949467309514E-16,-0.944706890811116));
#109033=DIRECTION('center_axis',(0.55230501554796,0.,-0.833642111340693));
#109034=DIRECTION('ref_axis',(0.,-1.,0.));
#109035=DIRECTION('center_axis',(6.93889390390723E-18,1.,2.22049474265475E-16));
#109036=DIRECTION('ref_axis',(-0.926903899779186,-1.15648231731787E-16,
0.375298761754069));
#109037=DIRECTION('center_axis',(-6.93889390390723E-18,-1.,-2.22049474265475E-16));
#109038=DIRECTION('ref_axis',(-0.926903899779186,-7.69032049202891E-17,
0.375298761754069));
#109039=DIRECTION('center_axis',(6.93889390390723E-18,1.,2.22049474265475E-16));
#109040=DIRECTION('ref_axis',(0.,0.,1.));
#109041=DIRECTION('center_axis',(0.,0.,-1.));
#109042=DIRECTION('ref_axis',(0.,-1.,0.));
#109043=DIRECTION('center_axis',(-6.93889390390723E-18,-1.,-2.22049474265475E-16));
#109044=DIRECTION('ref_axis',(0.957507731389333,-5.78241158658936E-17,0.288407601026141));
#109045=DIRECTION('center_axis',(6.93889390390723E-18,1.,2.22049474265475E-16));
#109046=DIRECTION('ref_axis',(0.957507731389333,-7.06848007423029E-17,0.288407601026141));
#109047=DIRECTION('center_axis',(0.,2.22049474265475E-16,-1.));
#109048=DIRECTION('ref_axis',(-0.707106781186548,-0.707106781186548,0.));
#109049=DIRECTION('center_axis',(0.,0.,-1.));
#109050=DIRECTION('ref_axis',(0.,-1.,0.));
#109051=DIRECTION('',(0.,-2.22049474265475E-16,1.));
#109052=DIRECTION('',(0.,2.22049474265475E-16,-1.));
#109053=DIRECTION('center_axis',(-6.93889390390723E-18,-1.,-2.22049474265475E-16));
#109054=DIRECTION('ref_axis',(0.,0.,-1.));
#109055=DIRECTION('center_axis',(6.93889390390723E-18,1.,2.22049474265475E-16));
#109056=DIRECTION('ref_axis',(-0.294329993497647,-2.16418819656757E-16,
0.955703853151003));
#109057=DIRECTION('center_axis',(-6.93889390390723E-18,-1.,-2.22049474265475E-16));
#109058=DIRECTION('ref_axis',(-0.294329993497647,-2.10171213548051E-16,
0.955703853151004));
#109059=DIRECTION('center_axis',(-0.988716140908567,0.130504856475735,0.0735450551914906));
#109060=DIRECTION('ref_axis',(-0.149801177254627,-0.861356769214109,-0.485411293051738));
#109061=DIRECTION('center_axis',(0.,1.,0.));
#109062=DIRECTION('ref_axis',(-0.294883912309791,0.,-0.95553308590591));
#109063=DIRECTION('center_axis',(-0.707106781186547,0.,-0.707106781186548));
#109064=DIRECTION('ref_axis',(-0.707106781186548,-1.57009245868377E-16,
0.707106781186547));
#109065=DIRECTION('',(0.,-1.,0.));
#109066=DIRECTION('',(-0.707106781186548,-1.57009245868377E-16,0.707106781186547));
#109067=DIRECTION('',(0.,1.,0.));
#109068=DIRECTION('center_axis',(0.,1.,0.));
#109069=DIRECTION('ref_axis',(-0.923879532511647,0.,-0.38268343236422));
#109070=DIRECTION('',(0.,1.,0.));
#109071=DIRECTION('center_axis',(0.,-1.,-2.22044604925031E-16));
#109072=DIRECTION('ref_axis',(-0.923879532511647,0.,-0.38268343236422));
#109073=DIRECTION('center_axis',(-1.,-5.22393909422894E-28,1.88212241265405E-12));
#109074=DIRECTION('ref_axis',(1.88212241265405E-12,-2.22044604925031E-16,
1.));
#109075=DIRECTION('',(0.,-1.,0.));
#109076=DIRECTION('',(1.88215207428297E-12,-2.22044604925031E-16,1.));
#109077=DIRECTION('center_axis',(0.,-1.,0.));
#109078=DIRECTION('ref_axis',(0.653822056396758,0.,0.756648345381865));
#109079=DIRECTION('',(0.,1.,0.));
#109080=DIRECTION('center_axis',(0.,1.,2.22044604925031E-16));
#109081=DIRECTION('ref_axis',(0.653822056396758,0.,0.756648345381865));
#109082=DIRECTION('center_axis',(0.,-1.,0.));
#109083=DIRECTION('ref_axis',(-0.436731370632224,0.,0.899591968564471));
#109084=DIRECTION('',(0.,-1.,0.));
#109085=DIRECTION('center_axis',(0.,-1.,-2.22044604925031E-16));
#109086=DIRECTION('ref_axis',(-0.436731370632224,0.,0.899591968564471));
#109087=DIRECTION('center_axis',(0.,-1.,0.));
#109088=DIRECTION('ref_axis',(0.436731370632225,0.,-0.89959196856447));
#109089=DIRECTION('',(0.,-1.,0.));
#109090=DIRECTION('center_axis',(0.,1.,2.22044604925031E-16));
#109091=DIRECTION('ref_axis',(0.436731370632225,0.,-0.89959196856447));
#109092=DIRECTION('center_axis',(6.93889390390723E-18,1.,2.22049474265475E-16));
#109093=DIRECTION('ref_axis',(-1.,6.93889390390723E-18,1.83750175990302E-19));
#109094=DIRECTION('center_axis',(1.65636802248512E-16,-2.22049474265475E-16,
1.));
#109095=DIRECTION('ref_axis',(0.707106781186548,-0.707106781186548,-2.4532694666934E-16));
#109096=DIRECTION('center_axis',(0.,0.,-1.));
#109097=DIRECTION('ref_axis',(1.,0.,0.));
#109098=DIRECTION('',(1.65636802248512E-16,-2.22049474265475E-16,1.));
#109099=DIRECTION('center_axis',(0.,0.,1.));
#109100=DIRECTION('ref_axis',(0.,-1.,0.));
#109101=DIRECTION('',(-1.65636802248512E-16,2.22049474265475E-16,-1.));
#109102=DIRECTION('center_axis',(-1.,0.,0.));
#109103=DIRECTION('ref_axis',(0.,-1.,0.));
#109104=DIRECTION('center_axis',(6.93889390390723E-18,1.,2.22049474265475E-16));
#109105=DIRECTION('ref_axis',(0.707106781186547,-1.15648231731787E-16,0.707106781186548));
#109106=DIRECTION('center_axis',(-6.93889390390723E-18,-1.,-2.22049474265475E-16));
#109107=DIRECTION('ref_axis',(0.707106781186547,-1.61919227945412E-16,0.707106781186548));
#109108=DIRECTION('center_axis',(-1.,6.93889390390724E-18,-6.93889390390729E-17));
#109109=DIRECTION('ref_axis',(0.,-0.707106781186548,0.707106781186548));
#109110=DIRECTION('center_axis',(-1.,0.,0.));
#109111=DIRECTION('ref_axis',(0.,-1.,0.));
#109112=DIRECTION('',(1.,-6.93889390390724E-18,6.93889390390729E-17));
#109113=DIRECTION('',(-1.,6.93889390390724E-18,-6.93889390390729E-17));
#109114=DIRECTION('center_axis',(6.93889390390723E-18,1.,2.22049474265475E-16));
#109115=DIRECTION('ref_axis',(0.,0.,1.));
#109116=DIRECTION('center_axis',(-0.914646181285313,0.,0.40425531914892));
#109117=DIRECTION('ref_axis',(0.,-1.,0.));
#109118=DIRECTION('center_axis',(-6.93889390390723E-18,-1.,-2.22049474265475E-16));
#109119=DIRECTION('ref_axis',(-0.206583903916408,2.20013709148278E-16,-0.978428888904379));
#109120=DIRECTION('center_axis',(6.93889390390723E-18,1.,2.22049474265475E-16));
#109121=DIRECTION('ref_axis',(-0.206583903916408,2.18693084178901E-16,-0.978428888904378));
#109122=DIRECTION('center_axis',(1.66533453693774E-14,0.,-1.));
#109123=DIRECTION('ref_axis',(0.,-1.,0.));
#109124=DIRECTION('center_axis',(6.93889390390723E-18,1.,2.22049474265475E-16));
#109125=DIRECTION('ref_axis',(-0.54577682290983,-2.31296463463574E-16,0.837930581596383));
#109126=DIRECTION('center_axis',(-6.93889390390723E-18,-1.,-2.22049474265475E-16));
#109127=DIRECTION('ref_axis',(-0.54577682290983,-1.82274957645058E-16,0.837930581596383));
#109128=DIRECTION('center_axis',(1.88016196282748E-14,2.22049474265475E-16,
-1.));
#109129=DIRECTION('ref_axis',(-0.707106781186548,-0.707106781186548,-1.3738309013483E-14));
#109130=DIRECTION('center_axis',(1.94289029309402E-14,0.,-1.));
#109131=DIRECTION('ref_axis',(0.,-1.,0.));
#109132=DIRECTION('',(-1.88016196282748E-14,-2.22049474265475E-16,1.));
#109133=DIRECTION('',(1.88016196282748E-14,2.22049474265475E-16,-1.));
#109134=DIRECTION('center_axis',(6.93889390390723E-18,1.,2.22049474265475E-16));
#109135=DIRECTION('ref_axis',(0.,-4.13106241720989E-16,1.));
#109136=DIRECTION('center_axis',(-0.567316408958496,0.,-0.823499904144765));
#109137=DIRECTION('ref_axis',(0.,-1.,0.));
#109138=DIRECTION('center_axis',(-6.93889390390723E-18,-1.,-2.22049474265475E-16));
#109139=DIRECTION('ref_axis',(0.95485598499061,5.33761069531325E-17,-0.297069096217718));
#109140=DIRECTION('center_axis',(6.93889390390723E-18,1.,2.22049474265475E-16));
#109141=DIRECTION('ref_axis',(0.95485598499061,5.93383922623034E-17,-0.297069096217718));
#109142=DIRECTION('center_axis',(0.994393511593655,0.,0.105742820562149));
#109143=DIRECTION('ref_axis',(0.,-1.,0.));
#109144=DIRECTION('center_axis',(6.93889390390723E-18,1.,2.22049474265475E-16));
#109145=DIRECTION('ref_axis',(-0.859376679196035,1.15648231731787E-16,-0.511343058282788));
#109146=DIRECTION('center_axis',(-6.93889390390723E-18,-1.,-2.22049474265475E-16));
#109147=DIRECTION('ref_axis',(-0.859376679196035,1.19506580861427E-16,-0.511343058282788));
#109148=DIRECTION('center_axis',(6.93889390390723E-18,1.,2.22049474265475E-16));
#109149=DIRECTION('ref_axis',(0.,-1.78573536624128E-16,1.));
#109150=DIRECTION('center_axis',(0.999122256992311,0.,-0.0418893254014727));
#109151=DIRECTION('ref_axis',(0.,-1.,0.));
#109152=DIRECTION('center_axis',(-6.93889390390723E-18,-1.,-2.22049474265475E-16));
#109153=DIRECTION('ref_axis',(-0.0320141760681106,-2.21667125556843E-16,
0.999487414893594));
#109154=DIRECTION('center_axis',(6.93889390390723E-18,1.,2.22049474265475E-16));
#109155=DIRECTION('ref_axis',(-0.0320141760681106,-2.21713512040924E-16,
0.999487414893594));
#109156=DIRECTION('center_axis',(0.707106781186548,0.,0.707106781186547));
#109157=DIRECTION('ref_axis',(0.,-1.,0.));
#109158=DIRECTION('center_axis',(6.93889390390723E-18,1.,2.22049474265475E-16));
#109159=DIRECTION('ref_axis',(0.363244855982583,1.73472347597681E-16,-0.931693712870379));
#109160=DIRECTION('center_axis',(-6.93889390390723E-18,-1.,-2.22049474265475E-16));
#109161=DIRECTION('ref_axis',(0.363244855982583,2.04361581602513E-16,-0.931693712870379));
#109162=DIRECTION('center_axis',(0.707106781186547,-1.61919227945412E-16,
0.707106781186548));
#109163=DIRECTION('ref_axis',(0.500000000000001,-0.707106781186547,-0.499999999999999));
#109164=DIRECTION('center_axis',(0.707106781186552,0.,0.707106781186543));
#109165=DIRECTION('ref_axis',(0.,-1.,0.));
#109166=DIRECTION('',(-0.707106781186547,1.61919227945412E-16,-0.707106781186548));
#109167=DIRECTION('',(0.707106781186547,-1.61919227945412E-16,0.707106781186548));
#109168=DIRECTION('center_axis',(6.93889390390723E-18,1.,2.22049474265475E-16));
#109169=DIRECTION('ref_axis',(0.923879532511287,8.67361737988403E-17,-0.38268343236509));
#109170=DIRECTION('center_axis',(-6.93889390390723E-18,-1.,-2.22049474265475E-16));
#109171=DIRECTION('ref_axis',(0.923879532511287,7.85639529106883E-17,-0.38268343236509));
#109172=DIRECTION('center_axis',(0.,-1.,0.));
#109173=DIRECTION('ref_axis',(-0.859376679196034,0.,-0.51134305828279));
#109174=DIRECTION('',(0.,1.,0.));
#109175=DIRECTION('center_axis',(0.,1.,2.22044604925031E-16));
#109176=DIRECTION('ref_axis',(-0.859376679196034,0.,-0.51134305828279));
#109177=DIRECTION('',(0.,-1.,-2.22044604925031E-16));
#109178=DIRECTION('center_axis',(0.,-1.,0.));
#109179=DIRECTION('ref_axis',(-0.28378257126716,0.,0.958888654769155));
#109180=DIRECTION('',(0.,-1.,0.));
#109181=DIRECTION('center_axis',(0.,1.,2.22044604925031E-16));
#109182=DIRECTION('ref_axis',(-0.28378257126716,0.,0.958888654769155));
#109183=DIRECTION('center_axis',(0.,1.,0.));
#109184=DIRECTION('ref_axis',(0.363244855982583,0.,-0.931693712870379));
#109185=DIRECTION('',(0.,1.,0.));
#109186=DIRECTION('center_axis',(0.,1.,2.22044604925031E-16));
#109187=DIRECTION('ref_axis',(0.363244855982583,0.,-0.931693712870379));
#109188=DIRECTION('center_axis',(-0.707106781186548,0.,0.707106781186547));
#109189=DIRECTION('ref_axis',(0.707106781186547,-1.57009245868378E-16,0.707106781186548));
#109190=DIRECTION('',(0.,-1.,0.));
#109191=DIRECTION('',(0.707106781186547,-1.57009245868378E-16,0.707106781186548));
#109192=DIRECTION('center_axis',(0.,-1.,0.));
#109193=DIRECTION('ref_axis',(0.923879532511287,0.,-0.382683432365089));
#109194=DIRECTION('',(0.,1.,0.));
#109195=DIRECTION('center_axis',(0.,1.,2.22044604925031E-16));
#109196=DIRECTION('ref_axis',(0.923879532511287,0.,-0.382683432365089));
#109197=DIRECTION('center_axis',(1.,0.,-1.65636802248512E-16));
#109198=DIRECTION('ref_axis',(1.65636802248512E-16,-2.28983498828938E-16,
1.));
#109199=DIRECTION('',(0.,-1.,0.));
#109200=DIRECTION('',(1.65636802248512E-16,-2.22044604925031E-16,1.));
#109201=DIRECTION('center_axis',(6.93889390390723E-18,1.,2.22049474265475E-16));
#109202=DIRECTION('ref_axis',(-1.,6.93889390390723E-18,1.83750175990302E-19));
#109203=DIRECTION('center_axis',(-2.04853783127104E-16,2.22049474265475E-16,
-1.));
#109204=DIRECTION('ref_axis',(-0.707106781186547,-0.707106781186548,0.));
#109205=DIRECTION('center_axis',(-3.79470760369927E-16,0.,1.));
#109206=DIRECTION('ref_axis',(-1.,0.,-3.79470760369927E-16));
#109207=DIRECTION('',(-2.04853783127104E-16,2.22049474265475E-16,-1.));
#109208=DIRECTION('center_axis',(0.,0.,-1.));
#109209=DIRECTION('ref_axis',(0.,-1.,0.));
#109210=DIRECTION('',(2.04853783127104E-16,-2.22049474265475E-16,1.));
#109211=DIRECTION('center_axis',(1.,0.,3.46944695195362E-16));
#109212=DIRECTION('ref_axis',(0.,-1.,0.));
#109213=DIRECTION('center_axis',(6.93889390390723E-18,1.,2.22049474265475E-16));
#109214=DIRECTION('ref_axis',(-0.707106781186547,1.15648231731787E-16,-0.707106781186548));
#109215=DIRECTION('center_axis',(-6.93889390390723E-18,-1.,-2.22049474265475E-16));
#109216=DIRECTION('ref_axis',(-0.707106781186547,1.61919227945412E-16,-0.707106781186548));
#109217=DIRECTION('center_axis',(1.,-6.93889390390728E-18,2.40389762145677E-16));
#109218=DIRECTION('ref_axis',(0.,-0.707106781186548,-0.707106781186547));
#109219=DIRECTION('center_axis',(1.,0.,1.38777878078145E-15));
#109220=DIRECTION('ref_axis',(0.,-1.,0.));
#109221=DIRECTION('',(-1.,6.93889390390728E-18,-2.40389762145677E-16));
#109222=DIRECTION('',(1.,-6.93889390390728E-18,2.40389762145677E-16));
#109223=DIRECTION('center_axis',(0.,0.,1.));
#109224=DIRECTION('ref_axis',(0.,-1.,0.));
#109225=DIRECTION('center_axis',(6.93889390390723E-18,1.,2.22049474265475E-16));
#109226=DIRECTION('ref_axis',(0.707106781186548,1.15648231731787E-16,-0.707106781186547));
#109227=DIRECTION('center_axis',(-6.93889390390723E-18,-1.,-2.22049474265475E-16));
#109228=DIRECTION('ref_axis',(0.707106781186548,1.52106150078638E-16,-0.707106781186547));
#109229=DIRECTION('center_axis',(-2.41949676183277E-16,-2.22049474265475E-16,
1.));
#109230=DIRECTION('ref_axis',(0.707106781186548,-0.707106781186548,0.));
#109231=DIRECTION('center_axis',(0.,0.,1.));
#109232=DIRECTION('ref_axis',(0.,-1.,0.));
#109233=DIRECTION('',(2.41949676183277E-16,2.22049474265475E-16,-1.));
#109234=DIRECTION('',(-2.41949676183277E-16,-2.22049474265475E-16,1.));
#109235=DIRECTION('center_axis',(6.93889390390723E-18,1.,2.22049474265475E-16));
#109236=DIRECTION('ref_axis',(0.,0.,1.));
#109237=DIRECTION('center_axis',(0.970096776450229,0.,0.242718446601972));
#109238=DIRECTION('ref_axis',(0.,-1.,0.));
#109239=DIRECTION('center_axis',(-6.93889390390723E-18,-1.,-2.22049474265475E-16));
#109240=DIRECTION('ref_axis',(-0.788263422531444,-1.31276371155002E-16,
0.615337936989922));
#109241=DIRECTION('center_axis',(6.93889390390723E-18,1.,2.22049474265475E-16));
#109242=DIRECTION('ref_axis',(-0.788263422531444,-1.31165789146938E-16,
0.615337936989922));
#109243=DIRECTION('center_axis',(-6.93889390390723E-18,-1.,-2.22049474265475E-16));
#109244=DIRECTION('ref_axis',(0.,0.,-1.));
#109245=DIRECTION('center_axis',(0.442477646994526,0.,0.896779533614694));
#109246=DIRECTION('ref_axis',(0.,-1.,0.));
#109247=DIRECTION('center_axis',(6.93889390390723E-18,1.,2.22049474265475E-16));
#109248=DIRECTION('ref_axis',(0.627860970415715,1.6821560979169E-16,-0.77832551148516));
#109249=DIRECTION('center_axis',(-6.93889390390723E-18,-1.,-2.22049474265475E-16));
#109250=DIRECTION('ref_axis',(0.627860970415715,1.68470109972568E-16,-0.77832551148516));
#109251=DIRECTION('center_axis',(-0.98636834994651,0.,-0.164552357089771));
#109252=DIRECTION('ref_axis',(0.,-1.,0.));
#109253=DIRECTION('center_axis',(6.93889390390723E-18,1.,2.22049474265475E-16));
#109254=DIRECTION('ref_axis',(0.802769817727363,-1.15648231731787E-16,0.596289040437585));
#109255=DIRECTION('center_axis',(-6.93889390390723E-18,-1.,-2.22049474265475E-16));
#109256=DIRECTION('ref_axis',(0.802769817727363,-1.37976002533899E-16,0.596289040437585));
#109257=DIRECTION('center_axis',(-6.93889390390723E-18,-1.,-2.22049474265475E-16));
#109258=DIRECTION('ref_axis',(0.,1.57234772945449E-16,-1.));
#109259=DIRECTION('center_axis',(-0.899591968564471,0.,-0.436731370632223));
#109260=DIRECTION('ref_axis',(0.,-1.,0.));
#109261=DIRECTION('center_axis',(6.93889390390723E-18,1.,2.22049474265475E-16));
#109262=DIRECTION('ref_axis',(-0.303756589059817,-2.08827432818175E-16,
0.952749670481573));
#109263=DIRECTION('center_axis',(-6.93889390390723E-18,-1.,-2.22049474265475E-16));
#109264=DIRECTION('ref_axis',(-0.303756589059817,-2.09449828692939E-16,
0.952749670481573));
#109265=DIRECTION('center_axis',(-6.93889390390723E-18,-1.,-2.22049474265475E-16));
#109266=DIRECTION('ref_axis',(0.,3.86164530304402E-16,-1.));
#109267=DIRECTION('center_axis',(-0.351876296299399,0.,-0.9360465117197));
#109268=DIRECTION('ref_axis',(0.,-1.,0.));
#109269=DIRECTION('center_axis',(6.93889390390723E-18,1.,2.22049474265475E-16));
#109270=DIRECTION('ref_axis',(-0.739004663706429,-1.43303243667649E-16,
0.673700309499815));
#109271=DIRECTION('center_axis',(-6.93889390390723E-18,-1.,-2.22049474265475E-16));
#109272=DIRECTION('ref_axis',(-0.739004663706429,-1.4446692458097E-16,0.673700309499816));
#109273=DIRECTION('center_axis',(6.93889390390723E-18,1.,2.22049474265475E-16));
#109274=DIRECTION('ref_axis',(-0.983881728593356,0.,0.178820424281317));
#109275=DIRECTION('center_axis',(-6.93889390390723E-18,-1.,-2.22049474265475E-16));
#109276=DIRECTION('ref_axis',(-0.983881728593356,-3.28799302708935E-17,
0.178820424281317));
#109277=DIRECTION('center_axis',(0.,-1.,-2.39272203583008E-16));
#109278=DIRECTION('ref_axis',(0.983984869082392,4.26507501169509E-17,-0.178252005365741));
#109279=DIRECTION('',(0.,-1.,-2.39272203583008E-16));
#109280=DIRECTION('center_axis',(0.,1.,2.22044604925031E-16));
#109281=DIRECTION('ref_axis',(0.983984869082392,4.26507501169509E-17,-0.178252005365741));
#109282=DIRECTION('',(0.,-1.,-2.39272203583008E-16));
#109283=DIRECTION('center_axis',(0.,1.,2.39272203583008E-16));
#109284=DIRECTION('ref_axis',(0.802769817727364,0.,0.596289040437585));
#109285=DIRECTION('',(0.,1.,2.22044604925031E-16));
#109286=DIRECTION('center_axis',(0.,1.,2.22044604925031E-16));
#109287=DIRECTION('ref_axis',(0.802769817727364,0.,0.596289040437585));
#109288=DIRECTION('center_axis',(0.,1.,2.22044604925031E-16));
#109289=DIRECTION('ref_axis',(-0.436731370632224,-1.99749543253629E-16,
0.89959196856447));
#109290=DIRECTION('',(0.,1.,3.21803775253669E-16));
#109291=DIRECTION('center_axis',(0.,-1.,-2.22044604925031E-16));
#109292=DIRECTION('ref_axis',(-0.436731370632224,-1.99749543253629E-16,
0.89959196856447));
#109293=DIRECTION('',(0.,1.,2.22044604925031E-16));
#109294=DIRECTION('center_axis',(0.,-1.,-2.22044604925031E-16));
#109295=DIRECTION('ref_axis',(-0.436731370632224,-1.99749543253629E-16,
0.89959196856447));
#109296=DIRECTION('center_axis',(0.,1.,2.22044604925031E-16));
#109297=DIRECTION('ref_axis',(0.17741935483871,2.18521943337466E-16,-0.98413534258689));
#109298=DIRECTION('',(0.,-1.,-2.22044604925031E-16));
#109299=DIRECTION('center_axis',(0.,1.,2.22044604925031E-16));
#109300=DIRECTION('ref_axis',(0.17741935483871,2.18521943337466E-16,-0.98413534258689));
#109301=DIRECTION('',(0.,-1.,-2.22044604925031E-16));
#109302=DIRECTION('center_axis',(1.00839335745948E-17,-0.819152044288994,
-0.573576436351042));
#109303=DIRECTION('ref_axis',(4.94261663173048E-17,0.573576436351042,-0.819152044288994));
#109304=DIRECTION('',(0.,-1.,-2.22044604925031E-16));
#109305=DIRECTION('center_axis',(0.,1.,2.22044604925031E-16));
#109306=DIRECTION('ref_axis',(0.17741935483871,2.18521943337466E-16,-0.98413534258689));
#109307=DIRECTION('center_axis',(-4.78544407166016E-17,1.,9.47442360904155E-17));
#109308=DIRECTION('ref_axis',(-0.983881728593356,0.,0.178820424281317));
#109309=DIRECTION('',(-4.78544407166016E-17,1.,9.47442360904155E-17));
#109310=DIRECTION('center_axis',(0.,1.,2.22044604925031E-16));
#109311=DIRECTION('ref_axis',(-0.983881728593356,0.,0.178820424281317));
#109312=DIRECTION('center_axis',(1.,4.78544407166016E-17,-2.04853783127104E-16));
#109313=DIRECTION('ref_axis',(2.04853783127104E-16,-2.28983498828938E-16,
1.));
#109314=DIRECTION('',(4.78544407166016E-17,-1.,-6.12536841172497E-17));
#109315=DIRECTION('',(-2.04853783127104E-16,2.22044604925031E-16,-1.));
#109316=DIRECTION('center_axis',(6.93889390390723E-18,1.,2.22049474265475E-16));
#109317=DIRECTION('ref_axis',(-1.,6.93889390390723E-18,1.83750175990302E-19));
#109318=DIRECTION('center_axis',(2.21497401043431E-17,-1.,-2.22049474265426E-16));
#109319=DIRECTION('ref_axis',(0.,2.85358528417711E-16,-1.));
#109320=DIRECTION('center_axis',(-2.21497401043431E-17,1.,2.22049474265426E-16));
#109321=DIRECTION('ref_axis',(-0.095969134594036,2.18898871406418E-16,-0.995384310306965));
#109322=DIRECTION('center_axis',(-0.981030928551421,0.,0.193851276048257));
#109323=DIRECTION('ref_axis',(0.,-1.,0.));
#109324=DIRECTION('center_axis',(2.21497401043431E-17,-1.,-2.22049474265426E-16));
#109325=DIRECTION('ref_axis',(-0.095969134594036,2.20376887935251E-16,-0.995384310306965));
#109326=DIRECTION('center_axis',(0.113781875054763,0.,-0.993505754844441));
#109327=DIRECTION('ref_axis',(0.,-1.,0.));
#109328=DIRECTION('center_axis',(-2.21497401043431E-17,1.,2.22049474265426E-16));
#109329=DIRECTION('ref_axis',(-0.677875792531132,-1.15648231731787E-16,
0.73517644814037));
#109330=DIRECTION('center_axis',(2.21497401043431E-17,-1.,-2.22049474265426E-16));
#109331=DIRECTION('ref_axis',(-0.677875792531132,-1.78260316429482E-16,
0.73517644814037));
#109332=DIRECTION('center_axis',(-2.21497401043431E-17,1.,2.22049474265426E-16));
#109333=DIRECTION('ref_axis',(0.,0.,1.));
#109334=DIRECTION('center_axis',(-0.368421052641889,0.,-0.92965903855674));
#109335=DIRECTION('ref_axis',(0.,-1.,0.));
#109336=DIRECTION('center_axis',(2.21497401043431E-17,-1.,-2.22049474265426E-16));
#109337=DIRECTION('ref_axis',(0.991347881177066,4.33680868994202E-17,-0.131260727126366));
#109338=DIRECTION('center_axis',(-2.21497401043431E-17,1.,2.22049474265426E-16));
#109339=DIRECTION('ref_axis',(0.991347881177066,5.11044733711702E-17,-0.131260727126366));
#109340=DIRECTION('center_axis',(1.,0.,1.68753899743024E-12));
#109341=DIRECTION('ref_axis',(0.,-1.,0.));
#109342=DIRECTION('center_axis',(-2.21497401043431E-17,1.,2.22049474265426E-16));
#109343=DIRECTION('ref_axis',(-0.827170191871152,1.15648231731787E-16,-0.56195148694513));
#109344=DIRECTION('center_axis',(2.21497401043431E-17,-1.,-2.22049474265426E-16));
#109345=DIRECTION('ref_axis',(-0.827170191871151,1.06459427466835E-16,-0.56195148694513));
#109346=DIRECTION('center_axis',(1.,2.21497401039684E-17,1.68718058920808E-12));
#109347=DIRECTION('ref_axis',(1.19327026859967E-12,-0.707106781186548,-0.707106781186548));
#109348=DIRECTION('',(-1.,-2.21497401039684E-17,-1.68718058920808E-12));
#109349=DIRECTION('',(1.,2.21497401039684E-17,1.68718058920808E-12));
#109350=DIRECTION('center_axis',(-0.707106781185951,0.,-0.707106781187144));
#109351=DIRECTION('ref_axis',(-0.707106781187144,0.,0.707106781185951));
#109352=DIRECTION('center_axis',(0.,0.,-1.));
#109353=DIRECTION('ref_axis',(0.719344700989996,-0.694653295650148,0.));
#109354=DIRECTION('',(4.9183381452852E-33,-2.22049474265426E-16,1.));
#109355=DIRECTION('',(0.,0.,-1.));
#109356=DIRECTION('center_axis',(-1.68718058920808E-12,-1.77635683940025E-16,
1.));
#109357=DIRECTION('ref_axis',(0.719344700989996,-0.694653295650148,0.));
#109358=DIRECTION('center_axis',(0.,1.,1.77635683940025E-16));
#109359=DIRECTION('ref_axis',(-0.827170191871152,0.,-0.561951486945128));
#109360=DIRECTION('',(0.,1.,1.77635683940025E-16));
#109361=DIRECTION('center_axis',(0.,1.,2.22044604925031E-16));
#109362=DIRECTION('ref_axis',(-0.827170191871152,0.,-0.561951486945128));
#109363=DIRECTION('',(0.,-1.,-1.77635683940025E-16));
#109364=DIRECTION('center_axis',(1.68718058920808E-12,1.77635683940025E-16,
-1.));
#109365=DIRECTION('ref_axis',(1.,2.21497401039684E-17,1.68718058920808E-12));
#109366=DIRECTION('center_axis',(1.68718058920808E-12,1.77635683940025E-16,
-1.));
#109367=DIRECTION('ref_axis',(-1.,-1.20024110770287E-15,-1.68709743142951E-12));
#109368=DIRECTION('',(0.,1.,1.77635683940025E-16));
#109369=DIRECTION('center_axis',(-1.68718058920808E-12,-1.77635683940025E-16,
1.));
#109370=DIRECTION('ref_axis',(1.,1.49541069999345E-33,0.));
#109371=DIRECTION('',(-3.81426075461834E-28,-1.,-1.77635683940025E-16));
#109372=DIRECTION('',(1.,-3.7462934736789E-28,1.68718058920808E-12));
#109373=DIRECTION('center_axis',(-1.68718058920808E-12,-1.77635683940025E-16,
1.));
#109374=DIRECTION('ref_axis',(-0.441505993976003,-0.897258300203047,-7.45059728147161E-13));
#109375=DIRECTION('',(1.,-3.7462934736789E-28,1.68718058920808E-12));
#109376=DIRECTION('center_axis',(0.,0.,1.));
#109377=DIRECTION('ref_axis',(-1.,-1.20024110770287E-15,0.));
#109378=DIRECTION('',(0.,0.,1.));
#109379=DIRECTION('center_axis',(-2.21497401043431E-17,1.,2.22049474265426E-16));
#109380=DIRECTION('ref_axis',(-1.,-2.21497401043431E-17,1.83750175990296E-19));
#109381=DIRECTION('center_axis',(0.,-1.,-1.77635683940025E-16));
#109382=DIRECTION('ref_axis',(0.835709485407066,9.75525066900838E-17,-0.549171790973149));
#109383=DIRECTION('',(0.,-1.,-1.77635683940025E-16));
#109384=DIRECTION('center_axis',(0.,1.,2.22044604925031E-16));
#109385=DIRECTION('ref_axis',(0.835709485407066,9.75525066900838E-17,-0.549171790973149));
#109386=DIRECTION('',(0.,-1.,-1.77635683940025E-16));
#109387=DIRECTION('',(0.,1.,1.77635683940025E-16));
#109388=DIRECTION('center_axis',(0.,1.,2.22044604925031E-16));
#109389=DIRECTION('ref_axis',(0.835709485407066,9.75525066900838E-17,-0.549171790973149));
#109390=DIRECTION('',(0.,-1.,-1.77635683940025E-16));
#109391=DIRECTION('',(0.,-1.,-1.77635683940025E-16));
#109392=DIRECTION('center_axis',(-1.88260317010131E-12,2.22049474265488E-16,
-1.));
#109393=DIRECTION('ref_axis',(-0.707106781186548,-0.707106781186548,1.33114401262784E-12));
#109394=DIRECTION('center_axis',(1.88321580552043E-12,0.,1.));
#109395=DIRECTION('ref_axis',(-1.,0.,1.88321580552043E-12));
#109396=DIRECTION('',(-1.88260317010131E-12,2.22049474265488E-16,-1.));
#109397=DIRECTION('center_axis',(-1.88182802673963E-12,2.77555756156289E-15,
-1.));
#109398=DIRECTION('ref_axis',(0.,-1.,-2.77555756156289E-15));
#109399=DIRECTION('',(1.88260317010131E-12,-2.22049474265488E-16,1.));
#109400=DIRECTION('center_axis',(6.93889390390723E-18,1.,2.22049474265475E-16));
#109401=DIRECTION('ref_axis',(0.,0.,1.));
#109402=DIRECTION('center_axis',(-0.707106781186549,0.,-0.707106781186546));
#109403=DIRECTION('ref_axis',(0.,-1.,0.));
#109404=DIRECTION('center_axis',(-6.93889390390723E-18,-1.,-2.22049474265475E-16));
#109405=DIRECTION('ref_axis',(0.923879532510926,8.67361737988403E-17,-0.382683432365961));
#109406=DIRECTION('center_axis',(6.93889390390723E-18,1.,2.22049474265475E-16));
#109407=DIRECTION('ref_axis',(0.923879532510926,7.85639529108843E-17,-0.382683432365961));
#109408=DIRECTION('center_axis',(-0.707106781186548,1.61919227945412E-16,
-0.707106781186548));
#109409=DIRECTION('ref_axis',(-0.500000000000002,-0.707106781186548,0.499999999999998));
#109410=DIRECTION('center_axis',(-0.707106781186548,0.,-0.707106781186548));
#109411=DIRECTION('ref_axis',(0.,-1.,0.));
#109412=DIRECTION('',(0.707106781186548,-1.61919227945412E-16,0.707106781186548));
#109413=DIRECTION('',(-0.707106781186548,1.61919227945412E-16,-0.707106781186548));
#109414=DIRECTION('center_axis',(0.760782493872049,0.,-0.649006931409693));
#109415=DIRECTION('ref_axis',(0.,-1.,0.));
#109416=DIRECTION('center_axis',(6.93889390390723E-18,1.,2.22049474265475E-16));
#109417=DIRECTION('ref_axis',(-0.999217609598081,0.,-0.0395495722998017));
#109418=DIRECTION('center_axis',(-6.93889390390723E-18,-1.,-2.22049474265475E-16));
#109419=DIRECTION('ref_axis',(-0.999217609598081,1.57154267165122E-17,-0.0395495722998017));
#109420=DIRECTION('center_axis',(-6.93889390390723E-18,-1.,-2.22049474265475E-16));
#109421=DIRECTION('ref_axis',(0.,3.86164530304402E-16,-1.));
#109422=DIRECTION('center_axis',(0.787785770581038,0.,-0.615949332063962));
#109423=DIRECTION('ref_axis',(0.,-1.,0.));
#109424=DIRECTION('center_axis',(6.93889390390723E-18,1.,2.22049474265475E-16));
#109425=DIRECTION('ref_axis',(-0.632622226422346,1.81014623580189E-16,-0.774460533943747));
#109426=DIRECTION('center_axis',(-6.93889390390723E-18,-1.,-2.22049474265475E-16));
#109427=DIRECTION('ref_axis',(-0.632622226422346,1.76358252911966E-16,-0.774460533943748));
#109428=DIRECTION('center_axis',(0.499999999999996,0.,0.866025403784441));
#109429=DIRECTION('ref_axis',(0.,-1.,0.));
#109430=DIRECTION('center_axis',(6.93889390390723E-18,1.,2.22049474265475E-16));
#109431=DIRECTION('ref_axis',(0.190629674628629,2.31296463463575E-16,-0.981662022872935));
#109432=DIRECTION('center_axis',(-6.93889390390723E-18,-1.,-2.22049474265475E-16));
#109433=DIRECTION('ref_axis',(0.190629674628629,2.16654776998133E-16,-0.981662022872935));
#109434=DIRECTION('center_axis',(0.5,-1.95769932562834E-16,0.866025403784439));
#109435=DIRECTION('ref_axis',(0.612372435695796,-0.707106781186546,-0.353553390593273));
#109436=DIRECTION('center_axis',(0.500000000000001,0.,0.866025403784438));
#109437=DIRECTION('ref_axis',(0.,-1.,0.));
#109438=DIRECTION('',(-0.5,1.95769932562834E-16,-0.866025403784439));
#109439=DIRECTION('',(0.5,-1.95769932562834E-16,0.866025403784439));
#109440=DIRECTION('center_axis',(-0.681760298603169,0.,0.73157562510551));
#109441=DIRECTION('ref_axis',(0.,-1.,0.));
#109442=DIRECTION('center_axis',(6.93889390390723E-18,1.,2.22049474265475E-16));
#109443=DIRECTION('ref_axis',(0.993590264000317,0.,0.113041529022662));
#109444=DIRECTION('center_axis',(-6.93889390390723E-18,-1.,-2.22049474265475E-16));
#109445=DIRECTION('ref_axis',(0.993590264000317,-3.19952295155008E-17,0.113041529022662));
#109446=DIRECTION('center_axis',(6.93889390390723E-18,1.,2.22049474265475E-16));
#109447=DIRECTION('ref_axis',(0.,0.,1.));
#109448=DIRECTION('center_axis',(0.681760298603169,0.,0.73157562510551));
#109449=DIRECTION('ref_axis',(0.,-1.,0.));
#109450=DIRECTION('center_axis',(-6.93889390390723E-18,-1.,-2.22049474265475E-16));
#109451=DIRECTION('ref_axis',(-1.,0.,-1.33226206458968E-16));
#109452=DIRECTION('center_axis',(-6.93889390390723E-18,-1.,-2.22049474265475E-16));
#109453=DIRECTION('ref_axis',(-1.,0.,-1.33226206458968E-16));
#109454=DIRECTION('center_axis',(6.93889390390723E-18,1.,2.22049474265475E-16));
#109455=DIRECTION('ref_axis',(-1.,6.93889390390726E-18,-1.33226206458968E-16));
#109456=DIRECTION('center_axis',(-0.500000000000002,-2.25347189810573E-16,
0.866025403784438));
#109457=DIRECTION('ref_axis',(0.,-1.,-2.60208521396521E-16));
#109458=DIRECTION('center_axis',(6.93889390390723E-18,1.,2.22049474265475E-16));
#109459=DIRECTION('ref_axis',(0.993590264000317,0.,-0.113041529022662));
#109460=DIRECTION('center_axis',(-6.93889390390723E-18,-1.,-2.22049474265475E-16));
#109461=DIRECTION('ref_axis',(0.993590264000316,1.82063946637941E-17,-0.113041529022662));
#109462=DIRECTION('center_axis',(-0.5,-1.88831038658927E-16,0.866025403784439));
#109463=DIRECTION('ref_axis',(0.612372435695792,-0.70710678118655,0.353553390593273));
#109464=DIRECTION('center_axis',(-0.500000000000002,0.,0.866025403784438));
#109465=DIRECTION('ref_axis',(0.,-1.,0.));
#109466=DIRECTION('',(0.5,1.88831038658927E-16,-0.866025403784439));
#109467=DIRECTION('',(-0.5,-1.88831038658927E-16,0.866025403784439));
#109468=DIRECTION('center_axis',(6.93889390390723E-18,1.,2.22049474265475E-16));
#109469=DIRECTION('ref_axis',(-0.258819045101613,-1.7347234759768E-16,0.965925826289312));
#109470=DIRECTION('center_axis',(-6.93889390390723E-18,-1.,-2.22049474265475E-16));
#109471=DIRECTION('ref_axis',(-0.258819045101613,-2.12687404012715E-16,
0.965925826289312));
#109472=DIRECTION('center_axis',(0.,-1.,-2.22044604925031E-16));
#109473=DIRECTION('ref_axis',(0.993590264000317,0.,0.113041529022661));
#109474=DIRECTION('',(0.,1.,2.22044604925031E-16));
#109475=DIRECTION('center_axis',(0.,-1.,-2.22044604925031E-16));
#109476=DIRECTION('ref_axis',(0.993590264000317,0.,0.113041529022661));
#109477=DIRECTION('',(1.32618116302315E-17,-1.,-2.29701315439687E-16));
#109478=DIRECTION('center_axis',(0.,1.,2.22044604925031E-16));
#109479=DIRECTION('ref_axis',(1.,0.,0.));
#109480=DIRECTION('center_axis',(0.,1.,2.22044604925031E-16));
#109481=DIRECTION('ref_axis',(1.,0.,0.));
#109482=DIRECTION('',(0.,-1.,-2.22044604925031E-16));
#109483=DIRECTION('',(0.,-1.,-2.22044604925031E-16));
#109484=DIRECTION('center_axis',(0.,1.,2.22044604925031E-16));
#109485=DIRECTION('ref_axis',(1.,0.,0.));
#109486=DIRECTION('',(0.,1.,2.22044604925031E-16));
#109487=DIRECTION('center_axis',(-6.93889390390723E-18,-1.,-2.22049474265475E-16));
#109488=DIRECTION('ref_axis',(0.5,-1.98254111540207E-16,0.866025403784439));
#109489=DIRECTION('',(0.,-1.,-2.22044604925031E-16));
#109490=DIRECTION('center_axis',(0.,1.,2.22044604925031E-16));
#109491=DIRECTION('ref_axis',(1.,0.,0.));
#109492=DIRECTION('',(0.,1.,2.22044604925031E-16));
#109493=DIRECTION('center_axis',(-6.93889390390723E-18,-1.,-2.22049474265475E-16));
#109494=DIRECTION('ref_axis',(0.5,1.98254111540207E-16,-0.866025403784438));
#109495=DIRECTION('',(0.,-1.,-2.22044604925031E-16));
#109496=DIRECTION('center_axis',(0.,1.,2.22044604925031E-16));
#109497=DIRECTION('ref_axis',(1.,0.,0.));
#109498=DIRECTION('center_axis',(0.,-1.,-2.22044604925031E-16));
#109499=DIRECTION('ref_axis',(0.993590264000316,0.,-0.113041529022664));
#109500=DIRECTION('',(1.32618116302315E-17,1.,2.29701315439688E-16));
#109501=DIRECTION('center_axis',(0.,-1.,-2.22044604925031E-16));
#109502=DIRECTION('ref_axis',(0.993590264000316,0.,-0.113041529022664));
#109503=DIRECTION('center_axis',(0.866025403784439,-1.26335723491828E-16,
0.5));
#109504=DIRECTION('ref_axis',(-0.5,-1.95761498617786E-16,0.866025403784439));
#109505=DIRECTION('',(-1.15316379899143E-28,-1.,-2.52671446983456E-16));
#109506=DIRECTION('',(0.5,1.92296268638356E-16,-0.866025403784439));
#109507=DIRECTION('center_axis',(-1.15316379899143E-28,-1.,-2.52671446983456E-16));
#109508=DIRECTION('ref_axis',(0.866025403784439,0.,0.5));
#109509=DIRECTION('',(1.15316379899143E-28,1.,2.52671446983456E-16));
#109510=DIRECTION('center_axis',(0.,-1.,-2.22044604925031E-16));
#109511=DIRECTION('ref_axis',(0.866025403784439,0.,0.5));
#109512=DIRECTION('center_axis',(1.,3.60363687185997E-28,-1.88260317010131E-12));
#109513=DIRECTION('ref_axis',(-1.88260317010131E-12,2.22049474265488E-16,
-1.));
#109514=DIRECTION('',(0.,1.,1.91417762866406E-16));
#109515=DIRECTION('',(-1.88260317010131E-12,2.22044604925031E-16,-1.));
#109516=DIRECTION('center_axis',(6.93889390390723E-18,1.,2.22049474265475E-16));
#109517=DIRECTION('ref_axis',(-1.,6.93889390390723E-18,1.83750175990302E-19));
#109518=DIRECTION('center_axis',(-6.93889390390723E-18,-1.,-2.22049474265475E-16));
#109519=DIRECTION('ref_axis',(0.,3.86164530304402E-16,-1.));
#109520=DIRECTION('center_axis',(-6.93889390390723E-18,-1.,-2.22049474265475E-16));
#109521=DIRECTION('ref_axis',(0.828643266372963,1.18548330240756E-16,-0.559777042307691));
#109522=DIRECTION('center_axis',(0.319238463372312,0.,0.947674418512859));
#109523=DIRECTION('ref_axis',(0.,-1.,0.));
#109524=DIRECTION('center_axis',(6.93889390390723E-18,1.,2.22049474265475E-16));
#109525=DIRECTION('ref_axis',(0.828643266372963,1.13134139737618E-16,-0.559777042307691));
#109526=DIRECTION('center_axis',(0.,0.,1.));
#109527=DIRECTION('ref_axis',(0.,-1.,0.));
#109528=DIRECTION('center_axis',(6.93889390390723E-18,1.,2.22049474265475E-16));
#109529=DIRECTION('ref_axis',(0.98683190526879,0.,-0.161749159947031));
#109530=DIRECTION('center_axis',(-6.93889390390723E-18,-1.,-2.22049474265475E-16));
#109531=DIRECTION('ref_axis',(0.98683190526879,2.90687940374697E-17,-0.161749159947031));
#109532=DIRECTION('center_axis',(-2.10803227901262E-16,-2.22049474265475E-16,
1.));
#109533=DIRECTION('ref_axis',(0.707106781186547,-0.707106781186548,0.));
#109534=DIRECTION('center_axis',(0.,0.,1.));
#109535=DIRECTION('ref_axis',(0.,-1.,0.));
#109536=DIRECTION('',(2.10803227901262E-16,2.22049474265475E-16,-1.));
#109537=DIRECTION('',(-2.10803227901262E-16,-2.22049474265475E-16,1.));
#109538=DIRECTION('center_axis',(-1.,0.,-3.46944695195361E-16));
#109539=DIRECTION('ref_axis',(0.,-1.,0.));
#109540=DIRECTION('center_axis',(6.93889390390723E-18,1.,2.22049474265475E-16));
#109541=DIRECTION('ref_axis',(0.707106781186548,-1.15648231731787E-16,0.707106781186547));
#109542=DIRECTION('center_axis',(-6.93889390390723E-18,-1.,-2.22049474265475E-16));
#109543=DIRECTION('ref_axis',(0.707106781186548,-1.61919227945412E-16,0.707106781186547));
#109544=DIRECTION('center_axis',(-1.,6.93889390390728E-18,-2.40389762145677E-16));
#109545=DIRECTION('ref_axis',(0.,-0.707106781186548,0.707106781186548));
#109546=DIRECTION('center_axis',(-1.,0.,0.));
#109547=DIRECTION('ref_axis',(0.,-1.,0.));
#109548=DIRECTION('',(1.,-6.93889390390728E-18,2.40389762145677E-16));
#109549=DIRECTION('',(-1.,6.93889390390728E-18,-2.40389762145677E-16));
#109550=DIRECTION('center_axis',(-0.292682926829268,0.,-0.956209550434764));
#109551=DIRECTION('ref_axis',(0.,-1.,0.));
#109552=DIRECTION('center_axis',(6.93889390390723E-18,1.,2.22049474265475E-16));
#109553=DIRECTION('ref_axis',(-0.594691967816421,-2.31296463463574E-16,
0.803953645065829));
#109554=DIRECTION('center_axis',(-6.93889390390723E-18,-1.,-2.22049474265475E-16));
#109555=DIRECTION('ref_axis',(-0.59469196781642,-1.74390979750496E-16,0.803953645065829));
#109556=DIRECTION('center_axis',(6.93889390390723E-18,1.,2.22049474265475E-16));
#109557=DIRECTION('ref_axis',(0.5,0.,-0.866025403784439));
#109558=DIRECTION('center_axis',(-0.974443225432437,0.,0.224633925329253));
#109559=DIRECTION('ref_axis',(0.,-1.,0.));
#109560=DIRECTION('center_axis',(6.93889390390723E-18,1.,2.22049474265475E-16));
#109561=DIRECTION('ref_axis',(0.5,1.88831038658927E-16,-0.866025403784438));
#109562=DIRECTION('center_axis',(-0.500000000000001,0.,-0.866025403784438));
#109563=DIRECTION('ref_axis',(0.,-1.,0.));
#109564=DIRECTION('center_axis',(6.93889390390723E-18,1.,2.22049474265475E-16));
#109565=DIRECTION('ref_axis',(-0.398898296183895,-2.31296463463574E-16,
0.916995174088493));
#109566=DIRECTION('center_axis',(-6.93889390390723E-18,-1.,-2.22049474265475E-16));
#109567=DIRECTION('ref_axis',(-0.398898296183895,-2.00850383354658E-16,
0.916995174088493));
#109568=DIRECTION('center_axis',(-0.5,1.95769932562834E-16,-0.866025403784439));
#109569=DIRECTION('ref_axis',(-0.612372435695794,-0.707106781186549,0.353553390593272));
#109570=DIRECTION('center_axis',(-0.500000000000001,0.,-0.866025403784438));
#109571=DIRECTION('ref_axis',(0.,-1.,0.));
#109572=DIRECTION('',(0.5,-1.95769932562834E-16,0.866025403784439));
#109573=DIRECTION('',(-0.5,1.95769932562834E-16,-0.866025403784439));
#109574=DIRECTION('center_axis',(0.927320654301968,0.,-0.374267824031094));
#109575=DIRECTION('ref_axis',(0.,-1.,0.));
#109576=DIRECTION('center_axis',(6.93889390390723E-18,1.,2.22049474265475E-16));
#109577=DIRECTION('ref_axis',(-0.945459087052697,1.15648231731787E-16,-0.325740870492914));
#109578=DIRECTION('center_axis',(-6.93889390390723E-18,-1.,-2.22049474265475E-16));
#109579=DIRECTION('ref_axis',(-0.945459087052697,7.88910293352734E-17,-0.325740870492914));
#109580=DIRECTION('center_axis',(-6.93889390390723E-18,-1.,-2.22049474265475E-16));
#109581=DIRECTION('ref_axis',(0.,3.86164530304402E-16,-1.));
#109582=DIRECTION('center_axis',(6.93889390390723E-18,1.,2.22049474265475E-16));
#109583=DIRECTION('ref_axis',(-0.185745985401917,2.18726003492728E-16,-0.982597796103304));
#109584=DIRECTION('center_axis',(-6.93889390390723E-18,-1.,-2.22049474265475E-16));
#109585=DIRECTION('ref_axis',(-0.185745985401917,2.19474195724934E-16,-0.982597796103304));
#109586=DIRECTION('center_axis',(6.93889390390723E-18,1.,2.22049474265475E-16));
#109587=DIRECTION('ref_axis',(0.,0.,1.));
#109588=DIRECTION('center_axis',(-6.93889390390723E-18,-1.,-2.22049474265475E-16));
#109589=DIRECTION('ref_axis',(-0.351073082383137,-2.08550719155025E-16,
0.936348060726354));
#109590=DIRECTION('center_axis',(6.93889390390723E-18,1.,2.22049474265475E-16));
#109591=DIRECTION('ref_axis',(-0.351073082383137,-2.05479535742609E-16,
0.936348060726354));
#109592=DIRECTION('center_axis',(-0.866025403784439,-1.26335723491828E-16,
0.5));
#109593=DIRECTION('ref_axis',(-0.5,1.88822604713879E-16,-0.866025403784439));
#109594=DIRECTION('',(1.4340744877117E-17,-1.,-2.27832548238107E-16));
#109595=DIRECTION('',(0.5,-1.92296268638356E-16,0.866025403784439));
#109596=DIRECTION('',(-1.32618116302315E-17,1.,2.29701315439687E-16));
#109597=DIRECTION('center_axis',(-1.4340744877117E-17,1.,2.27832548238107E-16));
#109598=DIRECTION('ref_axis',(-0.945459087052698,0.,-0.325740870492911));
#109599=DIRECTION('',(0.,1.,2.22044604925031E-16));
#109600=DIRECTION('center_axis',(0.,1.,2.22044604925031E-16));
#109601=DIRECTION('ref_axis',(-0.945459087052698,0.,-0.325740870492911));
#109602=DIRECTION('center_axis',(1.,0.,0.));
#109603=DIRECTION('ref_axis',(0.,-1.,0.));
#109604=DIRECTION('center_axis',(0.,1.,2.22044604925031E-16));
#109605=DIRECTION('ref_axis',(1.,0.,0.));
#109606=DIRECTION('',(0.,-1.,-2.22044604925031E-16));
#109607=DIRECTION('center_axis',(0.,1.,2.22044604925031E-16));
#109608=DIRECTION('ref_axis',(1.,0.,0.));
#109609=DIRECTION('',(0.,-1.,-2.22044604925031E-16));
#109610=DIRECTION('center_axis',(0.,-1.,-2.22044604925031E-16));
#109611=DIRECTION('ref_axis',(1.,0.,0.));
#109612=DIRECTION('',(0.,-1.,-2.22044604925031E-16));
#109613=DIRECTION('center_axis',(-2.37859513600921E-17,0.866025403784432,
0.500000000000011));
#109614=DIRECTION('ref_axis',(0.,0.500000000000011,-0.866025403784432));
#109615=DIRECTION('center_axis',(1.51594548245566E-16,-0.819152044288998,
0.573576436351038));
#109616=DIRECTION('ref_axis',(0.,-0.573576436351038,-0.819152044288998));
#109617=DIRECTION('center_axis',(1.51594548245566E-16,-0.819152044288998,
0.573576436351038));
#109618=DIRECTION('ref_axis',(0.,-0.573576436351038,-0.819152044288998));
#109619=DIRECTION('',(0.,-1.,-2.22044604925031E-16));
#109620=DIRECTION('center_axis',(0.,-1.,-2.22044604925031E-16));
#109621=DIRECTION('ref_axis',(1.,0.,0.));
#109622=DIRECTION('',(0.,1.,2.22044604925031E-16));
#109623=DIRECTION('center_axis',(0.,-1.,-2.22044604925031E-16));
#109624=DIRECTION('ref_axis',(1.,0.,0.));
#109625=DIRECTION('',(0.,1.,2.22044604925031E-16));
#109626=DIRECTION('center_axis',(6.93889390390723E-18,1.,2.22049474265475E-16));
#109627=DIRECTION('ref_axis',(-1.,6.93889390390723E-18,1.83750175990302E-19));
#109628=DIRECTION('center_axis',(-6.93889390390723E-18,-1.,-2.22049474265475E-16));
#109629=DIRECTION('ref_axis',(0.417899232327897,-3.86164530304402E-16,0.908493385567421));
#109630=DIRECTION('center_axis',(0.319238463372311,0.,-0.947674418512859));
#109631=DIRECTION('ref_axis',(0.947674418512859,0.,0.319238463372311));
#109632=DIRECTION('center_axis',(-6.93889390390723E-18,-1.,-2.22049474265475E-16));
#109633=DIRECTION('ref_axis',(0.417899232327897,-2.04630237074555E-16,0.908493385567421));
#109634=DIRECTION('center_axis',(-0.927320654301968,0.,-0.374267824031094));
#109635=DIRECTION('ref_axis',(0.,-1.,0.));
#109636=DIRECTION('center_axis',(6.93889390390723E-18,1.,2.22049474265475E-16));
#109637=DIRECTION('ref_axis',(0.417899232327897,-2.03641451527712E-16,0.908493385567421));
#109638=DIRECTION('center_axis',(0.500000000000001,0.,-0.866025403784438));
#109639=DIRECTION('ref_axis',(0.,-1.,0.));
#109640=DIRECTION('center_axis',(6.93889390390723E-18,1.,2.22049474265475E-16));
#109641=DIRECTION('ref_axis',(-0.945459087052697,-1.15648231731787E-16,
0.325740870492914));
#109642=DIRECTION('center_axis',(-6.93889390390723E-18,-1.,-2.22049474265475E-16));
#109643=DIRECTION('ref_axis',(-0.945459087052697,-6.5770148744186E-17,0.325740870492914));
#109644=DIRECTION('center_axis',(0.5,1.88831038658927E-16,-0.866025403784439));
#109645=DIRECTION('ref_axis',(-0.612372435695796,-0.707106781186547,-0.353553390593273));
#109646=DIRECTION('center_axis',(0.499999999999999,3.00462919747432E-16,
-0.866025403784439));
#109647=DIRECTION('ref_axis',(0.,-1.,-3.46944695195361E-16));
#109648=DIRECTION('',(-0.5,-1.88831038658927E-16,0.866025403784439));
#109649=DIRECTION('',(0.5,1.88831038658927E-16,-0.866025403784439));
#109650=DIRECTION('center_axis',(0.974443225432437,-1.55871097507791E-16,
0.224633925329254));
#109651=DIRECTION('ref_axis',(0.,-1.,-6.93889390390722E-16));
#109652=DIRECTION('center_axis',(6.93889390390723E-18,1.,2.22049474265475E-16));
#109653=DIRECTION('ref_axis',(-0.398898296183895,2.31296463463574E-16,-0.916995174088493));
#109654=DIRECTION('center_axis',(-6.93889390390723E-18,-1.,-2.22049474265475E-16));
#109655=DIRECTION('ref_axis',(-0.398898296183895,2.06386209265997E-16,-0.916995174088493));
#109656=DIRECTION('center_axis',(6.93889390390723E-18,1.,2.22049474265475E-16));
#109657=DIRECTION('ref_axis',(0.,0.,1.));
#109658=DIRECTION('center_axis',(0.292682926829268,0.,-0.956209550434764));
#109659=DIRECTION('ref_axis',(0.,-1.,0.));
#109660=DIRECTION('center_axis',(6.93889390390723E-18,1.,2.22049474265475E-16));
#109661=DIRECTION('ref_axis',(0.5,-1.95769932562834E-16,0.866025403784439));
#109662=DIRECTION('center_axis',(1.,0.,0.));
#109663=DIRECTION('ref_axis',(0.,-1.,0.));
#109664=DIRECTION('center_axis',(6.93889390390723E-18,1.,2.22049474265475E-16));
#109665=DIRECTION('ref_axis',(-0.59469196781642,2.31296463463574E-16,-0.80395364506583));
#109666=DIRECTION('center_axis',(-6.93889390390723E-18,-1.,-2.22049474265475E-16));
#109667=DIRECTION('ref_axis',(-0.59469196781642,1.82643988690864E-16,-0.80395364506583));
#109668=DIRECTION('center_axis',(1.,-6.93889390390728E-18,2.40389762145677E-16));
#109669=DIRECTION('ref_axis',(0.,-0.707106781186548,-0.707106781186547));
#109670=DIRECTION('center_axis',(1.,0.,6.93889390390723E-16));
#109671=DIRECTION('ref_axis',(0.,-1.,0.));
#109672=DIRECTION('',(-1.,6.93889390390728E-18,-2.40389762145677E-16));
#109673=DIRECTION('',(1.,-6.93889390390728E-18,2.40389762145677E-16));
#109674=DIRECTION('center_axis',(0.,0.,1.));
#109675=DIRECTION('ref_axis',(0.,-1.,0.));
#109676=DIRECTION('center_axis',(6.93889390390723E-18,1.,2.22049474265475E-16));
#109677=DIRECTION('ref_axis',(0.707106781186548,1.15648231731787E-16,-0.707106781186547));
#109678=DIRECTION('center_axis',(-6.93889390390723E-18,-1.,-2.22049474265475E-16));
#109679=DIRECTION('ref_axis',(0.707106781186548,1.52106150078638E-16,-0.707106781186547));
#109680=DIRECTION('center_axis',(-2.10803227901262E-16,-2.22049474265475E-16,
1.));
#109681=DIRECTION('ref_axis',(0.707106781186547,-0.707106781186548,0.));
#109682=DIRECTION('center_axis',(-8.67361737988403E-17,0.,1.));
#109683=DIRECTION('ref_axis',(0.,-1.,0.));
#109684=DIRECTION('',(2.10803227901262E-16,2.22049474265475E-16,-1.));
#109685=DIRECTION('',(-2.10803227901262E-16,-2.22049474265475E-16,1.));
#109686=DIRECTION('center_axis',(6.93889390390723E-18,1.,2.22049474265475E-16));
#109687=DIRECTION('ref_axis',(0.986831905268789,0.,0.161749159947033));
#109688=DIRECTION('center_axis',(-6.93889390390723E-18,-1.,-2.22049474265475E-16));
#109689=DIRECTION('ref_axis',(0.986831905268789,-4.27638378207716E-17,0.161749159947033));
#109690=DIRECTION('center_axis',(2.40389762145677E-16,6.12536841172497E-17,
-1.));
#109691=DIRECTION('ref_axis',(1.,6.93889390390718E-18,2.40389762145677E-16));
#109692=DIRECTION('',(4.78544407166015E-17,-1.,-6.12536841172497E-17));
#109693=DIRECTION('',(-1.,5.3377249763659E-32,-2.40389762145677E-16));
#109694=DIRECTION('',(3.86524912081669E-32,1.,6.12536841172497E-17));
#109695=DIRECTION('center_axis',(-4.78544407166015E-17,1.,6.12536841172497E-17));
#109696=DIRECTION('ref_axis',(0.707106781186548,0.,-0.707106781186548));
#109697=DIRECTION('',(-4.78544407166015E-17,1.,6.12536841172497E-17));
#109698=DIRECTION('center_axis',(0.,1.,2.22044604925031E-16));
#109699=DIRECTION('ref_axis',(0.707106781186548,0.,-0.707106781186548));
#109700=DIRECTION('center_axis',(-1.,-4.78544407166015E-17,-2.10803227901262E-16));
#109701=DIRECTION('ref_axis',(2.10803227901262E-16,2.28983498828939E-16,
-1.));
#109702=DIRECTION('',(4.78544407166016E-17,-1.,-3.64102766715121E-16));
#109703=DIRECTION('',(-2.10803227901262E-16,-2.22044604925031E-16,1.));
#109704=DIRECTION('center_axis',(-4.78544407166016E-17,1.,3.64102766715121E-16));
#109705=DIRECTION('ref_axis',(0.98683190526879,0.,0.161749159947033));
#109706=DIRECTION('',(0.,1.,2.22044604925031E-16));
#109707=DIRECTION('center_axis',(0.,1.,2.22044604925031E-16));
#109708=DIRECTION('ref_axis',(0.98683190526879,0.,0.161749159947033));
#109709=DIRECTION('center_axis',(0.,1.,2.22044604925031E-16));
#109710=DIRECTION('ref_axis',(1.,0.,0.));
#109711=DIRECTION('',(0.,-1.,-2.22044604925031E-16));
#109712=DIRECTION('center_axis',(0.,-1.,-2.22044604925031E-16));
#109713=DIRECTION('ref_axis',(1.,0.,0.));
#109714=DIRECTION('',(0.,-1.,-2.22044604925031E-16));
#109715=DIRECTION('center_axis',(0.,-1.,-2.22044604925031E-16));
#109716=DIRECTION('ref_axis',(1.,0.,0.));
#109717=DIRECTION('',(0.,1.,2.22044604925031E-16));
#109718=DIRECTION('center_axis',(1.00839335745948E-17,-0.819152044288994,
-0.573576436351042));
#109719=DIRECTION('ref_axis',(0.,0.573576436351042,-0.819152044288994));
#109720=DIRECTION('center_axis',(-1.47144065207334E-16,0.866025403784436,
-0.500000000000005));
#109721=DIRECTION('ref_axis',(0.,-0.500000000000005,-0.866025403784436));
#109722=DIRECTION('',(0.,1.,2.22044604925031E-16));
#109723=DIRECTION('center_axis',(0.,-1.,-2.22044604925031E-16));
#109724=DIRECTION('ref_axis',(1.,0.,0.));
#109725=DIRECTION('center_axis',(6.93889390390723E-18,1.,2.22049474265475E-16));
#109726=DIRECTION('ref_axis',(-1.,6.93889390390723E-18,1.83750175990302E-19));
#109727=DIRECTION('center_axis',(0.,1.,1.91417762866406E-16));
#109728=DIRECTION('ref_axis',(0.923879532510926,0.,-0.38268343236596));
#109729=DIRECTION('',(-1.74315279842105E-32,1.,1.91417762866406E-16));
#109730=DIRECTION('center_axis',(0.,1.,2.22044604925031E-16));
#109731=DIRECTION('ref_axis',(0.923879532510926,0.,-0.38268343236596));
#109732=DIRECTION('center_axis',(0.707106781186548,1.35352798162394E-16,
-0.707106781186548));
#109733=DIRECTION('ref_axis',(-0.707106781186548,1.61919227945412E-16,-0.707106781186548));
#109734=DIRECTION('',(-1.65275500460854E-17,-1.,-2.07945312912492E-16));
#109735=DIRECTION('',(-0.707106781186548,1.57009245868377E-16,-0.707106781186548));
#109736=DIRECTION('center_axis',(1.65275500460854E-17,1.,2.07945312912492E-16));
#109737=DIRECTION('ref_axis',(-0.999217609598081,0.,-0.0395495722997975));
#109738=DIRECTION('center_axis',(0.,1.,2.22044604925031E-16));
#109739=DIRECTION('ref_axis',(-0.999217609598081,0.,-0.0395495722997975));
#109740=DIRECTION('center_axis',(0.,1.,1.77635683940025E-16));
#109741=DIRECTION('ref_axis',(-0.677875792531128,0.,0.735176448140373));
#109742=DIRECTION('',(0.,1.,1.77635683940025E-16));
#109743=DIRECTION('center_axis',(0.,1.,2.22044604925031E-16));
#109744=DIRECTION('ref_axis',(-0.677875792531128,0.,0.735176448140373));
#109745=DIRECTION('center_axis',(0.,-1.,-1.77635683940025E-16));
#109746=DIRECTION('ref_axis',(0.991347881177066,2.3316589037557E-17,-0.131260727126366));
#109747=DIRECTION('center_axis',(0.,1.,2.22044604925031E-16));
#109748=DIRECTION('ref_axis',(-1.,0.,1.83750175990301E-19));
#109749=DIRECTION('center_axis',(2.89174624745853E-28,1.,2.27504718161182E-16));
#109750=DIRECTION('ref_axis',(-0.707106781186546,0.,0.707106781186549));
#109751=DIRECTION('center_axis',(0.,-1.,-2.22044604925031E-16));
#109752=DIRECTION('ref_axis',(-0.707106781186546,0.,0.707106781186549));
#109753=DIRECTION('',(2.89174624745853E-28,1.,2.27504718161182E-16));
#109754=DIRECTION('center_axis',(0.,-1.,-2.22044604925031E-16));
#109755=DIRECTION('ref_axis',(-0.707106781186546,0.,0.707106781186549));
#109756=DIRECTION('',(-2.89174624745853E-28,-1.,-2.27504718161182E-16));
#109757=DIRECTION('center_axis',(0.707106781186548,1.60870128963502E-16,
-0.707106781186548));
#109758=DIRECTION('ref_axis',(-0.707106781186548,1.61919227945507E-16,-0.707106781186548));
#109759=DIRECTION('',(0.707106781186548,-1.57009245868377E-16,0.707106781186548));
#109760=DIRECTION('',(0.707106781186548,-1.57009245868377E-16,0.707106781186548));
#109761=DIRECTION('',(2.09862273058998E-32,1.,2.27504718160893E-16));
#109762=DIRECTION('',(0.707106781186548,-1.57009245868377E-16,0.707106781186548));
#109763=DIRECTION('',(0.,-1.,-2.27504718160893E-16));
#109764=DIRECTION('',(0.707106781186548,-1.57009245868377E-16,0.707106781186548));
#109765=DIRECTION('',(2.73005661793073E-18,-1.,-2.24774661542962E-16));
#109766=DIRECTION('center_axis',(1.,-1.97827874126669E-27,7.42447950166969E-12));
#109767=DIRECTION('ref_axis',(7.42447950166969E-12,2.22049474265423E-16,
-1.));
#109768=DIRECTION('',(-7.42447950166969E-12,-2.22044604925031E-16,1.));
#109769=DIRECTION('',(9.65588433237313E-28,-1.,-3.96508223080413E-16));
#109770=DIRECTION('',(7.42447950166969E-12,2.22049474265423E-16,-1.));
#109771=DIRECTION('center_axis',(0.,-1.,-2.22044604925031E-16));
#109772=DIRECTION('ref_axis',(0.0584478133347438,0.,0.998290465303755));
#109773=DIRECTION('center_axis',(0.,-1.,-2.22044604925031E-16));
#109774=DIRECTION('ref_axis',(0.0584478133347438,0.,0.998290465303755));
#109775=DIRECTION('center_axis',(0.,-1.,-2.22044604925031E-16));
#109776=DIRECTION('ref_axis',(0.0584478133347438,0.,0.998290465303755));
#109777=DIRECTION('center_axis',(1.21828783833459E-17,-1.,-2.31570082641268E-16));
#109778=DIRECTION('ref_axis',(0.190629674628636,0.,-0.981662022872934));
#109779=DIRECTION('',(-1.21828783833459E-17,1.,2.31570082641268E-16));
#109780=DIRECTION('center_axis',(0.,1.,2.22044604925031E-16));
#109781=DIRECTION('ref_axis',(0.190629674628636,0.,-0.981662022872934));
#109782=DIRECTION('center_axis',(2.09862273058998E-32,1.,2.27504718160893E-16));
#109783=DIRECTION('ref_axis',(-0.923879532511288,0.,0.382683432365088));
#109784=DIRECTION('center_axis',(0.,-1.,-2.22044604925031E-16));
#109785=DIRECTION('ref_axis',(-0.923879532511288,0.,0.382683432365088));
#109786=DIRECTION('',(-2.09862273058998E-32,-1.,-2.27504718160893E-16));
#109787=DIRECTION('center_axis',(0.,-1.,-2.22044604925031E-16));
#109788=DIRECTION('ref_axis',(-0.923879532511288,0.,0.382683432365088));
#109789=DIRECTION('center_axis',(0.,-1.,-3.96508223080413E-16));
#109790=DIRECTION('ref_axis',(-0.598633244308989,0.,-0.80102324486128));
#109791=DIRECTION('center_axis',(0.,1.,2.22044604925031E-16));
#109792=DIRECTION('ref_axis',(-0.598633244308989,0.,-0.80102324486128));
#109793=DIRECTION('',(0.,1.,3.96508223080413E-16));
#109794=DIRECTION('center_axis',(0.,1.,2.22044604925031E-16));
#109795=DIRECTION('ref_axis',(-0.598633244308989,0.,-0.80102324486128));
#109796=DIRECTION('center_axis',(0.,-1.,-3.96508223080413E-16));
#109797=DIRECTION('ref_axis',(-1.,0.,1.837501759903E-19));
#109798=DIRECTION('center_axis',(6.93889390390723E-18,1.,2.22049474265475E-16));
#109799=DIRECTION('ref_axis',(-1.,6.93889390390723E-18,1.83750175990302E-19));
#109800=DIRECTION('',(0.,-1.,-3.96508223080413E-16));
#109801=DIRECTION('center_axis',(0.,1.,2.22044604925031E-16));
#109802=DIRECTION('ref_axis',(-1.,0.,1.837501759903E-19));
#109803=DIRECTION('center_axis',(1.,8.3944909223599E-32,-4.61226199516842E-16));
#109804=DIRECTION('ref_axis',(-4.61226199516842E-16,2.22049474265475E-16,
-1.));
#109805=DIRECTION('',(4.61226199516842E-16,-2.22044604925031E-16,1.));
#109806=DIRECTION('',(0.,1.,2.22044604925031E-16));
#109807=DIRECTION('',(4.61226199516842E-16,-2.22044604925031E-16,1.));
#109808=DIRECTION('center_axis',(0.,1.,2.22044604925031E-16));
#109809=DIRECTION('ref_axis',(-0.939690906904483,-7.59447731678524E-17,
0.342024852139477));
#109810=DIRECTION('center_axis',(0.,-1.,-2.22044604925031E-16));
#109811=DIRECTION('ref_axis',(-0.939690906904483,-7.59447731678524E-17,
0.342024852139477));
#109812=DIRECTION('center_axis',(0.,1.,2.22044604925031E-16));
#109813=DIRECTION('ref_axis',(0.,2.22044604925031E-16,-1.));
#109814=DIRECTION('',(0.,1.,2.22044604925031E-16));
#109815=DIRECTION('center_axis',(0.,-1.,-2.22044604925031E-16));
#109816=DIRECTION('ref_axis',(-1.,0.,0.));
#109817=DIRECTION('center_axis',(0.,-1.,-2.22044604925031E-16));
#109818=DIRECTION('ref_axis',(-1.,0.,0.));
#109819=DIRECTION('center_axis',(0.,1.,2.22044604925031E-16));
#109820=DIRECTION('ref_axis',(1.,0.,0.));
#109821=DIRECTION('center_axis',(0.,1.,2.22044604925031E-16));
#109822=DIRECTION('ref_axis',(1.,0.,0.));
#109823=DIRECTION('center_axis',(0.,-1.,-2.22044604925031E-16));
#109824=DIRECTION('ref_axis',(1.,0.,0.));
#109825=DIRECTION('',(0.,-1.,-2.22044604925031E-16));
#109826=DIRECTION('center_axis',(0.,1.,2.22044604925031E-16));
#109827=DIRECTION('ref_axis',(-1.,0.,0.));
#109828=DIRECTION('center_axis',(0.,-1.,-2.22044604925031E-16));
#109829=DIRECTION('ref_axis',(-1.,0.,0.));
#109830=DIRECTION('',(0.,1.,2.22044604925031E-16));
#109831=DIRECTION('center_axis',(1.,0.,0.));
#109832=DIRECTION('ref_axis',(0.,2.22044604925031E-16,-1.));
#109833=DIRECTION('',(0.,-1.,0.));
#109834=DIRECTION('',(0.,2.22044604925031E-16,-1.));
#109835=DIRECTION('',(0.,1.,2.22044604925031E-16));
#109836=DIRECTION('',(-6.34413156931604E-16,2.22044604925031E-16,-1.));
#109837=DIRECTION('',(0.,1.,2.22044604925031E-16));
#109838=DIRECTION('',(0.,2.22044604925031E-16,-1.));
#109839=DIRECTION('',(0.,1.,2.22044604925031E-16));
#109840=DIRECTION('',(0.,-2.22044604925031E-16,1.));
#109841=DIRECTION('',(0.,1.,2.22044604925031E-16));
#109842=DIRECTION('center_axis',(0.,-1.,0.));
#109843=DIRECTION('ref_axis',(-0.294883912309792,0.,-0.95553308590591));
#109844=DIRECTION('',(0.,1.,0.));
#109845=DIRECTION('center_axis',(0.,1.,2.22044604925031E-16));
#109846=DIRECTION('ref_axis',(-0.294883912309792,0.,-0.95553308590591));
#109847=DIRECTION('center_axis',(0.,-1.,0.));
#109848=DIRECTION('ref_axis',(-1.,0.,-6.93889390390723E-17));
#109849=DIRECTION('',(0.,-1.,0.));
#109850=DIRECTION('center_axis',(0.,1.,2.22044604925031E-16));
#109851=DIRECTION('ref_axis',(-1.,0.,-6.93889390390723E-17));
#109852=DIRECTION('center_axis',(0.,1.,0.));
#109853=DIRECTION('ref_axis',(-0.707106781186547,0.,-0.707106781186548));
#109854=DIRECTION('center_axis',(0.,1.,2.22044604925031E-16));
#109855=DIRECTION('ref_axis',(-0.707106781186547,0.,-0.707106781186548));
#109856=DIRECTION('center_axis',(0.,1.,2.22044604925031E-16));
#109857=DIRECTION('ref_axis',(0.707106781186548,0.,0.707106781186548));
#109858=DIRECTION('center_axis',(0.,-1.,-2.22044604925031E-16));
#109859=DIRECTION('ref_axis',(0.707106781186548,0.,0.707106781186548));
#109860=DIRECTION('',(0.,-1.,-2.22044604925031E-16));
#109861=DIRECTION('center_axis',(0.,-1.,-2.22044604925031E-16));
#109862=DIRECTION('ref_axis',(0.707106781186548,0.,0.707106781186548));
#109863=DIRECTION('center_axis',(-6.50074362628841E-34,-1.,-2.27504718160893E-16));
#109864=DIRECTION('ref_axis',(0.923879532511286,0.,0.382683432365092));
#109865=DIRECTION('center_axis',(0.,-1.,-2.22044604925031E-16));
#109866=DIRECTION('ref_axis',(0.923879532511286,0.,0.382683432365092));
#109867=DIRECTION('',(6.50074362628841E-34,1.,2.27504718160893E-16));
#109868=DIRECTION('center_axis',(0.,-1.,-2.22044604925031E-16));
#109869=DIRECTION('ref_axis',(0.923879532511286,0.,0.382683432365092));
#109870=DIRECTION('',(-6.50074362628841E-34,-1.,-2.27504718160893E-16));
#109871=DIRECTION('center_axis',(-0.707106781186547,1.60870128963502E-16,
-0.707106781186548));
#109872=DIRECTION('ref_axis',(-0.707106781186548,-1.52106150078733E-16,
0.707106781186547));
#109873=DIRECTION('',(0.707106781186548,1.57009245868377E-16,-0.707106781186547));
#109874=DIRECTION('',(0.,1.,2.27504718160893E-16));
#109875=DIRECTION('',(0.707106781186548,1.57009245868377E-16,-0.707106781186547));
#109876=DIRECTION('center_axis',(0.,-1.,-2.22044604925031E-16));
#109877=DIRECTION('ref_axis',(-0.926903899779187,0.,0.375298761754066));
#109878=DIRECTION('',(0.,1.,2.22044604925031E-16));
#109879=DIRECTION('center_axis',(0.,1.,2.22044604925031E-16));
#109880=DIRECTION('ref_axis',(-0.926903899779187,0.,0.375298761754066));
#109881=DIRECTION('center_axis',(1.,2.64363574135728E-32,-1.190587693968E-16));
#109882=DIRECTION('ref_axis',(-1.190587693968E-16,2.22044604925031E-16,
-1.));
#109883=DIRECTION('',(1.190587693968E-16,-2.22044604925031E-16,1.));
#109884=DIRECTION('',(0.,-1.,-2.22044604925031E-16));
#109885=DIRECTION('',(-1.190587693968E-16,2.22044604925031E-16,-1.));
#109886=DIRECTION('center_axis',(0.,1.,2.22044604925031E-16));
#109887=DIRECTION('ref_axis',(0.707106781186548,1.57009245868377E-16,-0.707106781186548));
#109888=DIRECTION('center_axis',(0.,-1.,-2.22044604925031E-16));
#109889=DIRECTION('ref_axis',(0.707106781186548,1.57009245868377E-16,-0.707106781186548));
#109890=DIRECTION('',(0.,1.,2.22044604925031E-16));
#109891=DIRECTION('center_axis',(0.,-1.,-2.22044604925031E-16));
#109892=DIRECTION('ref_axis',(0.707106781186548,1.57009245868377E-16,-0.707106781186548));
#109893=DIRECTION('center_axis',(0.,1.,2.22044604925031E-16));
#109894=DIRECTION('ref_axis',(0.905538513813742,0.,-0.424264068711928));
#109895=DIRECTION('center_axis',(0.,-1.,-2.22044604925031E-16));
#109896=DIRECTION('ref_axis',(0.905538513813742,0.,-0.424264068711928));
#109897=DIRECTION('',(0.,-1.,-2.22044604925031E-16));
#109898=DIRECTION('center_axis',(0.,-1.,-2.22044604925031E-16));
#109899=DIRECTION('ref_axis',(0.905538513813742,0.,-0.424264068711928));
#109900=DIRECTION('',(0.,1.,2.22044604925031E-16));
#109901=DIRECTION('center_axis',(0.,1.,2.22044604925031E-16));
#109902=DIRECTION('ref_axis',(-0.30491067796787,2.11471052309918E-16,-0.952380952382592));
#109903=DIRECTION('center_axis',(0.,-1.,-2.22044604925031E-16));
#109904=DIRECTION('ref_axis',(-0.30491067796787,2.11471052309918E-16,-0.952380952382592));
#109905=DIRECTION('center_axis',(0.,1.,2.22044604925031E-16));
#109906=DIRECTION('ref_axis',(-0.30491067796787,2.11471052309918E-16,-0.952380952382592));
#109907=DIRECTION('center_axis',(0.,1.,2.22044604925031E-16));
#109908=DIRECTION('ref_axis',(1.,0.,0.));
#109909=DIRECTION('center_axis',(0.,-1.,-2.22044604925031E-16));
#109910=DIRECTION('ref_axis',(1.,0.,0.));
#109911=DIRECTION('',(0.,-1.,-2.22044604925031E-16));
#109912=DIRECTION('center_axis',(0.,-1.,-2.22044604925031E-16));
#109913=DIRECTION('ref_axis',(1.,0.,0.));
#109914=DIRECTION('center_axis',(0.,-1.,-2.22044604925031E-16));
#109915=DIRECTION('ref_axis',(0.707106781186548,-1.57009245868377E-16,0.707106781186548));
#109916=DIRECTION('center_axis',(0.,-1.,-2.22044604925031E-16));
#109917=DIRECTION('ref_axis',(0.707106781186548,-1.57009245868377E-16,0.707106781186548));
#109918=DIRECTION('',(0.,-1.,-2.22044604925031E-16));
#109919=DIRECTION('center_axis',(0.,-1.,-2.22044604925031E-16));
#109920=DIRECTION('ref_axis',(0.707106781186548,-1.57009245868377E-16,0.707106781186548));
#109921=DIRECTION('center_axis',(0.,-1.,-2.22044604925031E-16));
#109922=DIRECTION('ref_axis',(-0.00296584926884181,-2.22043628341636E-16,
0.999995601859386));
#109923=DIRECTION('',(0.,1.,2.22044604925031E-16));
#109924=DIRECTION('center_axis',(0.,-1.,-2.22044604925031E-16));
#109925=DIRECTION('ref_axis',(-0.00296584926884181,-2.22043628341636E-16,
0.999995601859386));
#109926=DIRECTION('',(0.,-1.,-2.22044604925031E-16));
#109927=DIRECTION('center_axis',(0.,1.,2.22044604925031E-16));
#109928=DIRECTION('ref_axis',(-0.00296584926884181,-2.22043628341636E-16,
0.999995601859386));
#109929=DIRECTION('center_axis',(-7.93016446160826E-17,-3.1720657846433E-16,
1.));
#109930=DIRECTION('ref_axis',(1.33226762955019E-15,-1.,-3.1720657846433E-16));
#109931=DIRECTION('',(-7.93016446160826E-17,-3.1720657846433E-16,1.));
#109932=DIRECTION('',(-7.93016446160826E-17,-3.1720657846433E-16,1.));
#109933=DIRECTION('center_axis',(-1.58603289232165E-16,-3.1720657846433E-16,
1.));
#109934=DIRECTION('ref_axis',(-1.27675647831893E-15,-1.,-3.1720657846433E-16));
#109935=DIRECTION('',(-1.58603289232165E-16,-3.1720657846433E-16,1.));
#109936=DIRECTION('',(-1.58603289232165E-16,-3.1720657846433E-16,1.));
#109937=DIRECTION('center_axis',(0.,0.,1.));
#109938=DIRECTION('ref_axis',(1.,-7.0059776216349E-34,0.));
#109939=DIRECTION('center_axis',(0.,-2.22044604925031E-16,1.));
#109940=DIRECTION('ref_axis',(1.,-7.0059776216349E-34,0.));
#109941=DIRECTION('',(0.,0.,1.));
#109942=DIRECTION('center_axis',(1.68718058920808E-12,1.77635683940025E-16,
-1.));
#109943=DIRECTION('ref_axis',(1.,-7.0059776216349E-34,0.));
#109944=DIRECTION('center_axis',(-1.68718058920808E-12,-1.77635683940025E-16,
1.));
#109945=DIRECTION('ref_axis',(1.,0.,1.68718058920808E-12));
#109946=DIRECTION('',(-1.,7.0059776216349E-34,-1.68718058920808E-12));
#109947=DIRECTION('center_axis',(-1.68718058920808E-12,-1.77635683940025E-16,
1.));
#109948=DIRECTION('ref_axis',(0.441505993976003,0.897258300203047,0.));
#109949=DIRECTION('center_axis',(-1.68718058920808E-12,-1.77635683940025E-16,
1.));
#109950=DIRECTION('ref_axis',(1.,-2.99704178492074E-28,1.68718058920808E-12));
#109951=DIRECTION('center_axis',(-1.68753899746303E-12,0.,1.));
#109952=DIRECTION('ref_axis',(1.,-1.85111672238412E-28,1.04208212862878E-12));
#109953=DIRECTION('',(0.707106781194979,8.65956056243049E-17,-0.707106781178116));
#109954=DIRECTION('center_axis',(0.,0.,1.));
#109955=DIRECTION('ref_axis',(1.,-7.0059776216349E-34,0.));
#109956=DIRECTION('center_axis',(0.,-2.22044604925031E-16,1.));
#109957=DIRECTION('ref_axis',(1.,-7.0059776216349E-34,0.));
#109958=DIRECTION('',(0.,0.,1.));
#109959=DIRECTION('center_axis',(1.68718058920808E-12,1.77635683940025E-16,
-1.));
#109960=DIRECTION('ref_axis',(1.,-7.0059776216349E-34,0.));
#109961=DIRECTION('center_axis',(-1.68718058920808E-12,-1.77635683940025E-16,
1.));
#109962=DIRECTION('ref_axis',(1.,0.,1.68718058920808E-12));
#109963=DIRECTION('',(-1.,7.0059776216349E-34,-1.68718058920808E-12));
#109964=DIRECTION('center_axis',(-1.68718058920808E-12,-1.77635683940025E-16,
1.));
#109965=DIRECTION('ref_axis',(0.441505993976003,0.897258300203047,0.));
#109966=DIRECTION('center_axis',(-1.68718058920808E-12,-1.77635683940025E-16,
1.));
#109967=DIRECTION('ref_axis',(1.,-2.99704178492074E-28,1.68718058920808E-12));
#109968=DIRECTION('center_axis',(-1.6875389973825E-12,0.,1.));
#109969=DIRECTION('ref_axis',(1.,-1.85111672238412E-28,1.04208212862878E-12));
#109970=DIRECTION('',(0.707106781178108,8.65956056222387E-17,-0.707106781194987));
#109971=DIRECTION('center_axis',(1.68684510806422E-12,0.,-1.));
#109972=DIRECTION('ref_axis',(-0.441505993976003,-0.897258300203047,-4.62840134152024E-13));
#109973=DIRECTION('center_axis',(-1.68718058920808E-12,-1.77635683940025E-16,
1.));
#109974=DIRECTION('ref_axis',(1.,0.,1.68718058920808E-12));
#109975=DIRECTION('center_axis',(1.68718058920808E-12,1.77635683940025E-16,
-1.));
#109976=DIRECTION('ref_axis',(-1.,0.,0.));
#109977=DIRECTION('',(-1.,3.7462934736789E-28,-1.68718058920808E-12));
#109978=DIRECTION('',(-1.79863670155429E-15,-1.,-1.7763568394306E-16));
#109979=DIRECTION('center_axis',(-1.68718058920808E-12,-1.77635683940025E-16,
1.));
#109980=DIRECTION('ref_axis',(-1.,-1.77635683940025E-15,0.));
#109981=DIRECTION('',(-1.43890936124343E-15,1.,1.77635683937597E-16));
#109982=DIRECTION('',(-1.,3.7462934736789E-28,-1.68718058920808E-12));
#109983=DIRECTION('center_axis',(-1.68718058920808E-12,-1.77635683940025E-16,
1.));
#109984=DIRECTION('ref_axis',(1.,0.,1.68718058920808E-12));
#109985=DIRECTION('center_axis',(1.68718058920808E-12,1.77635683940025E-16,
-1.));
#109986=DIRECTION('ref_axis',(-1.,0.,0.));
#109987=DIRECTION('',(-1.,3.7462934736789E-28,-1.68718058920808E-12));
#109988=DIRECTION('',(1.61669403717014E-32,-1.,-1.77635683940025E-16));
#109989=DIRECTION('center_axis',(-1.68718058920808E-12,-1.77635683940025E-16,
1.));
#109990=DIRECTION('ref_axis',(-1.,7.0059776216349E-34,0.));
#109991=DIRECTION('',(-1.61669403717014E-32,1.,1.77635683940025E-16));
#109992=DIRECTION('',(-1.,3.7462934736789E-28,-1.68718058920808E-12));
#109993=DIRECTION('center_axis',(1.,-1.79863670155429E-15,1.85037170770859E-16));
#109994=DIRECTION('ref_axis',(1.79863670155429E-15,1.,1.7763568394306E-16));
#109995=DIRECTION('',(1.8503717077086E-16,2.22044604925031E-16,-1.));
#109996=DIRECTION('',(1.79863670155429E-15,1.,1.7763568394306E-16));
#109997=DIRECTION('',(-1.85037170770859E-16,0.,1.));
#109998=DIRECTION('center_axis',(-1.85037170770859E-16,0.,1.));
#109999=DIRECTION('ref_axis',(-1.,-1.77635683940025E-15,-1.85037170770859E-16));
#110000=DIRECTION('center_axis',(-1.68718058920808E-12,-1.77635683940025E-16,
1.));
#110001=DIRECTION('ref_axis',(-1.,-1.77635683940025E-15,0.));
#110002=DIRECTION('center_axis',(-1.68718058920808E-12,-1.77635683940025E-16,
1.));
#110003=DIRECTION('ref_axis',(-1.,-1.77635683940025E-15,0.));
#110004=DIRECTION('',(-1.85037170770859E-16,0.,1.));
#110005=DIRECTION('center_axis',(-1.,-1.43890936124343E-15,-1.85037170770859E-16));
#110006=DIRECTION('ref_axis',(1.43890936124343E-15,-1.,-1.77635683937597E-16));
#110007=DIRECTION('',(1.43890936124343E-15,-1.,-1.77635683937597E-16));
#110008=DIRECTION('',(-1.85037170770859E-16,-2.22044604925031E-16,1.));
#110009=DIRECTION('center_axis',(1.,1.61669403717014E-32,0.));
#110010=DIRECTION('ref_axis',(-1.61669403717014E-32,1.,1.77635683940025E-16));
#110011=DIRECTION('',(-3.58978188768097E-48,2.22044604925031E-16,-1.));
#110012=DIRECTION('',(-1.61669403717014E-32,1.,1.77635683940025E-16));
#110013=DIRECTION('',(0.,0.,1.));
#110014=DIRECTION('center_axis',(0.,0.,1.));
#110015=DIRECTION('ref_axis',(-1.,7.0059776216349E-34,0.));
#110016=DIRECTION('center_axis',(-1.68718058920808E-12,-1.77635683940025E-16,
1.));
#110017=DIRECTION('ref_axis',(-1.,7.0059776216349E-34,-1.57702134180175E-16));
#110018=DIRECTION('center_axis',(-1.68718058920808E-12,-1.77635683940025E-16,
1.));
#110019=DIRECTION('ref_axis',(-1.,7.0059776216349E-34,-1.57702134180175E-16));
#110020=DIRECTION('',(0.,0.,1.));
#110021=DIRECTION('center_axis',(-1.,-1.61669403717014E-32,0.));
#110022=DIRECTION('ref_axis',(1.61669403717014E-32,-1.,-1.77635683940025E-16));
#110023=DIRECTION('',(1.61669403717014E-32,-1.,-1.77635683940025E-16));
#110024=DIRECTION('',(3.58978188768097E-48,-2.22044604925031E-16,1.));
#110025=DIRECTION('center_axis',(0.577350269189626,0.577350269189625,0.577350269189626));
#110026=DIRECTION('ref_axis',(-0.707106781186548,0.,0.707106781186547));
#110027=DIRECTION('center_axis',(2.77555756159287E-17,-1.,-1.78063851184191E-16));
#110028=DIRECTION('ref_axis',(1.,2.77555756159287E-17,4.9422646860063E-33));
#110029=DIRECTION('center_axis',(0.408248290463863,-0.816496580927726,0.408248290463863));
#110030=DIRECTION('ref_axis',(0.707106781186547,0.,-0.707106781186548));
#110031=DIRECTION('center_axis',(2.77555756159287E-17,-1.,-1.78063851184191E-16));
#110032=DIRECTION('ref_axis',(-1.,0.,-1.68830924263176E-12));
#110033=DIRECTION('center_axis',(0.,1.,2.22044604925031E-16));
#110034=DIRECTION('ref_axis',(-1.,0.,-1.68830924263176E-12));
#110035=DIRECTION('center_axis',(0.577350269189626,0.577350269189626,0.577350269189626));
#110036=DIRECTION('ref_axis',(-0.707106781186547,0.,0.707106781186548));
#110037=DIRECTION('center_axis',(1.72173578928287E-15,-1.,-1.78063851181333E-16));
#110038=DIRECTION('ref_axis',(1.,1.72173578928287E-15,3.06578905356441E-31));
#110039=DIRECTION('center_axis',(0.408248290463863,-0.816496580927726,0.408248290463863));
#110040=DIRECTION('ref_axis',(0.707106781186548,0.,-0.707106781186548));
#110041=DIRECTION('center_axis',(1.72173578928287E-15,-1.,-1.78063851181333E-16));
#110042=DIRECTION('ref_axis',(-1.,-1.77635683940025E-15,-1.68779887675753E-12));
#110043=DIRECTION('center_axis',(0.,1.,2.22044604925031E-16));
#110044=DIRECTION('ref_axis',(-1.,-1.77635683940025E-15,-1.68779887675753E-12));
#110045=DIRECTION('center_axis',(-1.,1.5355029188888E-32,-1.73472347597681E-16));
#110046=DIRECTION('ref_axis',(2.32378448758667E-32,-1.,-2.22472772169198E-16));
#110047=DIRECTION('',(-1.73472347597681E-16,-2.22044604925031E-16,1.));
#110048=DIRECTION('',(2.31635696988567E-32,-1.,-2.22044604925031E-16));
#110049=DIRECTION('',(-1.73472347597681E-16,0.,1.));
#110050=DIRECTION('center_axis',(-1.73472347597681E-16,0.,1.));
#110051=DIRECTION('ref_axis',(-1.,7.0059776216349E-34,-1.73472347597681E-16));
#110052=DIRECTION('center_axis',(-1.73472347597681E-16,0.,1.));
#110053=DIRECTION('ref_axis',(-1.,7.0059776216349E-34,-1.73472347597681E-16));
#110054=DIRECTION('center_axis',(0.,-2.22044604925031E-16,1.));
#110055=DIRECTION('ref_axis',(-1.,7.0059776216349E-34,-1.73472347597681E-16));
#110056=DIRECTION('',(-1.73472347597681E-16,0.,1.));
#110057=DIRECTION('center_axis',(1.,-1.5355029188888E-32,1.73472347597681E-16));
#110058=DIRECTION('ref_axis',(-2.32378448758667E-32,1.,2.22472772169198E-16));
#110059=DIRECTION('',(-2.31635696988567E-32,1.,2.22044604925031E-16));
#110060=DIRECTION('',(1.73472347597681E-16,2.22044604925031E-16,-1.));
#110061=DIRECTION('center_axis',(0.,0.,1.));
#110062=DIRECTION('ref_axis',(1.96005385927235E-15,1.,0.));
#110063=DIRECTION('center_axis',(-1.,-3.59727340310858E-15,-1.73472347597681E-16));
#110064=DIRECTION('ref_axis',(3.59727340310858E-15,-1.,-2.22472772169197E-16));
#110065=DIRECTION('',(-1.7347234759768E-16,-2.22044604925031E-16,1.));
#110066=DIRECTION('',(3.59727340310858E-15,-1.,-2.22044604925031E-16));
#110067=DIRECTION('',(-1.73472347597681E-16,0.,1.));
#110068=DIRECTION('center_axis',(-1.73472347597681E-16,0.,1.));
#110069=DIRECTION('ref_axis',(1.,-7.0059776216349E-34,1.73472347597681E-16));
#110070=DIRECTION('center_axis',(-1.73472347597681E-16,0.,1.));
#110071=DIRECTION('ref_axis',(1.,-7.0059776216349E-34,1.73472347597681E-16));
#110072=DIRECTION('center_axis',(0.,-2.22044604925031E-16,1.));
#110073=DIRECTION('ref_axis',(1.,-7.0059776216349E-34,1.73472347597681E-16));
#110074=DIRECTION('',(-1.73472347597681E-16,0.,1.));
#110075=DIRECTION('center_axis',(1.,-3.23754606279772E-15,1.73472347597681E-16));
#110076=DIRECTION('ref_axis',(3.23754606279772E-15,1.,2.22472772169198E-16));
#110077=DIRECTION('',(3.23754606279772E-15,1.,2.22044604925031E-16));
#110078=DIRECTION('',(1.73472347597681E-16,2.22044604925031E-16,-1.));
#110079=DIRECTION('center_axis',(0.,0.,1.));
#110080=DIRECTION('ref_axis',(1.83697019872103E-16,1.,0.));
#110081=DIRECTION('center_axis',(0.,2.22044604925031E-16,-1.));
#110082=DIRECTION('ref_axis',(-1.,0.,0.));
#110083=DIRECTION('',(1.,0.,0.));
#110084=DIRECTION('',(0.,-1.,-2.22044604925031E-16));
#110085=DIRECTION('',(-1.,0.,0.));
#110086=DIRECTION('center_axis',(0.,2.22044604925031E-16,-1.));
#110087=DIRECTION('ref_axis',(-1.,0.,0.));
#110088=DIRECTION('',(1.,0.,0.));
#110089=DIRECTION('',(1.,0.,0.));
#110090=DIRECTION('center_axis',(0.,-2.46716227694479E-16,1.));
#110091=DIRECTION('ref_axis',(-0.803531498237542,0.595262237455166,1.46860853713914E-16));
#110092=DIRECTION('',(0.,2.46716227694479E-16,-1.));
#110093=DIRECTION('',(0.,2.46716227694479E-16,-1.));
#110094=DIRECTION('center_axis',(1.,-2.99689426160925E-28,1.68710148498153E-12));
#110095=DIRECTION('ref_axis',(-1.68710148498153E-12,-2.22049474265463E-16,
1.));
#110096=DIRECTION('center_axis',(1.,-6.81117991896132E-28,1.68711550397432E-12));
#110097=DIRECTION('ref_axis',(-1.68711550397432E-12,-2.22049474265463E-16,
1.));
#110098=DIRECTION('',(3.81426075461834E-28,1.,1.77635683940025E-16));
#110099=DIRECTION('',(-3.81426075461834E-28,-1.,-1.77635683940025E-16));
#110100=DIRECTION('',(-1.68711550397432E-12,-2.22044604925031E-16,1.));
#110101=DIRECTION('center_axis',(0.,1.,1.77635683940025E-16));
#110102=DIRECTION('ref_axis',(-0.421146106069637,0.,0.906992809972815));
#110103=DIRECTION('center_axis',(0.,1.,2.22044604925031E-16));
#110104=DIRECTION('ref_axis',(-0.421146106069637,0.,0.906992809972815));
#110105=DIRECTION('',(0.,-1.,-1.77635683940025E-16));
#110106=DIRECTION('',(3.81426075461834E-28,1.,1.77635683940025E-16));
#110107=DIRECTION('center_axis',(6.93889390390723E-18,1.,2.22049474265475E-16));
#110108=DIRECTION('ref_axis',(-1.,6.93889390390723E-18,1.83750175990302E-19));
#110109=DIRECTION('',(1.,-6.93889390428186E-18,1.68718058920808E-12));
#110110=DIRECTION('',(0.,-2.46716227694479E-16,1.));
#110111=DIRECTION('center_axis',(-6.93889390390723E-18,-1.,-2.22049474265475E-16));
#110112=DIRECTION('ref_axis',(0.004256401731842,1.77634074823828E-16,-0.99999094148112));
#110113=DIRECTION('',(1.68710148498153E-12,2.22049474265463E-16,-1.));
#110114=DIRECTION('center_axis',(-1.,2.99689426160925E-28,-1.68710148498153E-12));
#110115=DIRECTION('ref_axis',(1.68710148498153E-12,2.22049474265463E-16,
-1.));
#110116=DIRECTION('',(-8.96831017167883E-44,-1.,-1.77635683940025E-16));
#110117=DIRECTION('',(0.,1.,1.77635683940025E-16));
#110118=DIRECTION('',(9.25185853854297E-17,0.,-1.));
#110119=DIRECTION('center_axis',(0.,-2.46716227694479E-16,1.));
#110120=DIRECTION('ref_axis',(1.,1.49541069999345E-33,0.));
#110121=DIRECTION('',(0.,-2.46716227694479E-16,1.));
#110122=DIRECTION('center_axis',(-1.68718058920808E-12,-1.77635683940025E-16,
1.));
#110123=DIRECTION('ref_axis',(1.,1.49541069999345E-33,0.));
#110124=DIRECTION('center_axis',(0.,2.22044604925031E-16,-1.));
#110125=DIRECTION('ref_axis',(1.,0.,0.));
#110126=DIRECTION('center_axis',(0.,-2.22044604925031E-16,1.));
#110127=DIRECTION('ref_axis',(1.,0.,0.));
#110128=DIRECTION('center_axis',(0.,2.22044604925031E-16,-1.));
#110129=DIRECTION('ref_axis',(1.,0.,0.));
#110130=DIRECTION('center_axis',(0.,-3.1720657846433E-16,1.));
#110131=DIRECTION('ref_axis',(1.,0.,0.));
#110132=DIRECTION('center_axis',(0.,-2.22044604925031E-16,1.));
#110133=DIRECTION('ref_axis',(1.,0.,0.));
#110134=DIRECTION('',(0.,-3.1720657846433E-16,1.));
#110135=DIRECTION('center_axis',(1.68684510810446E-12,0.,-1.));
#110136=DIRECTION('ref_axis',(-0.441505993976003,-0.897258300203047,-4.62840134152023E-13));
#110137=DIRECTION('center_axis',(-1.68718058920808E-12,-1.77635683940025E-16,
1.));
#110138=DIRECTION('ref_axis',(-0.441505993976003,-0.897258300203047,-7.45059728147159E-13));
#110139=DIRECTION('center_axis',(-1.,6.81117991896132E-28,-1.68711550397432E-12));
#110140=DIRECTION('ref_axis',(1.68711550397432E-12,2.22049474265463E-16,
-1.));
#110141=DIRECTION('',(-3.81426075461834E-28,-1.,-1.77635683940025E-16));
#110142=DIRECTION('',(1.68711550397432E-12,2.22044604925031E-16,-1.));
#110143=DIRECTION('center_axis',(3.81426075461834E-28,1.,1.77635683940025E-16));
#110144=DIRECTION('ref_axis',(-0.707106781185354,0.,-0.707106781187741));
#110145=DIRECTION('',(3.81426075461834E-28,1.,1.77635683940025E-16));
#110146=DIRECTION('center_axis',(0.,1.,2.22044604925031E-16));
#110147=DIRECTION('ref_axis',(-0.707106781185354,0.,-0.707106781187741));
#110148=DIRECTION('center_axis',(1.68718058920808E-12,1.77635683940025E-16,
-1.));
#110149=DIRECTION('ref_axis',(1.,2.21497401039684E-17,1.68718058920808E-12));
#110150=DIRECTION('',(-8.31844254296254E-44,-1.,-1.77635683940025E-16));
#110151=DIRECTION('',(1.,-3.7462934736789E-28,1.68718058920808E-12));
#110152=DIRECTION('center_axis',(1.68718058920808E-12,1.77635683940025E-16,
-1.));
#110153=DIRECTION('ref_axis',(-1.,7.0059776216349E-34,-1.68741283569787E-12));
#110154=DIRECTION('center_axis',(-9.25185853854297E-17,0.,1.));
#110155=DIRECTION('ref_axis',(-1.,7.0059776216349E-34,-9.25185853854297E-17));
#110156=DIRECTION('',(9.25185853854297E-17,0.,-1.));
#110157=DIRECTION('center_axis',(0.,-1.,-1.77635683940025E-16));
#110158=DIRECTION('ref_axis',(0.8003905296798,0.,-0.599478940413164));
#110159=DIRECTION('center_axis',(0.,-1.,-2.22044604925031E-16));
#110160=DIRECTION('ref_axis',(0.8003905296798,0.,-0.599478940413164));
#110161=DIRECTION('',(0.,1.,1.77635683940025E-16));
#110162=DIRECTION('center_axis',(0.,1.,2.22044604925031E-16));
#110163=DIRECTION('ref_axis',(0.8003905296798,0.,-0.599478940413164));
#110164=DIRECTION('center_axis',(0.,1.,2.22044604925031E-16));
#110165=DIRECTION('ref_axis',(-1.,0.,0.));
#110166=DIRECTION('center_axis',(0.,1.,2.22044604925031E-16));
#110167=DIRECTION('ref_axis',(0.718172954054269,0.,0.695864647805135));
#110168=DIRECTION('center_axis',(0.,-1.,-2.22044604925031E-16));
#110169=DIRECTION('ref_axis',(-0.910370950513196,7.3504420940774E-17,-0.413793103448693));
#110170=DIRECTION('center_axis',(3.81426075461834E-28,1.,1.77635683940025E-16));
#110171=DIRECTION('ref_axis',(0.70710678118774,0.,-0.707106781185355));
#110172=DIRECTION('center_axis',(0.,1.,2.22044604925031E-16));
#110173=DIRECTION('ref_axis',(0.70710678118774,0.,-0.707106781185355));
#110174=DIRECTION('center_axis',(0.,-1.,-1.77635683940025E-16));
#110175=DIRECTION('ref_axis',(-0.910370950513196,7.3504420940774E-17,-0.413793103448693));
#110176=DIRECTION('center_axis',(0.,1.,2.22044604925031E-16));
#110177=DIRECTION('ref_axis',(-0.910370950513196,7.3504420940774E-17,-0.413793103448693));
#110178=DIRECTION('',(0.,-1.,-1.77635683940025E-16));
#110179=DIRECTION('center_axis',(0.,-1.,-1.77635683940025E-16));
#110180=DIRECTION('ref_axis',(0.718172954054269,0.,0.695864647805135));
#110181=DIRECTION('center_axis',(0.,-1.,-2.22044604925031E-16));
#110182=DIRECTION('ref_axis',(0.718172954054269,0.,0.695864647805135));
#110183=DIRECTION('',(0.,1.,1.77635683940025E-16));
#110184=DIRECTION('center_axis',(1.,9.15104299692007E-33,7.93016446160826E-17));
#110185=DIRECTION('ref_axis',(-2.32378448758667E-32,1.,1.77635683940025E-16));
#110186=DIRECTION('',(-7.93016446160826E-17,-2.22044604925031E-16,1.));
#110187=DIRECTION('',(0.,1.,1.77635683940025E-16));
#110188=DIRECTION('',(0.,-1.,-2.22044604925031E-16));
#110189=DIRECTION('center_axis',(-7.93016446160826E-17,-2.22044604925031E-16,
1.));
#110190=DIRECTION('ref_axis',(-0.707106781186547,0.707106781186548,0.));
#110191=DIRECTION('',(7.93016446160826E-17,2.22044604925031E-16,-1.));
#110192=DIRECTION('center_axis',(-1.,-9.15104299692007E-33,-7.93016446160826E-17));
#110193=DIRECTION('ref_axis',(2.32378448758667E-32,-1.,-1.77635683940025E-16));
#110194=DIRECTION('',(7.93016446160826E-17,2.22044604925031E-16,-1.));
#110195=DIRECTION('',(0.,1.,2.22044604925031E-16));
#110196=DIRECTION('',(0.,-1.,-1.77635683940025E-16));
#110197=DIRECTION('center_axis',(0.,-1.,-1.77635683940025E-16));
#110198=DIRECTION('ref_axis',(0.004256401731842,1.77634074823828E-16,-0.99999094148112));
#110199=DIRECTION('center_axis',(0.,-1.,-2.22044604925031E-16));
#110200=DIRECTION('ref_axis',(0.004256401731842,1.77634074823828E-16,-0.99999094148112));
#110201=DIRECTION('center_axis',(0.,1.,1.77635683940025E-16));
#110202=DIRECTION('ref_axis',(0.418454579663818,0.,0.908237724804678));
#110203=DIRECTION('center_axis',(0.,1.,2.22044604925031E-16));
#110204=DIRECTION('ref_axis',(0.418454579663818,0.,0.908237724804678));
#110205=DIRECTION('center_axis',(1.,-4.93575888202656E-33,1.58603289232165E-16));
#110206=DIRECTION('ref_axis',(-2.32378448758667E-32,1.,1.77635683940025E-16));
#110207=DIRECTION('',(-1.58603289232165E-16,-2.22044604925031E-16,1.));
#110208=DIRECTION('',(0.,-1.,-2.22044604925031E-16));
#110209=DIRECTION('center_axis',(0.,1.,2.22044604925031E-16));
#110210=DIRECTION('ref_axis',(1.,-3.42114081564477E-49,1.54074485025198E-33));
#110211=DIRECTION('center_axis',(0.,1.,2.22044604925031E-16));
#110212=DIRECTION('ref_axis',(1.,0.,0.));
#110213=DIRECTION('center_axis',(1.83750175990302E-19,-1.,-2.22039735584453E-16));
#110214=DIRECTION('ref_axis',(1.,1.83750175990302E-19,1.58154558548465E-33));
#110215=DIRECTION('',(0.,1.,2.22044604925031E-16));
#110216=DIRECTION('center_axis',(1.83750175990302E-19,-1.,-2.22039735584453E-16));
#110217=DIRECTION('ref_axis',(1.,1.83750175990302E-19,1.58154558548465E-33));
#110218=DIRECTION('center_axis',(-1.,4.93575888202656E-33,-1.58603289232165E-16));
#110219=DIRECTION('ref_axis',(2.32378448758667E-32,-1.,-1.77635683940025E-16));
#110220=DIRECTION('',(1.58603289232165E-16,2.22044604925031E-16,-1.));
#110221=DIRECTION('center_axis',(0.,1.,2.22044604925031E-16));
#110222=DIRECTION('ref_axis',(0.16256157635468,2.19091056557869E-16,-0.986698400674229));
#110223=DIRECTION('center_axis',(0.,1.,2.22044604925031E-16));
#110224=DIRECTION('ref_axis',(0.16256157635468,2.19091056557869E-16,-0.986698400674229));
#110225=DIRECTION('center_axis',(0.,-1.,-2.22044604925031E-16));
#110226=DIRECTION('ref_axis',(0.16256157635468,2.19091056557869E-16,-0.986698400674229));
#110227=DIRECTION('center_axis',(0.,-1.,-2.22044604925031E-16));
#110228=DIRECTION('ref_axis',(0.16256157635468,2.19091056557869E-16,-0.986698400674229));
#110229=DIRECTION('center_axis',(-7.93016446160826E-17,-2.22044604925031E-16,
1.));
#110230=DIRECTION('ref_axis',(0.707106781186547,0.707106781186548,0.));
#110231=DIRECTION('',(-7.93016446160826E-17,-2.22044604925031E-16,1.));
#110232=DIRECTION('center_axis',(-1.58603289232165E-16,-2.22044604925031E-16,
1.));
#110233=DIRECTION('ref_axis',(-0.707106781186547,0.707106781186548,0.));
#110234=DIRECTION('',(1.58603289232165E-16,2.22044604925031E-16,-1.));
#110235=DIRECTION('center_axis',(1.58603289232165E-16,2.22044604925031E-16,
-1.));
#110236=DIRECTION('ref_axis',(0.707106781186548,0.707106781186548,0.));
#110237=DIRECTION('',(-1.58603289232165E-16,-2.22044604925031E-16,1.));
#110238=DIRECTION('center_axis',(0.,1.,2.22044604925031E-16));
#110239=DIRECTION('ref_axis',(1.,0.,0.));
#110240=DIRECTION('',(-1.,2.89708077091569E-28,-1.30472918803582E-12));
#110241=DIRECTION('center_axis',(0.,2.22044604925031E-16,-1.));
#110242=DIRECTION('ref_axis',(-1.,0.,0.));
#110243=DIRECTION('',(1.,0.,0.));
#110244=DIRECTION('',(1.,0.,0.));
#110245=DIRECTION('',(1.,0.,0.));
#110246=DIRECTION('',(-1.,0.,0.));
#110247=DIRECTION('center_axis',(0.,-1.,-2.66453525910038E-16));
#110248=DIRECTION('ref_axis',(-0.655931289920099,0.,-0.75482060312617));
#110249=DIRECTION('',(0.,1.,2.66453525910038E-16));
#110250=DIRECTION('center_axis',(0.,1.,2.22044604925031E-16));
#110251=DIRECTION('ref_axis',(-0.655931289920099,0.,-0.75482060312617));
#110252=DIRECTION('',(0.,-1.,0.));
#110253=DIRECTION('center_axis',(0.,-1.,0.));
#110254=DIRECTION('ref_axis',(-0.457833560950813,0.,0.889037924088224));
#110255=DIRECTION('',(0.,1.,0.));
#110256=DIRECTION('center_axis',(0.,1.,2.22044604925031E-16));
#110257=DIRECTION('ref_axis',(-0.457833560950813,0.,0.889037924088224));
#110258=DIRECTION('center_axis',(1.,0.,1.90323947078569E-14));
#110259=DIRECTION('ref_axis',(-8.85696131249311E-15,-2.22044604925031E-16,
1.));
#110260=DIRECTION('center_axis',(1.,-4.17479820231099E-30,1.88016196282748E-14));
#110261=DIRECTION('ref_axis',(-1.85037170770859E-14,-2.22044604925031E-16,
1.));
#110262=DIRECTION('center_axis',(-1.,4.17479820231099E-30,-1.88016196282748E-14));
#110263=DIRECTION('ref_axis',(0.,-2.22044604925031E-16,1.));
#110264=DIRECTION('center_axis',(0.,1.,2.22044604925031E-16));
#110265=DIRECTION('ref_axis',(0.900018102197426,-9.67786997242177E-17,0.435852516015388));
#110266=DIRECTION('',(0.,-1.,-2.22044604925031E-16));
#110267=DIRECTION('center_axis',(-4.16333634234434E-17,1.,2.28983498828938E-16));
#110268=DIRECTION('ref_axis',(-1.,0.,0.));
#110269=DIRECTION('center_axis',(0.,1.,2.22044604925031E-16));
#110270=DIRECTION('ref_axis',(-1.,0.,0.));
#110271=DIRECTION('center_axis',(0.,-1.,0.));
#110272=DIRECTION('ref_axis',(-0.301695932343328,0.,0.953404197813021));
#110273=DIRECTION('center_axis',(-4.16333634234434E-17,1.,2.28983498828938E-16));
#110274=DIRECTION('ref_axis',(-1.,-4.16333634234434E-17,-6.93889390390723E-17));
#110275=DIRECTION('center_axis',(4.16333634234434E-17,-1.,-2.28983498828938E-16));
#110276=DIRECTION('ref_axis',(-1.,-4.16333634234434E-17,-6.93889390390723E-17));
#110277=DIRECTION('center_axis',(-1.,4.1086505480261E-30,-1.85037170770859E-14));
#110278=DIRECTION('ref_axis',(-1.26584900907556E-14,-0.898717034276078,
0.438529009647037));
#110279=DIRECTION('',(-1.,4.1086505480261E-30,-1.85037170770859E-14));
#110280=DIRECTION('center_axis',(0.,-1.,-2.66453525910038E-16));
#110281=DIRECTION('ref_axis',(-0.436731370632223,-2.39699451904355E-16,
0.899591968564471));
#110282=DIRECTION('',(0.,-1.,-2.66453525910038E-16));
#110283=DIRECTION('center_axis',(0.,1.,0.));
#110284=DIRECTION('ref_axis',(-0.975463667519713,0.,-0.220160471813156));
#110285=DIRECTION('',(0.,1.,0.));
#110286=DIRECTION('center_axis',(0.,1.,2.22044604925031E-16));
#110287=DIRECTION('ref_axis',(-0.975463667519713,0.,-0.220160471813156));
#110288=DIRECTION('',(0.,-1.,0.));
#110289=DIRECTION('center_axis',(0.,-1.,0.));
#110290=DIRECTION('ref_axis',(0.988823617405683,0.,0.14909008572249));
#110291=DIRECTION('center_axis',(0.,1.,2.22044604925031E-16));
#110292=DIRECTION('ref_axis',(-0.805424049353576,0.,-0.59269899672843));
#110293=DIRECTION('',(0.,1.,0.));
#110294=DIRECTION('center_axis',(0.,-1.,0.));
#110295=DIRECTION('ref_axis',(-0.00362742930711492,0.,-0.999993420856668));
#110296=DIRECTION('center_axis',(0.,1.,2.22044604925031E-16));
#110297=DIRECTION('ref_axis',(-0.00362742930711492,0.,-0.999993420856668));
#110298=DIRECTION('',(0.,-1.,0.));
#110299=DIRECTION('center_axis',(0.,-1.,0.));
#110300=DIRECTION('ref_axis',(0.456803537809492,0.,0.889567607236646));
#110301=DIRECTION('center_axis',(0.,1.,2.22044604925031E-16));
#110302=DIRECTION('ref_axis',(0.456803537809492,0.,0.889567607236646));
#110303=DIRECTION('center_axis',(1.23192613759945E-16,0.,1.));
#110304=DIRECTION('ref_axis',(-1.,-1.83750175990341E-19,1.751211913973E-16));
#110305=DIRECTION('center_axis',(1.23192613759945E-16,-2.22049474265475E-16,
1.));
#110306=DIRECTION('ref_axis',(-1.,-1.83750175990352E-19,2.22044604925031E-16));
#110307=DIRECTION('',(-0.707106781186548,-8.67255366190364E-17,-0.707106781186547));
#110308=DIRECTION('center_axis',(-1.23192613759945E-16,2.22049474265475E-16,
-1.));
#110309=DIRECTION('ref_axis',(-1.,-1.8375017599033E-19,1.23192613759945E-16));
#110310=DIRECTION('center_axis',(1.23192613759945E-16,-2.22049474265475E-16,
1.));
#110311=DIRECTION('ref_axis',(-1.,-1.8375017599033E-19,1.23192613759945E-16));
#110312=DIRECTION('center_axis',(1.23192613759945E-16,-2.22049474265475E-16,
1.));
#110313=DIRECTION('ref_axis',(-1.,-1.8375017599033E-19,1.23192613759945E-16));
#110314=DIRECTION('center_axis',(2.22044604925031E-16,-2.22044604925031E-16,
1.));
#110315=DIRECTION('ref_axis',(-1.,-1.83750175990352E-19,2.22044604925031E-16));
#110316=DIRECTION('',(2.22044604925031E-16,-2.22044604925031E-16,1.));
#110317=DIRECTION('center_axis',(1.23192613759945E-16,-2.22049474265475E-16,
1.));
#110318=DIRECTION('ref_axis',(-1.,-1.83750175990336E-19,1.52923281628809E-16));
#110319=DIRECTION('center_axis',(1.23192613759944E-16,-2.22044604925031E-16,
1.));
#110320=DIRECTION('ref_axis',(-1.,-1.83750175990329E-19,1.17513135154478E-16));
#110321=DIRECTION('',(-0.832050294337844,2.11185235656057E-17,-0.554700196225229));
#110322=DIRECTION('center_axis',(-1.23192613759945E-16,2.22049474265475E-16,
-1.));
#110323=DIRECTION('ref_axis',(-1.,-1.83750175990327E-19,1.11022302462516E-16));
#110324=DIRECTION('center_axis',(0.,1.,2.22044604925031E-16));
#110325=DIRECTION('ref_axis',(-1.,0.,0.));
#110326=DIRECTION('center_axis',(0.,-1.,-2.22044604925031E-16));
#110327=DIRECTION('ref_axis',(-1.,0.,0.));
#110328=DIRECTION('',(0.,1.,2.22044604925031E-16));
#110329=DIRECTION('center_axis',(0.,-1.,-2.22044604925031E-16));
#110330=DIRECTION('ref_axis',(-1.,0.,0.));
#110331=DIRECTION('center_axis',(-1.,4.1086505480261E-30,-1.85037170770859E-14));
#110332=DIRECTION('ref_axis',(-1.85037170770859E-14,-2.22044604925031E-16,
1.));
#110333=DIRECTION('center_axis',(0.,1.,2.22044604925031E-16));
#110334=DIRECTION('ref_axis',(-1.,0.,0.));
#110335=DIRECTION('center_axis',(0.,-1.,-2.22044604925031E-16));
#110336=DIRECTION('ref_axis',(-1.,0.,0.));
#110337=DIRECTION('',(0.,1.,2.22044604925031E-16));
#110338=DIRECTION('center_axis',(4.16333634234434E-17,-1.,-2.28983498828938E-16));
#110339=DIRECTION('ref_axis',(-1.,0.,0.));
#110340=DIRECTION('center_axis',(0.,-1.,-2.66453525910038E-16));
#110341=DIRECTION('ref_axis',(-0.6562461524672,0.,-0.754546875529941));
#110342=DIRECTION('',(0.,1.,2.66453525910038E-16));
#110343=DIRECTION('center_axis',(1.,0.,2.2204460492513E-14));
#110344=DIRECTION('ref_axis',(-1.00566802662866E-14,-2.22044604925031E-16,
1.));
#110345=DIRECTION('center_axis',(1.,-4.17479820231099E-30,1.88016196282748E-14));
#110346=DIRECTION('ref_axis',(-1.88016196282748E-14,-2.22044604925031E-16,
1.));
#110347=DIRECTION('',(-0.707106781186359,-2.43604851491997E-16,0.707106781186736));
#110348=DIRECTION('center_axis',(-1.,4.17479820231099E-30,-1.88016196282748E-14));
#110349=DIRECTION('ref_axis',(0.,-2.22044604925031E-16,1.));
#110350=DIRECTION('center_axis',(-1.,0.,0.));
#110351=DIRECTION('ref_axis',(0.,-2.22044604925031E-16,1.));
#110352=DIRECTION('',(-1.,0.,0.));
#110353=DIRECTION('center_axis',(-1.,4.17479820231099E-30,-1.88016196282748E-14));
#110354=DIRECTION('ref_axis',(0.,-2.22044604925031E-16,1.));
#110355=DIRECTION('center_axis',(0.,1.,2.22044604925031E-16));
#110356=DIRECTION('ref_axis',(0.718181642132044,1.54510999792355E-16,-0.695855681089492));
#110357=DIRECTION('center_axis',(0.,-1.,-2.22044604925031E-16));
#110358=DIRECTION('ref_axis',(0.718181642132044,1.54510999792355E-16,-0.695855681089492));
#110359=DIRECTION('',(0.,-1.,-2.22044604925031E-16));
#110360=DIRECTION('center_axis',(0.,-1.,-2.22044604925031E-16));
#110361=DIRECTION('ref_axis',(0.718181642132044,1.54510999792355E-16,-0.695855681089492));
#110362=DIRECTION('',(0.,1.,2.22044604925031E-16));
#110363=DIRECTION('center_axis',(0.,1.,2.22044604925031E-16));
#110364=DIRECTION('ref_axis',(-0.911330049261084,-9.14105459778262E-17,
0.411676500803472));
#110365=DIRECTION('',(0.,-1.,-2.22044604925031E-16));
#110366=DIRECTION('center_axis',(0.,1.,2.22044604925031E-16));
#110367=DIRECTION('ref_axis',(-0.911330049261084,-9.14105459778262E-17,
0.411676500803472));
#110368=DIRECTION('',(0.,1.,2.22044604925031E-16));
#110369=DIRECTION('center_axis',(0.,-1.,-2.22044604925031E-16));
#110370=DIRECTION('ref_axis',(-0.911330049261084,-9.14105459778262E-17,
0.411676500803472));
#110371=DIRECTION('center_axis',(0.,1.,2.22044604925031E-16));
#110372=DIRECTION('ref_axis',(-0.0029658492688445,2.22043628341636E-16,
-0.999995601859385));
#110373=DIRECTION('',(0.,1.,2.22044604925031E-16));
#110374=DIRECTION('center_axis',(0.,-1.,-2.22044604925031E-16));
#110375=DIRECTION('ref_axis',(-0.0029658492688445,2.22043628341636E-16,
-0.999995601859385));
#110376=DIRECTION('center_axis',(0.,1.,2.22044604925031E-16));
#110377=DIRECTION('ref_axis',(-0.0029658492688445,2.22043628341636E-16,
-0.999995601859385));
#110378=DIRECTION('center_axis',(0.,1.,2.22044604925031E-16));
#110379=DIRECTION('ref_axis',(0.157787733663648,2.19263064006667E-16,-0.987473053356541));
#110380=DIRECTION('',(0.,-1.,-2.22044604925031E-16));
#110381=DIRECTION('center_axis',(0.,-1.,-2.22044604925031E-16));
#110382=DIRECTION('ref_axis',(0.157787733663648,2.19263064006667E-16,-0.987473053356541));
#110383=DIRECTION('center_axis',(0.495885766569122,1.92820817704139E-16,
-0.868387762761633));
#110384=DIRECTION('ref_axis',(-0.868387762761633,1.16830990166913E-16,-0.495885766569122));
#110385=DIRECTION('',(0.,1.,2.22044604925031E-16));
#110386=DIRECTION('',(0.868387762761633,-1.10108759125787E-16,0.495885766569122));
#110387=DIRECTION('center_axis',(0.,1.,2.22044604925031E-16));
#110388=DIRECTION('ref_axis',(2.55004895630733E-36,-2.22044604925031E-16,
1.));
#110389=DIRECTION('center_axis',(0.,-1.,-2.22044604925031E-16));
#110390=DIRECTION('ref_axis',(2.55004895630733E-36,-2.22044604925031E-16,
1.));
#110391=DIRECTION('',(0.,1.,2.22044604925031E-16));
#110392=DIRECTION('center_axis',(0.,-1.,-2.22044604925031E-16));
#110393=DIRECTION('ref_axis',(-0.788263422531444,-1.36632469114311E-16,
0.615337936989922));
#110394=DIRECTION('',(0.,-1.,-2.77555756156289E-16));
#110395=DIRECTION('center_axis',(0.,-1.,-2.22044604925031E-16));
#110396=DIRECTION('ref_axis',(-0.788263422531444,-1.36632469114311E-16,
0.615337936989922));
#110397=DIRECTION('',(0.,-1.,-2.22044604925031E-16));
#110398=DIRECTION('',(0.,-1.,-2.77555756156289E-16));
#110399=DIRECTION('center_axis',(-1.26161707343768E-16,2.22044604925031E-16,
-1.));
#110400=DIRECTION('ref_axis',(-1.,-1.8375017599033E-19,1.26161707343768E-16));
#110401=DIRECTION('center_axis',(-1.16253719856037E-16,2.22044604925031E-16,
-1.));
#110402=DIRECTION('ref_axis',(-1.,-1.8375017599033E-19,1.26161707343768E-16));
#110403=DIRECTION('',(-1.26161707343768E-16,2.22044604925031E-16,-1.));
#110404=DIRECTION('center_axis',(1.23192613759945E-16,-2.22049474265475E-16,
1.));
#110405=DIRECTION('ref_axis',(-1.,-1.8375017599033E-19,1.26161707343768E-16));
#110406=DIRECTION('center_axis',(1.,-4.94335532585216E-32,2.22628932034678E-16));
#110407=DIRECTION('ref_axis',(2.22628932034678E-16,2.22044604925031E-16,
-1.));
#110408=DIRECTION('',(0.,-1.,-2.77555756156289E-16));
#110409=DIRECTION('',(2.22628932034678E-16,2.22044604925031E-16,-1.));
#110410=DIRECTION('center_axis',(0.,1.,2.22044604925031E-16));
#110411=DIRECTION('ref_axis',(-0.819288030372914,1.27316419425093E-16,-0.573382179080996));
#110412=DIRECTION('',(0.,1.,2.22044604925031E-16));
#110413=DIRECTION('center_axis',(0.,-1.,-2.22044604925031E-16));
#110414=DIRECTION('ref_axis',(-0.819288030372914,1.27316419425093E-16,-0.573382179080996));
#110415=DIRECTION('center_axis',(0.,-1.,-2.22044604925031E-16));
#110416=DIRECTION('ref_axis',(-0.59469196781642,0.,0.80395364506583));
#110417=DIRECTION('center_axis',(0.,-1.,-2.22044604925031E-16));
#110418=DIRECTION('ref_axis',(-0.59469196781642,0.,0.80395364506583));
#110419=DIRECTION('',(7.36237927774606E-33,-1.,-2.52671446983656E-16));
#110420=DIRECTION('center_axis',(0.,1.,2.22044604925031E-16));
#110421=DIRECTION('ref_axis',(-1.,0.,0.));
#110422=DIRECTION('',(-0.308815713730942,0.707106781186545,0.636107581272894));
#110423=DIRECTION('center_axis',(0.,-1.,-2.22044604925031E-16));
#110424=DIRECTION('ref_axis',(-1.,0.,0.));
#110425=DIRECTION('center_axis',(0.,1.,2.22044604925031E-16));
#110426=DIRECTION('ref_axis',(-1.,0.,0.));
#110427=DIRECTION('',(0.308815713730941,0.707106781186548,-0.636107581272892));
#110428=DIRECTION('center_axis',(0.,1.,2.22044604925031E-16));
#110429=DIRECTION('ref_axis',(-1.,0.,0.));
#110430=DIRECTION('center_axis',(0.,-1.,-2.22044604925031E-16));
#110431=DIRECTION('ref_axis',(-0.398898296183895,0.,0.916995174088493));
#110432=DIRECTION('center_axis',(0.,-1.,-2.22044604925031E-16));
#110433=DIRECTION('ref_axis',(-0.398898296183895,0.,0.916995174088493));
#110434=DIRECTION('center_axis',(0.,1.,2.22044604925031E-16));
#110435=DIRECTION('ref_axis',(1.,0.,0.));
#110436=DIRECTION('center_axis',(0.,-1.,-2.22044604925031E-16));
#110437=DIRECTION('ref_axis',(1.,0.,0.));
#110438=DIRECTION('center_axis',(0.,1.,2.22044604925031E-16));
#110439=DIRECTION('ref_axis',(1.,0.,0.));
#110440=DIRECTION('center_axis',(0.,-1.,-2.22044604925031E-16));
#110441=DIRECTION('ref_axis',(1.,0.,0.));
#110442=DIRECTION('center_axis',(0.,-1.,-2.22044604925031E-16));
#110443=DIRECTION('ref_axis',(-1.,0.,-6.93889390390723E-17));
#110444=DIRECTION('center_axis',(0.,1.,2.22044604925031E-16));
#110445=DIRECTION('ref_axis',(1.,0.,0.));
#110446=DIRECTION('',(0.,-1.,-2.22044604925031E-16));
#110447=DIRECTION('center_axis',(0.,1.,2.22044604925031E-16));
#110448=DIRECTION('ref_axis',(1.,0.,0.));
#110449=DIRECTION('center_axis',(0.,-1.,0.));
#110450=DIRECTION('ref_axis',(-1.,0.,-6.93889390390723E-17));
#110451=DIRECTION('',(0.,-1.,0.));
#110452=DIRECTION('center_axis',(-4.16333634234434E-17,1.,2.28983498828938E-16));
#110453=DIRECTION('ref_axis',(-1.,0.,-6.93889390390723E-17));
#110454=DIRECTION('center_axis',(0.,-1.,-2.22044604925031E-16));
#110455=DIRECTION('ref_axis',(1.,0.,0.));
#110456=DIRECTION('center_axis',(-4.16333634234434E-17,1.,2.28983498828938E-16));
#110457=DIRECTION('ref_axis',(-1.,-4.16333634234434E-17,-6.93889390390723E-17));
#110458=DIRECTION('center_axis',(0.,-1.,-2.22044604925031E-16));
#110459=DIRECTION('ref_axis',(0.89959196856447,-9.69738446503996E-17,0.436731370632224));
#110460=DIRECTION('center_axis',(0.,-1.,-2.22044604925031E-16));
#110461=DIRECTION('ref_axis',(0.89959196856447,-9.69738446503996E-17,0.436731370632224));
#110462=DIRECTION('center_axis',(0.,1.,2.22044604925031E-16));
#110463=DIRECTION('ref_axis',(0.89959196856447,-9.69738446503996E-17,0.436731370632224));
#110464=DIRECTION('center_axis',(0.,1.,2.22044604925031E-16));
#110465=DIRECTION('ref_axis',(-0.436731370632224,-1.99749543253629E-16,
0.89959196856447));
#110466=DIRECTION('center_axis',(0.,-1.,-2.22044604925031E-16));
#110467=DIRECTION('ref_axis',(-0.436731370632224,-1.99749543253629E-16,
0.89959196856447));
#110468=DIRECTION('center_axis',(0.,1.,2.22044604925031E-16));
#110469=DIRECTION('ref_axis',(-0.436731370632224,-1.99749543253629E-16,
0.89959196856447));
#110470=DIRECTION('center_axis',(-1.,4.1086505480261E-30,-1.85037170770859E-14));
#110471=DIRECTION('ref_axis',(-1.85037170770859E-14,-2.22044604925031E-16,
1.));
#110472=DIRECTION('center_axis',(-1.,4.17479820231099E-30,-1.88016196282748E-14));
#110473=DIRECTION('ref_axis',(-1.85037170770859E-14,-2.22044604925031E-16,
1.));
#110474=DIRECTION('',(-1.,4.1086505480261E-30,-1.85037170770859E-14));
#110475=DIRECTION('center_axis',(1.,-4.17479820231099E-30,1.88016196282748E-14));
#110476=DIRECTION('ref_axis',(0.,1.,2.22044604925031E-16));
#110477=DIRECTION('center_axis',(-1.23192613759945E-16,2.22044604925031E-16,
-1.));
#110478=DIRECTION('ref_axis',(-1.,-1.8375017599033E-19,1.24462157223372E-16));
#110479=DIRECTION('',(0.464833898989921,2.53608975501167E-16,-0.885397902837944));
#110480=DIRECTION('center_axis',(1.23192613759945E-16,-2.22049474265475E-16,
1.));
#110481=DIRECTION('ref_axis',(0.,-1.,-2.22049474265475E-16));
#110482=DIRECTION('center_axis',(-1.23192613759945E-16,2.22049474265475E-16,
-1.));
#110483=DIRECTION('ref_axis',(-1.,-1.83750175990328E-19,1.14692461221607E-16));
#110484=DIRECTION('center_axis',(1.23192613759945E-16,-2.22049474265475E-16,
1.));
#110485=DIRECTION('ref_axis',(-1.,-2.73548551187854E-32,1.23192613759945E-16));
#110486=DIRECTION('center_axis',(1.23192613759945E-16,-2.22044604925031E-16,
1.));
#110487=DIRECTION('ref_axis',(-1.,-1.4920830064792E-32,6.7195971141788E-17));
#110488=DIRECTION('center_axis',(-1.23192613759945E-16,2.22049474265475E-16,
-1.));
#110489=DIRECTION('ref_axis',(-1.,0.,0.));
#110490=DIRECTION('',(0.554700196225232,-2.52683460863366E-16,0.832050294337842));
#110491=DIRECTION('center_axis',(-1.23192613759945E-16,2.22049474265475E-16,
-1.));
#110492=DIRECTION('ref_axis',(-1.,0.,0.));
#110493=DIRECTION('center_axis',(0.,-1.,0.));
#110494=DIRECTION('ref_axis',(-1.,0.,0.));
#110495=DIRECTION('center_axis',(0.,1.,2.22044604925031E-16));
#110496=DIRECTION('ref_axis',(-1.,0.,0.));
#110497=DIRECTION('center_axis',(0.,-1.,0.));
#110498=DIRECTION('ref_axis',(-1.,0.,0.));
#110499=DIRECTION('center_axis',(0.,1.,2.22044604925031E-16));
#110500=DIRECTION('ref_axis',(-1.,0.,0.));
#110501=DIRECTION('center_axis',(0.,-1.,0.));
#110502=DIRECTION('ref_axis',(0.97760907194103,0.,0.210429328893571));
#110503=DIRECTION('center_axis',(0.,-1.,-2.22044604925031E-16));
#110504=DIRECTION('ref_axis',(-1.,0.,0.));
#110505=DIRECTION('center_axis',(-1.11022302462516E-16,2.22044604925031E-16,
-1.));
#110506=DIRECTION('ref_axis',(-1.,-1.83750175990327E-19,1.11022302462516E-16));
#110507=DIRECTION('',(-1.11022302462516E-16,2.22044604925031E-16,-1.));
#110508=DIRECTION('center_axis',(2.22044604925031E-16,-2.22044604925031E-16,
1.));
#110509=DIRECTION('ref_axis',(0.805763256495856,0.592237768536584,-4.74121826153412E-17));
#110510=DIRECTION('center_axis',(1.23192613759945E-16,-2.22049474265475E-16,
1.));
#110511=DIRECTION('ref_axis',(-1.,-1.83750175990352E-19,2.22044604925031E-16));
#110512=DIRECTION('center_axis',(-2.22044604925031E-16,2.22044604925031E-16,
-1.));
#110513=DIRECTION('ref_axis',(-1.,-1.83750175990352E-19,2.22044604925031E-16));
#110514=DIRECTION('center_axis',(1.23192613759945E-16,-2.22049474265475E-16,
1.));
#110515=DIRECTION('ref_axis',(-1.,-1.83750175990352E-19,2.22044604925031E-16));
#110516=DIRECTION('center_axis',(-1.11022302462516E-16,2.22044604925031E-16,
-1.));
#110517=DIRECTION('ref_axis',(0.589037115720846,0.808105980860968,1.14039316434621E-16));
#110518=DIRECTION('center_axis',(1.23192613759945E-16,-2.22049474265475E-16,
1.));
#110519=DIRECTION('ref_axis',(-1.,-1.83750175990327E-19,1.11022302462516E-16));
#110520=DIRECTION('center_axis',(1.23192613759945E-16,-2.22049474265475E-16,
1.));
#110521=DIRECTION('ref_axis',(-1.,-1.83750175990327E-19,1.11022302462516E-16));
#110522=DIRECTION('center_axis',(1.23192613759945E-16,-2.22049474265475E-16,
1.));
#110523=DIRECTION('ref_axis',(-1.,-1.83750175990327E-19,1.11022302462516E-16));
#110524=DIRECTION('center_axis',(1.23192613759945E-16,0.,1.));
#110525=DIRECTION('ref_axis',(1.,1.64129130712712E-32,-7.39155682559668E-17));
#110526=DIRECTION('center_axis',(1.23192613759945E-16,0.,1.));
#110527=DIRECTION('ref_axis',(1.,1.64129130712712E-32,-7.39155682559668E-17));
#110528=DIRECTION('center_axis',(1.23192613759945E-16,-2.22049474265475E-16,
1.));
#110529=DIRECTION('ref_axis',(1.,0.,0.));
#110530=DIRECTION('center_axis',(0.,-2.22044604925031E-16,1.));
#110531=DIRECTION('ref_axis',(1.,0.,0.));
#110532=DIRECTION('center_axis',(-0.683267731943171,1.85374434656938E-16,
-0.730167930331944));
#110533=DIRECTION('ref_axis',(0.730167930331944,1.86856382700914E-16,-0.683267731943171));
#110534=DIRECTION('',(-2.53017617534078E-17,1.,2.77555756156289E-16));
#110535=DIRECTION('center_axis',(-0.683267731943171,1.85374434656938E-16,
-0.730167930331944));
#110536=DIRECTION('ref_axis',(0.730167930331944,-1.90208386519252E-14,-0.683267731943171));
#110537=DIRECTION('',(0.730167930331944,1.51715913597344E-16,-0.683267731943171));
#110538=DIRECTION('center_axis',(-2.53017617534078E-17,1.,2.77555756156289E-16));
#110539=DIRECTION('ref_axis',(-0.683267731943172,0.,-0.730167930331943));
#110540=DIRECTION('center_axis',(0.,1.,2.22044604925031E-16));
#110541=DIRECTION('ref_axis',(-0.683267731943172,0.,-0.730167930331943));
#110542=DIRECTION('center_axis',(2.44942954807913E-14,2.99934041219171E-16,
-1.));
#110543=DIRECTION('ref_axis',(1.,4.16333634234378E-17,2.44942954807913E-14));
#110544=DIRECTION('',(1.,-7.34667303037021E-30,2.44942954807913E-14));
#110545=DIRECTION('',(0.,-1.,-2.99934041219171E-16));
#110546=DIRECTION('',(1.,4.16333634234378E-17,2.44942954807913E-14));
#110547=DIRECTION('',(-8.62629387613302E-31,1.,2.99934041219171E-16));
#110548=DIRECTION('center_axis',(-1.,3.53805783332294E-31,-1.17961196366423E-15));
#110549=DIRECTION('ref_axis',(1.17961196366423E-15,2.28983498828939E-16,
-1.));
#110550=DIRECTION('',(-2.63976927864639E-32,-1.,-2.77555756156289E-16));
#110551=DIRECTION('',(1.17961196366423E-15,2.28983498828939E-16,-1.));
#110552=DIRECTION('',(0.,1.,2.99934041219171E-16));
#110553=DIRECTION('center_axis',(-1.,3.53805783332294E-31,-1.17961196366423E-15));
#110554=DIRECTION('ref_axis',(-1.40115152357497E-16,0.992920511302924,0.118780714907517));
#110555=DIRECTION('center_axis',(0.,-1.,-2.99934041219171E-16));
#110556=DIRECTION('ref_axis',(-0.707106781186541,0.,-0.707106781186554));
#110557=DIRECTION('center_axis',(0.,-1.,-2.22044604925031E-16));
#110558=DIRECTION('ref_axis',(-0.707106781186541,0.,-0.707106781186554));
#110559=DIRECTION('center_axis',(1.,-6.86520621803209E-30,2.57651168044591E-14));
#110560=DIRECTION('ref_axis',(2.57571741713036E-14,0.,-1.));
#110561=DIRECTION('center_axis',(2.14231643585101E-14,-0.555555555545262,
-0.831479419289976));
#110562=DIRECTION('ref_axis',(-1.41861830924326E-14,-0.831479419289976,
0.555555555545262));
#110563=DIRECTION('center_axis',(1.,-6.86520621803209E-30,2.57651168044591E-14));
#110564=DIRECTION('ref_axis',(1.97107954957864E-14,0.643991722633251,-0.765032457598929));
#110565=DIRECTION('center_axis',(-1.,0.,0.));
#110566=DIRECTION('ref_axis',(0.,0.640782340939398,-0.767722600644416));
#110567=DIRECTION('center_axis',(1.,-3.53805783332294E-31,1.17961196366423E-15));
#110568=DIRECTION('ref_axis',(-1.30104260698261E-16,0.992920511302924,0.118780714907517));
#110569=DIRECTION('',(-1.,0.,0.));
#110570=DIRECTION('',(-1.,0.,0.));
#110571=DIRECTION('center_axis',(-1.,0.,0.));
#110572=DIRECTION('ref_axis',(0.,-0.881917103691109,0.471404520785583));
#110573=DIRECTION('center_axis',(-1.,0.,0.));
#110574=DIRECTION('ref_axis',(0.,-0.881917103691109,0.471404520785584));
#110575=DIRECTION('center_axis',(-0.221755562098149,-0.912048152143364,
-0.344953096594898));
#110576=DIRECTION('ref_axis',(0.493196961917217,-0.410083123490685,0.767195274088514));
#110577=DIRECTION('center_axis',(0.,-1.,0.));
#110578=DIRECTION('ref_axis',(1.,0.,2.77555756156286E-14));
#110579=DIRECTION('center_axis',(1.,1.48359792176586E-14,2.22044604925059E-14));
#110580=DIRECTION('ref_axis',(-2.22044604925059E-14,0.,1.));
#110581=DIRECTION('center_axis',(-8.62629387613302E-31,1.,2.99934041219171E-16));
#110582=DIRECTION('ref_axis',(0.707106781186528,0.,0.707106781186567));
#110583=DIRECTION('center_axis',(0.,1.,2.22044604925031E-16));
#110584=DIRECTION('ref_axis',(0.707106781186528,0.,0.707106781186567));
#110585=DIRECTION('center_axis',(0.248654602219127,-0.206751184253524,-0.94626890290499));
#110586=DIRECTION('ref_axis',(0.72760687511296,-0.604990141980321,0.323380833376045));
#110587=DIRECTION('center_axis',(0.,-0.555555555565834,0.831479419276231));
#110588=DIRECTION('ref_axis',(0.,-0.831479419276231,-0.555555555565833));
#110589=DIRECTION('center_axis',(0.,-1.,0.));
#110590=DIRECTION('ref_axis',(1.,0.,0.));
#110591=DIRECTION('center_axis',(1.,0.,0.));
#110592=DIRECTION('ref_axis',(0.,-0.471404520796493,0.881917103685277));
#110593=DIRECTION('center_axis',(1.,1.85449740220717E-14,2.77555756156289E-14));
#110594=DIRECTION('ref_axis',(-2.77555756156289E-14,0.,1.));
#110595=DIRECTION('center_axis',(0.,-0.305555555545279,-0.952174250058998));
#110596=DIRECTION('ref_axis',(1.,0.,0.));
#110597=DIRECTION('center_axis',(-1.,3.53805783332294E-31,-1.17961196366423E-15));
#110598=DIRECTION('ref_axis',(-8.88178419700126E-16,0.,1.));
#110599=DIRECTION('center_axis',(-2.63976927864639E-32,-1.,-2.77555756156289E-16));
#110600=DIRECTION('ref_axis',(0.707106781186544,0.,0.707106781186551));
#110601=DIRECTION('center_axis',(0.,1.,2.22044604925031E-16));
#110602=DIRECTION('ref_axis',(0.707106781186544,0.,0.707106781186551));
#110603=DIRECTION('center_axis',(0.,1.,2.22044604925031E-16));
#110604=DIRECTION('ref_axis',(-1.,0.,0.));
#110605=DIRECTION('',(0.,1.,2.22044604925031E-16));
#110606=DIRECTION('center_axis',(-4.16333634234434E-17,1.,2.28983498828938E-16));
#110607=DIRECTION('ref_axis',(-1.,0.,0.));
#110608=DIRECTION('center_axis',(0.,1.,2.66453525910038E-16));
#110609=DIRECTION('ref_axis',(0.971814489841705,0.,-0.235746892521843));
#110610=DIRECTION('center_axis',(0.,-1.,-2.66453525910038E-16));
#110611=DIRECTION('ref_axis',(-0.436731370632223,-2.39699451904355E-16,
0.899591968564471));
#110612=DIRECTION('',(0.,-1.,-2.66453525910038E-16));
#110613=DIRECTION('center_axis',(0.,1.,2.22044604925031E-16));
#110614=DIRECTION('ref_axis',(-0.436731370632223,-2.39699451904355E-16,
0.899591968564471));
#110615=DIRECTION('',(0.,1.,2.66453525910038E-16));
#110616=DIRECTION('center_axis',(0.,1.,0.));
#110617=DIRECTION('ref_axis',(-0.301492073683253,-2.34187669256869E-17,
0.953468683023292));
#110618=DIRECTION('center_axis',(0.,-1.,-2.66453525910038E-16));
#110619=DIRECTION('ref_axis',(-0.659606396000608,0.,-0.751611204250635));
#110620=DIRECTION('center_axis',(-0.619186432486295,-0.785244014192337,
6.07756750723163E-15));
#110621=DIRECTION('ref_axis',(0.684676922246484,-0.539886523461806,0.489632570329433));
#110622=DIRECTION('center_axis',(1.26161707343768E-16,-2.22044604925031E-16,
1.));
#110623=DIRECTION('ref_axis',(-1.,-1.8375017599033E-19,1.26161707343768E-16));
#110624=DIRECTION('center_axis',(-1.26161707343768E-16,2.22044604925031E-16,
-1.));
#110625=DIRECTION('ref_axis',(0.69507377161985,0.718938420176691,0.));
#110626=DIRECTION('center_axis',(1.26161707343768E-16,-2.22044604925031E-16,
1.));
#110627=DIRECTION('ref_axis',(-1.,-1.8375017599033E-19,1.26161707343768E-16));
#110628=DIRECTION('center_axis',(-6.93889390390729E-17,0.,1.));
#110629=DIRECTION('ref_axis',(-1.,-2.65392283312903E-15,-6.93889390390729E-17));
#110630=DIRECTION('',(0.,-1.,0.));
#110631=DIRECTION('',(-1.,1.5407439555098E-32,-6.93889390390729E-17));
#110632=DIRECTION('',(0.,1.,0.));
#110633=DIRECTION('center_axis',(0.,-1.,0.));
#110634=DIRECTION('ref_axis',(0.707106781186547,0.,0.707106781186547));
#110635=DIRECTION('center_axis',(0.,1.,2.22044604925031E-16));
#110636=DIRECTION('ref_axis',(0.707106781186547,0.,0.707106781186547));
#110637=DIRECTION('center_axis',(0.,-1.,0.));
#110638=DIRECTION('ref_axis',(6.93889390390723E-17,0.,-1.));
#110639=DIRECTION('',(0.,-1.,0.));
#110640=DIRECTION('center_axis',(0.,1.,2.22044604925031E-16));
#110641=DIRECTION('ref_axis',(6.93889390390723E-17,0.,-1.));
#110642=DIRECTION('center_axis',(0.,-1.,-2.66453525910038E-16));
#110643=DIRECTION('ref_axis',(0.752694710045468,0.,-0.658369708803169));
#110644=DIRECTION('center_axis',(0.,1.,2.22044604925031E-16));
#110645=DIRECTION('ref_axis',(0.752694710045468,0.,-0.658369708803169));
#110646=DIRECTION('center_axis',(1.16253719856037E-16,-2.22044604925031E-16,
1.));
#110647=DIRECTION('ref_axis',(1.,2.58135112964991E-32,-1.16253719856037E-16));
#110648=DIRECTION('',(4.004083039641E-17,1.,2.22044604925031E-16));
#110649=DIRECTION('',(-1.,-2.58135112964991E-32,1.16253719856037E-16));
#110650=DIRECTION('',(0.,-1.,-2.22044604925031E-16));
#110651=DIRECTION('',(-1.,-1.83750175990151E-19,-6.09920703375441E-16));
#110652=DIRECTION('center_axis',(0.,1.,2.22044604925031E-16));
#110653=DIRECTION('ref_axis',(0.707106781186543,-1.57009245868379E-16,0.707106781186552));
#110654=DIRECTION('center_axis',(0.,-1.,-2.22044604925031E-16));
#110655=DIRECTION('ref_axis',(0.707106781186543,-1.57009245868379E-16,0.707106781186552));
#110656=DIRECTION('',(0.,1.,2.22044604925031E-16));
#110657=DIRECTION('center_axis',(0.,-1.,-2.22044604925031E-16));
#110658=DIRECTION('ref_axis',(0.707106781186543,-1.57009245868379E-16,0.707106781186552));
#110659=DIRECTION('center_axis',(0.,1.,2.22044604925031E-16));
#110660=DIRECTION('ref_axis',(-0.707106781186541,1.57009245868379E-16,-0.707106781186554));
#110661=DIRECTION('center_axis',(0.,1.,2.22044604925031E-16));
#110662=DIRECTION('ref_axis',(-0.707106781186541,1.57009245868379E-16,-0.707106781186554));
#110663=DIRECTION('',(0.,1.,2.22044604925031E-16));
#110664=DIRECTION('center_axis',(0.,1.,2.22044604925031E-16));
#110665=DIRECTION('ref_axis',(-0.707106781186541,1.57009245868379E-16,-0.707106781186554));
#110666=DIRECTION('',(0.,-1.,-2.22044604925031E-16));
#110667=DIRECTION('center_axis',(0.,2.22044604925031E-16,-1.));
#110668=DIRECTION('ref_axis',(-1.,0.,0.));
#110669=DIRECTION('',(1.,0.,0.));
#110670=DIRECTION('',(0.,-1.,-2.22044604925031E-16));
#110671=DIRECTION('',(1.,0.,0.));
#110672=DIRECTION('center_axis',(0.,-1.,-2.22044604925031E-16));
#110673=DIRECTION('ref_axis',(0.707106781186548,-1.57009245868377E-16,0.707106781186548));
#110674=DIRECTION('center_axis',(0.,-1.,-2.22044604925031E-16));
#110675=DIRECTION('ref_axis',(0.707106781186548,-1.57009245868377E-16,0.707106781186548));
#110676=DIRECTION('',(0.,1.,2.22044604925031E-16));
#110677=DIRECTION('center_axis',(0.,-1.,-2.22044604925031E-16));
#110678=DIRECTION('ref_axis',(0.707106781186548,-1.57009245868377E-16,0.707106781186548));
#110679=DIRECTION('center_axis',(0.,1.,2.22044604925031E-16));
#110680=DIRECTION('ref_axis',(0.89959196856447,-9.69738446503996E-17,0.436731370632224));
#110681=DIRECTION('center_axis',(0.,-1.,-2.22044604925031E-16));
#110682=DIRECTION('ref_axis',(0.89959196856447,-9.69738446503996E-17,0.436731370632224));
#110683=DIRECTION('center_axis',(0.,1.,2.22044604925031E-16));
#110684=DIRECTION('ref_axis',(0.89959196856447,-9.69738446503996E-17,0.436731370632224));
#110685=DIRECTION('center_axis',(0.,-1.,-2.22044604925031E-16));
#110686=DIRECTION('ref_axis',(1.,0.,0.));
#110687=DIRECTION('center_axis',(0.,1.,2.22044604925031E-16));
#110688=DIRECTION('ref_axis',(0.707106781186548,-1.57009245868377E-16,0.707106781186548));
#110689=DIRECTION('',(-1.88205007134457E-12,2.22044604925031E-16,-1.));
#110690=DIRECTION('center_axis',(0.,1.,2.22044604925031E-16));
#110691=DIRECTION('ref_axis',(-0.923879532511647,0.,-0.382683432364221));
#110692=DIRECTION('center_axis',(0.,-1.,0.));
#110693=DIRECTION('ref_axis',(-0.545776822909828,0.,0.837930581596384));
#110694=DIRECTION('',(4.17479820231099E-30,1.,7.84929678246568E-44));
#110695=DIRECTION('center_axis',(0.,1.,2.22044604925031E-16));
#110696=DIRECTION('ref_axis',(-0.545776822909828,0.,0.837930581596384));
#110697=DIRECTION('center_axis',(0.,1.,1.60901887626834E-16));
#110698=DIRECTION('ref_axis',(0.371940837143503,0.,0.92825643744872));
#110699=DIRECTION('center_axis',(4.05090206454524E-44,-1.,-2.22044604925031E-16));
#110700=DIRECTION('ref_axis',(-0.707106781185726,-1.5700924586856E-16,0.707106781187369));
#110701=DIRECTION('center_axis',(0.707106781185727,2.27549631693565E-16,
-0.707106781187368));
#110702=DIRECTION('ref_axis',(-0.707106781187368,1.61919227945235E-16,-0.707106781185727));
#110703=DIRECTION('',(8.41078048960407E-18,1.,2.77555756156289E-16));
#110704=DIRECTION('',(0.707106781187368,-1.57009245868195E-16,0.707106781185727));
#110705=DIRECTION('center_axis',(8.41078048960409E-18,1.,2.77555756156289E-16));
#110706=DIRECTION('ref_axis',(-0.382683432364555,0.,0.923879532511508));
#110707=DIRECTION('center_axis',(1.93528837224907E-48,1.,2.22044604925031E-16));
#110708=DIRECTION('ref_axis',(-0.707106781185727,-1.5700924586856E-16,0.707106781187368));
#110709=DIRECTION('center_axis',(0.683267731942997,-2.89517588606287E-16,
0.730167930332108));
#110710=DIRECTION('ref_axis',(-0.730167930332108,-1.86856382700881E-16,
0.683267731942997));
#110711=DIRECTION('',(0.730167930332109,1.51715913597305E-16,-0.683267731942995));
#110712=DIRECTION('',(-1.27117486340087E-16,-1.,-2.77555756156289E-16));
#110713=DIRECTION('',(-0.730167930332108,-1.51715913597305E-16,0.683267731942997));
#110714=DIRECTION('',(0.,-1.,-2.22044604925031E-16));
#110715=DIRECTION('center_axis',(-1.27117486340087E-16,-1.,-2.77555756156289E-16));
#110716=DIRECTION('ref_axis',(0.367309181526879,0.,0.930098900744461));
#110717=DIRECTION('center_axis',(-1.069105884037E-48,1.,2.22044604925031E-16));
#110718=DIRECTION('ref_axis',(-1.38777878078144E-15,-2.22044604925031E-16,
1.));
#110719=DIRECTION('center_axis',(0.,1.,2.22044604925031E-16));
#110720=DIRECTION('ref_axis',(0.367309181526879,0.,0.930098900744461));
#110721=DIRECTION('center_axis',(1.,4.28276345240491E-28,-1.88249434430459E-12));
#110722=DIRECTION('ref_axis',(-1.88249434430459E-12,2.22049474265623E-16,
-1.));
#110723=DIRECTION('',(1.88249434430459E-12,-2.22044604925031E-16,1.));
#110724=DIRECTION('',(0.,1.,2.27504718160893E-16));
#110725=DIRECTION('',(1.88249434430459E-12,-2.22044604925031E-16,1.));
#110726=DIRECTION('',(8.56552690482593E-29,-1.,-1.82003774528629E-16));
#110727=DIRECTION('',(7.83875492500777E-29,1.,2.69144975666705E-16));
#110728=DIRECTION('',(1.88259220622152E-12,-2.22049474265488E-16,1.));
#110729=DIRECTION('',(-1.02786322857718E-29,1.,2.22044604925031E-16));
#110730=DIRECTION('center_axis',(-8.56552690482593E-29,1.,1.82003774528629E-16));
#110731=DIRECTION('ref_axis',(-0.923879532510705,0.,0.382683432366494));
#110732=DIRECTION('center_axis',(0.,-1.,-2.22044604925031E-16));
#110733=DIRECTION('ref_axis',(-0.923879532510705,0.,0.382683432366494));
#110734=DIRECTION('',(-8.56552690482593E-29,1.,1.82003774528629E-16));
#110735=DIRECTION('center_axis',(0.707106781185727,1.28696103170951E-16,
-0.707106781187368));
#110736=DIRECTION('ref_axis',(-0.707106781187368,1.6191922794533E-16,-0.707106781185727));
#110737=DIRECTION('',(-4.004083039641E-17,-1.,-2.22044604925031E-16));
#110738=DIRECTION('',(0.707106781187368,-1.57009245868195E-16,0.707106781185727));
#110739=DIRECTION('center_axis',(4.004083039641E-17,1.,2.22044604925031E-16));
#110740=DIRECTION('ref_axis',(-0.382683432364554,0.,0.923879532511509));
#110741=DIRECTION('center_axis',(0.,-1.,-2.22044604925031E-16));
#110742=DIRECTION('ref_axis',(-0.382683432364554,0.,0.923879532511509));
#110743=DIRECTION('center_axis',(0.,-1.,-2.22044604925031E-16));
#110744=DIRECTION('ref_axis',(1.,0.,0.));
#110745=DIRECTION('center_axis',(0.,-1.,-2.22044604925031E-16));
#110746=DIRECTION('ref_axis',(0.923879532511287,0.,-0.38268343236509));
#110747=DIRECTION('',(-0.707106781186547,1.57009245868378E-16,-0.707106781186548));
#110748=DIRECTION('center_axis',(0.,-1.,-2.22044604925031E-16));
#110749=DIRECTION('ref_axis',(0.707106781186561,1.57009245868375E-16,-0.707106781186534));
#110750=DIRECTION('',(-3.65372513458554E-16,-2.22044604925031E-16,1.));
#110751=DIRECTION('',(-1.190587693968E-16,2.22044604925031E-16,-1.));
#110752=DIRECTION('center_axis',(1.,2.64363574135728E-32,-1.190587693968E-16));
#110753=DIRECTION('ref_axis',(-1.190587693968E-16,2.22044604925031E-16,
-1.));
#110754=DIRECTION('',(-6.50074362628842E-34,-1.,-2.27504718160893E-16));
#110755=DIRECTION('',(1.190587693968E-16,-2.22044604925031E-16,1.));
#110756=DIRECTION('center_axis',(6.50074362628842E-34,1.,2.27504718160893E-16));
#110757=DIRECTION('ref_axis',(0.923879532511287,0.,-0.38268343236509));
#110758=DIRECTION('center_axis',(0.,-1.,-2.22044604925031E-16));
#110759=DIRECTION('ref_axis',(0.923879532511287,0.,-0.38268343236509));
#110760=DIRECTION('',(6.50074362628842E-34,1.,2.27504718160893E-16));
#110761=DIRECTION('center_axis',(0.,1.,2.27504718160893E-16));
#110762=DIRECTION('ref_axis',(-0.923879532511647,0.,-0.382683432364221));
#110763=DIRECTION('',(0.,-1.,-2.27504718160893E-16));
#110764=DIRECTION('center_axis',(0.,1.,2.22044604925031E-16));
#110765=DIRECTION('ref_axis',(-0.923879532511647,0.,-0.382683432364221));
#110766=DIRECTION('center_axis',(0.,1.,2.22044604925031E-16));
#110767=DIRECTION('ref_axis',(-0.136414717731255,-2.19968891577408E-16,
0.990651818141118));
#110768=DIRECTION('',(0.,1.,2.22044604925031E-16));
#110769=DIRECTION('center_axis',(0.,1.,2.22044604925031E-16));
#110770=DIRECTION('ref_axis',(0.683267731942997,-1.62129849619521E-16,0.730167930332107));
#110771=DIRECTION('center_axis',(0.,-1.,-2.22044604925031E-16));
#110772=DIRECTION('ref_axis',(-0.136414717731255,-2.19968891577408E-16,
0.990651818141118));
#110773=DIRECTION('center_axis',(0.,1.,2.22044604925031E-16));
#110774=DIRECTION('ref_axis',(1.,0.,0.));
#110775=DIRECTION('center_axis',(0.,-1.,-2.22044604925031E-16));
#110776=DIRECTION('ref_axis',(-0.986133812836816,0.,-0.165952111104148));
#110777=DIRECTION('',(3.65372513458554E-16,2.22044604925031E-16,-1.));
#110778=DIRECTION('center_axis',(0.,-1.,-2.22044604925031E-16));
#110779=DIRECTION('ref_axis',(0.707106781186561,1.57009245868375E-16,-0.707106781186534));
#110780=DIRECTION('center_axis',(0.,-1.,-2.22044604925031E-16));
#110781=DIRECTION('ref_axis',(1.,0.,0.));
#110782=DIRECTION('center_axis',(0.,1.,2.22044604925031E-16));
#110783=DIRECTION('ref_axis',(-0.986133812836816,0.,-0.165952111104148));
#110784=DIRECTION('',(0.,-1.,-2.22044604925031E-16));
#110785=DIRECTION('center_axis',(0.,-1.,-2.22044604925031E-16));
#110786=DIRECTION('ref_axis',(-0.986133812836816,0.,-0.165952111104148));
#110787=DIRECTION('center_axis',(0.,1.,2.22044604925031E-16));
#110788=DIRECTION('ref_axis',(1.,0.,0.));
#110789=DIRECTION('center_axis',(0.,-1.,-2.22044604925031E-16));
#110790=DIRECTION('ref_axis',(-1.,0.,0.));
#110791=DIRECTION('center_axis',(0.,1.,2.22044604925031E-16));
#110792=DIRECTION('ref_axis',(1.,0.,0.));
#110793=DIRECTION('',(0.,-1.,-2.22044604925031E-16));
#110794=DIRECTION('center_axis',(0.,-1.,-2.22044604925031E-16));
#110795=DIRECTION('ref_axis',(-1.,0.,0.));
#110796=DIRECTION('center_axis',(0.,1.,2.22044604925031E-16));
#110797=DIRECTION('ref_axis',(-0.297808776285592,0.,-0.954625545838408));
#110798=DIRECTION('center_axis',(0.,-1.,-2.22044604925031E-16));
#110799=DIRECTION('ref_axis',(-0.297808776285592,0.,-0.954625545838408));
#110800=DIRECTION('center_axis',(0.,-1.,-2.22044604925031E-16));
#110801=DIRECTION('ref_axis',(-0.297808776285592,0.,-0.954625545838408));
#110802=DIRECTION('center_axis',(0.,1.,2.22044604925031E-16));
#110803=DIRECTION('ref_axis',(1.,0.,0.));
#110804=DIRECTION('center_axis',(0.,-1.,-2.22044604925031E-16));
#110805=DIRECTION('ref_axis',(-1.,0.,0.));
#110806=DIRECTION('center_axis',(0.,-1.,-2.22044604925031E-16));
#110807=DIRECTION('ref_axis',(-1.,0.,0.));
#110808=DIRECTION('',(0.,-1.,-2.22044604925031E-16));
#110809=DIRECTION('center_axis',(0.,1.,2.22044604925031E-16));
#110810=DIRECTION('ref_axis',(-1.,0.,0.));
#110811=DIRECTION('center_axis',(0.,1.,2.22044604925031E-16));
#110812=DIRECTION('ref_axis',(-1.,0.,0.));
#110813=DIRECTION('center_axis',(0.,1.,2.22044604925031E-16));
#110814=DIRECTION('ref_axis',(-1.,0.,0.));
#110815=DIRECTION('center_axis',(0.,1.,0.));
#110816=DIRECTION('ref_axis',(-1.,0.,0.));
#110817=DIRECTION('',(-0.707106781186548,-0.707106781186548,8.65956056235493E-17));
#110818=DIRECTION('center_axis',(-0.866025403784439,3.06268420586249E-17,
-0.5));
#110819=DIRECTION('ref_axis',(0.5,1.95761498617786E-16,-0.866025403784439));
#110820=DIRECTION('',(6.96245110587154E-17,-1.,-1.81846874723086E-16));
#110821=DIRECTION('',(-0.5,-1.92296268638356E-16,0.866025403784439));
#110822=DIRECTION('',(-7.52889106048643E-17,1.,1.91657902531386E-16));
#110823=DIRECTION('center_axis',(0.,1.,2.22044604925031E-16));
#110824=DIRECTION('ref_axis',(1.,0.,0.));
#110825=DIRECTION('center_axis',(0.,-1.,-2.22044604925031E-16));
#110826=DIRECTION('ref_axis',(0.641711497466635,0.,0.766946121979327));
#110827=DIRECTION('',(1.,2.73910036535074E-32,-1.2335811384724E-16));
#110828=DIRECTION('center_axis',(0.,-1.,-2.22044604925031E-16));
#110829=DIRECTION('ref_axis',(-0.641711497466635,0.,0.766946121979327));
#110830=DIRECTION('center_axis',(0.,1.,2.22044604925031E-16));
#110831=DIRECTION('ref_axis',(0.98683190526879,0.,-0.161749159947031));
#110832=DIRECTION('',(-2.10803227901262E-16,-2.22044604925031E-16,1.));
#110833=DIRECTION('center_axis',(0.,1.,2.22044604925031E-16));
#110834=DIRECTION('ref_axis',(0.707106781186547,0.,0.707106781186548));
#110835=DIRECTION('',(1.,-5.3377249763659E-32,2.40389762145677E-16));
#110836=DIRECTION('center_axis',(0.,-1.,-2.22044604925031E-16));
#110837=DIRECTION('ref_axis',(-0.59469196781642,0.,-0.80395364506583));
#110838=DIRECTION('center_axis',(0.,-1.,-2.22044604925031E-16));
#110839=DIRECTION('ref_axis',(-0.650397979794319,0.,-0.759593620220357));
#110840=DIRECTION('',(-1.,-2.73910036535074E-32,1.2335811384724E-16));
#110841=DIRECTION('center_axis',(0.,-1.,-2.22044604925031E-16));
#110842=DIRECTION('ref_axis',(0.650397979794315,0.,-0.759593620220361));
#110843=DIRECTION('center_axis',(0.,1.,2.22044604925031E-16));
#110844=DIRECTION('ref_axis',(-0.707106781186548,0.,-0.707106781186548));
#110845=DIRECTION('',(-1.,5.3377249763659E-32,-2.40389762145677E-16));
#110846=DIRECTION('center_axis',(0.,-1.,-2.22044604925031E-16));
#110847=DIRECTION('ref_axis',(0.707106781186547,0.,-0.707106781186548));
#110848=DIRECTION('',(2.41949676183277E-16,2.22044604925031E-16,-1.));
#110849=DIRECTION('center_axis',(0.,-1.,-2.22044604925031E-16));
#110850=DIRECTION('ref_axis',(-1.,1.45619093356108E-31,-6.0908498285001E-16));
#110851=DIRECTION('center_axis',(0.,-1.,-2.22044604925031E-16));
#110852=DIRECTION('ref_axis',(0.664346409066274,0.,-0.747424811443096));
#110853=DIRECTION('center_axis',(0.,-1.,-2.22044604925031E-16));
#110854=DIRECTION('ref_axis',(0.707106781186561,1.57009245868375E-16,-0.707106781186534));
#110855=DIRECTION('center_axis',(0.,1.,2.22044604925031E-16));
#110856=DIRECTION('ref_axis',(0.707106781186548,-1.57009245868377E-16,0.707106781186548));
#110857=DIRECTION('center_axis',(7.52889106048643E-17,-1.,-1.91657902531386E-16));
#110858=DIRECTION('ref_axis',(-0.945459087052696,0.,0.325740870492916));
#110859=DIRECTION('center_axis',(0.,1.,2.22044604925031E-16));
#110860=DIRECTION('ref_axis',(-0.945459087052696,0.,0.325740870492916));
#110861=DIRECTION('center_axis',(0.,-2.22044604925031E-16,1.));
#110862=DIRECTION('ref_axis',(1.,0.,0.));
#110863=DIRECTION('center_axis',(0.,0.880412421871567,0.474208780406102));
#110864=DIRECTION('ref_axis',(0.,0.474208780406102,-0.880412421871567));
#110865=DIRECTION('center_axis',(-3.94297421746172E-16,-0.913923057046371,
0.405887479234104));
#110866=DIRECTION('ref_axis',(0.,-0.405887479234104,-0.913923057046371));
#110867=DIRECTION('',(0.,-2.22044604925031E-16,1.));
#110868=DIRECTION('center_axis',(2.37859513600921E-17,-0.866025403784432,
-0.500000000000011));
#110869=DIRECTION('ref_axis',(1.586190700722E-16,-0.500000000000011,0.866025403784432));
#110870=DIRECTION('center_axis',(-2.37859513600921E-17,0.866025403784432,
0.500000000000011));
#110871=DIRECTION('ref_axis',(0.,-0.500000000000011,0.866025403784432));
#110872=DIRECTION('center_axis',(2.37859513600921E-17,-0.866025403784432,
-0.500000000000011));
#110873=DIRECTION('ref_axis',(0.,-0.500000000000011,0.866025403784432));
#110874=DIRECTION('',(-1.,-9.86864910777917E-17,1.2335811384724E-16));
#110875=DIRECTION('center_axis',(2.37859513600921E-17,-0.866025403784432,
-0.500000000000011));
#110876=DIRECTION('ref_axis',(-3.0046291974743E-16,-0.500000000000011,0.866025403784432));
#110877=DIRECTION('center_axis',(1.2335811384724E-16,1.06734344607313E-15,
1.));
#110878=DIRECTION('ref_axis',(-1.11022302462516E-16,1.,-1.06734344607313E-15));
#110879=DIRECTION('',(1.59056477988302E-31,-1.,1.06734344607313E-15));
#110880=DIRECTION('',(-1.,-2.73910036535073E-32,1.2335811384724E-16));
#110881=DIRECTION('',(-1.59056477988302E-31,1.,-1.06734344607313E-15));
#110882=DIRECTION('',(-1.,-9.86864910777917E-17,1.2335811384724E-16));
#110883=DIRECTION('center_axis',(-1.2335811384724E-16,4.26937378429254E-16,
-1.));
#110884=DIRECTION('ref_axis',(1.11022302462516E-16,-1.,-4.26937378429254E-16));
#110885=DIRECTION('',(2.52751860804106E-32,1.,4.26937378429254E-16));
#110886=DIRECTION('',(-1.,-9.86864910777917E-17,1.2335811384724E-16));
#110887=DIRECTION('',(-2.52751860804106E-32,-1.,-4.26937378429254E-16));
#110888=DIRECTION('',(1.,2.73910036535074E-32,-1.2335811384724E-16));
#110889=DIRECTION('center_axis',(-1.51594548245566E-16,0.819152044288998,
-0.573576436351038));
#110890=DIRECTION('ref_axis',(-3.3847457739984E-17,-0.573576436351038,-0.819152044288998));
#110891=DIRECTION('center_axis',(1.51594548245566E-16,-0.819152044288998,
0.573576436351038));
#110892=DIRECTION('ref_axis',(9.28221823687422E-33,0.573576436351038,0.819152044288998));
#110893=DIRECTION('center_axis',(-1.51594548245566E-16,0.819152044288998,
-0.573576436351038));
#110894=DIRECTION('ref_axis',(2.13150342243378E-16,0.573576436351038,0.819152044288998));
#110895=DIRECTION('center_axis',(-1.51594548245566E-16,0.819152044288998,
-0.573576436351038));
#110896=DIRECTION('ref_axis',(2.13150342243378E-16,0.573576436351038,0.819152044288998));
#110897=DIRECTION('center_axis',(-1.2335811384724E-16,6.93700665664735E-16,
-1.));
#110898=DIRECTION('ref_axis',(1.11022302462516E-16,-1.,-6.93700665664735E-16));
#110899=DIRECTION('',(-5.8182602037469E-32,-1.,-6.93700665664735E-16));
#110900=DIRECTION('',(5.8182602037469E-32,1.,6.93700665664735E-16));
#110901=DIRECTION('center_axis',(0.,1.,2.22044604925031E-16));
#110902=DIRECTION('ref_axis',(-0.641711497466635,0.,0.766946121979327));
#110903=DIRECTION('center_axis',(0.,-1.,-2.22044604925031E-16));
#110904=DIRECTION('ref_axis',(0.641711497466635,0.,0.766946121979327));
#110905=DIRECTION('center_axis',(0.,-1.,-2.22044604925031E-16));
#110906=DIRECTION('ref_axis',(0.641711497466635,0.,0.766946121979327));
#110907=DIRECTION('center_axis',(0.,-1.,-2.22044604925031E-16));
#110908=DIRECTION('ref_axis',(0.641711497466635,0.,0.766946121979327));
#110909=DIRECTION('center_axis',(0.,1.,2.22044604925031E-16));
#110910=DIRECTION('ref_axis',(-0.641711497466633,0.,0.766946121979329));
#110911=DIRECTION('center_axis',(0.,-1.,-2.22044604925031E-16));
#110912=DIRECTION('ref_axis',(-0.641711497466633,0.,0.766946121979329));
#110913=DIRECTION('center_axis',(0.,1.,2.22044604925031E-16));
#110914=DIRECTION('ref_axis',(0.650397979794315,0.,-0.759593620220361));
#110915=DIRECTION('center_axis',(0.,-1.,-2.22044604925031E-16));
#110916=DIRECTION('ref_axis',(0.650397979794315,0.,-0.759593620220361));
#110917=DIRECTION('center_axis',(-1.00839335745948E-17,0.819152044288994,
0.573576436351042));
#110918=DIRECTION('ref_axis',(0.,0.573576436351042,-0.819152044288994));
#110919=DIRECTION('center_axis',(0.,-1.,-2.22044604925031E-16));
#110920=DIRECTION('ref_axis',(-0.650397979794316,0.,-0.75959362022036));
#110921=DIRECTION('center_axis',(0.,-1.,-2.22044604925031E-16));
#110922=DIRECTION('ref_axis',(-0.650397979794316,0.,-0.75959362022036));
#110923=DIRECTION('center_axis',(-1.00839335745948E-17,0.819152044288994,
0.573576436351042));
#110924=DIRECTION('ref_axis',(-1.42100228162251E-16,0.573576436351042,-0.819152044288995));
#110925=DIRECTION('center_axis',(1.2335811384724E-16,-1.72794927465785E-15,
1.));
#110926=DIRECTION('ref_axis',(-1.11022302462516E-16,1.,1.72794927465785E-15));
#110927=DIRECTION('',(-1.85765559691991E-31,-1.,-1.72794927465785E-15));
#110928=DIRECTION('',(-1.,-9.86864910777917E-17,1.2335811384724E-16));
#110929=DIRECTION('',(1.85765559691991E-31,1.,1.72794927465785E-15));
#110930=DIRECTION('center_axis',(0.,-1.,-2.22044604925031E-16));
#110931=DIRECTION('ref_axis',(-0.650397979794319,0.,-0.759593620220357));
#110932=DIRECTION('center_axis',(1.47144065207334E-16,-0.866025403784436,
0.500000000000005));
#110933=DIRECTION('ref_axis',(-3.75578649684289E-16,-0.500000000000005,
-0.866025403784436));
#110934=DIRECTION('center_axis',(0.,1.,2.22044604925031E-16));
#110935=DIRECTION('ref_axis',(0.650397979794315,0.,-0.759593620220361));
#110936=DIRECTION('center_axis',(1.47144065207334E-16,-0.866025403784436,
0.500000000000005));
#110937=DIRECTION('ref_axis',(-7.51157299368577E-17,-0.500000000000005,
-0.866025403784436));
#110938=DIRECTION('center_axis',(1.47144065207334E-16,-0.866025403784436,
0.500000000000005));
#110939=DIRECTION('ref_axis',(4.7596767609683E-17,0.500000000000005,0.866025403784436));
#110940=DIRECTION('center_axis',(-1.47144065207334E-16,0.866025403784436,
-0.500000000000005));
#110941=DIRECTION('ref_axis',(0.,-0.500000000000005,-0.866025403784436));
#110942=DIRECTION('center_axis',(0.,-0.913923057046369,-0.40588747923411));
#110943=DIRECTION('ref_axis',(0.,-0.40588747923411,0.913923057046369));
#110944=DIRECTION('center_axis',(0.736991631393267,0.387681384808809,0.553666396965732));
#110945=DIRECTION('ref_axis',(0.,-0.819152044288996,0.57357643635104));
#110946=DIRECTION('center_axis',(0.,0.880412421871569,-0.474208780406097));
#110947=DIRECTION('ref_axis',(0.,0.474208780406097,0.880412421871569));
#110948=DIRECTION('center_axis',(-1.00839335745948E-17,0.819152044288994,
0.573576436351042));
#110949=DIRECTION('ref_axis',(-1.61207010943858E-16,0.573576436351042,-0.819152044288994));
#110950=DIRECTION('center_axis',(1.00839335745948E-17,-0.819152044288994,
-0.573576436351042));
#110951=DIRECTION('ref_axis',(-6.17444843556704E-34,0.573576436351042,-0.819152044288995));
#110952=DIRECTION('center_axis',(0.,1.,2.22044604925031E-16));
#110953=DIRECTION('ref_axis',(0.664346409066274,0.,-0.747424811443096));
#110954=DIRECTION('center_axis',(0.,-1.,-2.22044604925031E-16));
#110955=DIRECTION('ref_axis',(0.664346409066274,0.,-0.747424811443096));
#110956=DIRECTION('',(0.,-1.,-2.22044604925031E-16));
#110957=DIRECTION('center_axis',(4.78544407166016E-17,-1.,-6.12536841172497E-17));
#110958=DIRECTION('ref_axis',(-0.707106781186548,0.,-0.707106781186548));
#110959=DIRECTION('',(-4.78544407166016E-17,1.,6.12536841172497E-17));
#110960=DIRECTION('center_axis',(-4.30715231393665E-32,-1.,-6.12536841172497E-17));
#110961=DIRECTION('ref_axis',(0.707106781186547,0.,-0.707106781186548));
#110962=DIRECTION('',(4.30715231393665E-32,1.,6.12536841172497E-17));
#110963=DIRECTION('',(-4.30715231393665E-32,-1.,-6.12536841172497E-17));
#110964=DIRECTION('center_axis',(2.40389762145677E-16,6.12536841172497E-17,
-1.));
#110965=DIRECTION('ref_axis',(1.,6.93889390390718E-18,2.40389762145677E-16));
#110966=DIRECTION('center_axis',(0.,-1.,-2.22044604925031E-16));
#110967=DIRECTION('ref_axis',(-0.398898296183895,0.,-0.916995174088493));
#110968=DIRECTION('center_axis',(0.,-1.,-2.22044604925031E-16));
#110969=DIRECTION('ref_axis',(-0.398898296183895,0.,-0.916995174088493));
#110970=DIRECTION('center_axis',(0.,1.,2.69144975666705E-16));
#110971=DIRECTION('ref_axis',(0.877755401836952,0.,-0.479109021566127));
#110972=DIRECTION('',(9.91356230361479E-29,-1.,-2.69144975666705E-16));
#110973=DIRECTION('center_axis',(0.,-1.,-2.22044604925031E-16));
#110974=DIRECTION('ref_axis',(0.877755401836952,0.,-0.479109021566127));
#110975=DIRECTION('',(0.,1.,2.69144975666705E-16));
#110976=DIRECTION('center_axis',(0.,1.,2.69144975666705E-16));
#110977=DIRECTION('ref_axis',(-0.674528301887451,-1.98696006215612E-16,
0.738248989130924));
#110978=DIRECTION('',(0.,-1.,-2.69144975666705E-16));
#110979=DIRECTION('center_axis',(0.,1.,2.22044604925031E-16));
#110980=DIRECTION('ref_axis',(-0.674528301887451,-1.98696006215612E-16,
0.738248989130924));
#110981=DIRECTION('center_axis',(0.,1.,2.69144975666705E-16));
#110982=DIRECTION('ref_axis',(-0.439524536496337,0.,-0.898230583880153));
#110983=DIRECTION('center_axis',(0.,-1.,-2.22044604925031E-16));
#110984=DIRECTION('ref_axis',(-0.439524536496337,0.,-0.898230583880153));
#110985=DIRECTION('center_axis',(0.,1.,2.22044604925031E-16));
#110986=DIRECTION('ref_axis',(1.,0.,0.));
#110987=DIRECTION('center_axis',(0.,-1.,-2.22044604925031E-16));
#110988=DIRECTION('ref_axis',(-0.385275875185828,0.,-0.922801441264476));
#110989=DIRECTION('',(-1.88260317010131E-12,2.22044604925031E-16,-1.));
#110990=DIRECTION('center_axis',(0.,1.,2.22044604925031E-16));
#110991=DIRECTION('ref_axis',(0.707106781186561,1.57009245868375E-16,-0.707106781186534));
#110992=DIRECTION('center_axis',(0.,1.,2.22044604925031E-16));
#110993=DIRECTION('ref_axis',(-0.385275875185828,0.,-0.922801441264476));
#110994=DIRECTION('center_axis',(0.,-1.,-2.22044604925031E-16));
#110995=DIRECTION('ref_axis',(-0.385275875185828,0.,-0.922801441264476));
#110996=DIRECTION('center_axis',(0.,-1.,-2.22044604925031E-16));
#110997=DIRECTION('ref_axis',(-0.59469196781642,0.,-0.80395364506583));
#110998=DIRECTION('center_axis',(-2.40389762145677E-16,-2.52671446983656E-16,
1.));
#110999=DIRECTION('ref_axis',(-1.,-6.93889390390718E-18,-2.40389762145677E-16));
#111000=DIRECTION('',(-4.78544407166016E-17,1.,2.52671446983656E-16));
#111001=DIRECTION('center_axis',(4.78544407166016E-17,-1.,-2.52671446983656E-16));
#111002=DIRECTION('ref_axis',(0.707106781186547,0.,0.707106781186548));
#111003=DIRECTION('',(4.78544407166016E-17,-1.,-2.52671446983656E-16));
#111004=DIRECTION('center_axis',(-1.,-4.78544407166015E-17,-2.10803227901262E-16));
#111005=DIRECTION('ref_axis',(2.10803227901262E-16,2.28983498828939E-16,
-1.));
#111006=DIRECTION('',(-4.78544407166015E-17,1.,7.99864431349418E-17));
#111007=DIRECTION('center_axis',(-4.78544407166015E-17,1.,7.99864431349418E-17));
#111008=DIRECTION('ref_axis',(0.98683190526879,0.,-0.161749159947031));
#111009=DIRECTION('center_axis',(0.,-1.,-2.22044604925031E-16));
#111010=DIRECTION('ref_axis',(0.707106781186548,-1.57009245868377E-16,0.707106781186548));
#111011=DIRECTION('center_axis',(0.,-1.,-2.39272203583008E-16));
#111012=DIRECTION('ref_axis',(-1.,1.45619093356108E-31,-6.0908498285001E-16));
#111013=DIRECTION('',(0.,-1.,-2.39272203583008E-16));
#111014=DIRECTION('center_axis',(1.,-5.78918321765678E-32,2.41949676183277E-16));
#111015=DIRECTION('ref_axis',(-2.41949676183277E-16,-2.22049474265475E-16,
1.));
#111016=DIRECTION('center_axis',(0.,-1.,-2.22044604925031E-16));
#111017=DIRECTION('ref_axis',(0.707106781186561,1.57009245868375E-16,-0.707106781186534));
#111018=DIRECTION('',(0.,-1.,-2.22044604925031E-16));
#111019=DIRECTION('center_axis',(1.,-4.17479820231099E-30,1.88016196282748E-14));
#111020=DIRECTION('ref_axis',(-1.88016196282748E-14,-2.22044604925031E-16,
1.));
#111021=DIRECTION('',(-1.88016196282748E-14,-2.22044604925031E-16,1.));
#111022=DIRECTION('center_axis',(1.,6.05828807443126E-28,-1.88260317010131E-12));
#111023=DIRECTION('ref_axis',(-1.88260317010131E-12,2.22049474265488E-16,
-1.));
#111024=DIRECTION('',(-8.96831017167883E-44,1.,3.21803775253669E-16));
#111025=DIRECTION('center_axis',(0.,1.,3.21803775253669E-16));
#111026=DIRECTION('ref_axis',(-0.923879532510705,0.,0.382683432366495));
#111027=DIRECTION('center_axis',(-1.23192613759945E-16,2.22044604925031E-16,
-1.));
#111028=DIRECTION('ref_axis',(0.555094454892529,0.831787320261355,1.17579893590648E-16));
#111029=DIRECTION('center_axis',(1.23192613759945E-16,0.,1.));
#111030=DIRECTION('ref_axis',(0.791958354931176,0.610575109265604,-1.02206428667277E-16));
#111031=DIRECTION('center_axis',(6.93889390390722E-18,1.,2.22049474265475E-16));
#111032=DIRECTION('ref_axis',(-1.,6.93889390390721E-18,1.83750175990302E-19));
#111033=DIRECTION('center_axis',(0.808736084303188,0.,-0.588171697675047));
#111034=DIRECTION('ref_axis',(-0.588171697675046,-5.25462354708949E-17,
-0.808736084303188));
#111035=DIRECTION('center_axis',(-0.707106781186548,-1.60870128963501E-16,
0.707106781186547));
#111036=DIRECTION('ref_axis',(0.707106781186547,-1.61919227945507E-16,0.707106781186548));
#111037=DIRECTION('',(-0.707106781186547,1.57009245868378E-16,-0.707106781186548));
#111038=DIRECTION('',(-6.34155293819033E-44,-1.,-2.27504718160893E-16));
#111039=DIRECTION('',(-0.707106781186547,1.57009245868378E-16,-0.707106781186547));
#111040=DIRECTION('center_axis',(6.34155293819033E-44,1.,2.27504718160893E-16));
#111041=DIRECTION('ref_axis',(-0.923879532510926,0.,0.38268343236596));
#111042=DIRECTION('center_axis',(0.,1.,2.22044604925031E-16));
#111043=DIRECTION('ref_axis',(-0.923879532510926,0.,0.38268343236596));
#111044=DIRECTION('',(0.,1.,2.77555756156289E-16));
#111045=DIRECTION('center_axis',(4.32964835625641E-44,-1.,-2.22044604925031E-16));
#111046=DIRECTION('ref_axis',(-1.,-4.17772723536479E-28,1.88148108204444E-12));
#111047=DIRECTION('center_axis',(-1.,-4.28175312849965E-28,1.88205025509474E-12));
#111048=DIRECTION('ref_axis',(1.88205025509474E-12,-2.22049474265623E-16,
1.));
#111049=DIRECTION('',(-1.88205025509474E-12,2.22044604925031E-16,-1.));
#111050=DIRECTION('',(-1.88221415680549E-12,2.22044604925031E-16,-1.));
#111051=DIRECTION('center_axis',(0.,-1.,-2.77555756156289E-16));
#111052=DIRECTION('ref_axis',(-1.,0.,0.));
#111053=DIRECTION('center_axis',(-4.3296825676447E-44,1.,2.22044604925031E-16));
#111054=DIRECTION('ref_axis',(-1.,-4.3296825676447E-44,-9.61382655183462E-60));
#111055=DIRECTION('center_axis',(0.,-2.22044604925031E-16,1.));
#111056=DIRECTION('ref_axis',(1.,0.,0.));
#111057=DIRECTION('',(0.,-2.22044604925031E-16,1.));
#111058=DIRECTION('center_axis',(0.,-1.,-2.22044604925031E-16));
#111059=DIRECTION('ref_axis',(1.,0.,0.));
#111060=DIRECTION('center_axis',(0.,1.,2.22044604925031E-16));
#111061=DIRECTION('ref_axis',(0.923879532510927,0.,-0.382683432365958));
#111062=DIRECTION('center_axis',(0.,1.,2.27504718160893E-16));
#111063=DIRECTION('ref_axis',(0.923879532510927,0.,-0.382683432365958));
#111064=DIRECTION('center_axis',(0.,-1.,-2.22044604925031E-16));
#111065=DIRECTION('ref_axis',(0.923879532510927,0.,-0.382683432365958));
#111066=DIRECTION('center_axis',(0.,1.,2.22044604925031E-16));
#111067=DIRECTION('ref_axis',(-1.,2.71926214689378E-32,-1.22464679914735E-16));
#111068=DIRECTION('center_axis',(0.866025403784439,1.26335723491828E-16,
-0.5));
#111069=DIRECTION('ref_axis',(0.5,-1.88822604713879E-16,0.866025403784439));
#111070=DIRECTION('',(-0.5,1.92296268638356E-16,-0.866025403784439));
#111071=DIRECTION('center_axis',(0.,1.,2.22044604925031E-16));
#111072=DIRECTION('ref_axis',(-1.,2.71926214689378E-32,-1.22464679914735E-16));
#111073=DIRECTION('center_axis',(0.,1.,2.22044604925031E-16));
#111074=DIRECTION('ref_axis',(1.,0.,0.));
#138715=CARTESIAN_POINT('',(0.,0.,0.));
#138716=CARTESIAN_POINT('Origin',(-13.5573012957478,-1.4,11.3142715795005));
#138717=CARTESIAN_POINT('',(-14.6656854249453,-1.4,10.771572875254));
#138718=CARTESIAN_POINT('',(-14.3828427124711,-1.,10.4887301627791));
#138719=CARTESIAN_POINT('Origin',(-14.3828427124711,-1.4,10.4887301627791));
#138720=CARTESIAN_POINT('',(-14.2088773290073,-1.,10.6626955462424));
#138721=CARTESIAN_POINT('',(-13.5573012957478,-1.,11.3142715795005));
#138722=CARTESIAN_POINT('',(-14.4917200414816,-1.4,10.9455382587174));
#138723=CARTESIAN_POINT('Origin',(-14.2088773290073,-1.4,10.6626955462424));
#138724=CARTESIAN_POINT('',(-13.8401440082221,-1.4,11.5971142919754));
#138725=CARTESIAN_POINT('Ctrl Pts',(-14.4917200414816,-1.4,10.9455382587174));
#138726=CARTESIAN_POINT('Ctrl Pts',(-14.1184687028433,-1.4,11.3187895973548));
#138727=CARTESIAN_POINT('Ctrl Pts',(-13.6284819468182,-1.4,11.1224579837265));
#138728=CARTESIAN_POINT('Ctrl Pts',(-13.1384951907931,-1.4,10.9261263700981));
#138729=CARTESIAN_POINT('Ctrl Pts',(-13.1262499063287,-1.4,10.398411317633));
#138730=CARTESIAN_POINT('Ctrl Pts',(-14.4917200414816,-1.,10.9455382587174));
#138731=CARTESIAN_POINT('Ctrl Pts',(-14.1184687028433,-1.,11.3187895973548));
#138732=CARTESIAN_POINT('Ctrl Pts',(-13.6284819468182,-1.,11.1224579837265));
#138733=CARTESIAN_POINT('Ctrl Pts',(-13.1384951907931,-1.,10.9261263700981));
#138734=CARTESIAN_POINT('Ctrl Pts',(-13.1262499063287,-1.,10.398411317633));
#138735=CARTESIAN_POINT('Ctrl Pts',(-14.2088773290073,-1.,10.6626955462424));
#138736=CARTESIAN_POINT('Ctrl Pts',(-14.0222516596882,-1.,10.8493212155611));
#138737=CARTESIAN_POINT('Ctrl Pts',(-13.7772582816756,-1.,10.751155408747));
#138738=CARTESIAN_POINT('Ctrl Pts',(-13.5322649036631,-1.,10.6529896019328));
#138739=CARTESIAN_POINT('Ctrl Pts',(-13.5261422614309,-1.,10.3891320757002));
#138740=CARTESIAN_POINT('',(-13.5261422614309,-1.,10.3891320757002));
#138741=CARTESIAN_POINT('',(-13.1262499063287,-1.4,10.398411317633));
#138742=CARTESIAN_POINT('Origin',(-13.5261422614309,-1.4,10.3891320757002));
#138743=CARTESIAN_POINT('Origin',(-13.926034616533,-1.4,10.3798528337675));
#138744=CARTESIAN_POINT('Origin',(-13.926034616533,-1.,10.3798528337675));
#138745=CARTESIAN_POINT('Origin',(-8.47750127826606,-1.4,10.5062825051013));
#138746=CARTESIAN_POINT('',(-9.51278842517889,-1.,5.56354232141399));
#138747=CARTESIAN_POINT('',(-9.43078548284916,-1.4,5.95504649437932));
#138748=CARTESIAN_POINT('Origin',(-9.51278842517889,-1.4,5.56354232141399));
#138749=CARTESIAN_POINT('Origin',(-8.47750127826606,-1.4,10.5062825051013));
#138750=CARTESIAN_POINT('Origin',(-8.47750127826606,-1.,10.5062825051013));
#138751=CARTESIAN_POINT('Ctrl Pts',(-9.43078548284916,-1.4,5.95504649437932));
#138752=CARTESIAN_POINT('Ctrl Pts',(-9.03827037400146,-1.4,5.87283180534908));
#138753=CARTESIAN_POINT('Ctrl Pts',(-8.86928360398281,-1.4,5.50914122625096));
#138754=CARTESIAN_POINT('Ctrl Pts',(-8.70029683396417,-1.4,5.14545064715283));
#138755=CARTESIAN_POINT('Ctrl Pts',(-8.89058649647474,-1.4,4.79243901829667));
#138756=CARTESIAN_POINT('Ctrl Pts',(-9.43078548284916,-1.,5.95504649437932));
#138757=CARTESIAN_POINT('Ctrl Pts',(-9.03827037400146,-1.,5.87283180534908));
#138758=CARTESIAN_POINT('Ctrl Pts',(-8.86928360398281,-1.,5.50914122625096));
#138759=CARTESIAN_POINT('Ctrl Pts',(-8.70029683396417,-1.,5.14545064715283));
#138760=CARTESIAN_POINT('Ctrl Pts',(-8.89058649647474,-1.,4.79243901829667));
#138761=CARTESIAN_POINT('Ctrl Pts',(-9.51278842517889,-1.,5.56354232141399));
#138762=CARTESIAN_POINT('Ctrl Pts',(-9.31653087075504,-1.,5.52243497689887));
#138763=CARTESIAN_POINT('Ctrl Pts',(-9.23203748574572,-1.,5.34058968734981));
#138764=CARTESIAN_POINT('Ctrl Pts',(-9.1475441007364,-1.,5.15874439780075));
#138765=CARTESIAN_POINT('Ctrl Pts',(-9.24268893199168,-1.,4.98223858337267));
#138766=CARTESIAN_POINT('',(-9.24268893199168,-1.,4.98223858337267));
#138767=CARTESIAN_POINT('',(-8.89058649647473,-1.4,4.79243901829667));
#138768=CARTESIAN_POINT('Origin',(-9.24268893199168,-1.4,4.98223858337267));
#138769=CARTESIAN_POINT('Origin',(-9.59479136750862,-1.4,5.17203814844866));
#138770=CARTESIAN_POINT('Origin',(-9.59479136750862,-1.,5.17203814844866));
#138771=CARTESIAN_POINT('Origin',(9.00768359641396E-11,-1.4,2.56054600265843E-10));
#138772=CARTESIAN_POINT('',(-10.4918084095504,-1.,-0.414676126038993));
#138773=CARTESIAN_POINT('',(-10.0921204701253,-1.4,-0.398878940274965));
#138774=CARTESIAN_POINT('Origin',(-10.4918084095504,-1.4,-0.414676126038993));
#138775=CARTESIAN_POINT('Origin',(9.00768359641396E-11,-1.4,2.56054600265843E-10));
#138776=CARTESIAN_POINT('Origin',(9.00768387396972E-11,-1.,2.56054689085632E-10));
#138777=CARTESIAN_POINT('Ctrl Pts',(-10.0921204701253,-1.4,-0.398878940274966));
#138778=CARTESIAN_POINT('Ctrl Pts',(-10.0765894685756,-1.4,-0.791832096572013));
#138779=CARTESIAN_POINT('Ctrl Pts',(-10.3782486193375,-1.4,-1.04413182272041));
#138780=CARTESIAN_POINT('Ctrl Pts',(-10.6799077700994,-1.4,-1.29643154886882));
#138781=CARTESIAN_POINT('Ctrl Pts',(-11.063924568312,-1.4,-1.21167015586761));
#138782=CARTESIAN_POINT('Ctrl Pts',(-10.0921204701253,-0.999999999999999,
-0.398878940274966));
#138783=CARTESIAN_POINT('Ctrl Pts',(-10.0765894685756,-0.999999999999999,
-0.791832096572014));
#138784=CARTESIAN_POINT('Ctrl Pts',(-10.3782486193375,-0.999999999999999,
-1.04413182272042));
#138785=CARTESIAN_POINT('Ctrl Pts',(-10.6799077700994,-0.999999999999999,
-1.29643154886882));
#138786=CARTESIAN_POINT('Ctrl Pts',(-11.063924568312,-0.999999999999999,
-1.21167015586761));
#138787=CARTESIAN_POINT('Ctrl Pts',(-10.4918084095504,-1.,-0.41467612603899));
#138788=CARTESIAN_POINT('Ctrl Pts',(-10.4840429087756,-1.,-0.611152704187514));
#138789=CARTESIAN_POINT('Ctrl Pts',(-10.6348724841566,-1.,-0.737302567261716));
#138790=CARTESIAN_POINT('Ctrl Pts',(-10.7857020595375,-1.,-0.863452430335917));
#138791=CARTESIAN_POINT('Ctrl Pts',(-10.9777104586438,-1.,-0.821071733835315));
#138792=CARTESIAN_POINT('',(-10.9777104586438,-1.,-0.821071733835314));
#138793=CARTESIAN_POINT('',(-11.063924568312,-1.4,-1.21167015586761));
#138794=CARTESIAN_POINT('Origin',(-10.9777104586438,-1.4,-0.821071733835314));
#138795=CARTESIAN_POINT('Origin',(-10.8914963489756,-1.4,-0.430473311803018));
#138796=CARTESIAN_POINT('Origin',(-10.8914963489756,-1.,-0.430473311803018));
#138797=CARTESIAN_POINT('Origin',(-8.47750127826606,-1.4,10.5062825051013));
#138798=CARTESIAN_POINT('',(-14.3008035257912,-1.,0.473877462741344));
#138799=CARTESIAN_POINT('',(-14.5016070515679,-1.4,0.127932461280656));
#138800=CARTESIAN_POINT('Origin',(-14.3008035257912,-1.4,0.473877462741344));
#138801=CARTESIAN_POINT('Origin',(-8.47750127826606,-1.4,10.5062825051013));
#138802=CARTESIAN_POINT('Origin',(-8.47750127826606,-1.,10.5062825051013));
#138803=CARTESIAN_POINT('Ctrl Pts',(-14.5016070515679,-1.4,0.127932461280656));
#138804=CARTESIAN_POINT('Ctrl Pts',(-14.9000000000149,-1.4,0.359179359934449));
#138805=CARTESIAN_POINT('Ctrl Pts',(-14.9000000000144,-1.4,0.819822464202032));
#138806=CARTESIAN_POINT('Ctrl Pts',(-14.5016070515679,-0.999999999999999,
0.127932461280656));
#138807=CARTESIAN_POINT('Ctrl Pts',(-14.9000000000149,-0.999999999999999,
0.359179359934449));
#138808=CARTESIAN_POINT('Ctrl Pts',(-14.9000000000144,-1.,0.819822464202032));
#138809=CARTESIAN_POINT('Ctrl Pts',(-14.3008035257912,-1.,0.473877462741344));
#138810=CARTESIAN_POINT('Ctrl Pts',(-14.5000000000146,-1.,0.589500912068241));
#138811=CARTESIAN_POINT('Ctrl Pts',(-14.5000000000144,-1.,0.819822464202032));
#138812=CARTESIAN_POINT('',(-14.5000000000144,-1.,0.819822464202785));
#138813=CARTESIAN_POINT('',(-14.9000000000144,-1.4,0.819822464203537));
#138814=CARTESIAN_POINT('Origin',(-14.5000000000144,-1.4,0.819822464202785));
#138815=CARTESIAN_POINT('Origin',(-14.1000000000144,-1.4,0.819822464202032));
#138816=CARTESIAN_POINT('Origin',(-14.1000000000144,-1.,0.819822464202032));
#138817=CARTESIAN_POINT('Origin',(-14.5000000000079,-1.4,4.28313090144278));
#138818=CARTESIAN_POINT('',(-14.4999999999968,-1.,10.2058874503049));
#138819=CARTESIAN_POINT('',(-14.8999999999968,-1.4,10.2058874503056));
#138820=CARTESIAN_POINT('Origin',(-14.4999999999968,-1.4,10.2058874503049));
#138821=CARTESIAN_POINT('',(-14.9000000000079,-1.4,4.28313090144353));
#138822=CARTESIAN_POINT('',(-14.5000000000079,-1.,4.28313090144278));
#138823=CARTESIAN_POINT('Ctrl Pts',(-14.8999999999968,-1.4,10.2058874503041));
#138824=CARTESIAN_POINT('Ctrl Pts',(-14.8999999999965,-1.4,10.537258300203));
#138825=CARTESIAN_POINT('Ctrl Pts',(-14.6656854249453,-1.4,10.771572875254));
#138826=CARTESIAN_POINT('Ctrl Pts',(-14.8999999999968,-1.,10.2058874503041));
#138827=CARTESIAN_POINT('Ctrl Pts',(-14.8999999999965,-1.,10.537258300203));
#138828=CARTESIAN_POINT('Ctrl Pts',(-14.6656854249453,-1.,10.771572875254));
#138829=CARTESIAN_POINT('Ctrl Pts',(-14.4999999999968,-1.,10.2058874503041));
#138830=CARTESIAN_POINT('Ctrl Pts',(-14.4999999999966,-1.,10.3715728752536));
#138831=CARTESIAN_POINT('Ctrl Pts',(-14.3828427124711,-1.,10.4887301627791));
#138832=CARTESIAN_POINT('Origin',(-14.0999999999968,-1.4,10.2058874503041));
#138833=CARTESIAN_POINT('Origin',(-14.0999999999968,-1.,10.2058874503041));
#138834=CARTESIAN_POINT('Origin',(-8.47750127826606,-2.6,10.5062825051013));
#138835=CARTESIAN_POINT('',(-14.5016070515679,-2.6,0.127932461280655));
#138836=CARTESIAN_POINT('',(-14.5016070515679,-2.6,0.127932461280655));
#138837=CARTESIAN_POINT('',(-15.8541129444743,-2.6,1.0413155043157));
#138838=CARTESIAN_POINT('Origin',(-8.47750127826606,-2.6,10.5062825051013));
#138839=CARTESIAN_POINT('',(-15.8541129444743,-10.1,1.0413155043157));
#138840=CARTESIAN_POINT('',(-15.8541129444743,-2.6,1.0413155043157));
#138841=CARTESIAN_POINT('',(-12.1362808769477,-10.1,-0.922336477447361));
#138842=CARTESIAN_POINT('Origin',(-8.47750127826606,-10.1,10.5062825051013));
#138843=CARTESIAN_POINT('',(-12.136280876716,-7.19501169002543,-0.922336477521518));
#138844=CARTESIAN_POINT('',(-12.1362808769477,-2.6,-0.922336477447359));
#138845=CARTESIAN_POINT('',(-8.68954964093271,-5.49648661887902,-1.49184382745125));
#138846=CARTESIAN_POINT('Ctrl Pts',(-8.68954964093266,-5.4964866188789,
-1.49184382745125));
#138847=CARTESIAN_POINT('Ctrl Pts',(-8.87481436092436,-5.43513385013829,
-1.4885695594993));
#138848=CARTESIAN_POINT('Ctrl Pts',(-9.26624052344372,-5.36455736140126,
-1.47266896725833));
#138849=CARTESIAN_POINT('Ctrl Pts',(-9.8483467388184,-5.48100398345319,
-1.41973709154106));
#138850=CARTESIAN_POINT('Ctrl Pts',(-10.8839646004455,-6.01582765661507,
-1.27510485735236));
#138851=CARTESIAN_POINT('Ctrl Pts',(-11.5886799961236,-6.67315581787308,
-1.09764645444795));
#138852=CARTESIAN_POINT('Ctrl Pts',(-12.1362808769477,-7.19501169024617,
-0.922336477447363));
#138853=CARTESIAN_POINT('',(-8.68954964093293,-2.6,-1.49184382745124));
#138854=CARTESIAN_POINT('',(-8.68954964093293,-2.6,-1.49184382745124));
#138855=CARTESIAN_POINT('',(-11.063924568312,-2.6,-1.21167015586761));
#138856=CARTESIAN_POINT('Origin',(-8.47750127826606,-2.6,10.5062825051013));
#138857=CARTESIAN_POINT('',(-11.063924568312,-2.6,-1.21167015586761));
#138858=CARTESIAN_POINT('Origin',(-14.1000000000144,-2.6,0.819822464202031));
#138859=CARTESIAN_POINT('',(-14.9000000000144,-2.6,0.819822464203537));
#138860=CARTESIAN_POINT('',(-14.9000000000144,-2.6,0.819822464203537));
#138861=CARTESIAN_POINT('Origin',(-14.1000000000144,-2.6,0.819822464202031));
#138862=CARTESIAN_POINT('Origin',(-14.9000000000153,-1.6,0.369640547868617));
#138863=CARTESIAN_POINT('',(-14.8999999999968,-2.6,10.2058874503056));
#138864=CARTESIAN_POINT('',(-14.8999999999968,-1.6,10.2058874503056));
#138865=CARTESIAN_POINT('',(-14.9000000000324,-2.6,-8.71274169982173));
#138866=CARTESIAN_POINT('Origin',(-14.0999999999968,-1.6,10.2058874503041));
#138867=CARTESIAN_POINT('',(-14.6656854249453,-2.6,10.771572875254));
#138868=CARTESIAN_POINT('',(-14.6656854249453,-1.6,10.771572875254));
#138869=CARTESIAN_POINT('Origin',(-14.0999999999968,-2.6,10.2058874503041));
#138870=CARTESIAN_POINT('Origin',(-14.8999999999961,-1.6,10.5372583002038));
#138871=CARTESIAN_POINT('',(-14.4917200414816,-2.6,10.9455382587174));
#138872=CARTESIAN_POINT('',(-14.4917200414816,-2.6,10.9455382587174));
#138873=CARTESIAN_POINT('',(-14.8999999999961,-2.6,10.5372583002038));
#138874=CARTESIAN_POINT('Origin',(-8.31993898771739,-1.,8.19662125500606));
#138875=CARTESIAN_POINT('Origin',(-11.9915184469055,-1.4,-6.13955455136528));
#138876=CARTESIAN_POINT('',(-11.5237848152765,-1.4,-6.09584299941717));
#138877=CARTESIAN_POINT('',(-11.8824156877396,-0.999999999999998,-5.91868799012766));
#138878=CARTESIAN_POINT('Origin',(-11.8824156877396,-1.4,-5.91868799012766));
#138879=CARTESIAN_POINT('',(-14.7997235069111,-0.999999999999996,-11.8244574777011));
#138880=CARTESIAN_POINT('',(-11.9915184469055,-0.999999999999998,-6.13955455136528));
#138881=CARTESIAN_POINT('',(-14.441092634448,-1.4,-12.0016124869907));
#138882=CARTESIAN_POINT('Origin',(-14.7997235069111,-1.4,-11.8244574777011));
#138883=CARTESIAN_POINT('',(-11.6328875744424,-1.4,-6.3167095606548));
#138884=CARTESIAN_POINT('Ctrl Pts',(-14.441092634448,-1.4,-12.0016124869907));
#138885=CARTESIAN_POINT('Ctrl Pts',(-14.6327150753576,-1.4,-12.3895310868797));
#138886=CARTESIAN_POINT('Ctrl Pts',(-15.0612959521201,-1.4,-12.3302147141527));
#138887=CARTESIAN_POINT('Ctrl Pts',(-14.441092634448,-0.999999999999997,
-12.0016124869907));
#138888=CARTESIAN_POINT('Ctrl Pts',(-14.6327150753576,-0.999999999999997,
-12.3895310868797));
#138889=CARTESIAN_POINT('Ctrl Pts',(-15.0612959521201,-0.999999999999997,
-12.3302147141527));
#138890=CARTESIAN_POINT('Ctrl Pts',(-14.7997235069111,-0.999999999999997,
-11.8244574777011));
#138891=CARTESIAN_POINT('Ctrl Pts',(-14.8635976538809,-0.999999999999997,
-11.9537636776641));
#138892=CARTESIAN_POINT('Ctrl Pts',(-15.0064579461351,-0.999999999999997,
-11.9339915534218));
#138893=CARTESIAN_POINT('',(-15.0064579461351,-0.999999999999996,-11.9339915534218));
#138894=CARTESIAN_POINT('',(-15.0612959521201,-1.4,-12.3302147141527));
#138895=CARTESIAN_POINT('Origin',(-15.0064579461351,-1.4,-11.9339915534218));
#138896=CARTESIAN_POINT('Origin',(-14.9790389431426,-1.4,-11.7358799730564));
#138897=CARTESIAN_POINT('Origin',(-14.9790389431426,-0.999999999999996,
-11.7358799730564));
#138898=CARTESIAN_POINT('Origin',(-15.5,-1.4,-15.5));
#138899=CARTESIAN_POINT('',(-16.5800000000255,-0.999999999999996,-12.065818874907));
#138900=CARTESIAN_POINT('',(-16.4600000000227,-1.4,-12.4473945554729));
#138901=CARTESIAN_POINT('Origin',(-16.5800000000255,-1.4,-12.065818874907));
#138902=CARTESIAN_POINT('Origin',(-15.5,-1.4,-15.5));
#138903=CARTESIAN_POINT('Origin',(-15.5,-0.999999999999996,-15.5));
#138904=CARTESIAN_POINT('Ctrl Pts',(-16.4600000000227,-1.4,-12.4473945554729));
#138905=CARTESIAN_POINT('Ctrl Pts',(-16.8465727653177,-1.4,-12.5689660659206));
#138906=CARTESIAN_POINT('Ctrl Pts',(-17.1732863826715,-1.4,-12.3292238142085));
#138907=CARTESIAN_POINT('Ctrl Pts',(-17.5000000000253,-1.4,-12.0894815624965));
#138908=CARTESIAN_POINT('Ctrl Pts',(-17.5000000000283,-1.4,-11.6842431943471));
#138909=CARTESIAN_POINT('Ctrl Pts',(-16.4600000000227,-0.999999999999995,
-12.4473945554729));
#138910=CARTESIAN_POINT('Ctrl Pts',(-16.8465727653177,-0.999999999999996,
-12.5689660659206));
#138911=CARTESIAN_POINT('Ctrl Pts',(-17.1732863826715,-0.999999999999996,
-12.3292238142085));
#138912=CARTESIAN_POINT('Ctrl Pts',(-17.5000000000253,-0.999999999999996,
-12.0894815624965));
#138913=CARTESIAN_POINT('Ctrl Pts',(-17.5000000000283,-0.999999999999996,
-11.6842431943471));
#138914=CARTESIAN_POINT('Ctrl Pts',(-16.5800000000255,-0.999999999999997,
-12.065818874907));
#138915=CARTESIAN_POINT('Ctrl Pts',(-16.773286382673,-0.999999999999997,
-12.1266046301309));
#138916=CARTESIAN_POINT('Ctrl Pts',(-16.9366431913499,-0.999999999999997,
-12.0067335042748));
#138917=CARTESIAN_POINT('Ctrl Pts',(-17.1000000000268,-0.999999999999997,
-11.8868623784188));
#138918=CARTESIAN_POINT('Ctrl Pts',(-17.1000000000283,-0.999999999999997,
-11.6842431943441));
#138919=CARTESIAN_POINT('',(-17.1000000000283,-0.999999999999996,-11.6842431943441));
#138920=CARTESIAN_POINT('',(-17.5000000000283,-1.4,-11.6842431943471));
#138921=CARTESIAN_POINT('Origin',(-17.1000000000283,-1.4,-11.6842431943441));
#138922=CARTESIAN_POINT('Origin',(-16.7000000000283,-1.4,-11.6842431943411));
#138923=CARTESIAN_POINT('Origin',(-16.7000000000283,-0.999999999999996,
-11.6842431943411));
#138924=CARTESIAN_POINT('Origin',(-17.1000000000372,-1.4,-10.4863375378306));
#138925=CARTESIAN_POINT('',(-17.1000000000286,-0.999999999999996,-11.6441125497194));
#138926=CARTESIAN_POINT('',(-17.5000000000286,-1.4,-11.6441125497224));
#138927=CARTESIAN_POINT('Origin',(-17.1000000000286,-1.4,-11.6441125497194));
#138928=CARTESIAN_POINT('',(-17.5000000000372,-1.4,-10.4863375378336));
#138929=CARTESIAN_POINT('',(-17.1000000000372,-0.999999999999997,-10.4863375378306));
#138930=CARTESIAN_POINT('Ctrl Pts',(-17.5000000000286,-1.4,-11.6441125497165));
#138931=CARTESIAN_POINT('Ctrl Pts',(-17.5000000000299,-1.4,-11.3127416998175));
#138932=CARTESIAN_POINT('Ctrl Pts',(-17.2656854249779,-1.4,-11.0784271247672));
#138933=CARTESIAN_POINT('Ctrl Pts',(-17.5000000000286,-0.999999999999995,
-11.6441125497165));
#138934=CARTESIAN_POINT('Ctrl Pts',(-17.5000000000299,-0.999999999999995,
-11.3127416998175));
#138935=CARTESIAN_POINT('Ctrl Pts',(-17.2656854249779,-0.999999999999995,
-11.0784271247672));
#138936=CARTESIAN_POINT('Ctrl Pts',(-17.1000000000286,-0.999999999999996,
-11.6441125497165));
#138937=CARTESIAN_POINT('Ctrl Pts',(-17.1000000000293,-0.999999999999996,
-11.478427124767));
#138938=CARTESIAN_POINT('Ctrl Pts',(-16.9828427125033,-0.999999999999996,
-11.3612698372419));
#138939=CARTESIAN_POINT('',(-16.9828427125033,-0.999999999999996,-11.3612698372419));
#138940=CARTESIAN_POINT('',(-17.2656854249779,-1.4,-11.0784271247672));
#138941=CARTESIAN_POINT('Origin',(-16.9828427125033,-1.4,-11.3612698372419));
#138942=CARTESIAN_POINT('Origin',(-16.7000000000286,-1.4,-11.6441125497165));
#138943=CARTESIAN_POINT('Origin',(-16.7000000000286,-0.999999999999996,
-11.6441125497165));
#138944=CARTESIAN_POINT('Origin',(-15.2217176089063,-1.4,-9.6001447336449));
#138945=CARTESIAN_POINT('',(-14.8514718626079,-0.999999999999997,-9.22989898734649));
#138946=CARTESIAN_POINT('',(-15.1343145750825,-1.4,-8.94705627487187));
#138947=CARTESIAN_POINT('Origin',(-14.8514718626079,-1.4,-9.22989898734649));
#138948=CARTESIAN_POINT('',(-15.5045603213809,-1.4,-9.31730202117028));
#138949=CARTESIAN_POINT('',(-15.2217176089063,-0.999999999999997,-9.6001447336449));
#138950=CARTESIAN_POINT('Origin',(-15.7000000000318,-1.4,-8.38137084992263));
#138951=CARTESIAN_POINT('',(-14.5000000000318,-0.999999999999997,-8.38137084992489));
#138952=CARTESIAN_POINT('',(-14.9000000000318,-1.4,-8.38137084992414));
#138953=CARTESIAN_POINT('Origin',(-14.5000000000318,-1.4,-8.38137084992489));
#138954=CARTESIAN_POINT('Origin',(-15.7000000000318,-1.4,-8.38137084992263));
#138955=CARTESIAN_POINT('Origin',(-15.7000000000318,-0.999999999999997,
-8.38137084992263));
#138956=CARTESIAN_POINT('Origin',(-14.5000000000293,-1.4,-7.09270838774364));
#138957=CARTESIAN_POINT('',(-14.5000000000203,-0.999999999999999,-2.31508669338342));
#138958=CARTESIAN_POINT('',(-14.9000000000203,-1.4,-2.31508669338267));
#138959=CARTESIAN_POINT('Origin',(-14.5000000000203,-1.4,-2.31508669338342));
#138960=CARTESIAN_POINT('',(-14.9000000000293,-1.4,-7.09270838774289));
#138961=CARTESIAN_POINT('',(-14.5000000000293,-0.999999999999998,-7.09270838774364));
#138962=CARTESIAN_POINT('Ctrl Pts',(-14.9000000000203,-1.4,-2.31508669338417));
#138963=CARTESIAN_POINT('Ctrl Pts',(-14.9000000000199,-1.4,-1.88217329548528));
#138964=CARTESIAN_POINT('Ctrl Pts',(-14.5375908403063,-1.4,-1.64537462353789));
#138965=CARTESIAN_POINT('Ctrl Pts',(-14.1751816805932,-1.4,-1.40857595159125));
#138966=CARTESIAN_POINT('Ctrl Pts',(-13.7787143587772,-1.4,-1.58243702489929));
#138967=CARTESIAN_POINT('Ctrl Pts',(-14.9000000000203,-0.999999999999991,
-2.31508669338417));
#138968=CARTESIAN_POINT('Ctrl Pts',(-14.9000000000199,-0.999999999999992,
-1.88217329548528));
#138969=CARTESIAN_POINT('Ctrl Pts',(-14.5375908403063,-0.999999999999992,
-1.64537462353789));
#138970=CARTESIAN_POINT('Ctrl Pts',(-14.1751816805932,-0.999999999999992,
-1.40857595159125));
#138971=CARTESIAN_POINT('Ctrl Pts',(-13.7787143587772,-0.999999999999992,
-1.58243702489929));
#138972=CARTESIAN_POINT('Ctrl Pts',(-14.5000000000203,-0.999999999999998,
-2.31508669338417));
#138973=CARTESIAN_POINT('Ctrl Pts',(-14.5000000000201,-0.999999999999998,
-2.09862999443473));
#138974=CARTESIAN_POINT('Ctrl Pts',(-14.3187954201633,-0.999999999999998,
-1.98023065846104));
#138975=CARTESIAN_POINT('Ctrl Pts',(-14.1375908403068,-0.999999999999998,
-1.86183132248772));
#138976=CARTESIAN_POINT('Ctrl Pts',(-13.9393571793988,-0.999999999999998,
-1.94876185914174));
#138977=CARTESIAN_POINT('',(-13.9393571793988,-0.999999999999999,-1.94876185914173));
#138978=CARTESIAN_POINT('',(-13.7787143587772,-1.4,-1.58243702489929));
#138979=CARTESIAN_POINT('Origin',(-13.9393571793988,-1.4,-1.94876185914173));
#138980=CARTESIAN_POINT('Origin',(-14.1000000000203,-1.4,-2.31508669338417));
#138981=CARTESIAN_POINT('Origin',(-14.1000000000203,-0.999999999999999,
-2.31508669338417));
#138982=CARTESIAN_POINT('Origin',(-8.47750127826606,-1.4,10.5062825051013));
#138983=CARTESIAN_POINT('',(-12.9945355807443,-0.999999999999999,-2.32167138904082));
#138984=CARTESIAN_POINT('',(-12.8616816306714,-1.4,-1.9443786274484));
#138985=CARTESIAN_POINT('Origin',(-12.9945355807443,-1.4,-2.32167138904082));
#138986=CARTESIAN_POINT('Origin',(-8.47750127826606,-1.4,10.5062825051013));
#138987=CARTESIAN_POINT('Origin',(-8.47750127826606,-1.,10.5062825051013));
#138988=CARTESIAN_POINT('Ctrl Pts',(-12.8616816306714,-1.4,-1.9443786274484));
#138989=CARTESIAN_POINT('Ctrl Pts',(-12.3961845071422,-1.4,-2.10829147684258));
#138990=CARTESIAN_POINT('Ctrl Pts',(-12.4672085468558,-1.4,-2.59666692666902));
#138991=CARTESIAN_POINT('Ctrl Pts',(-12.8616816306714,-0.999999999999995,
-1.9443786274484));
#138992=CARTESIAN_POINT('Ctrl Pts',(-12.3961845071422,-0.999999999999995,
-2.10829147684258));
#138993=CARTESIAN_POINT('Ctrl Pts',(-12.4672085468558,-0.999999999999994,
-2.59666692666902));
#138994=CARTESIAN_POINT('Ctrl Pts',(-12.9945355807443,-0.999999999999998,
-2.32167138904082));
#138995=CARTESIAN_POINT('Ctrl Pts',(-12.8393698729012,-0.999999999999998,
-2.37630900550554));
#138996=CARTESIAN_POINT('Ctrl Pts',(-12.8630445528057,-0.999999999999998,
-2.53910082211435));
#138997=CARTESIAN_POINT('',(-12.8630445528057,-0.999999999999998,-2.53910082211435));
#138998=CARTESIAN_POINT('',(-12.4672085468558,-1.4,-2.59666692666902));
#138999=CARTESIAN_POINT('Origin',(-12.8630445528057,-1.4,-2.53910082211435));
#139000=CARTESIAN_POINT('Origin',(-13.0609625557807,-1.4,-2.51031776983702));
#139001=CARTESIAN_POINT('Origin',(-13.0609625557807,-0.999999999999998,
-2.51031776983702));
#139002=CARTESIAN_POINT('Origin',(-9.35,-1.4,-3.05000000003699));
#139003=CARTESIAN_POINT('',(-11.9482823515746,-0.999999999999998,-5.46897267898486));
#139004=CARTESIAN_POINT('',(-11.6555181429464,-1.4,-5.19641237713157));
#139005=CARTESIAN_POINT('Origin',(-11.9482823515746,-1.4,-5.46897267898486));
#139006=CARTESIAN_POINT('',(-12.5,-1.4,-3.05000000003699));
#139007=CARTESIAN_POINT('Origin',(-9.35,-1.4,-3.05000000003699));
#139008=CARTESIAN_POINT('Origin',(-9.35,-1.4,-3.05000000003699));
#139009=CARTESIAN_POINT('Origin',(-9.35,-0.999999999999998,-3.05000000003699));
#139010=CARTESIAN_POINT('Ctrl Pts',(-11.6555181429464,-1.4,-5.19641237713157));
#139011=CARTESIAN_POINT('Ctrl Pts',(-11.2791734498063,-1.4,-5.60065413761314));
#139012=CARTESIAN_POINT('Ctrl Pts',(-11.5237848152765,-1.4,-6.09584299941717));
#139013=CARTESIAN_POINT('Ctrl Pts',(-11.6555181429464,-0.999999999999997,
-5.19641237713157));
#139014=CARTESIAN_POINT('Ctrl Pts',(-11.2791734498063,-0.999999999999996,
-5.60065413761314));
#139015=CARTESIAN_POINT('Ctrl Pts',(-11.5237848152765,-0.999999999999996,
-6.09584299941717));
#139016=CARTESIAN_POINT('Ctrl Pts',(-11.9482823515746,-0.999999999999998,
-5.46897267898485));
#139017=CARTESIAN_POINT('Ctrl Pts',(-11.7601100050045,-0.999999999999998,
-5.67109355922564));
#139018=CARTESIAN_POINT('Ctrl Pts',(-11.8824156877396,-0.999999999999998,
-5.91868799012765));
#139019=CARTESIAN_POINT('Origin',(-12.2410465602027,-1.4,-5.74153298083814));
#139020=CARTESIAN_POINT('Origin',(-12.2410465602027,-0.999999999999998,
-5.74153298083814));
#139021=CARTESIAN_POINT('Origin',(-14.9000000000324,-1.6,-8.71274169982173));
#139022=CARTESIAN_POINT('',(-14.9000000000203,-10.1,-2.31508669338267));
#139023=CARTESIAN_POINT('',(-14.9000000000203,-10.3,-2.31508669338267));
#139024=CARTESIAN_POINT('',(-14.9000000000318,-10.1,-8.38137084992414));
#139025=CARTESIAN_POINT('',(-14.9000000000291,-10.1,-6.97072868003485));
#139026=CARTESIAN_POINT('',(-14.9000000000318,-1.6,-8.38137084992414));
#139027=CARTESIAN_POINT('Origin',(-14.1000000000203,-10.3,-2.31508669338417));
#139028=CARTESIAN_POINT('',(-13.7787143587772,-10.1,-1.58243702489929));
#139029=CARTESIAN_POINT('',(-13.7787143587772,-10.3,-1.58243702489929));
#139030=CARTESIAN_POINT('Origin',(-14.1000000000203,-10.1,-2.31508669338417));
#139031=CARTESIAN_POINT('Origin',(-8.47750127826606,-10.3,10.5062825051013));
#139032=CARTESIAN_POINT('',(-12.8616816306714,-10.1,-1.9443786274484));
#139033=CARTESIAN_POINT('',(-12.8616816306714,-10.3,-1.9443786274484));
#139034=CARTESIAN_POINT('Origin',(-8.47750127826606,-10.1,10.5062825051013));
#139035=CARTESIAN_POINT('Origin',(-13.0609625557807,-10.3,-2.51031776983702));
#139036=CARTESIAN_POINT('',(-12.4672085468558,-10.1,-2.59666692666902));
#139037=CARTESIAN_POINT('',(-12.4672085468558,-10.3,-2.59666692666902));
#139038=CARTESIAN_POINT('Origin',(-13.0609625557807,-10.1,-2.51031776983702));
#139039=CARTESIAN_POINT('Origin',(-9.35,-10.3,-3.05000000003699));
#139040=CARTESIAN_POINT('',(-12.5,-10.4,-3.05000000003699));
#139041=CARTESIAN_POINT('Origin',(-9.35,-10.4,-3.05000000003699));
#139042=CARTESIAN_POINT('',(-12.5,-10.3,-3.05000000003699));
#139043=CARTESIAN_POINT('',(-11.6555181429464,-10.1,-5.19641237713158));
#139044=CARTESIAN_POINT('',(-11.6555181429464,-10.3,-5.19641237713158));
#139045=CARTESIAN_POINT('',(-9.76798833941153,-10.1,-6.17214441503704));
#139046=CARTESIAN_POINT('Origin',(-9.35,-10.1,-3.05000000003699));
#139047=CARTESIAN_POINT('',(-9.76798833941153,-1.4,-6.17214441503704));
#139048=CARTESIAN_POINT('',(-9.76798833941153,-10.3,-6.17214441503704));
#139049=CARTESIAN_POINT('',(-8.1843866565298,-1.4,-5.97640488205934));
#139050=CARTESIAN_POINT('Origin',(-9.35,-1.4,-3.05000000003699));
#139051=CARTESIAN_POINT('',(-8.1843866565298,-10.1,-5.97640488205934));
#139052=CARTESIAN_POINT('',(-8.1843866565298,-10.3,-5.97640488205934));
#139053=CARTESIAN_POINT('',(-6.64846378001877,-10.1,-4.66993890386316));
#139054=CARTESIAN_POINT('Origin',(-9.35,-10.1,-3.05000000003699));
#139055=CARTESIAN_POINT('',(-6.64846378001877,-7.05,-4.66993890386316));
#139056=CARTESIAN_POINT('',(-6.64846378001877,-10.3,-4.66993890386316));
#139057=CARTESIAN_POINT('',(-11.5368071934914,-7.05,-0.782760643794657));
#139058=CARTESIAN_POINT('Origin',(-9.35,-7.05,-3.05000000003699));
#139059=CARTESIAN_POINT('',(-11.5368071934914,-10.1,-0.782760643794658));
#139060=CARTESIAN_POINT('',(-11.5368071934914,-2.6,-0.782760643794656));
#139061=CARTESIAN_POINT('Origin',(-9.35,-10.1,-3.05000000003699));
#139062=CARTESIAN_POINT('Origin',(-12.2410465602027,-10.3,-5.74153298083814));
#139063=CARTESIAN_POINT('',(-11.5237848152765,-10.1,-6.09584299941718));
#139064=CARTESIAN_POINT('',(-11.5237848152765,-10.3,-6.09584299941718));
#139065=CARTESIAN_POINT('Origin',(-12.2410465602027,-10.1,-5.74153298083814));
#139066=CARTESIAN_POINT('Origin',(-11.2373003829631,-10.3,-5.51588670961375));
#139067=CARTESIAN_POINT('',(-14.441092634448,-10.1,-12.0016124869907));
#139068=CARTESIAN_POINT('',(-14.441092634448,-10.3,-12.0016124869907));
#139069=CARTESIAN_POINT('',(-12.0443465189275,-10.1,-7.14966303363441));
#139070=CARTESIAN_POINT('Origin',(-15.3583079095877,-0.999999999999998,
-5.47267507566318));
#139071=CARTESIAN_POINT('Origin',(-5.6920614055489E-17,-1.4,9.32936375408611E-17));
#139072=CARTESIAN_POINT('',(-7.49853797666954,-1.4,-6.15320473424437));
#139073=CARTESIAN_POINT('',(-7.8077560370881,-0.999999999999998,-6.40694513526671));
#139074=CARTESIAN_POINT('Origin',(-7.8077560370881,-1.4,-6.40694513526671));
#139075=CARTESIAN_POINT('',(-1.36872658490553,-0.999999999999997,-10.0068270614005));
#139076=CARTESIAN_POINT('Origin',(-5.6920614055489E-17,-0.999999999999999,
1.82111479510874E-16));
#139077=CARTESIAN_POINT('',(-1.3145195915239,-1.4,-9.61051707935543));
#139078=CARTESIAN_POINT('Origin',(-1.36872658490553,-1.4,-10.0068270614005));
#139079=CARTESIAN_POINT('Origin',(-5.6920614055489E-17,-1.4,9.32936375408611E-17));
#139080=CARTESIAN_POINT('Ctrl Pts',(-1.3145195915239,-1.4,-9.61051707935543));
#139081=CARTESIAN_POINT('Ctrl Pts',(-0.796043967664363,-1.4,-9.68143380107428));
#139082=CARTESIAN_POINT('Ctrl Pts',(-0.795830131689239,-1.4,-10.2047368760032));
#139083=CARTESIAN_POINT('Ctrl Pts',(-1.3145195915239,-0.999999999999992,
-9.61051707935543));
#139084=CARTESIAN_POINT('Ctrl Pts',(-0.796043967664363,-0.999999999999992,
-9.68143380107428));
#139085=CARTESIAN_POINT('Ctrl Pts',(-0.795830131689239,-0.999999999999992,
-10.2047368760032));
#139086=CARTESIAN_POINT('Ctrl Pts',(-1.36872658490553,-0.999999999999997,
-10.0068270614005));
#139087=CARTESIAN_POINT('Ctrl Pts',(-1.19590137695235,-0.999999999999997,
-10.0304659686401));
#139088=CARTESIAN_POINT('Ctrl Pts',(-1.19583009829398,-0.999999999999997,
-10.2049003269497));
#139089=CARTESIAN_POINT('',(-1.19583009829397,-0.999999999999997,-10.2049003269497));
#139090=CARTESIAN_POINT('',(-0.795830131689239,-1.4,-10.2047368760032));
#139091=CARTESIAN_POINT('Origin',(-1.19583009829397,-1.4,-10.2049003269497));
#139092=CARTESIAN_POINT('Origin',(-1.39583008159634,-1.4,-10.204982052423));
#139093=CARTESIAN_POINT('Origin',(-1.39583008159634,-0.999999999999997,
-10.204982052423));
#139094=CARTESIAN_POINT('Origin',(-1.19695920643336,-1.4,-7.44172747482704));
#139095=CARTESIAN_POINT('',(-1.19309433051448,-0.999999999999995,-16.8999182745535));
#139096=CARTESIAN_POINT('',(-0.79309436390975,-1.39999999999999,-16.899754823607));
#139097=CARTESIAN_POINT('Origin',(-1.19309433051448,-1.39999999999999,-16.8999182745535));
#139098=CARTESIAN_POINT('',(-0.796959239828628,-1.4,-7.44156402388053));
#139099=CARTESIAN_POINT('',(-1.19695920643336,-0.999999999999997,-7.44172747482704));
#139100=CARTESIAN_POINT('Ctrl Pts',(-0.793094363909749,-1.39999999999999,
-16.899754823607));
#139101=CARTESIAN_POINT('Ctrl Pts',(-0.792992779166526,-1.39999999999999,
-17.1483547538275));
#139102=CARTESIAN_POINT('Ctrl Pts',(-0.968743571003919,-1.39999999999999,
-17.3241773769272));
#139103=CARTESIAN_POINT('Ctrl Pts',(-1.14449436284124,-1.39999999999999,
-17.5000000000268));
#139104=CARTESIAN_POINT('Ctrl Pts',(-1.39309431381685,-1.39999999999999,
-17.5000000000267));
#139105=CARTESIAN_POINT('Ctrl Pts',(-0.793094363909749,-0.999999999999954,
-16.899754823607));
#139106=CARTESIAN_POINT('Ctrl Pts',(-0.792992779166526,-0.999999999999954,
-17.1483547538275));
#139107=CARTESIAN_POINT('Ctrl Pts',(-0.968743571003919,-0.999999999999954,
-17.3241773769272));
#139108=CARTESIAN_POINT('Ctrl Pts',(-1.14449436284124,-0.999999999999954,
-17.5000000000268));
#139109=CARTESIAN_POINT('Ctrl Pts',(-1.39309431381685,-0.999999999999954,
-17.5000000000267));
#139110=CARTESIAN_POINT('Ctrl Pts',(-1.19309433051452,-0.999999999999994,
-16.8999182745535));
#139111=CARTESIAN_POINT('Ctrl Pts',(-1.19306046893345,-0.999999999999994,
-16.9827849179603));
#139112=CARTESIAN_POINT('Ctrl Pts',(-1.25164406621257,-0.999999999999994,
-17.0413924589935));
#139113=CARTESIAN_POINT('Ctrl Pts',(-1.31022766349166,-0.999999999999994,
-17.1000000000267));
#139114=CARTESIAN_POINT('Ctrl Pts',(-1.39309431381685,-0.999999999999994,
-17.1000000000267));
#139115=CARTESIAN_POINT('',(-1.39309431381659,-0.999999999999995,-17.1000000000267));
#139116=CARTESIAN_POINT('',(-1.39309431381607,-1.39999999999999,-17.5000000000267));
#139117=CARTESIAN_POINT('Origin',(-1.39309431381659,-1.39999999999999,-17.1000000000267));
#139118=CARTESIAN_POINT('Origin',(-1.39309431381685,-1.39999999999999,-16.9000000000267));
#139119=CARTESIAN_POINT('Origin',(-1.39309431381685,-0.999999999999995,
-16.9000000000267));
#139120=CARTESIAN_POINT('Origin',(-8.07557849842838,-1.4,-17.1000000000355));
#139121=CARTESIAN_POINT('',(-11.9672956534847,-0.999999999999995,-17.1000000000405));
#139122=CARTESIAN_POINT('',(-11.9672956534841,-1.39999999999999,-17.5000000000405));
#139123=CARTESIAN_POINT('Origin',(-11.9672956534847,-1.4,-17.1000000000405));
#139124=CARTESIAN_POINT('',(-8.07557849842786,-1.4,-17.5000000000355));
#139125=CARTESIAN_POINT('',(-8.07557849842838,-0.999999999999995,-17.1000000000355));
#139126=CARTESIAN_POINT('Ctrl Pts',(-11.9672956534849,-1.4,-17.5000000000405));
#139127=CARTESIAN_POINT('Ctrl Pts',(-12.2850405509874,-1.4,-17.5000000000406));
#139128=CARTESIAN_POINT('Ctrl Pts',(-12.4635977686079,-1.4,-17.2371708922072));
#139129=CARTESIAN_POINT('Ctrl Pts',(-12.6421549862285,-1.4,-16.9743417843737));
#139130=CARTESIAN_POINT('Ctrl Pts',(-12.5250910766189,-1.4,-16.6789473684552));
#139131=CARTESIAN_POINT('Ctrl Pts',(-11.9672956534849,-0.999999999999995,
-17.5000000000405));
#139132=CARTESIAN_POINT('Ctrl Pts',(-12.2850405509874,-0.999999999999995,
-17.5000000000406));
#139133=CARTESIAN_POINT('Ctrl Pts',(-12.4635977686079,-0.999999999999995,
-17.2371708922072));
#139134=CARTESIAN_POINT('Ctrl Pts',(-12.6421549862285,-0.999999999999995,
-16.9743417843737));
#139135=CARTESIAN_POINT('Ctrl Pts',(-12.5250910766189,-0.999999999999995,
-16.6789473684552));
#139136=CARTESIAN_POINT('Ctrl Pts',(-11.9672956534849,-0.999999999999996,
-17.1000000000405));
#139137=CARTESIAN_POINT('Ctrl Pts',(-12.0732106193191,-0.999999999999996,
-17.1000000000406));
#139138=CARTESIAN_POINT('Ctrl Pts',(-12.1327296918593,-0.999999999999996,
-17.0123902974294));
#139139=CARTESIAN_POINT('Ctrl Pts',(-12.1922487643995,-0.999999999999996,
-16.9247805948183));
#139140=CARTESIAN_POINT('Ctrl Pts',(-12.1532274611963,-0.999999999999996,
-16.8263157895121));
#139141=CARTESIAN_POINT('',(-12.1532274611963,-0.999999999999995,-16.8263157895121));
#139142=CARTESIAN_POINT('',(-12.5250910766189,-1.4,-16.6789473684552));
#139143=CARTESIAN_POINT('Origin',(-12.1532274611963,-1.4,-16.8263157895121));
#139144=CARTESIAN_POINT('Origin',(-11.9672956534849,-1.4,-16.9000000000405));
#139145=CARTESIAN_POINT('Origin',(-11.9672956534849,-0.999999999999995,
-16.9000000000405));
#139146=CARTESIAN_POINT('Origin',(-15.5,-1.4,-15.5));
#139147=CARTESIAN_POINT('',(-12.9679245658186,-0.999999999999996,-12.9409779220149));
#139148=CARTESIAN_POINT('',(-13.2492662807277,-1.4,-13.2253137084577));
#139149=CARTESIAN_POINT('Origin',(-12.9679245658186,-1.4,-12.9409779220149));
#139150=CARTESIAN_POINT('Origin',(-15.5,-1.4,-15.5));
#139151=CARTESIAN_POINT('Origin',(-15.5,-0.999999999999996,-15.5));
#139152=CARTESIAN_POINT('Ctrl Pts',(-13.2492662807277,-1.4,-13.2253137084577));
#139153=CARTESIAN_POINT('Ctrl Pts',(-13.5568224579683,-1.4,-12.9209961147482));
#139154=CARTESIAN_POINT('Ctrl Pts',(-13.3652000170587,-1.4,-12.5330775148592));
#139155=CARTESIAN_POINT('Ctrl Pts',(-13.2492662807277,-0.999999999999995,
-13.2253137084577));
#139156=CARTESIAN_POINT('Ctrl Pts',(-13.5568224579683,-0.999999999999995,
-12.9209961147482));
#139157=CARTESIAN_POINT('Ctrl Pts',(-13.3652000170587,-0.999999999999995,
-12.5330775148592));
#139158=CARTESIAN_POINT('Ctrl Pts',(-12.9679245658186,-0.999999999999997,
-12.9409779220149));
#139159=CARTESIAN_POINT('Ctrl Pts',(-13.0704432915655,-0.999999999999997,
-12.8395387241117));
#139160=CARTESIAN_POINT('Ctrl Pts',(-13.0065691445957,-0.999999999999997,
-12.7102325241487));
#139161=CARTESIAN_POINT('',(-13.0065691445957,-0.999999999999996,-12.7102325241487));
#139162=CARTESIAN_POINT('',(-13.3652000170587,-1.4,-12.5330775148592));
#139163=CARTESIAN_POINT('Origin',(-13.0065691445957,-1.4,-12.7102325241487));
#139164=CARTESIAN_POINT('Origin',(-12.8272537083641,-1.4,-12.7988100287935));
#139165=CARTESIAN_POINT('Origin',(-12.8272537083641,-0.999999999999996,
-12.7988100287935));
#139166=CARTESIAN_POINT('Origin',(-11.9125686467803,-1.4,-10.4955485895535));
#139167=CARTESIAN_POINT('',(-10.0269206021976,-0.999999999999998,-6.678261084678));
#139168=CARTESIAN_POINT('',(-10.3855514746607,-1.4,-6.50110607538848));
#139169=CARTESIAN_POINT('Origin',(-10.0269206021976,-1.4,-6.678261084678));
#139170=CARTESIAN_POINT('',(-12.2711995192434,-1.4,-10.318393580264));
#139171=CARTESIAN_POINT('',(-11.9125686467803,-0.999999999999997,-10.4955485895535));
#139172=CARTESIAN_POINT('Ctrl Pts',(-10.3855514746607,-1.4,-6.50110607538848));
#139173=CARTESIAN_POINT('Ctrl Pts',(-10.1948244706177,-1.4,-6.11500018915609));
#139174=CARTESIAN_POINT('Ctrl Pts',(-9.76798833941153,-1.4,-6.17214441503704));
#139175=CARTESIAN_POINT('Ctrl Pts',(-10.3855514746607,-0.999999999999997,
-6.50110607538848));
#139176=CARTESIAN_POINT('Ctrl Pts',(-10.1948244706177,-0.999999999999997,
-6.11500018915609));
#139177=CARTESIAN_POINT('Ctrl Pts',(-9.76798833941153,-0.999999999999997,
-6.17214441503704));
#139178=CARTESIAN_POINT('Ctrl Pts',(-10.0269206021976,-0.999999999999998,
-6.678261084678));
#139179=CARTESIAN_POINT('Ctrl Pts',(-9.96334493418329,-0.999999999999998,
-6.54955912260054));
#139180=CARTESIAN_POINT('Ctrl Pts',(-9.82106622378125,-0.999999999999998,
-6.56860719789419));
#139181=CARTESIAN_POINT('',(-9.82106622378125,-0.999999999999998,-6.56860719789418));
#139182=CARTESIAN_POINT('Origin',(-9.82106622378125,-1.4,-6.56860719789418));
#139183=CARTESIAN_POINT('Origin',(-9.84760516596611,-1.4,-6.76683858932276));
#139184=CARTESIAN_POINT('Origin',(-9.84760516596611,-0.999999999999998,
-6.76683858932276));
#139185=CARTESIAN_POINT('Origin',(-9.35,-1.4,-3.05000000003699));
#139186=CARTESIAN_POINT('',(-8.03637226370819,-0.999999999999998,-6.34801185120503));
#139187=CARTESIAN_POINT('Origin',(-8.03637226370819,-1.4,-6.34801185120503));
#139188=CARTESIAN_POINT('Origin',(-9.35,-0.999999999999998,-3.05000000003699));
#139189=CARTESIAN_POINT('Ctrl Pts',(-8.18438665652981,-1.4,-5.97640488205934));
#139190=CARTESIAN_POINT('Ctrl Pts',(-7.77682733610448,-1.4,-5.81407034487284));
#139191=CARTESIAN_POINT('Ctrl Pts',(-7.49853797666954,-1.4,-6.15320473424437));
#139192=CARTESIAN_POINT('Ctrl Pts',(-8.18438665652981,-0.999999999999996,
-5.97640488205934));
#139193=CARTESIAN_POINT('Ctrl Pts',(-7.77682733610448,-0.999999999999996,
-5.81407034487284));
#139194=CARTESIAN_POINT('Ctrl Pts',(-7.49853797666954,-0.999999999999996,
-6.15320473424437));
#139195=CARTESIAN_POINT('Ctrl Pts',(-8.03637226370819,-0.999999999999998,
-6.34801185120503));
#139196=CARTESIAN_POINT('Ctrl Pts',(-7.90051915689975,-0.999999999999998,
-6.29390033880953));
#139197=CARTESIAN_POINT('Ctrl Pts',(-7.8077560370881,-0.999999999999998,
-6.40694513526671));
#139198=CARTESIAN_POINT('Origin',(-7.96236506729739,-1.4,-6.53381533577788));
#139199=CARTESIAN_POINT('Origin',(-7.96236506729739,-0.999999999999998,
-6.53381533577788));
#139200=CARTESIAN_POINT('Origin',(-12.8272537083641,-10.3,-12.7988100287935));
#139201=CARTESIAN_POINT('',(-13.3652000170587,-10.1,-12.5330775148592));
#139202=CARTESIAN_POINT('',(-13.3652000170587,-10.3,-12.5330775148592));
#139203=CARTESIAN_POINT('',(-13.4147698236169,-10.1,-12.6770528346803));
#139204=CARTESIAN_POINT('Origin',(-12.8272537083641,-10.1,-12.7988100287935));
#139205=CARTESIAN_POINT('',(-13.4147698236169,-10.3,-12.6770528346803));
#139206=CARTESIAN_POINT('',(-13.4147698236169,-10.3,-12.6770528346803));
#139207=CARTESIAN_POINT('',(-13.2492662807277,-10.3,-13.2253137084577));
#139208=CARTESIAN_POINT('Origin',(-12.8272537083641,-10.3,-12.7988100287935));
#139209=CARTESIAN_POINT('',(-13.2492662807277,-10.3,-13.2253137084577));
#139210=CARTESIAN_POINT('Origin',(-13.5898168899543,-10.3,-12.9877897209636));
#139211=CARTESIAN_POINT('',(-10.3855514746607,-10.1,-6.50110607538849));
#139212=CARTESIAN_POINT('',(-10.3855514746607,-10.3,-6.50110607538848));
#139213=CARTESIAN_POINT('',(-12.6826584637285,-10.1,-11.1513470532436));
#139214=CARTESIAN_POINT('Origin',(-9.84760516596611,-10.3,-6.76683858932276));
#139215=CARTESIAN_POINT('Origin',(-9.84760516596611,-10.1,-6.76683858932276));
#139216=CARTESIAN_POINT('Origin',(-7.96236506729739,-10.3,-6.53381533577788));
#139217=CARTESIAN_POINT('',(-7.49853797666954,-10.1,-6.15320473424437));
#139218=CARTESIAN_POINT('',(-7.49853797666954,-10.3,-6.15320473424437));
#139219=CARTESIAN_POINT('Origin',(-7.96236506729739,-10.1,-6.53381533577788));
#139220=CARTESIAN_POINT('Origin',(-5.6920614055489E-17,-10.3,-2.28766658394441E-15));
#139221=CARTESIAN_POINT('',(-1.3145195915239,-10.1,-9.61051707935543));
#139222=CARTESIAN_POINT('',(-1.3145195915239,-10.3,-9.61051707935543));
#139223=CARTESIAN_POINT('Origin',(-5.6920614055489E-17,-10.1,-2.23416185986609E-15));
#139224=CARTESIAN_POINT('Origin',(-15.3583079095877,-0.999999999999998,
-5.47267507566318));
#139225=CARTESIAN_POINT('Origin',(1.2059399467532,-1.4,-14.5360946469435));
#139226=CARTESIAN_POINT('',(0.80690597004293,-1.4,-16.9002451764429));
#139227=CARTESIAN_POINT('',(1.20690593664767,-0.999999999999996,-16.9000817254963));
#139228=CARTESIAN_POINT('Origin',(1.20690593664767,-1.4,-16.9000817254963));
#139229=CARTESIAN_POINT('',(1.20416970133443,-0.999999999999998,-10.2039196212706));
#139230=CARTESIAN_POINT('',(1.2059399467532,-0.999999999999997,-14.5360946469435));
#139231=CARTESIAN_POINT('',(0.804169734729696,-1.4,-10.2040830722172));
#139232=CARTESIAN_POINT('Origin',(1.20416970133443,-1.4,-10.2039196212706));
#139233=CARTESIAN_POINT('',(0.805939980148468,-1.4,-14.5362580978901));
#139234=CARTESIAN_POINT('Ctrl Pts',(0.804169734729695,-1.4,-10.2040830722172));
#139235=CARTESIAN_POINT('Ctrl Pts',(0.80395589875457,-1.4,-9.68077999728824));
#139236=CARTESIAN_POINT('Ctrl Pts',(1.32237339244619,-1.4,-9.60943957263028));
#139237=CARTESIAN_POINT('Ctrl Pts',(0.804169734729694,-0.999999999999995,
-10.2040830722172));
#139238=CARTESIAN_POINT('Ctrl Pts',(0.803955898754569,-0.999999999999995,
-9.68077999728824));
#139239=CARTESIAN_POINT('Ctrl Pts',(1.32237339244619,-0.999999999999995,
-9.60943957263028));
#139240=CARTESIAN_POINT('Ctrl Pts',(1.20416970133443,-0.999999999999997,
-10.2039196212706));
#139241=CARTESIAN_POINT('Ctrl Pts',(1.20409842267606,-0.999999999999997,
-10.029485262961));
#139242=CARTESIAN_POINT('Ctrl Pts',(1.37690425390659,-0.999999999999997,
-10.0057051214084));
#139243=CARTESIAN_POINT('',(1.37690425390659,-0.999999999999998,-10.0057051214084));
#139244=CARTESIAN_POINT('',(1.32237339244619,-1.4,-9.60943957263028));
#139245=CARTESIAN_POINT('Origin',(1.37690425390659,-1.4,-10.0057051214084));
#139246=CARTESIAN_POINT('Origin',(1.4041696846368,-1.4,-10.2038378957974));
#139247=CARTESIAN_POINT('Origin',(1.4041696846368,-0.999999999999998,-10.2038378957974));
#139248=CARTESIAN_POINT('Origin',(-5.6920614055489E-17,-1.4,9.32936375408611E-17));
#139249=CARTESIAN_POINT('',(5.63745932045745,-0.999999999999998,-8.38027760346821));
#139250=CARTESIAN_POINT('',(5.41419360512517,-1.4,-8.0483854216423));
#139251=CARTESIAN_POINT('Origin',(5.63745932045745,-1.4,-8.38027760346821));
#139252=CARTESIAN_POINT('Origin',(-5.6920614055489E-17,-1.4,9.32936375408611E-17));
#139253=CARTESIAN_POINT('Origin',(-5.41450564939261E-17,-1.,1.82113427247051E-16));
#139254=CARTESIAN_POINT('Ctrl Pts',(5.41419360512517,-1.4,-8.0483854216423));
#139255=CARTESIAN_POINT('Ctrl Pts',(5.79937046939362,-1.4,-7.78927480428087));
#139256=CARTESIAN_POINT('Ctrl Pts',(6.14689326954821,-1.4,-8.09705302340923));
#139257=CARTESIAN_POINT('Ctrl Pts',(5.41419360512517,-0.999999999999997,
-8.0483854216423));
#139258=CARTESIAN_POINT('Ctrl Pts',(5.79937046939362,-0.999999999999997,
-7.78927480428087));
#139259=CARTESIAN_POINT('Ctrl Pts',(6.14689326954821,-0.999999999999997,
-8.09705302340923));
#139260=CARTESIAN_POINT('Ctrl Pts',(5.63745932045745,-0.999999999999998,
-8.38027760346822));
#139261=CARTESIAN_POINT('Ctrl Pts',(5.76585160854694,-0.999999999999998,
-8.29390739768107));
#139262=CARTESIAN_POINT('Ctrl Pts',(5.8816925419318,-0.999999999999998,
-8.39650013739052));
#139263=CARTESIAN_POINT('',(5.8816925419318,-0.999999999999998,-8.39650013739052));
#139264=CARTESIAN_POINT('',(6.14689326954821,-1.4,-8.09705302340923));
#139265=CARTESIAN_POINT('Origin',(5.8816925419318,-1.4,-8.39650013739052));
#139266=CARTESIAN_POINT('Origin',(5.74909217812359,-1.4,-8.54622369438117));
#139267=CARTESIAN_POINT('Origin',(5.74909217812359,-0.999999999999998,-8.54622369438117));
#139268=CARTESIAN_POINT('Origin',(8.6,-1.4,-5.32716721908225));
#139269=CARTESIAN_POINT('',(7.1958904109589,-0.999999999999998,-9.17924149951387));
#139270=CARTESIAN_POINT('',(7.33287671232876,-1.4,-8.80342937459372));
#139271=CARTESIAN_POINT('Origin',(7.1958904109589,-1.4,-9.17924149951387));
#139272=CARTESIAN_POINT('Origin',(8.6,-1.4,-5.32716721908225));
#139273=CARTESIAN_POINT('Origin',(8.6,-0.999999999999999,-5.32716721908225));
#139274=CARTESIAN_POINT('Origin',(6.1,-1.4,-12.1857384988751));
#139275=CARTESIAN_POINT('',(9.3,-0.999999999999997,-12.1857384988752));
#139276=CARTESIAN_POINT('',(9.7,-1.4,-12.1857384988752));
#139277=CARTESIAN_POINT('Origin',(9.3,-1.4,-12.1857384988752));
#139278=CARTESIAN_POINT('Origin',(6.1,-1.4,-12.1857384988751));
#139279=CARTESIAN_POINT('Origin',(6.1,-0.999999999999997,-12.1857384988751));
#139280=CARTESIAN_POINT('Origin',(9.3,-1.4,-11.8807427340099));
#139281=CARTESIAN_POINT('',(9.3,-0.999999999999997,-15.1));
#139282=CARTESIAN_POINT('',(9.7,-1.4,-15.1));
#139283=CARTESIAN_POINT('Origin',(9.3,-1.4,-15.1));
#139284=CARTESIAN_POINT('',(9.7,-1.4,-11.8807427340099));
#139285=CARTESIAN_POINT('',(9.3,-0.999999999999997,-11.8807427340099));
#139286=CARTESIAN_POINT('Origin',(15.1,-1.4,-15.1));
#139287=CARTESIAN_POINT('',(9.56715263178558,-0.999999999999996,-16.8400000000123));
#139288=CARTESIAN_POINT('',(9.94872831235209,-1.4,-16.7200000000114));
#139289=CARTESIAN_POINT('Origin',(9.56715263178558,-1.4,-16.8400000000123));
#139290=CARTESIAN_POINT('Origin',(15.1,-1.4,-15.1));
#139291=CARTESIAN_POINT('Origin',(15.1,-0.999999999999997,-15.1));
#139292=CARTESIAN_POINT('Ctrl Pts',(9.94872831235209,-1.4,-16.7200000000114));
#139293=CARTESIAN_POINT('Ctrl Pts',(10.0399069451865,-1.4,-17.0099295739836));
#139294=CARTESIAN_POINT('Ctrl Pts',(9.86010025640058,-1.4,-17.2549647869982));
#139295=CARTESIAN_POINT('Ctrl Pts',(9.68029356761475,-1.4,-17.5000000000127));
#139296=CARTESIAN_POINT('Ctrl Pts',(9.37636479150232,-1.4,-17.5000000000127));
#139297=CARTESIAN_POINT('Ctrl Pts',(9.94872831235209,-0.999999999999947,
-16.7200000000114));
#139298=CARTESIAN_POINT('Ctrl Pts',(10.0399069451865,-0.999999999999947,
-17.0099295739836));
#139299=CARTESIAN_POINT('Ctrl Pts',(9.86010025640058,-0.999999999999947,
-17.2549647869982));
#139300=CARTESIAN_POINT('Ctrl Pts',(9.68029356761475,-0.999999999999947,
-17.5000000000127));
#139301=CARTESIAN_POINT('Ctrl Pts',(9.37636479150232,-0.999999999999947,
-17.5000000000127));
#139302=CARTESIAN_POINT('Ctrl Pts',(9.56715263178553,-0.999999999999996,
-16.8400000000123));
#139303=CARTESIAN_POINT('Ctrl Pts',(9.59754550939699,-0.999999999999996,
-16.9366431913363));
#139304=CARTESIAN_POINT('Ctrl Pts',(9.53760994646837,-0.999999999999996,
-17.0183215956745));
#139305=CARTESIAN_POINT('Ctrl Pts',(9.47767438353977,-0.999999999999996,
-17.1000000000126));
#139306=CARTESIAN_POINT('Ctrl Pts',(9.37636479150232,-0.999999999999996,
-17.1000000000126));
#139307=CARTESIAN_POINT('',(9.37636479150258,-0.999999999999996,-17.1000000000127));
#139308=CARTESIAN_POINT('',(9.3763647915031,-1.4,-17.5000000000127));
#139309=CARTESIAN_POINT('Origin',(9.37636479150258,-1.4,-17.1000000000127));
#139310=CARTESIAN_POINT('Origin',(9.37636479150232,-1.4,-16.9000000000127));
#139311=CARTESIAN_POINT('Origin',(9.37636479150232,-0.999999999999996,-16.9000000000127));
#139312=CARTESIAN_POINT('Origin',(1.35908660826565,-1.4,-17.1000000000231));
#139313=CARTESIAN_POINT('',(1.40690591995029,-0.999999999999996,-17.1000000000231));
#139314=CARTESIAN_POINT('',(1.40690591995081,-1.4,-17.5000000000231));
#139315=CARTESIAN_POINT('Origin',(1.40690591995029,-1.4,-17.1000000000231));
#139316=CARTESIAN_POINT('',(1.35908660826617,-1.4,-17.5000000000231));
#139317=CARTESIAN_POINT('',(1.35908660826565,-0.999999999999996,-17.1000000000231));
#139318=CARTESIAN_POINT('Ctrl Pts',(1.40690591995003,-1.4,-17.5000000000231));
#139319=CARTESIAN_POINT('Ctrl Pts',(0.807151046297258,-1.4,-17.5000000000232));
#139320=CARTESIAN_POINT('Ctrl Pts',(0.806905970042931,-1.4,-16.9002451764429));
#139321=CARTESIAN_POINT('Ctrl Pts',(1.40690591995003,-0.999999999999993,
-17.5000000000231));
#139322=CARTESIAN_POINT('Ctrl Pts',(0.807151046297256,-0.999999999999993,
-17.5000000000232));
#139323=CARTESIAN_POINT('Ctrl Pts',(0.806905970042928,-0.999999999999994,
-16.9002451764429));
#139324=CARTESIAN_POINT('Ctrl Pts',(1.40690591995003,-0.999999999999996,
-17.1000000000231));
#139325=CARTESIAN_POINT('Ctrl Pts',(1.20698762873244,-0.999999999999996,
-17.1000000000231));
#139326=CARTESIAN_POINT('Ctrl Pts',(1.20690593664767,-0.999999999999996,
-16.9000817254963));
#139327=CARTESIAN_POINT('Origin',(1.40690591995003,-1.4,-16.9000000000231));
#139328=CARTESIAN_POINT('Origin',(1.40690591995003,-0.999999999999996,-16.9000000000231));
#139329=CARTESIAN_POINT('Origin',(9.7,-10.3,-12.1857384988752));
#139330=CARTESIAN_POINT('',(9.7,-10.3,-15.1));
#139331=CARTESIAN_POINT('',(9.7,-10.3,-15.1));
#139332=CARTESIAN_POINT('',(9.7,-10.3,-13.400000000037));
#139333=CARTESIAN_POINT('',(9.7,-10.3,-6.31786924944886));
#139334=CARTESIAN_POINT('',(9.7,-7.5,-13.400000000037));
#139335=CARTESIAN_POINT('',(9.7,-10.3,-13.400000000037));
#139336=CARTESIAN_POINT('',(9.7,-7.5,-12.1857384988752));
#139337=CARTESIAN_POINT('',(9.7,-7.5,-6.9928692494393));
#139338=CARTESIAN_POINT('',(9.7,-10.3,-12.1857384988752));
#139339=CARTESIAN_POINT('Origin',(15.1,-10.3,-15.1));
#139340=CARTESIAN_POINT('',(9.94872831235209,-10.3,-16.7200000000114));
#139341=CARTESIAN_POINT('',(9.94872831235209,-10.3,-16.7200000000114));
#139342=CARTESIAN_POINT('Origin',(15.1,-10.3,-15.1));
#139343=CARTESIAN_POINT('Origin',(9.37636479150232,-10.3,-16.9000000000127));
#139344=CARTESIAN_POINT('',(9.3763647915031,-10.3,-17.5000000000127));
#139345=CARTESIAN_POINT('',(9.3763647915031,-10.3,-17.5000000000127));
#139346=CARTESIAN_POINT('Origin',(9.37636479150232,-10.3,-16.9000000000127));
#139347=CARTESIAN_POINT('Origin',(9.81984848702787,-10.3,-17.5000000000121));
#139348=CARTESIAN_POINT('',(1.40690591995081,-10.3,-17.5000000000231));
#139349=CARTESIAN_POINT('',(1.40690591995081,-10.3,-17.5000000000231));
#139350=CARTESIAN_POINT('',(4.90992424351377,-10.3,-17.5000000000185));
#139351=CARTESIAN_POINT('Origin',(1.40690591995003,-10.3,-16.9000000000231));
#139352=CARTESIAN_POINT('',(0.806905970042931,-10.3,-16.9002451764429));
#139353=CARTESIAN_POINT('',(0.80690597004293,-10.3,-16.9002451764429));
#139354=CARTESIAN_POINT('Origin',(1.40690591995003,-10.3,-16.9000000000231));
#139355=CARTESIAN_POINT('Origin',(0.807151046297361,-10.3,-17.5000000000239));
#139356=CARTESIAN_POINT('',(0.804169734729696,-7.5,-10.2040830722172));
#139357=CARTESIAN_POINT('',(0.804169734729696,-10.3,-10.2040830722172));
#139358=CARTESIAN_POINT('',(0.803800167715777,-7.5,-9.29967232166704));
#139359=CARTESIAN_POINT('',(0.8039501151761,-7.5,-9.66662632470086));
#139360=CARTESIAN_POINT('',(0.803800167715815,-10.3,-9.29967232166704));
#139361=CARTESIAN_POINT('',(0.803800167715815,2.06492719942056E-15,-9.29967232166704));
#139362=CARTESIAN_POINT('',(0.803667430903156,-10.3,-8.97483651150704));
#139363=CARTESIAN_POINT('Origin',(-7.10167527050325,-0.999999999999997,
-11.5757469691446));
#139364=CARTESIAN_POINT('Origin',(6.1,-1.4,-12.1857384988751));
#139365=CARTESIAN_POINT('',(10.9,-1.4,-12.1857384988751));
#139366=CARTESIAN_POINT('',(11.3,-0.999999999999998,-12.1857384988751));
#139367=CARTESIAN_POINT('Origin',(11.3,-1.4,-12.1857384988751));
#139368=CARTESIAN_POINT('',(10.2531207906145,-0.999999999999999,-9.05658722439743));
#139369=CARTESIAN_POINT('Origin',(6.1,-0.999999999999998,-12.1857384988751));
#139370=CARTESIAN_POINT('',(9.93364996056724,-1.4,-9.29729116858802));
#139371=CARTESIAN_POINT('Origin',(10.2531207906145,-1.4,-9.05658722439743));
#139372=CARTESIAN_POINT('Origin',(6.1,-1.4,-12.1857384988751));
#139373=CARTESIAN_POINT('Ctrl Pts',(9.93364996056724,-1.4,-9.29729116858803));
#139374=CARTESIAN_POINT('Ctrl Pts',(9.73388216166068,-1.4,-9.03215224555127));
#139375=CARTESIAN_POINT('Ctrl Pts',(9.85238729399619,-1.4,-8.72205168831346));
#139376=CARTESIAN_POINT('Ctrl Pts',(9.97089242633171,-1.4,-8.41195113107564));
#139377=CARTESIAN_POINT('Ctrl Pts',(10.2965705850743,-1.4,-8.34761172707562));
#139378=CARTESIAN_POINT('Ctrl Pts',(9.93364996056724,-0.999999999999997,
-9.29729116858803));
#139379=CARTESIAN_POINT('Ctrl Pts',(9.73388216166068,-0.999999999999997,
-9.03215224555127));
#139380=CARTESIAN_POINT('Ctrl Pts',(9.85238729399619,-0.999999999999997,
-8.72205168831346));
#139381=CARTESIAN_POINT('Ctrl Pts',(9.97089242633171,-0.999999999999997,
-8.41195113107564));
#139382=CARTESIAN_POINT('Ctrl Pts',(10.2965705850743,-0.999999999999997,
-8.34761172707562));
#139383=CARTESIAN_POINT('Ctrl Pts',(10.2531207906145,-0.999999999999999,
-9.05658722439743));
#139384=CARTESIAN_POINT('Ctrl Pts',(10.1865315243123,-0.999999999999999,
-8.96820758338518));
#139385=CARTESIAN_POINT('Ctrl Pts',(10.2260332350908,-0.999999999999999,
-8.86484073097258));
#139386=CARTESIAN_POINT('Ctrl Pts',(10.2655349458693,-0.999999999999999,
-8.76147387855997));
#139387=CARTESIAN_POINT('Ctrl Pts',(10.3740943321169,-0.999999999999999,
-8.74002741055996));
#139388=CARTESIAN_POINT('',(10.3740943321169,-0.999999999999999,-8.74002741055996));
#139389=CARTESIAN_POINT('',(10.2965705850743,-1.4,-8.34761172707562));
#139390=CARTESIAN_POINT('Origin',(10.3740943321169,-1.4,-8.74002741055996));
#139391=CARTESIAN_POINT('Origin',(10.4128562056381,-1.4,-8.93623525230213));
#139392=CARTESIAN_POINT('Origin',(10.4128562056381,-0.999999999999999,-8.93623525230213));
#139393=CARTESIAN_POINT('Origin',(9.25,-1.4,-3.05000000003699));
#139394=CARTESIAN_POINT('',(11.7830419496669,-0.999999999999999,-8.26763341771092));
#139395=CARTESIAN_POINT('',(11.608349401414,-1.4,-7.90779663028513));
#139396=CARTESIAN_POINT('Origin',(11.7830419496669,-1.4,-8.26763341771092));
#139397=CARTESIAN_POINT('Origin',(9.25,-1.4,-3.05000000003699));
#139398=CARTESIAN_POINT('Origin',(9.25,-1.,-3.05000000003699));
#139399=CARTESIAN_POINT('Origin',(15.1,-1.4,-15.1));
#139400=CARTESIAN_POINT('',(14.0444055417443,-0.999999999999999,-7.57875248631252));
#139401=CARTESIAN_POINT('',(13.9888110834979,-1.4,-7.18263475607025));
#139402=CARTESIAN_POINT('Origin',(14.0444055417443,-1.4,-7.57875248631252));
#139403=CARTESIAN_POINT('Origin',(15.1,-1.4,-15.1));
#139404=CARTESIAN_POINT('Origin',(15.1,-0.999999999999998,-15.1));
#139405=CARTESIAN_POINT('Ctrl Pts',(13.9888110834979,-1.4,-7.18263475607025));
#139406=CARTESIAN_POINT('Ctrl Pts',(14.3498084270918,-1.4,-7.13196938511294));
#139407=CARTESIAN_POINT('Ctrl Pts',(14.6249042135416,-1.4,-7.37115209806196));
#139408=CARTESIAN_POINT('Ctrl Pts',(14.8999999999911,-1.4,-7.61033481101023));
#139409=CARTESIAN_POINT('Ctrl Pts',(14.8999999999907,-1.4,-7.97487021655479));
#139410=CARTESIAN_POINT('Ctrl Pts',(13.9888110834979,-0.999999999999998,
-7.18263475607025));
#139411=CARTESIAN_POINT('Ctrl Pts',(14.3498084270918,-0.999999999999998,
-7.13196938511294));
#139412=CARTESIAN_POINT('Ctrl Pts',(14.6249042135416,-0.999999999999998,
-7.37115209806196));
#139413=CARTESIAN_POINT('Ctrl Pts',(14.8999999999911,-0.999999999999998,
-7.61033481101023));
#139414=CARTESIAN_POINT('Ctrl Pts',(14.8999999999907,-0.999999999999998,
-7.97487021655479));
#139415=CARTESIAN_POINT('Ctrl Pts',(14.0444055417443,-0.999999999999999,
-7.57875248631252));
#139416=CARTESIAN_POINT('Ctrl Pts',(14.2249042135413,-0.999999999999999,
-7.55341980083387));
#139417=CARTESIAN_POINT('Ctrl Pts',(14.3624521067662,-0.999999999999999,
-7.67301115730838));
#139418=CARTESIAN_POINT('Ctrl Pts',(14.4999999999909,-0.999999999999999,
-7.79260251378251));
#139419=CARTESIAN_POINT('Ctrl Pts',(14.4999999999907,-0.999999999999999,
-7.97487021655479));
#139420=CARTESIAN_POINT('',(14.4999999999907,-0.999999999999999,-7.97487021655555));
#139421=CARTESIAN_POINT('',(14.8999999999907,-1.4,-7.9748702165563));
#139422=CARTESIAN_POINT('Origin',(14.4999999999907,-1.4,-7.97487021655555));
#139423=CARTESIAN_POINT('Origin',(14.0999999999907,-1.4,-7.97487021655479));
#139424=CARTESIAN_POINT('Origin',(14.0999999999907,-0.999999999999999,-7.97487021655479));
#139425=CARTESIAN_POINT('Origin',(14.4999999999885,-1.4,-9.18002967894291));
#139426=CARTESIAN_POINT('',(14.49999999999,-0.999999999999999,-8.38137084991965));
#139427=CARTESIAN_POINT('',(14.89999999999,-1.4,-8.3813708499204));
#139428=CARTESIAN_POINT('Origin',(14.49999999999,-1.4,-8.38137084991965));
#139429=CARTESIAN_POINT('',(14.8999999999885,-1.4,-9.18002967894366));
#139430=CARTESIAN_POINT('',(14.4999999999885,-0.999999999999999,-9.18002967894291));
#139431=CARTESIAN_POINT('Origin',(15.69999999999,-1.4,-8.38137084992191));
#139432=CARTESIAN_POINT('',(14.8514718625661,-0.999999999999999,-9.22989898734576));
#139433=CARTESIAN_POINT('',(15.1343145750407,-1.4,-8.94705627487115));
#139434=CARTESIAN_POINT('Origin',(14.8514718625661,-1.4,-9.22989898734576));
#139435=CARTESIAN_POINT('Origin',(15.69999999999,-1.4,-8.38137084992191));
#139436=CARTESIAN_POINT('Origin',(15.69999999999,-0.999999999999999,-8.38137084992191));
#139437=CARTESIAN_POINT('Origin',(14.895654763942,-1.4,-9.27408188872161));
#139438=CARTESIAN_POINT('',(16.9828427124746,-0.999999999999998,-11.3612698372543));
#139439=CARTESIAN_POINT('',(17.2656854249492,-1.4,-11.0784271247796));
#139440=CARTESIAN_POINT('Origin',(16.9828427124746,-1.4,-11.3612698372543));
#139441=CARTESIAN_POINT('',(15.1784974764166,-1.4,-8.991239176247));
#139442=CARTESIAN_POINT('',(14.895654763942,-0.999999999999999,-9.27408188872161));
#139443=CARTESIAN_POINT('Ctrl Pts',(17.2656854249492,-1.4,-11.0784271247796));
#139444=CARTESIAN_POINT('Ctrl Pts',(17.5,-1.4,-11.3127416998304));
#139445=CARTESIAN_POINT('Ctrl Pts',(17.5,-1.4,-11.6441125497289));
#139446=CARTESIAN_POINT('Ctrl Pts',(17.2656854249492,-0.999999999999998,
-11.0784271247796));
#139447=CARTESIAN_POINT('Ctrl Pts',(17.5,-0.999999999999998,-11.3127416998304));
#139448=CARTESIAN_POINT('Ctrl Pts',(17.5,-0.999999999999998,-11.6441125497289));
#139449=CARTESIAN_POINT('Ctrl Pts',(16.9828427124746,-0.999999999999998,
-11.3612698372543));
#139450=CARTESIAN_POINT('Ctrl Pts',(17.1,-0.999999999999998,-11.4784271247796));
#139451=CARTESIAN_POINT('Ctrl Pts',(17.1,-0.999999999999998,-11.6441125497289));
#139452=CARTESIAN_POINT('',(17.1,-0.999999999999998,-11.6441125497289));
#139453=CARTESIAN_POINT('',(17.5,-1.4,-11.6441125497289));
#139454=CARTESIAN_POINT('Origin',(17.1,-1.4,-11.6441125497289));
#139455=CARTESIAN_POINT('Origin',(16.7,-1.4,-11.6441125497289));
#139456=CARTESIAN_POINT('Origin',(16.7,-0.999999999999998,-11.6441125497289));
#139457=CARTESIAN_POINT('Origin',(17.1,-1.4,-9.52070091529622));
#139458=CARTESIAN_POINT('',(17.1,-0.999999999999998,-11.8673540249511));
#139459=CARTESIAN_POINT('',(17.5,-1.4,-11.8673540249511));
#139460=CARTESIAN_POINT('Origin',(17.1,-1.4,-11.8673540249511));
#139461=CARTESIAN_POINT('',(17.5,-1.4,-9.52070091529622));
#139462=CARTESIAN_POINT('',(17.1,-0.999999999999999,-9.52070091529622));
#139463=CARTESIAN_POINT('Ctrl Pts',(17.5,-1.4,-11.8673540249511));
#139464=CARTESIAN_POINT('Ctrl Pts',(17.5,-1.4,-12.2106641181924));
#139465=CARTESIAN_POINT('Ctrl Pts',(17.2040270258257,-1.4,-12.3846233624993));
#139466=CARTESIAN_POINT('Ctrl Pts',(16.9080540516514,-1.4,-12.5585826068061));
#139467=CARTESIAN_POINT('Ctrl Pts',(16.6081081081081,-1.4,-12.3915668857698));
#139468=CARTESIAN_POINT('Ctrl Pts',(17.5,-0.999999999999996,-11.8673540249511));
#139469=CARTESIAN_POINT('Ctrl Pts',(17.5,-0.999999999999996,-12.2106641181924));
#139470=CARTESIAN_POINT('Ctrl Pts',(17.2040270258257,-0.999999999999996,
-12.3846233624993));
#139471=CARTESIAN_POINT('Ctrl Pts',(16.9080540516514,-0.999999999999996,
-12.5585826068061));
#139472=CARTESIAN_POINT('Ctrl Pts',(16.6081081081081,-0.999999999999996,
-12.3915668857698));
#139473=CARTESIAN_POINT('Ctrl Pts',(17.1,-0.999999999999998,-11.8673540249511));
#139474=CARTESIAN_POINT('Ctrl Pts',(17.1,-0.999999999999998,-11.9817907226982));
#139475=CARTESIAN_POINT('Ctrl Pts',(17.0013423419419,-0.999999999999998,
-12.0397771374671));
#139476=CARTESIAN_POINT('Ctrl Pts',(16.9026846838838,-0.999999999999998,
-12.0977635522361));
#139477=CARTESIAN_POINT('Ctrl Pts',(16.8027027027027,-0.999999999999998,
-12.042091645224));
#139478=CARTESIAN_POINT('',(16.8027027027027,-0.999999999999998,-12.042091645224));
#139479=CARTESIAN_POINT('',(16.6081081081081,-1.4,-12.3915668857698));
#139480=CARTESIAN_POINT('Origin',(16.8027027027027,-1.4,-12.042091645224));
#139481=CARTESIAN_POINT('Origin',(16.9,-1.4,-11.8673540249511));
#139482=CARTESIAN_POINT('Origin',(16.9,-0.999999999999998,-11.8673540249511));
#139483=CARTESIAN_POINT('Origin',(15.1,-1.4,-15.1));
#139484=CARTESIAN_POINT('',(12.0487179487179,-0.999999999999998,-13.3854511253615));
#139485=CARTESIAN_POINT('',(12.3974358974359,-1.4,-13.5813995681774));
#139486=CARTESIAN_POINT('Origin',(12.0487179487179,-1.4,-13.3854511253615));
#139487=CARTESIAN_POINT('Origin',(15.1,-1.4,-15.1));
#139488=CARTESIAN_POINT('Origin',(15.1,-0.999999999999998,-15.1));
#139489=CARTESIAN_POINT('Ctrl Pts',(12.3974358974359,-1.4,-13.5813995681774));
#139490=CARTESIAN_POINT('Ctrl Pts',(12.0949042531665,-1.4,-14.1197973880112));
#139491=CARTESIAN_POINT('Ctrl Pts',(11.4974521265833,-1.4,-13.9634370201832));
#139492=CARTESIAN_POINT('Ctrl Pts',(10.9,-1.4,-13.8070766523552));
#139493=CARTESIAN_POINT('Ctrl Pts',(10.9,-1.4,-13.1895026825457));
#139494=CARTESIAN_POINT('Ctrl Pts',(12.3974358974359,-0.999999999999997,
-13.5813995681774));
#139495=CARTESIAN_POINT('Ctrl Pts',(12.0949042531665,-0.999999999999996,
-14.1197973880112));
#139496=CARTESIAN_POINT('Ctrl Pts',(11.4974521265833,-0.999999999999996,
-13.9634370201832));
#139497=CARTESIAN_POINT('Ctrl Pts',(10.9,-0.999999999999996,-13.8070766523552));
#139498=CARTESIAN_POINT('Ctrl Pts',(10.9,-0.999999999999997,-13.1895026825457));
#139499=CARTESIAN_POINT('Ctrl Pts',(12.0487179487179,-0.999999999999999,
-13.3854511253615));
#139500=CARTESIAN_POINT('Ctrl Pts',(11.8974521265833,-0.999999999999999,
-13.6546500352785));
#139501=CARTESIAN_POINT('Ctrl Pts',(11.5987260632916,-0.999999999999999,
-13.5764698513645));
#139502=CARTESIAN_POINT('Ctrl Pts',(11.3,-0.999999999999999,-13.4982896674504));
#139503=CARTESIAN_POINT('Ctrl Pts',(11.3,-0.999999999999999,-13.1895026825457));
#139504=CARTESIAN_POINT('',(11.3,-0.999999999999998,-13.1895026825457));
#139505=CARTESIAN_POINT('',(10.9,-1.4,-13.1895026825457));
#139506=CARTESIAN_POINT('Origin',(11.3,-1.4,-13.1895026825457));
#139507=CARTESIAN_POINT('Origin',(11.7,-1.4,-13.1895026825457));
#139508=CARTESIAN_POINT('Origin',(11.7,-0.999999999999998,-13.1895026825457));
#139509=CARTESIAN_POINT('Origin',(11.3,-1.4,-13.1762595651582));
#139510=CARTESIAN_POINT('',(10.9,-1.4,-13.1762595651582));
#139511=CARTESIAN_POINT('',(11.3,-0.999999999999998,-13.1762595651582));
#139512=CARTESIAN_POINT('Origin',(16.7,-4.55,-11.6441125497289));
#139513=CARTESIAN_POINT('',(17.5,-7.5,-11.6441125497289));
#139514=CARTESIAN_POINT('',(17.5,-4.55,-11.6441125497289));
#139515=CARTESIAN_POINT('',(17.2656854249492,-7.5,-11.0784271247796));
#139516=CARTESIAN_POINT('Origin',(16.7,-7.5,-11.6441125497289));
#139517=CARTESIAN_POINT('',(17.2656854249492,-4.55,-11.0784271247796));
#139518=CARTESIAN_POINT('Origin',(17.5,-7.5,-7.788882700276));
#139519=CARTESIAN_POINT('',(17.5,-7.5,-11.8673540249511));
#139520=CARTESIAN_POINT('',(17.5,-7.5,-11.8673540249511));
#139521=CARTESIAN_POINT('',(17.5,-7.5,-4.79444135013972));
#139522=CARTESIAN_POINT('Origin',(16.9,-7.5,-11.8673540249511));
#139523=CARTESIAN_POINT('',(16.6081081081081,-7.5,-12.3915668857698));
#139524=CARTESIAN_POINT('',(16.6081081081081,-7.5,-12.3915668857698));
#139525=CARTESIAN_POINT('Origin',(16.9,-7.5,-11.8673540249511));
#139526=CARTESIAN_POINT('Origin',(15.1,-7.5,-15.1));
#139527=CARTESIAN_POINT('',(12.3974358974359,-7.5,-13.5813995681774));
#139528=CARTESIAN_POINT('',(12.3974358974359,-7.5,-13.5813995681774));
#139529=CARTESIAN_POINT('Origin',(15.1,-7.5,-15.1));
#139530=CARTESIAN_POINT('Origin',(11.7,-7.5,-13.1895026825457));
#139531=CARTESIAN_POINT('',(10.9,-7.5,-13.1895026825457));
#139532=CARTESIAN_POINT('',(10.9,-7.5,-13.1895026825457));
#139533=CARTESIAN_POINT('Origin',(11.7,-7.5,-13.1895026825457));
#139534=CARTESIAN_POINT('Origin',(10.9,-10.3,-15.1));
#139535=CARTESIAN_POINT('',(10.9,-7.5,-12.1857384988751));
#139536=CARTESIAN_POINT('',(10.9,-8.9,-12.1857384988751));
#139537=CARTESIAN_POINT('',(10.9,-7.5,-12.5463002638159));
#139538=CARTESIAN_POINT('Origin',(6.1,-8.9,-12.1857384988751));
#139539=CARTESIAN_POINT('',(9.93364996056724,-7.5,-9.29729116858802));
#139540=CARTESIAN_POINT('',(9.93364996056724,-8.9,-9.29729116858802));
#139541=CARTESIAN_POINT('Origin',(6.1,-7.5,-12.1857384988751));
#139542=CARTESIAN_POINT('Origin',(13.4742124752016,-0.999999999999998,-11.2525191303165));
#139543=CARTESIAN_POINT('Origin',(15.1,-1.4,-15.1));
#139544=CARTESIAN_POINT('',(14.1784701326418,-1.4,-5.75034285186144));
#139545=CARTESIAN_POINT('',(14.1392350663191,-1.,-5.35227174066313));
#139546=CARTESIAN_POINT('Origin',(14.1392350663191,-1.4,-5.35227174066313));
#139547=CARTESIAN_POINT('',(10.822232934276,-1.,-6.28853108686908));
#139548=CARTESIAN_POINT('Origin',(15.1,-0.999999999999998,-15.1));
#139549=CARTESIAN_POINT('',(10.9969254825289,-1.4,-6.64836787429487));
#139550=CARTESIAN_POINT('Origin',(10.822232934276,-1.4,-6.28853108686908));
#139551=CARTESIAN_POINT('Origin',(15.1,-1.4,-15.1));
#139552=CARTESIAN_POINT('Origin',(9.24999999999998,-1.4,-3.05000000003696));
#139553=CARTESIAN_POINT('',(8.1053957606026,-1.,-6.46319222069398));
#139554=CARTESIAN_POINT('',(7.97821751178067,-1.4,-6.84243580076698));
#139555=CARTESIAN_POINT('Origin',(8.1053957606026,-1.4,-6.46319222069398));
#139556=CARTESIAN_POINT('Origin',(9.24999999999998,-1.4,-3.05000000003696));
#139557=CARTESIAN_POINT('Origin',(9.24999999999998,-1.,-3.05000000003696));
#139558=CARTESIAN_POINT('Ctrl Pts',(7.97821751178067,-1.4,-6.84243580076698));
#139559=CARTESIAN_POINT('Ctrl Pts',(7.68528093764713,-1.4,-6.74420035929417));
#139560=CARTESIAN_POINT('Ctrl Pts',(7.59510710075531,-1.4,-6.44868264820621));
#139561=CARTESIAN_POINT('Ctrl Pts',(7.5049332638635,-1.4,-6.15316493711826));
#139562=CARTESIAN_POINT('Ctrl Pts',(7.69312168782831,-1.4,-5.90811972595898));
#139563=CARTESIAN_POINT('Ctrl Pts',(7.97821751178067,-0.999999999999999,
-6.84243580076698));
#139564=CARTESIAN_POINT('Ctrl Pts',(7.68528093764713,-0.999999999999999,
-6.74420035929417));
#139565=CARTESIAN_POINT('Ctrl Pts',(7.59510710075531,-0.999999999999999,
-6.44868264820621));
#139566=CARTESIAN_POINT('Ctrl Pts',(7.5049332638635,-0.999999999999999,
-6.15316493711826));
#139567=CARTESIAN_POINT('Ctrl Pts',(7.69312168782831,-1.,-5.90811972595898));
#139568=CARTESIAN_POINT('Ctrl Pts',(8.1053957606026,-1.,-6.46319222069398));
#139569=CARTESIAN_POINT('Ctrl Pts',(8.00775023589142,-1.,-6.43044707353637));
#139570=CARTESIAN_POINT('Ctrl Pts',(7.97769229026082,-1.,-6.33194116984039));
#139571=CARTESIAN_POINT('Ctrl Pts',(7.94763434463021,-1.,-6.2334352661444));
#139572=CARTESIAN_POINT('Ctrl Pts',(8.01036381928515,-1.,-6.15175352909131));
#139573=CARTESIAN_POINT('',(8.01036381928515,-1.,-6.15175352909131));
#139574=CARTESIAN_POINT('',(7.69312168782831,-1.4,-5.90811972595898));
#139575=CARTESIAN_POINT('Origin',(8.01036381928515,-1.4,-6.15175352909131));
#139576=CARTESIAN_POINT('Origin',(8.16898488501357,-1.4,-6.27357043065747));
#139577=CARTESIAN_POINT('Origin',(8.16898488501357,-1.,-6.27357043065747));
#139578=CARTESIAN_POINT('Origin',(-2.12720466293355E-17,-1.4,-4.34446022993834E-16));
#139579=CARTESIAN_POINT('',(10.0541415178882,-1.,0.961373152462686));
#139580=CARTESIAN_POINT('',(9.65595769539761,-1.4,0.923298968206739));
#139581=CARTESIAN_POINT('Origin',(10.0541415178882,-1.4,0.961373152462686));
#139582=CARTESIAN_POINT('Origin',(-2.12720466293355E-17,-1.4,-4.34446022993834E-16));
#139583=CARTESIAN_POINT('Origin',(-1.84964890677726E-17,-1.,-3.45626233287644E-16));
#139584=CARTESIAN_POINT('Ctrl Pts',(9.65595769539761,-1.4,0.923298968206736));
#139585=CARTESIAN_POINT('Ctrl Pts',(9.60913873782649,-1.4,1.41293654954985));
#139586=CARTESIAN_POINT('Ctrl Pts',(10.0800826957381,-1.4,1.55488289278605));
#139587=CARTESIAN_POINT('Ctrl Pts',(9.65595769539761,-1.,0.923298968206736));
#139588=CARTESIAN_POINT('Ctrl Pts',(9.60913873782649,-1.,1.41293654954985));
#139589=CARTESIAN_POINT('Ctrl Pts',(10.0800826957381,-1.,1.55488289278605));
#139590=CARTESIAN_POINT('Ctrl Pts',(10.0541415178882,-1.,0.961373152462686));
#139591=CARTESIAN_POINT('Ctrl Pts',(10.0385351986979,-1.,1.12458567957706));
#139592=CARTESIAN_POINT('Ctrl Pts',(10.1955165180017,-1.,1.17190112732246));
#139593=CARTESIAN_POINT('',(10.1955165180017,-1.,1.17190112732246));
#139594=CARTESIAN_POINT('',(10.0800826957381,-1.4,1.55488289278605));
#139595=CARTESIAN_POINT('Origin',(10.1955165180017,-1.4,1.17190112732246));
#139596=CARTESIAN_POINT('Origin',(10.2532334291335,-1.4,0.980410244590661));
#139597=CARTESIAN_POINT('Origin',(10.2532334291335,-1.,0.980410244590661));
#139598=CARTESIAN_POINT('Origin',(15.1,-1.4,-15.1));
#139599=CARTESIAN_POINT('',(14.07589629876,-1.,1.86407781553888));
#139600=CARTESIAN_POINT('',(14.0517925975114,-1.4,2.2633509195493));
#139601=CARTESIAN_POINT('Origin',(14.07589629876,-1.4,1.86407781553888));
#139602=CARTESIAN_POINT('Origin',(15.1,-1.4,-15.1));
#139603=CARTESIAN_POINT('Origin',(15.1,-0.999999999999998,-15.1));
#139604=CARTESIAN_POINT('Ctrl Pts',(14.0517925975114,-1.4,2.2633509195493));
#139605=CARTESIAN_POINT('Ctrl Pts',(14.3967534618246,-1.4,2.2841758474804));
#139606=CARTESIAN_POINT('Ctrl Pts',(14.6483767309169,-1.4,2.04728472062595));
#139607=CARTESIAN_POINT('Ctrl Pts',(14.9000000000088,-1.4,1.81039359377226));
#139608=CARTESIAN_POINT('Ctrl Pts',(14.9000000000085,-1.4,1.46480471152845));
#139609=CARTESIAN_POINT('Ctrl Pts',(14.0517925975114,-1.,2.2633509195493));
#139610=CARTESIAN_POINT('Ctrl Pts',(14.3967534618246,-1.,2.2841758474804));
#139611=CARTESIAN_POINT('Ctrl Pts',(14.6483767309169,-1.,2.04728472062595));
#139612=CARTESIAN_POINT('Ctrl Pts',(14.9000000000088,-1.,1.81039359377226));
#139613=CARTESIAN_POINT('Ctrl Pts',(14.9000000000085,-1.,1.46480471152845));
#139614=CARTESIAN_POINT('Ctrl Pts',(14.07589629876,-1.,1.86407781553887));
#139615=CARTESIAN_POINT('Ctrl Pts',(14.2483767309166,-1.,1.87449027950442));
#139616=CARTESIAN_POINT('Ctrl Pts',(14.3741883654627,-1.,1.7560447160772));
#139617=CARTESIAN_POINT('Ctrl Pts',(14.5000000000087,-1.,1.63759915265035));
#139618=CARTESIAN_POINT('Ctrl Pts',(14.5000000000085,-1.,1.46480471152845));
#139619=CARTESIAN_POINT('',(14.5000000000085,-1.,1.46480471152769));
#139620=CARTESIAN_POINT('',(14.9000000000085,-1.4,1.46480471152694));
#139621=CARTESIAN_POINT('Origin',(14.5000000000085,-1.4,1.46480471152769));
#139622=CARTESIAN_POINT('Origin',(14.1000000000085,-1.4,1.46480471152845));
#139623=CARTESIAN_POINT('Origin',(14.1000000000085,-1.,1.46480471152845));
#139624=CARTESIAN_POINT('Origin',(14.5000000000057,-1.4,-0.0418535935887179));
#139625=CARTESIAN_POINT('',(14.4999999999964,-1.,-4.95420062946558));
#139626=CARTESIAN_POINT('',(14.8999999999964,-1.4,-4.95420062946633));
#139627=CARTESIAN_POINT('Origin',(14.4999999999964,-1.4,-4.95420062946558));
#139628=CARTESIAN_POINT('',(14.9000000000057,-1.4,-0.0418535935894708));
#139629=CARTESIAN_POINT('',(14.5000000000057,-1.,-0.0418535935887179));
#139630=CARTESIAN_POINT('Ctrl Pts',(14.8999999999964,-1.4,-4.95420062946483));
#139631=CARTESIAN_POINT('Ctrl Pts',(14.8999999999957,-1.4,-5.67922673365207));
#139632=CARTESIAN_POINT('Ctrl Pts',(14.1784701326418,-1.4,-5.75034285186144));
#139633=CARTESIAN_POINT('Ctrl Pts',(14.8999999999964,-0.999999999999999,
-4.95420062946483));
#139634=CARTESIAN_POINT('Ctrl Pts',(14.8999999999957,-0.999999999999998,
-5.67922673365208));
#139635=CARTESIAN_POINT('Ctrl Pts',(14.1784701326418,-0.999999999999998,
-5.75034285186144));
#139636=CARTESIAN_POINT('Ctrl Pts',(14.4999999999964,-1.,-4.95420062946483));
#139637=CARTESIAN_POINT('Ctrl Pts',(14.4999999999961,-1.,-5.31671368155845));
#139638=CARTESIAN_POINT('Ctrl Pts',(14.1392350663191,-1.,-5.35227174066313));
#139639=CARTESIAN_POINT('Origin',(14.0999999999964,-1.4,-4.95420062946483));
#139640=CARTESIAN_POINT('Origin',(14.0999999999964,-1.,-4.95420062946483));
#139641=CARTESIAN_POINT('Origin',(15.1,-7.5,-15.1));
#139642=CARTESIAN_POINT('',(14.0517925975114,-6.6,2.2633509195493));
#139643=CARTESIAN_POINT('',(14.0517925975114,-7.5,2.2633509195493));
#139644=CARTESIAN_POINT('',(10.0800826957381,-6.6,1.55488289278605));
#139645=CARTESIAN_POINT('Origin',(15.1,-6.6,-15.1));
#139646=CARTESIAN_POINT('',(10.0800826957381,-7.5,1.55488289278604));
#139647=CARTESIAN_POINT('Origin',(14.1000000000085,-7.5,1.46480471152845));
#139648=CARTESIAN_POINT('',(14.9000000000085,-6.6,1.46480471152694));
#139649=CARTESIAN_POINT('',(14.9000000000085,-7.5,1.46480471152694));
#139650=CARTESIAN_POINT('Origin',(14.1000000000085,-6.6,1.46480471152845));
#139651=CARTESIAN_POINT('Origin',(14.9000000000101,-1.6,2.29381194316098));
#139652=CARTESIAN_POINT('',(14.8999999999964,-6.6,-4.95420062946633));
#139653=CARTESIAN_POINT('',(14.8999999999964,-7.5,-4.95420062946633));
#139654=CARTESIAN_POINT('',(14.9000000000107,-6.6,2.61274169977414));
#139655=CARTESIAN_POINT('Origin',(14.0999999999964,-7.5,-4.95420062946483));
#139656=CARTESIAN_POINT('',(14.1784701326418,-6.6,-5.75034285186144));
#139657=CARTESIAN_POINT('',(14.1784701326418,-7.5,-5.75034285186144));
#139658=CARTESIAN_POINT('Origin',(14.0999999999964,-6.6,-4.95420062946483));
#139659=CARTESIAN_POINT('Origin',(15.1,-7.5,-15.1));
#139660=CARTESIAN_POINT('',(10.9969254825289,-6.6,-6.64836787429487));
#139661=CARTESIAN_POINT('',(10.9969254825289,-7.5,-6.64836787429487));
#139662=CARTESIAN_POINT('Origin',(15.1,-6.6,-15.1));
#139663=CARTESIAN_POINT('Origin',(12.2475425854112,-1.,-2.37751913033493));
#139664=CARTESIAN_POINT('Origin',(7.1,-1.4,10.2));
#139665=CARTESIAN_POINT('',(8.08895342530817,-1.4,6.7385016073135));
#139666=CARTESIAN_POINT('',(8.1988371392313,-1.,6.35389067479278));
#139667=CARTESIAN_POINT('Origin',(8.1988371392313,-1.4,6.35389067479278));
#139668=CARTESIAN_POINT('',(10.1654292935143,-1.,7.63034180357297));
#139669=CARTESIAN_POINT('Origin',(7.1,-1.,10.2));
#139670=CARTESIAN_POINT('',(9.85888636416284,-1.4,7.88730762321568));
#139671=CARTESIAN_POINT('Origin',(10.1654292935143,-1.4,7.63034180357297));
#139672=CARTESIAN_POINT('Origin',(7.1,-1.4,10.2));
#139673=CARTESIAN_POINT('Ctrl Pts',(9.85888636416284,-1.40000000000001,
7.88730762321567));
#139674=CARTESIAN_POINT('Ctrl Pts',(10.0378132267164,-1.40000000000001,
8.10075532868519));
#139675=CARTESIAN_POINT('Ctrl Pts',(10.3106112119491,-1.40000000000001,
8.15693365516831));
#139676=CARTESIAN_POINT('Ctrl Pts',(9.85888636416284,-1.,7.88730762321567));
#139677=CARTESIAN_POINT('Ctrl Pts',(10.0378132267164,-1.,8.10075532868519));
#139678=CARTESIAN_POINT('Ctrl Pts',(10.3106112119491,-1.,8.15693365516831));
#139679=CARTESIAN_POINT('Ctrl Pts',(10.1654292935143,-1.00000000000001,
7.63034180357297));
#139680=CARTESIAN_POINT('Ctrl Pts',(10.254892724791,-1.00000000000001,7.73706565630773));
#139681=CARTESIAN_POINT('Ctrl Pts',(10.3912917174074,-1.00000000000001,
7.76515481954929));
#139682=CARTESIAN_POINT('',(10.3912917174074,-1.,7.76515481954929));
#139683=CARTESIAN_POINT('',(10.3106112119491,-1.40000000000001,8.15693365516831));
#139684=CARTESIAN_POINT('Origin',(10.3912917174074,-1.40000000000001,7.76515481954929));
#139685=CARTESIAN_POINT('Origin',(10.4719722228657,-1.40000000000001,7.37337598393028));
#139686=CARTESIAN_POINT('Origin',(10.4719722228657,-1.,7.37337598393028));
#139687=CARTESIAN_POINT('Origin',(15.1,-1.4,-15.1));
#139688=CARTESIAN_POINT('',(13.5486494229367,-1.,8.19335849549308));
#139689=CARTESIAN_POINT('',(13.5220680886962,-1.4,8.5924743090986));
#139690=CARTESIAN_POINT('Origin',(13.5486494229367,-1.4,8.19335849549308));
#139691=CARTESIAN_POINT('Origin',(15.1,-1.4,-15.1));
#139692=CARTESIAN_POINT('Origin',(15.1,-0.999999999999998,-15.1));
#139693=CARTESIAN_POINT('Origin',(13.4954867544557,-1.40000000000001,8.99159012270412));
#139694=CARTESIAN_POINT('',(14.2949988360186,-1.,8.96365391975718));
#139695=CARTESIAN_POINT('',(13.8952427952371,-1.40000000000001,8.97762202123065));
#139696=CARTESIAN_POINT('Origin',(14.2949988360186,-1.40000000000001,8.96365391975718));
#139697=CARTESIAN_POINT('Origin',(13.4954867544557,-1.40000000000001,8.99159012270412));
#139698=CARTESIAN_POINT('Origin',(13.4954867544557,-1.,8.99159012270412));
#139699=CARTESIAN_POINT('Origin',(6.09999999999969,-1.4,9.24999999996331));
#139700=CARTESIAN_POINT('',(14.2987503886286,-1.,9.10684950238171));
#139701=CARTESIAN_POINT('',(13.8988113452808,-1.4,9.11383245348325));
#139702=CARTESIAN_POINT('Origin',(14.2987503886286,-1.4,9.10684950238171));
#139703=CARTESIAN_POINT('Origin',(6.09999999999969,-1.4,9.24999999996331));
#139704=CARTESIAN_POINT('Origin',(6.09999999999969,-1.,9.24999999996331));
#139705=CARTESIAN_POINT('Ctrl Pts',(13.8988113452808,-1.4,9.11383245348325));
#139706=CARTESIAN_POINT('Ctrl Pts',(13.9121679064567,-1.4,9.87881136017178));
#139707=CARTESIAN_POINT('Ctrl Pts',(14.6769816890462,-1.4,9.89957198073334));
#139708=CARTESIAN_POINT('Ctrl Pts',(13.8988113452808,-1.,9.11383245348325));
#139709=CARTESIAN_POINT('Ctrl Pts',(13.9121679064567,-1.,9.87881136017178));
#139710=CARTESIAN_POINT('Ctrl Pts',(14.6769816890462,-1.,9.89957198073334));
#139711=CARTESIAN_POINT('Ctrl Pts',(14.2987503886286,-1.,9.10684950238171));
#139712=CARTESIAN_POINT('Ctrl Pts',(14.3054286692165,-1.,9.48933895572597));
#139713=CARTESIAN_POINT('Ctrl Pts',(14.6878355605112,-1.,9.49971926600675));
#139714=CARTESIAN_POINT('',(14.6878355605112,-1.,9.49971926600675));
#139715=CARTESIAN_POINT('',(14.6769816890462,-1.4,9.89957198073334));
#139716=CARTESIAN_POINT('Origin',(14.6878355605112,-1.4,9.49971926600675));
#139717=CARTESIAN_POINT('Origin',(14.6986894319763,-1.4,9.09986655128017));
#139718=CARTESIAN_POINT('Origin',(14.6986894319763,-1.,9.09986655128017));
#139719=CARTESIAN_POINT('Origin',(12.9190134222136,-1.4,9.45170516624805));
#139720=CARTESIAN_POINT('',(16.8945730642675,-1.,9.55962043546442));
#139721=CARTESIAN_POINT('',(16.8837191928024,-1.4,9.959473150191));
#139722=CARTESIAN_POINT('Origin',(16.8945730642675,-1.4,9.55962043546442));
#139723=CARTESIAN_POINT('',(12.9081595507485,-1.4,9.85155788097463));
#139724=CARTESIAN_POINT('',(12.9190134222136,-1.,9.45170516624805));
#139725=CARTESIAN_POINT('Ctrl Pts',(16.8837191928024,-1.4,9.959473150191));
#139726=CARTESIAN_POINT('Ctrl Pts',(17.1369366949554,-1.4,9.96634665665939));
#139727=CARTESIAN_POINT('Ctrl Pts',(17.3184683474777,-1.4,9.78967575464012));
#139728=CARTESIAN_POINT('Ctrl Pts',(17.5,-1.4,9.61300485262085));
#139729=CARTESIAN_POINT('Ctrl Pts',(17.5,-1.4,9.35969407810112));
#139730=CARTESIAN_POINT('Ctrl Pts',(16.8837191928024,-1.,9.959473150191));
#139731=CARTESIAN_POINT('Ctrl Pts',(17.1369366949554,-1.,9.96634665665939));
#139732=CARTESIAN_POINT('Ctrl Pts',(17.3184683474777,-1.,9.78967575464012));
#139733=CARTESIAN_POINT('Ctrl Pts',(17.5,-1.,9.61300485262085));
#139734=CARTESIAN_POINT('Ctrl Pts',(17.5,-1.,9.35969407810112));
#139735=CARTESIAN_POINT('Ctrl Pts',(16.8945730642675,-1.,9.55962043546442));
#139736=CARTESIAN_POINT('Ctrl Pts',(16.9789788983185,-1.,9.56191160428721));
#139737=CARTESIAN_POINT('Ctrl Pts',(17.0394894491592,-1.,9.50302130361412));
#139738=CARTESIAN_POINT('Ctrl Pts',(17.1,-1.,9.44413100294103));
#139739=CARTESIAN_POINT('Ctrl Pts',(17.1,-1.,9.35969407810112));
#139740=CARTESIAN_POINT('',(17.1,-1.,9.35969407810112));
#139741=CARTESIAN_POINT('',(17.5,-1.4,9.35969407810112));
#139742=CARTESIAN_POINT('Origin',(17.1,-1.4,9.35969407810112));
#139743=CARTESIAN_POINT('Origin',(16.9,-1.4,9.35969407810112));
#139744=CARTESIAN_POINT('Origin',(16.9,-1.,9.35969407810112));
#139745=CARTESIAN_POINT('Origin',(17.1,-1.4,3.79934138063425));
#139746=CARTESIAN_POINT('',(17.1,-1.,5.54411254966196));
#139747=CARTESIAN_POINT('',(17.5,-1.4,5.54411254966196));
#139748=CARTESIAN_POINT('Origin',(17.1,-1.4,5.54411254966196));
#139749=CARTESIAN_POINT('',(17.5,-1.4,3.79934138063425));
#139750=CARTESIAN_POINT('',(17.1,-1.,3.79934138063425));
#139751=CARTESIAN_POINT('Ctrl Pts',(17.5,-1.4,5.54411254966196));
#139752=CARTESIAN_POINT('Ctrl Pts',(17.5,-1.4,5.21274169976348));
#139753=CARTESIAN_POINT('Ctrl Pts',(17.2656854249492,-1.4,4.97842712471272));
#139754=CARTESIAN_POINT('Ctrl Pts',(17.5,-1.,5.54411254966196));
#139755=CARTESIAN_POINT('Ctrl Pts',(17.5,-1.,5.21274169976348));
#139756=CARTESIAN_POINT('Ctrl Pts',(17.2656854249492,-1.,4.97842712471272));
#139757=CARTESIAN_POINT('Ctrl Pts',(17.1,-1.,5.54411254966196));
#139758=CARTESIAN_POINT('Ctrl Pts',(17.1,-1.,5.37842712471272));
#139759=CARTESIAN_POINT('Ctrl Pts',(16.9828427124746,-1.,5.26126983718734));
#139760=CARTESIAN_POINT('',(16.9828427124746,-1.,5.26126983718734));
#139761=CARTESIAN_POINT('',(17.2656854249492,-1.4,4.97842712471272));
#139762=CARTESIAN_POINT('Origin',(16.9828427124746,-1.4,5.26126983718734));
#139763=CARTESIAN_POINT('Origin',(16.7,-1.4,5.54411254966196));
#139764=CARTESIAN_POINT('Origin',(16.7,-1.,5.54411254966196));
#139765=CARTESIAN_POINT('Origin',(14.2407923014043,-1.4,2.51921942611707));
#139766=CARTESIAN_POINT('',(16.1199627900832,-1.,4.39838991479596));
#139767=CARTESIAN_POINT('',(16.4028055025579,-1.4,4.11554720232134));
#139768=CARTESIAN_POINT('Origin',(16.1199627900832,-1.4,4.39838991479596));
#139769=CARTESIAN_POINT('',(14.523635013879,-1.4,2.23637671364245));
#139770=CARTESIAN_POINT('',(14.2407923014043,-1.,2.51921942611707));
#139771=CARTESIAN_POINT('Ctrl Pts',(16.4028055025579,-1.4,4.11554720232134));
#139772=CARTESIAN_POINT('Ctrl Pts',(16.1560511668722,-1.4,3.86879286663565));
#139773=CARTESIAN_POINT('Ctrl Pts',(15.8073298678648,-1.4,3.88178748005695));
#139774=CARTESIAN_POINT('Ctrl Pts',(16.4028055025579,-1.,4.11554720232134));
#139775=CARTESIAN_POINT('Ctrl Pts',(16.1560511668722,-1.,3.86879286663565));
#139776=CARTESIAN_POINT('Ctrl Pts',(15.8073298678648,-1.,3.88178748005695));
#139777=CARTESIAN_POINT('Ctrl Pts',(16.1199627900832,-1.,4.39838991479596));
#139778=CARTESIAN_POINT('Ctrl Pts',(15.9965856222404,-1.,4.27501274695311));
#139779=CARTESIAN_POINT('Ctrl Pts',(15.8222249727367,-1.,4.28151005366376));
#139780=CARTESIAN_POINT('',(15.8222249727367,-1.,4.28151005366376));
#139781=CARTESIAN_POINT('',(15.8073298678648,-1.4,3.88178748005695));
#139782=CARTESIAN_POINT('Origin',(15.8222249727367,-1.4,4.28151005366376));
#139783=CARTESIAN_POINT('Origin',(15.8371200776086,-1.4,4.68123262727058));
#139784=CARTESIAN_POINT('Origin',(15.8371200776086,-1.,4.68123262727058));
#139785=CARTESIAN_POINT('Origin',(15.1,-1.4,-15.1));
#139786=CARTESIAN_POINT('',(9.66476438899747,-1.,3.51780746286748));
#139787=CARTESIAN_POINT('',(9.77686021437815,-1.4,3.13383542491129));
#139788=CARTESIAN_POINT('Origin',(9.66476438899747,-1.4,3.51780746286748));
#139789=CARTESIAN_POINT('Origin',(15.1,-1.4,-15.1));
#139790=CARTESIAN_POINT('Origin',(15.1,-0.999999999999998,-15.1));
#139791=CARTESIAN_POINT('Ctrl Pts',(9.77686021437815,-1.4,3.13383542491129));
#139792=CARTESIAN_POINT('Ctrl Pts',(9.24757706328966,-1.4,2.97931784077377));
#139793=CARTESIAN_POINT('Ctrl Pts',(9.04898541943487,-1.4,3.49368900717495));
#139794=CARTESIAN_POINT('Ctrl Pts',(9.77686021437815,-0.999999999999996,
3.13383542491129));
#139795=CARTESIAN_POINT('Ctrl Pts',(9.24757706328966,-0.999999999999996,
2.97931784077376));
#139796=CARTESIAN_POINT('Ctrl Pts',(9.04898541943487,-0.999999999999996,
3.49368900717495));
#139797=CARTESIAN_POINT('Ctrl Pts',(9.66476438899747,-1.,3.51780746286748));
#139798=CARTESIAN_POINT('Ctrl Pts',(9.48833667196797,-1.,3.4663016014883));
#139799=CARTESIAN_POINT('Ctrl Pts',(9.42213945734972,-1.,3.63775865695536));
#139800=CARTESIAN_POINT('',(9.42213945734971,-1.,3.63775865695536));
#139801=CARTESIAN_POINT('',(9.04898541943487,-1.4,3.49368900717495));
#139802=CARTESIAN_POINT('Origin',(9.42213945734971,-1.4,3.63775865695536));
#139803=CARTESIAN_POINT('Origin',(9.60871647630713,-1.4,3.70979348184556));
#139804=CARTESIAN_POINT('Origin',(9.60871647630713,-1.,3.70979348184556));
#139805=CARTESIAN_POINT('Origin',(-2.12720466293355E-17,-1.4,-4.34446022993834E-16));
#139806=CARTESIAN_POINT('',(8.09351144286873,-1.,6.04194277729877));
#139807=CARTESIAN_POINT('',(7.77297633622046,-1.4,5.8026579148315));
#139808=CARTESIAN_POINT('Origin',(8.09351144286873,-1.4,6.04194277729877));
#139809=CARTESIAN_POINT('Origin',(-2.12720466293355E-17,-1.4,-4.34446022993834E-16));
#139810=CARTESIAN_POINT('Origin',(-1.84964890677726E-17,-1.,-3.45626233287644E-16));
#139811=CARTESIAN_POINT('Ctrl Pts',(7.77297633622047,-1.4,5.80265791483149));
#139812=CARTESIAN_POINT('Ctrl Pts',(7.58454074891624,-1.4,6.05507764773938));
#139813=CARTESIAN_POINT('Ctrl Pts',(7.68530753049779,-1.4,6.35352320031752));
#139814=CARTESIAN_POINT('Ctrl Pts',(7.78607431207935,-1.4,6.65196875289566));
#139815=CARTESIAN_POINT('Ctrl Pts',(8.08895342530817,-1.4,6.7385016073135));
#139816=CARTESIAN_POINT('Ctrl Pts',(7.77297633622047,-1.,5.80265791483149));
#139817=CARTESIAN_POINT('Ctrl Pts',(7.58454074891624,-1.,6.05507764773938));
#139818=CARTESIAN_POINT('Ctrl Pts',(7.68530753049779,-1.,6.35352320031752));
#139819=CARTESIAN_POINT('Ctrl Pts',(7.78607431207935,-1.,6.65196875289566));
#139820=CARTESIAN_POINT('Ctrl Pts',(8.08895342530817,-1.,6.7385016073135));
#139821=CARTESIAN_POINT('Ctrl Pts',(8.09351144286873,-1.,6.04194277729878));
#139822=CARTESIAN_POINT('Ctrl Pts',(8.03069958043399,-1.,6.12608268826807));
#139823=CARTESIAN_POINT('Ctrl Pts',(8.06428850762784,-1.,6.22556453912745));
#139824=CARTESIAN_POINT('Ctrl Pts',(8.09787743482169,-1.,6.32504638998683));
#139825=CARTESIAN_POINT('Ctrl Pts',(8.1988371392313,-1.,6.35389067479278));
#139826=CARTESIAN_POINT('Origin',(8.25377899619286,-1.4,6.16158520853242));
#139827=CARTESIAN_POINT('Origin',(8.25377899619286,-1.,6.16158520853242));
#139828=CARTESIAN_POINT('Origin',(16.7,-4.55,5.54411254966196));
#139829=CARTESIAN_POINT('',(17.2656854249492,-7.5,4.97842712471272));
#139830=CARTESIAN_POINT('',(17.2656854249492,-4.55,4.97842712471272));
#139831=CARTESIAN_POINT('',(17.5,-7.5,5.54411254966196));
#139832=CARTESIAN_POINT('Origin',(16.7,-7.5,5.54411254966196));
#139833=CARTESIAN_POINT('',(17.5,-4.55,5.54411254966196));
#139834=CARTESIAN_POINT('Origin',(17.9686291501015,-1.6,5.68137084986501));
#139835=CARTESIAN_POINT('',(16.4028055025579,-7.5,4.11554720232134));
#139836=CARTESIAN_POINT('',(16.4028055025579,-7.5,4.11554720232134));
#139837=CARTESIAN_POINT('',(17.9686291501015,-7.5,5.68137084986501));
#139838=CARTESIAN_POINT('Origin',(15.8371200776086,-7.5,4.68123262727057));
#139839=CARTESIAN_POINT('',(15.8073298678648,-7.5,3.88178748005694));
#139840=CARTESIAN_POINT('',(15.8073298678648,-7.5,3.88178748005694));
#139841=CARTESIAN_POINT('Origin',(15.8371200776086,-7.5,4.68123262727057));
#139842=CARTESIAN_POINT('Origin',(15.1,-7.5,-15.1));
#139843=CARTESIAN_POINT('',(9.77686021437815,-7.5,3.13383542491129));
#139844=CARTESIAN_POINT('',(9.77686021437815,-7.5,3.13383542491129));
#139845=CARTESIAN_POINT('Origin',(15.1,-7.5,-15.1));
#139846=CARTESIAN_POINT('Origin',(9.60871647630713,-7.5,3.70979348184556));
#139847=CARTESIAN_POINT('',(9.04898541943487,-7.5,3.49368900717495));
#139848=CARTESIAN_POINT('',(9.04898541943487,-7.5,3.49368900717495));
#139849=CARTESIAN_POINT('Origin',(9.60871647630713,-7.5,3.70979348184556));
#139850=CARTESIAN_POINT('Origin',(-2.12720466293355E-17,-7.5,-1.66578428666901E-15));
#139851=CARTESIAN_POINT('',(7.77297633622046,-7.5,5.8026579148315));
#139852=CARTESIAN_POINT('',(7.77297633622046,-7.5,5.8026579148315));
#139853=CARTESIAN_POINT('Origin',(-2.12720466293355E-17,-7.5,-1.66578428666901E-15));
#139854=CARTESIAN_POINT('Origin',(8.25377899619286,-10.3,6.16158520853241));
#139855=CARTESIAN_POINT('',(8.08895342530817,-7.5,6.7385016073135));
#139856=CARTESIAN_POINT('',(8.08895342530817,-10.3,6.7385016073135));
#139857=CARTESIAN_POINT('Origin',(8.25377899619286,-7.5,6.16158520853241));
#139858=CARTESIAN_POINT('Origin',(7.1,-10.3,10.2));
#139859=CARTESIAN_POINT('',(9.85888636416284,-10.3,7.88730762321568));
#139860=CARTESIAN_POINT('',(9.85888636416284,-10.3,7.88730762321568));
#139861=CARTESIAN_POINT('',(6.86069632012767,-10.3,6.60796245164397));
#139862=CARTESIAN_POINT('Origin',(7.1,-10.3,10.2));
#139863=CARTESIAN_POINT('',(6.86069632012767,-7.5,6.60796245164398));
#139864=CARTESIAN_POINT('',(6.86069632012767,-1.92632982761137E-14,6.60796245164398));
#139865=CARTESIAN_POINT('Origin',(7.1,-7.5,10.2));
#139866=CARTESIAN_POINT('Origin',(12.2475425854112,-1.,-2.37751913033493));
#139867=CARTESIAN_POINT('Origin',(-8.47750127826606,-1.4,10.5062825051013));
#139868=CARTESIAN_POINT('',(-3.82759827224048,-1.4,10.4762486150055));
#139869=CARTESIAN_POINT('',(-3.42760661580818,-1.,10.4736650545671));
#139870=CARTESIAN_POINT('Origin',(-3.42760661580818,-1.4,10.4736650545671));
#139871=CARTESIAN_POINT('',(-6.8700032327,-1.,15.2936043068503));
#139872=CARTESIAN_POINT('Origin',(-8.47750127826606,-1.,10.5062825051013));
#139873=CARTESIAN_POINT('',(-6.99732981056662,-1.4,14.9144105007712));
#139874=CARTESIAN_POINT('Origin',(-6.8700032327,-1.4,15.2936043068503));
#139875=CARTESIAN_POINT('Origin',(-8.47750127826606,-1.4,10.5062825051013));
#139876=CARTESIAN_POINT('Ctrl Pts',(-6.99732981056662,-1.4,14.9144105007712));
#139877=CARTESIAN_POINT('Ctrl Pts',(-7.59675516644186,-1.4,15.1156869404874));
#139878=CARTESIAN_POINT('Ctrl Pts',(-7.53937602191996,-1.4,15.7453936946397));
#139879=CARTESIAN_POINT('Ctrl Pts',(-7.48199687739805,-1.4,16.3751004487919));
#139880=CARTESIAN_POINT('Ctrl Pts',(-6.85606479211595,-1.4,16.4647218026392));
#139881=CARTESIAN_POINT('Ctrl Pts',(-6.99732981056662,-1.,14.9144105007711));
#139882=CARTESIAN_POINT('Ctrl Pts',(-7.59675516644186,-1.,15.1156869404874));
#139883=CARTESIAN_POINT('Ctrl Pts',(-7.53937602191996,-1.,15.7453936946397));
#139884=CARTESIAN_POINT('Ctrl Pts',(-7.48199687739805,-1.,16.3751004487919));
#139885=CARTESIAN_POINT('Ctrl Pts',(-6.85606479211595,-1.,16.4647218026392));
#139886=CARTESIAN_POINT('Ctrl Pts',(-6.8700032327,-1.,15.2936043068503));
#139887=CARTESIAN_POINT('Ctrl Pts',(-7.16971591063762,-1.,15.3942425267084));
#139888=CARTESIAN_POINT('Ctrl Pts',(-7.14102633837667,-1.,15.7090959037845));
#139889=CARTESIAN_POINT('Ctrl Pts',(-7.11233676611572,-1.,16.0239492808607));
#139890=CARTESIAN_POINT('Ctrl Pts',(-6.79937072347466,-1.,16.0687599577843));
#139891=CARTESIAN_POINT('',(-6.79937072347466,-1.,16.0687599577843));
#139892=CARTESIAN_POINT('',(-6.85606479211595,-1.4,16.4647218026392));
#139893=CARTESIAN_POINT('Origin',(-6.79937072347466,-1.4,16.0687599577843));
#139894=CARTESIAN_POINT('Origin',(-6.74267665483338,-1.4,15.6727981129294));
#139895=CARTESIAN_POINT('Origin',(-6.74267665483338,-1.,15.6727981129294));
#139896=CARTESIAN_POINT('Origin',(-4.95681349263295,-1.4,3.2));
#139897=CARTESIAN_POINT('',(-4.95681349263295,-1.,16.2));
#139898=CARTESIAN_POINT('',(-4.95681349263295,-1.4,16.6));
#139899=CARTESIAN_POINT('Origin',(-4.95681349263295,-1.4,16.2));
#139900=CARTESIAN_POINT('Origin',(-4.95681349263295,-1.4,3.2));
#139901=CARTESIAN_POINT('Origin',(-4.95681349263295,-1.,3.2));
#139902=CARTESIAN_POINT('Origin',(-6.63837624017517,-1.4,16.2));
#139903=CARTESIAN_POINT('',(1.39248124878044,-1.,16.2));
#139904=CARTESIAN_POINT('',(1.39248124878044,-1.4,16.6));
#139905=CARTESIAN_POINT('Origin',(1.39248124878044,-1.4,16.2));
#139906=CARTESIAN_POINT('',(-6.63837624017517,-1.4,16.6));
#139907=CARTESIAN_POINT('',(-6.63837624017517,-1.,16.2));
#139908=CARTESIAN_POINT('Ctrl Pts',(1.39248124878044,-1.4,16.6));
#139909=CARTESIAN_POINT('Ctrl Pts',(1.87120813518912,-1.4,16.6));
#139910=CARTESIAN_POINT('Ctrl Pts',(2.09748000071234,-1.4,16.178122678207));
#139911=CARTESIAN_POINT('Ctrl Pts',(1.39248124878044,-1.,16.6));
#139912=CARTESIAN_POINT('Ctrl Pts',(1.87120813518912,-1.,16.6));
#139913=CARTESIAN_POINT('Ctrl Pts',(2.09748000071234,-1.,16.178122678207));
#139914=CARTESIAN_POINT('Ctrl Pts',(1.39248124878044,-1.,16.2));
#139915=CARTESIAN_POINT('Ctrl Pts',(1.63184469198478,-1.,16.2));
#139916=CARTESIAN_POINT('Ctrl Pts',(1.74498062474639,-1.,15.9890613391035));
#139917=CARTESIAN_POINT('',(1.74498062474639,-1.,15.9890613391035));
#139918=CARTESIAN_POINT('',(2.09748000071234,-1.4,16.178122678207));
#139919=CARTESIAN_POINT('Origin',(1.74498062474639,-1.4,15.9890613391035));
#139920=CARTESIAN_POINT('Origin',(1.39248124878044,-1.4,15.8));
#139921=CARTESIAN_POINT('Origin',(1.39248124878044,-1.,15.8));
#139922=CARTESIAN_POINT('Origin',(-8.47750127826606,-1.4,10.5062825051013));
#139923=CARTESIAN_POINT('',(3.12239099121706,-1.,10.5562758685179));
#139924=CARTESIAN_POINT('',(3.52238727637165,-1.4,10.5579997776013));
#139925=CARTESIAN_POINT('Origin',(3.12239099121706,-1.4,10.5562758685179));
#139926=CARTESIAN_POINT('Origin',(-8.47750127826606,-1.4,10.5062825051013));
#139927=CARTESIAN_POINT('Origin',(-8.47750127826606,-1.,10.5062825051013));
#139928=CARTESIAN_POINT('Ctrl Pts',(3.52238727637165,-1.4,10.5579997776013));
#139929=CARTESIAN_POINT('Ctrl Pts',(3.52408213740859,-1.4,10.1647434712322));
#139930=CARTESIAN_POINT('Ctrl Pts',(3.21373231632171,-1.4,9.92321421088415));
#139931=CARTESIAN_POINT('Ctrl Pts',(2.90338249523483,-1.4,9.68168495053607));
#139932=CARTESIAN_POINT('Ctrl Pts',(2.52258592029807,-1.4,9.77990594406283));
#139933=CARTESIAN_POINT('Ctrl Pts',(3.52238727637165,-1.,10.5579997776013));
#139934=CARTESIAN_POINT('Ctrl Pts',(3.52408213740859,-1.,10.1647434712322));
#139935=CARTESIAN_POINT('Ctrl Pts',(3.21373231632171,-1.,9.92321421088415));
#139936=CARTESIAN_POINT('Ctrl Pts',(2.90338249523483,-1.,9.68168495053607));
#139937=CARTESIAN_POINT('Ctrl Pts',(2.52258592029807,-1.,9.77990594406283));
#139938=CARTESIAN_POINT('Ctrl Pts',(3.12239099121706,-1.,10.5562758685179));
#139939=CARTESIAN_POINT('Ctrl Pts',(3.12323842173553,-1.,10.3596477153334));
#139940=CARTESIAN_POINT('Ctrl Pts',(2.96806351119209,-1.,10.2388830851594));
#139941=CARTESIAN_POINT('Ctrl Pts',(2.81288860064865,-1.,10.1181184549853));
#139942=CARTESIAN_POINT('Ctrl Pts',(2.62249031318027,-1.,10.1672289517487));
#139943=CARTESIAN_POINT('',(2.62249031318027,-1.,10.1672289517487));
#139944=CARTESIAN_POINT('',(2.52258592029807,-1.4,9.77990594406283));
#139945=CARTESIAN_POINT('Origin',(2.62249031318027,-1.4,10.1672289517487));
#139946=CARTESIAN_POINT('Origin',(2.72239470606247,-1.4,10.5545519594346));
#139947=CARTESIAN_POINT('Origin',(2.72239470606247,-1.,10.5545519594346));
#139948=CARTESIAN_POINT('Origin',(9.00768359641396E-11,-1.4,2.56054600265843E-10));
#139949=CARTESIAN_POINT('',(-2.91650982324592,-1.,10.0868216227845));
#139950=CARTESIAN_POINT('',(-2.80540468711597,-1.4,9.70256175144017));
#139951=CARTESIAN_POINT('Origin',(-2.91650982324592,-1.4,10.0868216227845));
#139952=CARTESIAN_POINT('Origin',(9.00768359641396E-11,-1.4,2.56054600265843E-10));
#139953=CARTESIAN_POINT('Origin',(9.00768387396972E-11,-1.,2.56054689085632E-10));
#139954=CARTESIAN_POINT('Ctrl Pts',(-2.80540468711597,-1.4,9.70256175144017));
#139955=CARTESIAN_POINT('Ctrl Pts',(-3.19065678822161,-1.4,9.59116972138524));
#139956=CARTESIAN_POINT('Ctrl Pts',(-3.51042264606467,-1.4,9.83319691391525));
#139957=CARTESIAN_POINT('Ctrl Pts',(-3.83018850390773,-1.4,10.0752241064453));
#139958=CARTESIAN_POINT('Ctrl Pts',(-3.82759827224048,-1.4,10.4762486150055));
#139959=CARTESIAN_POINT('Ctrl Pts',(-2.80540468711597,-1.,9.70256175144017));
#139960=CARTESIAN_POINT('Ctrl Pts',(-3.19065678822161,-1.,9.59116972138524));
#139961=CARTESIAN_POINT('Ctrl Pts',(-3.51042264606467,-1.,9.83319691391525));
#139962=CARTESIAN_POINT('Ctrl Pts',(-3.83018850390773,-1.,10.0752241064453));
#139963=CARTESIAN_POINT('Ctrl Pts',(-3.82759827224049,-1.,10.4762486150055));
#139964=CARTESIAN_POINT('Ctrl Pts',(-2.91650982324592,-1.,10.0868216227845));
#139965=CARTESIAN_POINT('Ctrl Pts',(-3.10913587379874,-1.,10.031125607757));
#139966=CARTESIAN_POINT('Ctrl Pts',(-3.26901880272027,-1.,10.152139204022));
#139967=CARTESIAN_POINT('Ctrl Pts',(-3.4289017316418,-1.,10.273152800287));
#139968=CARTESIAN_POINT('Ctrl Pts',(-3.42760661580818,-1.,10.4736650545671));
#139969=CARTESIAN_POINT('Origin',(-3.02761495937587,-1.4,10.4710814941288));
#139970=CARTESIAN_POINT('Origin',(-3.02761495937587,-1.,10.4710814941288));
#139971=CARTESIAN_POINT('Origin',(-8.47750127826606,-2.6,10.5062825051013));
#139972=CARTESIAN_POINT('',(3.52238727637165,-2.6,10.5579997776013));
#139973=CARTESIAN_POINT('',(3.52238727637165,-2.6,10.5579997776013));
#139974=CARTESIAN_POINT('',(3.51261604728234,-2.6,10.0193671946169));
#139975=CARTESIAN_POINT('Origin',(-8.47750127826606,-2.6,10.5062825051013));
#139976=CARTESIAN_POINT('',(3.51261604728234,-10.3,10.0193671946169));
#139977=CARTESIAN_POINT('',(3.51261604728234,-2.6,10.0193671946169));
#139978=CARTESIAN_POINT('',(1.22705833076043,-10.3,17.5647187904871));
#139979=CARTESIAN_POINT('Origin',(-8.47750127826606,-10.3,10.5062825051013));
#139980=CARTESIAN_POINT('',(1.22705833076043,-2.6,17.5647187904871));
#139981=CARTESIAN_POINT('',(1.22705833076043,-2.6,17.5647187904871));
#139982=CARTESIAN_POINT('',(2.09748000071234,-2.6,16.178122678207));
#139983=CARTESIAN_POINT('Origin',(-8.47750127826606,-2.6,10.5062825051013));
#139984=CARTESIAN_POINT('',(2.09748000071234,-2.6,16.178122678207));
#139985=CARTESIAN_POINT('Origin',(2.72239470606247,-2.6,10.5545519594346));
#139986=CARTESIAN_POINT('',(2.52258592029807,-2.6,9.77990594406283));
#139987=CARTESIAN_POINT('',(2.52258592029807,-2.6,9.77990594406283));
#139988=CARTESIAN_POINT('Origin',(2.72239470606247,-2.6,10.5545519594346));
#139989=CARTESIAN_POINT('Origin',(9.00768359641396E-11,-2.6,2.56054600265843E-10));
#139990=CARTESIAN_POINT('',(-2.80540468711597,-2.6,9.70256175144017));
#139991=CARTESIAN_POINT('',(-2.80540468711597,-2.6,9.70256175144017));
#139992=CARTESIAN_POINT('Origin',(9.00768359641396E-11,-2.6,2.56054600265843E-10));
#139993=CARTESIAN_POINT('Origin',(-3.02761495937587,-2.6,10.4710814941288));
#139994=CARTESIAN_POINT('',(-3.82759827224048,-2.6,10.4762486150055));
#139995=CARTESIAN_POINT('',(-3.82759827224048,-2.6,10.4762486150055));
#139996=CARTESIAN_POINT('Origin',(-3.02761495937587,-2.6,10.4710814941288));
#139997=CARTESIAN_POINT('Origin',(-8.47750127826606,-2.6,10.5062825051013));
#139998=CARTESIAN_POINT('',(-6.99732981056662,-2.6,14.9144105007712));
#139999=CARTESIAN_POINT('',(-6.99732981056662,-2.6,14.9144105007712));
#140000=CARTESIAN_POINT('Origin',(-8.47750127826606,-2.6,10.5062825051013));
#140001=CARTESIAN_POINT('Origin',(-8.31993898771739,-1.,8.19662125500606));
#140002=CARTESIAN_POINT('Origin',(5.39067671315598,-1.4,15.8));
#140003=CARTESIAN_POINT('',(4.34802179419235,-1.4,16.2));
#140004=CARTESIAN_POINT('',(4.34802179419235,-1.,15.8));
#140005=CARTESIAN_POINT('Origin',(4.34802179419235,-1.4,15.8));
#140006=CARTESIAN_POINT('',(9.34289321881345,-1.,15.8));
#140007=CARTESIAN_POINT('',(5.39067671315598,-1.,15.8));
#140008=CARTESIAN_POINT('',(9.34289321881345,-1.4,16.2));
#140009=CARTESIAN_POINT('Origin',(9.34289321881345,-1.4,15.8));
#140010=CARTESIAN_POINT('',(5.39067671315598,-1.4,16.2));
#140011=CARTESIAN_POINT('Ctrl Pts',(9.34289321881345,-1.4,16.2));
#140012=CARTESIAN_POINT('Ctrl Pts',(9.94289321881345,-1.4,16.2));
#140013=CARTESIAN_POINT('Ctrl Pts',(9.94289321881345,-1.4,15.6));
#140014=CARTESIAN_POINT('Ctrl Pts',(9.34289321881345,-1.,16.2));
#140015=CARTESIAN_POINT('Ctrl Pts',(9.94289321881345,-1.,16.2));
#140016=CARTESIAN_POINT('Ctrl Pts',(9.94289321881345,-1.,15.6));
#140017=CARTESIAN_POINT('Ctrl Pts',(9.34289321881345,-1.,15.8));
#140018=CARTESIAN_POINT('Ctrl Pts',(9.54289321881345,-1.,15.8));
#140019=CARTESIAN_POINT('Ctrl Pts',(9.54289321881345,-1.,15.6));
#140020=CARTESIAN_POINT('',(9.54289321881345,-1.,15.6));
#140021=CARTESIAN_POINT('',(9.94289321881345,-1.4,15.6));
#140022=CARTESIAN_POINT('Origin',(9.54289321881345,-1.4,15.6));
#140023=CARTESIAN_POINT('Origin',(9.34289321881345,-1.4,15.6));
#140024=CARTESIAN_POINT('Origin',(9.34289321881345,-1.,15.6));
#140025=CARTESIAN_POINT('Origin',(9.54289321881345,-1.4,15.2521525008107));
#140026=CARTESIAN_POINT('',(9.54289321881345,-1.,13.7509759234611));
#140027=CARTESIAN_POINT('',(9.94289321881345,-1.4,13.7509759234611));
#140028=CARTESIAN_POINT('Origin',(9.54289321881345,-1.4,13.7509759234611));
#140029=CARTESIAN_POINT('',(9.94289321881345,-1.4,15.2521525008107));
#140030=CARTESIAN_POINT('',(9.54289321881345,-1.,15.2521525008107));
#140031=CARTESIAN_POINT('Ctrl Pts',(9.94289321881345,-1.4,13.7509759234611));
#140032=CARTESIAN_POINT('Ctrl Pts',(9.94289321881345,-1.4,13.39656921145));
#140033=CARTESIAN_POINT('Ctrl Pts',(9.63250676288208,-1.4,13.2255009049379));
#140034=CARTESIAN_POINT('Ctrl Pts',(9.32212030695072,-1.4,13.0544325984258));
#140035=CARTESIAN_POINT('Ctrl Pts',(9.0224799018401,-1.4,13.243693648681));
#140036=CARTESIAN_POINT('Ctrl Pts',(9.94289321881345,-1.,13.7509759234611));
#140037=CARTESIAN_POINT('Ctrl Pts',(9.94289321881345,-1.,13.39656921145));
#140038=CARTESIAN_POINT('Ctrl Pts',(9.63250676288208,-1.,13.2255009049379));
#140039=CARTESIAN_POINT('Ctrl Pts',(9.32212030695072,-1.,13.0544325984258));
#140040=CARTESIAN_POINT('Ctrl Pts',(9.0224799018401,-1.,13.243693648681));
#140041=CARTESIAN_POINT('Ctrl Pts',(9.54289321881345,-1.,13.7509759234611));
#140042=CARTESIAN_POINT('Ctrl Pts',(9.54289321881345,-1.,13.6328403527907));
#140043=CARTESIAN_POINT('Ctrl Pts',(9.43943106683633,-1.,13.5758175839534));
#140044=CARTESIAN_POINT('Ctrl Pts',(9.3359689148592,-1.,13.518794815116));
#140045=CARTESIAN_POINT('Ctrl Pts',(9.23608877982233,-1.,13.5818818318677));
#140046=CARTESIAN_POINT('',(9.23608877982233,-1.,13.5818818318677));
#140047=CARTESIAN_POINT('',(9.0224799018401,-1.4,13.243693648681));
#140048=CARTESIAN_POINT('Origin',(9.23608877982233,-1.4,13.5818818318677));
#140049=CARTESIAN_POINT('Origin',(9.34289321881345,-1.4,13.7509759234611));
#140050=CARTESIAN_POINT('Origin',(9.34289321881345,-1.,13.7509759234611));
#140051=CARTESIAN_POINT('Origin',(7.1,-1.4,10.2));
#140052=CARTESIAN_POINT('',(5.02890240319562,-1.,13.6220687813823));
#140053=CARTESIAN_POINT('',(5.23601216287606,-1.4,13.279861903244));
#140054=CARTESIAN_POINT('Origin',(5.02890240319562,-1.4,13.6220687813823));
#140055=CARTESIAN_POINT('Origin',(7.1,-1.4,10.2));
#140056=CARTESIAN_POINT('Origin',(7.1,-1.,10.2));
#140057=CARTESIAN_POINT('Ctrl Pts',(5.23601216287606,-1.4,13.279861903244));
#140058=CARTESIAN_POINT('Ctrl Pts',(4.97614696981528,-1.4,13.1225868128749));
#140059=CARTESIAN_POINT('Ctrl Pts',(4.69555487551437,-1.4,13.2389201667807));
#140060=CARTESIAN_POINT('Ctrl Pts',(4.41496278121346,-1.4,13.3552535206864));
#140061=CARTESIAN_POINT('Ctrl Pts',(4.34261496676317,-1.4,13.6502639719579));
#140062=CARTESIAN_POINT('Ctrl Pts',(5.23601216287606,-1.,13.279861903244));
#140063=CARTESIAN_POINT('Ctrl Pts',(4.97614696981528,-1.,13.1225868128749));
#140064=CARTESIAN_POINT('Ctrl Pts',(4.69555487551437,-1.,13.2389201667807));
#140065=CARTESIAN_POINT('Ctrl Pts',(4.41496278121346,-1.,13.3552535206864));
#140066=CARTESIAN_POINT('Ctrl Pts',(4.34261496676317,-1.,13.6502639719579));
#140067=CARTESIAN_POINT('Ctrl Pts',(5.02890240319562,-1.,13.6220687813823));
#140068=CARTESIAN_POINT('Ctrl Pts',(4.94228067217536,-1.,13.5696437512592));
#140069=CARTESIAN_POINT('Ctrl Pts',(4.84874997407506,-1.,13.6084215358945));
#140070=CARTESIAN_POINT('Ctrl Pts',(4.75521927597476,-1.,13.6471993205297));
#140071=CARTESIAN_POINT('Ctrl Pts',(4.73110333782466,-1.,13.7455361376202));
#140072=CARTESIAN_POINT('',(4.73110333782466,-1.,13.7455361376202));
#140073=CARTESIAN_POINT('',(4.34261496676317,-1.4,13.6502639719579));
#140074=CARTESIAN_POINT('Origin',(4.73110333782466,-1.4,13.7455361376202));
#140075=CARTESIAN_POINT('Origin',(4.9253475233554,-1.4,13.7931722204514));
#140076=CARTESIAN_POINT('Origin',(4.9253475233554,-1.,13.7931722204514));
#140077=CARTESIAN_POINT('Origin',(-8.47750127826606,-1.4,10.5062825051013));
#140078=CARTESIAN_POINT('',(4.16214464821469,-1.,15.5261780073203));
#140079=CARTESIAN_POINT('',(3.79039035625937,-1.4,15.3785340219609));
#140080=CARTESIAN_POINT('Origin',(4.16214464821469,-1.4,15.5261780073203));
#140081=CARTESIAN_POINT('Origin',(-8.47750127826606,-1.4,10.5062825051013));
#140082=CARTESIAN_POINT('Origin',(-8.47750127826606,-1.,10.5062825051013));
#140083=CARTESIAN_POINT('Ctrl Pts',(3.79039035625937,-1.4,15.3785340219609));
#140084=CARTESIAN_POINT('Ctrl Pts',(3.67305500089253,-1.4,15.673973906285));
#140085=CARTESIAN_POINT('Ctrl Pts',(3.8515947669147,-1.4,15.9369869531425));
#140086=CARTESIAN_POINT('Ctrl Pts',(4.03013453293687,-1.4,16.2));
#140087=CARTESIAN_POINT('Ctrl Pts',(4.34802179419235,-1.4,16.2));
#140088=CARTESIAN_POINT('Ctrl Pts',(3.79039035625937,-0.999999999999999,
15.3785340219609));
#140089=CARTESIAN_POINT('Ctrl Pts',(3.67305500089253,-0.999999999999999,
15.673973906285));
#140090=CARTESIAN_POINT('Ctrl Pts',(3.8515947669147,-0.999999999999999,
15.9369869531425));
#140091=CARTESIAN_POINT('Ctrl Pts',(4.03013453293687,-0.999999999999999,
16.2));
#140092=CARTESIAN_POINT('Ctrl Pts',(4.34802179419235,-0.999999999999999,
16.2));
#140093=CARTESIAN_POINT('Ctrl Pts',(4.16214464821469,-1.,15.5261780073203));
#140094=CARTESIAN_POINT('Ctrl Pts',(4.12303286309241,-1.,15.6246579687617));
#140095=CARTESIAN_POINT('Ctrl Pts',(4.18254611843313,-1.,15.7123289843808));
#140096=CARTESIAN_POINT('Ctrl Pts',(4.24205937377385,-1.,15.8));
#140097=CARTESIAN_POINT('Ctrl Pts',(4.34802179419235,-1.,15.8));
#140098=CARTESIAN_POINT('Origin',(4.34802179419235,-1.4,15.6));
#140099=CARTESIAN_POINT('Origin',(4.34802179419235,-1.,15.6));
#140100=CARTESIAN_POINT('Origin',(4.9253475233554,-10.3,13.7931722204514));
#140101=CARTESIAN_POINT('',(4.34261496676317,-10.3,13.6502639719579));
#140102=CARTESIAN_POINT('',(4.34261496676317,-10.3,13.6502639719579));
#140103=CARTESIAN_POINT('',(5.23601216287606,-10.3,13.279861903244));
#140104=CARTESIAN_POINT('Origin',(4.9253475233554,-10.3,13.7931722204514));
#140105=CARTESIAN_POINT('',(5.23601216287606,-10.3,13.279861903244));
#140106=CARTESIAN_POINT('Origin',(-8.47750127826606,-10.3,10.5062825051013));
#140107=CARTESIAN_POINT('',(3.79039035625937,-10.3,15.3785340219609));
#140108=CARTESIAN_POINT('',(3.79039035625937,-10.3,15.3785340219609));
#140109=CARTESIAN_POINT('Origin',(-8.47750127826606,-10.3,10.5062825051013));
#140110=CARTESIAN_POINT('Origin',(4.34802179419235,-10.3,15.6));
#140111=CARTESIAN_POINT('',(4.34802179419235,-10.3,16.2));
#140112=CARTESIAN_POINT('',(4.34802179419235,-10.3,16.2));
#140113=CARTESIAN_POINT('Origin',(4.34802179419235,-10.3,15.6));
#140114=CARTESIAN_POINT('Origin',(3.87327121127015,-10.3,16.2));
#140115=CARTESIAN_POINT('',(9.34289321881345,-10.3,16.2));
#140116=CARTESIAN_POINT('',(9.34289321881345,-10.3,16.2));
#140117=CARTESIAN_POINT('',(1.93663560562379,-10.3,16.2));
#140118=CARTESIAN_POINT('Origin',(6.9080822150418,-1.,14.3043050016214));
#140119=CARTESIAN_POINT('Ctrl Pts',(-6.55757245707085,-7.39135402382937,
-5.14568636426237));
#140120=CARTESIAN_POINT('Ctrl Pts',(-6.75982089367161,-7.08279689100774,
-4.90112778377594));
#140121=CARTESIAN_POINT('Ctrl Pts',(-7.14201290222532,-6.4731824979059,
-4.38535750463086));
#140122=CARTESIAN_POINT('Ctrl Pts',(-7.56887561359513,-5.75729102255351,
-3.6687283197766));
#140123=CARTESIAN_POINT('Ctrl Pts',(-7.8920474790012,-5.32284996799027,
-3.00366070100896));
#140124=CARTESIAN_POINT('Ctrl Pts',(-8.06413796370095,-5.26314068500446,
-2.52167799537569));
#140125=CARTESIAN_POINT('Ctrl Pts',(-8.15634056422202,-5.39508785844239,
-2.13936273187432));
#140126=CARTESIAN_POINT('Ctrl Pts',(-8.19249518591845,-5.49079764276997,
-1.95623948829439));
#140127=CARTESIAN_POINT('Ctrl Pts',(-8.20848794733666,-5.54462134203543,
-1.86605338286933));
#140128=CARTESIAN_POINT('Ctrl Pts',(-6.59430671722206,-7.38479153604685,
-5.18370054092997));
#140129=CARTESIAN_POINT('Ctrl Pts',(-6.79566621980483,-7.07478422459138,
-4.93751456041579));
#140130=CARTESIAN_POINT('Ctrl Pts',(-7.17539501607384,-6.46212556707381,
-4.41814889099274));
#140131=CARTESIAN_POINT('Ctrl Pts',(-7.59517884839189,-5.74110238786913,
-3.69584015502338));
#140132=CARTESIAN_POINT('Ctrl Pts',(-7.91048502875434,-5.30205110155698,
-3.01914042655875));
#140133=CARTESIAN_POINT('Ctrl Pts',(-8.0839783182176,-5.24156135558239,
-2.52556156479809));
#140134=CARTESIAN_POINT('Ctrl Pts',(-8.18241342906123,-5.37510035618311,
-2.13771736365271));
#140135=CARTESIAN_POINT('Ctrl Pts',(-8.22157653308709,-5.47181651588286,
-1.95300235825357));
#140136=CARTESIAN_POINT('Ctrl Pts',(-8.2390509222775,-5.52617607587092,
-1.86220817076219));
#140137=CARTESIAN_POINT('Ctrl Pts',(-6.63595837298398,-7.34560921902525,
-5.26646136899686));
#140138=CARTESIAN_POINT('Ctrl Pts',(-6.83696744747848,-7.03490859729009,
-5.01596598714684));
#140139=CARTESIAN_POINT('Ctrl Pts',(-7.2145648216538,-6.4206676920658,-4.48700804201576));
#140140=CARTESIAN_POINT('Ctrl Pts',(-7.62626818611773,-5.69746584040132,
-3.74806941119204));
#140141=CARTESIAN_POINT('Ctrl Pts',(-7.93365762652132,-5.25679153997054,
-3.04563128053137));
#140142=CARTESIAN_POINT('Ctrl Pts',(-8.11137309037109,-5.19604966097288,
-2.52942016455644));
#140143=CARTESIAN_POINT('Ctrl Pts',(-8.21991249163311,-5.33007531761683,
-2.12876153722579));
#140144=CARTESIAN_POINT('Ctrl Pts',(-8.26402480718159,-5.42712564949736,
-1.93944532704854));
#140145=CARTESIAN_POINT('Ctrl Pts',(-8.28394949950606,-5.48167291123861,
-1.84665693304245));
#140146=CARTESIAN_POINT('Ctrl Pts',(-6.61728073072348,-7.27860819075006,
-5.33501354889539));
#140147=CARTESIAN_POINT('Ctrl Pts',(-6.82106903448059,-6.96941256165192,
-5.08222060797199));
#140148=CARTESIAN_POINT('Ctrl Pts',(-7.20417049462418,-6.35841500575385,
-4.54716168525424));
#140149=CARTESIAN_POINT('Ctrl Pts',(-7.62219974155008,-5.64034159634881,
-3.79386037188604));
#140150=CARTESIAN_POINT('Ctrl Pts',(-7.93630514231034,-5.20403706084519,
-3.06676953823316));
#140151=CARTESIAN_POINT('Ctrl Pts',(-8.12120138882497,-5.1440183658169,
-2.52725608769133));
#140152=CARTESIAN_POINT('Ctrl Pts',(-8.23556860403889,-5.27658630428028,
-2.11084110731329));
#140153=CARTESIAN_POINT('Ctrl Pts',(-8.2820116585493,-5.37269616280061,
-1.91519718281657));
#140154=CARTESIAN_POINT('Ctrl Pts',(-8.30297761570752,-5.42673591685656,
-1.81954222176521));
#140155=CARTESIAN_POINT('Ctrl Pts',(-6.59975017030691,-7.24993266759206,
-5.35661252001056));
#140156=CARTESIAN_POINT('Ctrl Pts',(-6.8050244734344,-6.94137553477043,
-5.10369911401669));
#140157=CARTESIAN_POINT('Ctrl Pts',(-7.19130954300827,-6.33176114166859,
-4.56771477257368));
#140158=CARTESIAN_POINT('Ctrl Pts',(-7.61421928816731,-5.6158696663162,
-3.8104955293341));
#140159=CARTESIAN_POINT('Ctrl Pts',(-7.93365040706529,-5.18142861175297,
-3.0744143426353));
#140160=CARTESIAN_POINT('Ctrl Pts',(-8.12203784210238,-5.12171932876715,
-2.52526953516964));
#140161=CARTESIAN_POINT('Ctrl Pts',(-8.23787448960478,-5.25366650220508,
-2.10202721872779));
#140162=CARTESIAN_POINT('Ctrl Pts',(-8.28468233453968,-5.34937628653266,
-1.90364658626372));
#140163=CARTESIAN_POINT('Ctrl Pts',(-8.30575868734589,-5.40319998579812,
-1.80675748997431));
#140164=CARTESIAN_POINT('',(-6.73177848765117,-7.12225772049266,-4.9282600804168));
#140165=CARTESIAN_POINT('',(-6.59975017049921,-7.24993266730301,-5.35661251977363));
#140166=CARTESIAN_POINT('Ctrl Pts',(-6.73176791483545,-7.12238125060388,
-4.92820584999411));
#140167=CARTESIAN_POINT('Ctrl Pts',(-6.73291165817144,-7.12938693500352,
-4.94184209885323));
#140168=CARTESIAN_POINT('Ctrl Pts',(-6.73358004363714,-7.13594979039427,
-4.95571899778471));
#140169=CARTESIAN_POINT('Ctrl Pts',(-6.73375401539604,-7.14213917334584,
-4.96978923814906));
#140170=CARTESIAN_POINT('Ctrl Pts',(-6.73399096594941,-7.1505691491342,
-4.98895298783715));
#140171=CARTESIAN_POINT('Ctrl Pts',(-6.7333094802454,-7.15824588042621,
-5.00833307284922));
#140172=CARTESIAN_POINT('Ctrl Pts',(-6.73168615754098,-7.16532994738964,
-5.02780762926736));
#140173=CARTESIAN_POINT('Ctrl Pts',(-6.72999471031469,-7.17271130501096,
-5.04809945685464));
#140174=CARTESIAN_POINT('Ctrl Pts',(-6.72728147209107,-7.17944881713203,
-5.06849489905558));
#140175=CARTESIAN_POINT('Ctrl Pts',(-6.72349592319277,-7.18568153871056,
-5.08888655201071));
#140176=CARTESIAN_POINT('Ctrl Pts',(-6.7196452262645,-7.19202152334213,
-5.10962913849061));
#140177=CARTESIAN_POINT('Ctrl Pts',(-6.71468577087202,-7.19783862981343,
-5.1303691323216));
#140178=CARTESIAN_POINT('Ctrl Pts',(-6.70852834943669,-7.20324367517375,
-5.15100588876705));
#140179=CARTESIAN_POINT('Ctrl Pts',(-6.70717535709377,-7.20443134521752,
-5.1555404774332));
#140180=CARTESIAN_POINT('Ctrl Pts',(-6.70576436140481,-7.20559900428378,
-5.16007008359584));
#140181=CARTESIAN_POINT('Ctrl Pts',(-6.70429412847365,-7.20674764453472,
-5.16459361682719));
#140182=CARTESIAN_POINT('Ctrl Pts',(-6.70322323205129,-7.20758429749579,
-5.16788849306837));
#140183=CARTESIAN_POINT('Ctrl Pts',(-6.70212287726058,-7.2084093020696,
-5.17117411068902));
#140184=CARTESIAN_POINT('Ctrl Pts',(-6.70099292278369,-7.2092231196394,
-5.17444999841023));
#140185=CARTESIAN_POINT('Ctrl Pts',(-6.69378551829264,-7.21441404770547,
-5.19534521884339));
#140186=CARTESIAN_POINT('Ctrl Pts',(-6.68537758112975,-7.21915261740078,
-5.21584416659399));
#140187=CARTESIAN_POINT('Ctrl Pts',(-6.67585574084893,-7.22361502853928,
-5.23585192639533));
#140188=CARTESIAN_POINT('Ctrl Pts',(-6.66582683814292,-7.22831507452013,
-5.25692515074012));
#140189=CARTESIAN_POINT('Ctrl Pts',(-6.65456230470562,-7.2327077631601,
-5.27745486626376));
#140190=CARTESIAN_POINT('Ctrl Pts',(-6.64211215477387,-7.23696957402667,
-5.29732416150095));
#140191=CARTESIAN_POINT('Ctrl Pts',(-6.62966200484213,-7.24123138489323,
-5.31719345673814));
#140192=CARTESIAN_POINT('Ctrl Pts',(-6.61602588604064,-7.24536099521506,
-5.33640382478608));
#140193=CARTESIAN_POINT('Ctrl Pts',(-6.60120676753226,-7.2495243906536,
-5.3548105998295));
#140194=CARTESIAN_POINT('Ctrl Pts',(-6.6007224198111,-7.2496604669723,-5.35541220643256));
#140195=CARTESIAN_POINT('Ctrl Pts',(-6.60023688716911,-7.24979655733683,
-5.35601284816904));
#140196=CARTESIAN_POINT('Ctrl Pts',(-6.59975017030691,-7.24993266759206,
-5.35661252001056));
#140197=CARTESIAN_POINT('',(-8.30575868734442,-5.40319998579812,-1.80675748998109));
#140198=CARTESIAN_POINT('Ctrl Pts',(-6.59975017030691,-7.24993266759206,
-5.35661252001056));
#140199=CARTESIAN_POINT('Ctrl Pts',(-6.8050244734344,-6.94137553477043,
-5.10369911401669));
#140200=CARTESIAN_POINT('Ctrl Pts',(-7.19130954300827,-6.33176114166859,
-4.56771477257368));
#140201=CARTESIAN_POINT('Ctrl Pts',(-7.61421928816731,-5.6158696663162,
-3.8104955293341));
#140202=CARTESIAN_POINT('Ctrl Pts',(-7.93365040706529,-5.18142861175297,
-3.0744143426353));
#140203=CARTESIAN_POINT('Ctrl Pts',(-8.12203784210238,-5.12171932876715,
-2.52526953516964));
#140204=CARTESIAN_POINT('Ctrl Pts',(-8.23787448960478,-5.25366650220508,
-2.10202721872779));
#140205=CARTESIAN_POINT('Ctrl Pts',(-8.28468233453968,-5.34937628653266,
-1.90364658626372));
#140206=CARTESIAN_POINT('Ctrl Pts',(-8.30575868734589,-5.40319998579812,
-1.80675748997431));
#140207=CARTESIAN_POINT('',(-8.20848794733666,-5.54462134203543,-1.86605338286933));
#140208=CARTESIAN_POINT('Origin',(-8.11032907117305,-5.40319998579812,-1.76424554903373));
#140209=CARTESIAN_POINT('Ctrl Pts',(-8.20848794733666,-5.54462134203543,
-1.86605338286933));
#140210=CARTESIAN_POINT('Ctrl Pts',(-8.19249518591845,-5.49079764276997,
-1.95623948829439));
#140211=CARTESIAN_POINT('Ctrl Pts',(-8.15634056422202,-5.39508785844239,
-2.13936273187432));
#140212=CARTESIAN_POINT('Ctrl Pts',(-8.06413796370095,-5.26314068500446,
-2.52167799537569));
#140213=CARTESIAN_POINT('Ctrl Pts',(-7.8920474790012,-5.32284996799027,
-3.00366070100896));
#140214=CARTESIAN_POINT('Ctrl Pts',(-7.56887561359513,-5.75729102255351,
-3.6687283197766));
#140215=CARTESIAN_POINT('Ctrl Pts',(-7.19183563386273,-6.38962479209568,
-4.30171369454974));
#140216=CARTESIAN_POINT('Ctrl Pts',(-6.87047660210866,-6.90569934085639,
-4.74940342070924));
#140217=CARTESIAN_POINT('Ctrl Pts',(-6.73179386229792,-7.12234071719252,
-4.92817240258013));
#140218=CARTESIAN_POINT('Ctrl Pts',(-8.20848794733648,-5.54462134203483,
-1.86605338287034));
#140219=CARTESIAN_POINT('Ctrl Pts',(-8.22570432892313,-5.60256313961292,
-1.76896705962691));
#140220=CARTESIAN_POINT('Ctrl Pts',(-8.30203822855091,-5.67885398422639,
-1.60363731207959));
#140221=CARTESIAN_POINT('Ctrl Pts',(-8.51961092920762,-5.69711542803795,
-1.45079338011714));
#140222=CARTESIAN_POINT('Ctrl Pts',(-8.66564229791336,-5.66327831149784,
-1.42362085501337));
#140223=CARTESIAN_POINT('Ctrl Pts',(-8.73598097951737,-5.63790797511633,
-1.42417566375139));
#140224=CARTESIAN_POINT('Ctrl Pts',(-8.26197315348204,-5.51234212624656,
-1.85932426168421));
#140225=CARTESIAN_POINT('Ctrl Pts',(-8.27437032427531,-5.56818098336045,
-1.77251643685663));
#140226=CARTESIAN_POINT('Ctrl Pts',(-8.3392891469759,-5.642057191414,-1.62376201038179));
#140227=CARTESIAN_POINT('Ctrl Pts',(-8.5321969224146,-5.65975617308337,
-1.4872628671831));
#140228=CARTESIAN_POINT('Ctrl Pts',(-8.66236637734033,-5.62701114347325,
-1.46459597020112));
#140229=CARTESIAN_POINT('Ctrl Pts',(-8.7247932961205,-5.6024788095447,-1.46627251165308));
#140230=CARTESIAN_POINT('Ctrl Pts',(-8.29926952018809,-5.45811715826701,
-1.8365885308239));
#140231=CARTESIAN_POINT('Ctrl Pts',(-8.31007945872644,-5.51489858344653,
-1.76137839707867));
#140232=CARTESIAN_POINT('Ctrl Pts',(-8.36725749645066,-5.58989957876681,
-1.63099116012873));
#140233=CARTESIAN_POINT('Ctrl Pts',(-8.53788390290437,-5.60786132493498,
-1.51041285785609));
#140234=CARTESIAN_POINT('Ctrl Pts',(-8.65267646235137,-5.57461521980001,
-1.49020536934065));
#140235=CARTESIAN_POINT('Ctrl Pts',(-8.70746447552891,-5.54969839474843,
-1.49152721040301));
#140236=CARTESIAN_POINT('Ctrl Pts',(-8.30575868734471,-5.40319998579752,
-1.80675748997975));
#140237=CARTESIAN_POINT('Ctrl Pts',(-8.32052873133615,-5.46114178337561,
-1.73885882518281));
#140238=CARTESIAN_POINT('Ctrl Pts',(-8.37815380678821,-5.53743262798908,
-1.62294165666584));
#140239=CARTESIAN_POINT('Ctrl Pts',(-8.53500933031641,-5.55569407180065,
-1.5139172416936));
#140240=CARTESIAN_POINT('Ctrl Pts',(-8.63932760832842,-5.52185695526053,
-1.49273142435505));
#140241=CARTESIAN_POINT('Ctrl Pts',(-8.6895496409325,-5.49648661887902,
-1.49184382745125));
#140242=CARTESIAN_POINT('',(-8.73598097951737,-5.63790797511633,-1.42417566375139));
#140243=CARTESIAN_POINT('Origin',(-8.68601550155451,-5.49648661887902,-1.29187505524205));
#140244=CARTESIAN_POINT('Ctrl Pts',(-8.73598097951737,-5.63790797511633,
-1.42417566375139));
#140245=CARTESIAN_POINT('Ctrl Pts',(-8.66564229791336,-5.66327831149784,
-1.42362085501337));
#140246=CARTESIAN_POINT('Ctrl Pts',(-8.51961092920762,-5.69711542803795,
-1.45079338011714));
#140247=CARTESIAN_POINT('Ctrl Pts',(-8.30203822855091,-5.67885398422639,
-1.60363731207959));
#140248=CARTESIAN_POINT('Ctrl Pts',(-8.22570432892313,-5.60256313961292,
-1.76896705962691));
#140249=CARTESIAN_POINT('Ctrl Pts',(-8.20848794733648,-5.54462134203483,
-1.86605338287034));
#140250=CARTESIAN_POINT('Ctrl Pts',(-8.30575868734471,-5.40319998579752,
-1.80675748997975));
#140251=CARTESIAN_POINT('Ctrl Pts',(-8.32052873133615,-5.46114178337561,
-1.73885882518281));
#140252=CARTESIAN_POINT('Ctrl Pts',(-8.37815380678821,-5.53743262798908,
-1.62294165666584));
#140253=CARTESIAN_POINT('Ctrl Pts',(-8.53500933031641,-5.55569407180065,
-1.5139172416936));
#140254=CARTESIAN_POINT('Ctrl Pts',(-8.63932760832842,-5.52185695526053,
-1.49273142435505));
#140255=CARTESIAN_POINT('Ctrl Pts',(-8.6895496409325,-5.49648661887902,
-1.49184382745125));
#140256=CARTESIAN_POINT('Ctrl Pts',(-8.73598097951772,-5.63790797511621,
-1.42417566375139));
#140257=CARTESIAN_POINT('Ctrl Pts',(-8.90608013788385,-5.5765552063756,
-1.42551735081822));
#140258=CARTESIAN_POINT('Ctrl Pts',(-9.2607737387321,-5.50597871763856,
-1.41691940563236));
#140259=CARTESIAN_POINT('Ctrl Pts',(-9.78761036667993,-5.6224253396905,
-1.35940353299553));
#140260=CARTESIAN_POINT('Ctrl Pts',(-10.7490450394837,-6.15724901285239,
-1.19114732392076));
#140261=CARTESIAN_POINT('Ctrl Pts',(-11.4346764894942,-6.81457717411039,
-1.0024272195599));
#140262=CARTESIAN_POINT('Ctrl Pts',(-11.9675786126161,-7.33643304648348,
-0.82348831362286));
#140263=CARTESIAN_POINT('Ctrl Pts',(-8.72958801757661,-5.61766273764671,
-1.4482310054095));
#140264=CARTESIAN_POINT('Ctrl Pts',(-8.90186687848093,-5.55573534105649,
-1.4479368219087));
#140265=CARTESIAN_POINT('Ctrl Pts',(-9.26239084548173,-5.48442219169093,
-1.43692373533481));
#140266=CARTESIAN_POINT('Ctrl Pts',(-9.79819135996713,-5.60204483004328,
-1.38216037519801));
#140267=CARTESIAN_POINT('Ctrl Pts',(-10.7695899593085,-6.14160038605648,
-1.2249245242093));
#140268=CARTESIAN_POINT('Ctrl Pts',(-11.4562523641124,-6.80244679525222,
-1.04191725589513));
#140269=CARTESIAN_POINT('Ctrl Pts',(-11.9907277518307,-7.32656702812379,
-0.865930760169916));
#140270=CARTESIAN_POINT('Ctrl Pts',(-8.71496589733162,-5.57251604392361,
-1.48117231511046));
#140271=CARTESIAN_POINT('Ctrl Pts',(-8.89218445918492,-5.51039924206827,
-1.47848223790221));
#140272=CARTESIAN_POINT('Ctrl Pts',(-9.26474568365955,-5.43887548480292,
-1.46396685256936));
#140273=CARTESIAN_POINT('Ctrl Pts',(-9.81889517320176,-5.55689222737881,
-1.41257201003397));
#140274=CARTESIAN_POINT('Ctrl Pts',(-10.8151018059367,-6.09806657044163,
-1.27028840934711));
#140275=CARTESIAN_POINT('Ctrl Pts',(-11.5087297589057,-6.76059811347898,
-1.09631471034077));
#140276=CARTESIAN_POINT('Ctrl Pts',(-12.0490661719394,-7.28572395405559,
-0.924516784598555));
#140277=CARTESIAN_POINT('Ctrl Pts',(-8.69722742718828,-5.51929166568008,
-1.49170813443058));
#140278=CARTESIAN_POINT('Ctrl Pts',(-8.88012225811069,-5.45771058941653,
-1.4883556607762));
#140279=CARTESIAN_POINT('Ctrl Pts',(-9.26595248827283,-5.38685152183972,
-1.47253893791997));
#140280=CARTESIAN_POINT('Ctrl Pts',(-9.83983744636612,-5.50376842165011,
-1.42058142214234));
#140281=CARTESIAN_POINT('Ctrl Pts',(-10.8642279877717,-6.04048923813472,
-1.27865017845492));
#140282=CARTESIAN_POINT('Ctrl Pts',(-11.5663403083829,-6.69937482262425,
-1.10351864069462));
#140283=CARTESIAN_POINT('Ctrl Pts',(-12.1123767090216,-7.22220505445906,
-0.929989202773578));
#140284=CARTESIAN_POINT('Ctrl Pts',(-8.68954964093266,-5.4964866188789,
-1.49184382745125));
#140285=CARTESIAN_POINT('Ctrl Pts',(-8.87481436092436,-5.43513385013829,
-1.4885695594993));
#140286=CARTESIAN_POINT('Ctrl Pts',(-9.26624052344372,-5.36455736140126,
-1.47266896725833));
#140287=CARTESIAN_POINT('Ctrl Pts',(-9.8483467388184,-5.48100398345319,
-1.41973709154106));
#140288=CARTESIAN_POINT('Ctrl Pts',(-10.8839646004455,-6.01582765661507,
-1.27510485735236));
#140289=CARTESIAN_POINT('Ctrl Pts',(-11.5886799961236,-6.67315581787308,
-1.09764645444795));
#140290=CARTESIAN_POINT('Ctrl Pts',(-12.1362808769477,-7.19501169024617,
-0.922336477447363));
#140291=CARTESIAN_POINT('',(-11.720329716163,-7.09759078643408,-0.903811780387333));
#140292=CARTESIAN_POINT('Ctrl Pts',(-12.1362808769477,-7.19501169024617,
-0.922336477447363));
#140293=CARTESIAN_POINT('Ctrl Pts',(-12.1356058178704,-7.1949090851414,
-0.92255259213136));
#140294=CARTESIAN_POINT('Ctrl Pts',(-12.1349303707403,-7.19480649116483,
-0.92276748566852));
#140295=CARTESIAN_POINT('Ctrl Pts',(-12.1342545392746,-7.19470390378757,
-0.922981158839793));
#140296=CARTESIAN_POINT('Ctrl Pts',(-12.1124520082791,-7.19139440343733,
-0.929874321079293));
#140297=CARTESIAN_POINT('Ctrl Pts',(-12.0903590888155,-7.18810662017071,
-0.935467523380962));
#140298=CARTESIAN_POINT('Ctrl Pts',(-12.0680949384848,-7.18469061225302,
-0.939801108152501));
#140299=CARTESIAN_POINT('Ctrl Pts',(-12.0461316693408,-7.18132076879709,
-0.944076128186122));
#140300=CARTESIAN_POINT('Ctrl Pts',(-12.0240005435959,-7.17782726878866,
-0.947125084551186));
#140301=CARTESIAN_POINT('Ctrl Pts',(-12.0018081000388,-7.17405656013424,
-0.948939718809822));
#140302=CARTESIAN_POINT('Ctrl Pts',(-11.9835242742012,-7.17094996305561,
-0.950434752768501));
#140303=CARTESIAN_POINT('Ctrl Pts',(-11.9651983957458,-7.16765532782976,
-0.951091096725075));
#140304=CARTESIAN_POINT('Ctrl Pts',(-11.9468945090915,-7.16407368887123,
-0.950881242320794));
#140305=CARTESIAN_POINT('Ctrl Pts',(-11.9365164786444,-7.16204295305734,
-0.950762258006794));
#140306=CARTESIAN_POINT('Ctrl Pts',(-11.9261456459944,-7.15991966508634,
-0.950364375632169));
#140307=CARTESIAN_POINT('Ctrl Pts',(-11.9157926875919,-7.15769064124147,
-0.949694791663599));
#140308=CARTESIAN_POINT('Ctrl Pts',(-11.8946462833602,-7.15313775525154,
-0.948327134930536));
#140309=CARTESIAN_POINT('Ctrl Pts',(-11.8738130426135,-7.14819787356317,
-0.945844033494343));
#140310=CARTESIAN_POINT('Ctrl Pts',(-11.8533514464485,-7.14276269857209,
-0.942352303314894));
#140311=CARTESIAN_POINT('Ctrl Pts',(-11.8333562318705,-7.13745140763763,
-0.938940160214053));
#140312=CARTESIAN_POINT('Ctrl Pts',(-11.8137150547943,-7.1316677042646,
-0.93456377027132));
#140313=CARTESIAN_POINT('Ctrl Pts',(-11.7945026420297,-7.12527752047938,
-0.929293324324193));
#140314=CARTESIAN_POINT('Ctrl Pts',(-11.7764881809649,-7.11928578386585,
-0.924351506527949));
#140315=CARTESIAN_POINT('Ctrl Pts',(-11.7588502247179,-7.11276106497496,
-0.918622782484977));
#140316=CARTESIAN_POINT('Ctrl Pts',(-11.7416771845018,-7.1055583986353,
-0.912152583906187));
#140317=CARTESIAN_POINT('Ctrl Pts',(-11.7346823377481,-7.10262464045215,
-0.909517171250373));
#140318=CARTESIAN_POINT('Ctrl Pts',(-11.7277649828676,-7.09957797351498,
-0.906758662971134));
#140319=CARTESIAN_POINT('Ctrl Pts',(-11.7209327506114,-7.09640666702022,
-0.903879959984334));
#140320=CARTESIAN_POINT('Ctrl Pts',(-11.7212088289358,-7.09667288316797,
-0.903792747022583));
#140321=CARTESIAN_POINT('Ctrl Pts',(-11.2647820308748,-6.65654480564138,
-1.04798290473443));
#140322=CARTESIAN_POINT('Ctrl Pts',(-10.6507952163715,-6.10259492893934,
-1.20834156836267));
#140323=CARTESIAN_POINT('Ctrl Pts',(-9.78761036667993,-5.6224253396905,
-1.35940353299553));
#140324=CARTESIAN_POINT('Ctrl Pts',(-9.2607737387321,-5.50597871763856,
-1.41691940563236));
#140325=CARTESIAN_POINT('Ctrl Pts',(-8.90608013788385,-5.5765552063756,
-1.42551735081822));
#140326=CARTESIAN_POINT('Ctrl Pts',(-8.73598097951772,-5.63790797511621,
-1.42417566375139));
#140327=CARTESIAN_POINT('Origin',(-8.69661791968849,4.20059847321333E-16,
-1.89178137186966));
#140328=CARTESIAN_POINT('',(-8.30575868734294,-2.6,-1.80675748998788));
#140329=CARTESIAN_POINT('',(-8.30575868734294,4.011807530597E-16,-1.80675748998788));
#140330=CARTESIAN_POINT('Origin',(-8.69661791968849,-2.6,-1.89178137186966));
#140331=CARTESIAN_POINT('Origin',(0.,0.,0.));
#140332=CARTESIAN_POINT('',(-6.59975017030735,-10.1,-5.35661252001003));
#140333=CARTESIAN_POINT('',(-6.59975017030735,-10.3,-5.35661252001003));
#140334=CARTESIAN_POINT('',(0.00347333261335205,-10.1,-8.49999929035314));
#140335=CARTESIAN_POINT('Origin',(0.,-10.1,-2.24265050974282E-15));
#140336=CARTESIAN_POINT('',(0.00347333261332719,-7.5,-8.49999929035059));
#140337=CARTESIAN_POINT('',(0.00347333261332719,1.88737898428894E-15,-8.49999929035059));
#140338=CARTESIAN_POINT('',(5.63796910874814,-7.5,-6.36107729310073));
#140339=CARTESIAN_POINT('Origin',(0.,-7.5,-1.66533453693773E-15));
#140340=CARTESIAN_POINT('',(6.27943617390152,-6.6,-5.72875914469243));
#140341=CARTESIAN_POINT('Ctrl Pts',(5.63796910874819,-7.49999999999993,
-6.36107729310069));
#140342=CARTESIAN_POINT('Ctrl Pts',(5.67409984605671,-7.45172701336858,
-6.32905378962232));
#140343=CARTESIAN_POINT('Ctrl Pts',(5.70986959776522,-7.40356504020207,
-6.29680055298516));
#140344=CARTESIAN_POINT('Ctrl Pts',(5.92847216942438,-7.10694555119756,
-6.09631105969112));
#140345=CARTESIAN_POINT('Ctrl Pts',(6.10772709056793,-6.85356360695371,
-5.9169737653527));
#140346=CARTESIAN_POINT('Ctrl Pts',(6.27943617390152,-6.6,-5.72875914469242));
#140347=CARTESIAN_POINT('',(8.44432226295358,-6.6,0.971298882623956));
#140348=CARTESIAN_POINT('Origin',(-7.2099444470286E-17,-6.6,-1.49003062450498E-15));
#140349=CARTESIAN_POINT('',(8.28947420569055,-7.5,1.88005781644903));
#140350=CARTESIAN_POINT('Ctrl Pts',(8.28947420569055,-7.5,1.88005781644903));
#140351=CARTESIAN_POINT('Ctrl Pts',(8.29772790894898,-7.46315114007885,
1.84366592484676));
#140352=CARTESIAN_POINT('Ctrl Pts',(8.30574546103206,-7.42632827323882,
1.8072042671372));
#140353=CARTESIAN_POINT('Ctrl Pts',(8.31352574751022,-7.3895345357671,1.77067491242312));
#140354=CARTESIAN_POINT('Ctrl Pts',(8.36906359788408,-7.12689059686646,
1.5099182112324));
#140355=CARTESIAN_POINT('Ctrl Pts',(8.41310047956988,-6.86272854589131,
1.24273623855277));
#140356=CARTESIAN_POINT('Ctrl Pts',(8.44432226295358,-6.6,0.971298882623954));
#140357=CARTESIAN_POINT('',(5.03883335853763,-7.5,6.8454480046881));
#140358=CARTESIAN_POINT('Origin',(0.,-7.5,-1.66533453693773E-15));
#140359=CARTESIAN_POINT('',(5.03883335853763,-10.3,6.8454480046881));
#140360=CARTESIAN_POINT('',(5.03883335853763,-4.81067232832666E-17,6.84544800468811));
#140361=CARTESIAN_POINT('',(5.03722331003166,-10.3,6.84663284577709));
#140362=CARTESIAN_POINT('Origin',(-7.2099444470286E-17,-10.3,-2.28766658394441E-15));
#140363=CARTESIAN_POINT('',(5.03722331003166,-2.6,6.84663284577709));
#140364=CARTESIAN_POINT('',(5.03722331003166,-2.6,6.84663284577709));
#140365=CARTESIAN_POINT('',(-8.5,-2.6,-1.61826575208033E-15));
#140366=CARTESIAN_POINT('Origin',(0.,-2.6,-5.77315972805081E-16));
#140367=CARTESIAN_POINT('',(-8.5,2.31137282485971E-31,-1.04094977927525E-15));
#140368=CARTESIAN_POINT('',(-8.5,2.31137282485971E-31,-1.04094977927525E-15));
#140369=CARTESIAN_POINT('Origin',(0.,0.,0.));
#140370=CARTESIAN_POINT('Origin',(0.,-2.6,-5.77315972805081E-16));
#140371=CARTESIAN_POINT('Origin',(-9.35,-6.25,-3.05000000003699));
#140372=CARTESIAN_POINT('Ctrl Pts',(-11.5368071934914,-7.05,-0.782760643794657));
#140373=CARTESIAN_POINT('Ctrl Pts',(-11.5844488890167,-7.05,-0.828712211368656));
#140374=CARTESIAN_POINT('Ctrl Pts',(-11.6417386809522,-7.06395036419954,
-0.867768806826326));
#140375=CARTESIAN_POINT('Ctrl Pts',(-11.7073160840573,-7.09173525292199,
-0.898191855681428));
#140376=CARTESIAN_POINT('Ctrl Pts',(-11.71381758951,-7.09460545954183,-0.901067364263082));
#140377=CARTESIAN_POINT('Ctrl Pts',(-11.720329716163,-7.09759078643408,
-0.903811780387334));
#140378=CARTESIAN_POINT('Ctrl Pts',(-6.73177848765117,-7.12225772049266,
-4.9282600804168));
#140379=CARTESIAN_POINT('Ctrl Pts',(-6.72976354048857,-7.10991695334985,
-4.90428006259042));
#140380=CARTESIAN_POINT('Ctrl Pts',(-6.72623571781636,-7.09867178972273,
-4.87972758418512));
#140381=CARTESIAN_POINT('Ctrl Pts',(-6.7076526749211,-7.06395036419954,
-4.79132127310591));
#140382=CARTESIAN_POINT('Ctrl Pts',(-6.68250369548387,-7.05,-4.72670651672613));
#140383=CARTESIAN_POINT('Ctrl Pts',(-6.64846378001877,-7.05,-4.66993890386316));
#140384=CARTESIAN_POINT('Origin',(-16.1000000000146,-2.6,0.725816604289514));
#140385=CARTESIAN_POINT('',(-16.5000000000146,-10.1,0.725816604290266));
#140386=CARTESIAN_POINT('Origin',(-16.1000000000146,-10.1,0.725816604289513));
#140387=CARTESIAN_POINT('',(-16.5000000000146,-2.6,0.725816604290267));
#140388=CARTESIAN_POINT('Origin',(-16.1000000000146,-2.6,0.725816604289514));
#140389=CARTESIAN_POINT('',(-16.5000000000146,-2.6,0.725816604290267));
#140390=CARTESIAN_POINT('Origin',(-15.7415106627401,-10.1,-2.75165772610856));
#140391=CARTESIAN_POINT('',(-16.5000000000305,-10.1,-7.71862915012594));
#140392=CARTESIAN_POINT('',(-16.5000000000167,-10.1,-0.400828863065334));
#140393=CARTESIAN_POINT('',(-16.7343145750813,-10.1,-8.28431457507367));
#140394=CARTESIAN_POINT('Origin',(-17.3000000000305,-10.1,-7.71862915012444));
#140395=CARTESIAN_POINT('',(-17.8000000000336,-10.1,-9.35000000002598));
#140396=CARTESIAN_POINT('',(-15.7571789150852,-10.1,-7.30717891507761));
#140397=CARTESIAN_POINT('',(-16.6686291501351,-10.1,-10.4813708499245));
#140398=CARTESIAN_POINT('',(-17.8000000000336,-10.1,-9.35000000002598));
#140399=CARTESIAN_POINT('',(-15.1343145750825,-10.1,-8.94705627487187));
#140400=CARTESIAN_POINT('',(-15.691493490136,-10.1,-9.50423518992531));
#140401=CARTESIAN_POINT('Origin',(-15.7000000000318,-10.1,-8.38137084992263));
#140402=CARTESIAN_POINT('Origin',(-11.9533418970136,-10.1,-0.350905528319928));
#140403=CARTESIAN_POINT('Origin',(-16.5000000000123,-24.4,1.94999999997646));
#140404=CARTESIAN_POINT('',(-16.4999999999955,-2.6,10.8686291501049));
#140405=CARTESIAN_POINT('',(-16.4999999999949,-2.6,11.2000000000031));
#140406=CARTESIAN_POINT('',(-16.4999999999955,-3.44027676348872E-15,10.8686291501049));
#140407=CARTESIAN_POINT('',(-16.4999999999955,-24.4,10.8686291501049));
#140408=CARTESIAN_POINT('',(-16.5000000000305,6.86923662425558E-16,-7.71862915012594));
#140409=CARTESIAN_POINT('',(-16.5000000000059,-2.22044604925031E-15,5.37500000000578));
#140410=CARTESIAN_POINT('',(-16.5000000000305,-24.4,-7.71862915012594));
#140411=CARTESIAN_POINT('Origin',(11.2581254575403,-10.3,-18.3));
#140412=CARTESIAN_POINT('',(11.8728253843338,-10.3,-17.788));
#140413=CARTESIAN_POINT('',(11.2581254575403,-10.3,-19.1000000000102));
#140414=CARTESIAN_POINT('Origin',(11.2581254575403,-10.3,-18.3));
#140415=CARTESIAN_POINT('',(11.2581254575403,-7.5,-19.1));
#140416=CARTESIAN_POINT('',(11.2581254575403,-10.3,-19.1));
#140417=CARTESIAN_POINT('',(11.8728253843338,-7.5,-17.788));
#140418=CARTESIAN_POINT('Origin',(11.2581254575403,-7.5,-18.3));
#140419=CARTESIAN_POINT('',(11.8728253843338,-10.3,-17.788));
#140420=CARTESIAN_POINT('Origin',(-2.25730545366787E-11,-10.3,-0.450000000022575));
#140421=CARTESIAN_POINT('',(10.9,-10.3,-15.1));
#140422=CARTESIAN_POINT('Origin',(15.1,-10.3,-15.1));
#140423=CARTESIAN_POINT('',(10.9,-10.3,-13.800000000037));
#140424=CARTESIAN_POINT('',(10.9,-10.3,-11.6000000000162));
#140425=CARTESIAN_POINT('',(10.5,-10.3,-13.400000000037));
#140426=CARTESIAN_POINT('Origin',(10.5,-10.3,-13.800000000037));
#140427=CARTESIAN_POINT('',(5.24999999998871,-10.3,-13.400000000037));
#140428=CARTESIAN_POINT('',(-0.796199698700571,-10.3,-9.30032612545083));
#140429=CARTESIAN_POINT('Origin',(0.00380023450634744,-10.3,-9.29999922356006));
#140430=CARTESIAN_POINT('',(-0.79309436390975,-10.3,-16.899754823607));
#140431=CARTESIAN_POINT('',(-0.797984158749954,-10.3,-4.93336481758792));
#140432=CARTESIAN_POINT('',(-1.39309431381607,-10.3,-17.5000000000267));
#140433=CARTESIAN_POINT('Origin',(-1.39309431381685,-10.3,-16.9000000000267));
#140434=CARTESIAN_POINT('',(-11.9672956534841,-10.3,-17.5000000000405));
#140435=CARTESIAN_POINT('',(-0.39642454364202,-10.3,-17.5000000000254));
#140436=CARTESIAN_POINT('',(-12.5250910766189,-10.3,-16.6789473684552));
#140437=CARTESIAN_POINT('Origin',(-11.9672956534849,-10.3,-16.9000000000405));
#140438=CARTESIAN_POINT('Origin',(-15.5,-10.3,-15.5));
#140439=CARTESIAN_POINT('',(-13.9781746176887,-10.3,-12.419231543135));
#140440=CARTESIAN_POINT('Origin',(-9.35,-10.3,-3.05000000003699));
#140441=CARTESIAN_POINT('',(-14.5846229736965,-10.3,-12.1880260147795));
#140442=CARTESIAN_POINT('Origin',(-15.5,-10.3,-15.5));
#140443=CARTESIAN_POINT('',(-15.0612959521201,-10.3,-12.3302147141527));
#140444=CARTESIAN_POINT('Origin',(-14.9790389431426,-10.3,-11.7358799730564));
#140445=CARTESIAN_POINT('',(-16.4600000000227,-10.3,-12.4473945554729));
#140446=CARTESIAN_POINT('Origin',(-15.5,-10.3,-15.5));
#140447=CARTESIAN_POINT('',(-17.5000000000283,-10.3,-11.6842431943471));
#140448=CARTESIAN_POINT('Origin',(-16.7000000000283,-10.3,-11.6842431943411));
#140449=CARTESIAN_POINT('',(-17.5000000000286,-10.3,-11.6441125497224));
#140450=CARTESIAN_POINT('',(-17.5,-10.3,-15.4999999999881));
#140451=CARTESIAN_POINT('',(-17.2656854249779,-10.3,-11.0784271247672));
#140452=CARTESIAN_POINT('Origin',(-16.7000000000286,-10.3,-11.6441125497165));
#140453=CARTESIAN_POINT('',(-16.6686291501351,-10.3,-10.4813708499245));
#140454=CARTESIAN_POINT('',(-17.5000000000311,-10.3,-11.3127416998205));
#140455=CARTESIAN_POINT('',(-17.8000000000336,-10.3,-9.35000000002598));
#140456=CARTESIAN_POINT('',(-15.0093145750824,-10.3,-12.1406854249771));
#140457=CARTESIAN_POINT('',(-18.8656854249492,-10.3,-10.4156854249416));
#140458=CARTESIAN_POINT('',(-16.5000000000311,-10.3,-8.05000000002353));
#140459=CARTESIAN_POINT('',(-19.1,-10.3,-10.9813708498909));
#140460=CARTESIAN_POINT('Origin',(-18.3,-10.3,-10.9813708498909));
#140461=CARTESIAN_POINT('',(-19.1,-10.3,-15.5));
#140462=CARTESIAN_POINT('',(-19.1,-10.3,4.01764068713489));
#140463=CARTESIAN_POINT('',(-15.5,-10.3,-19.1000000000451));
#140464=CARTESIAN_POINT('Origin',(-15.5,-10.3,-15.5));
#140465=CARTESIAN_POINT('',(-15.5,-10.3,-19.1000000000451));
#140466=CARTESIAN_POINT('',(-17.1,-10.3,-15.5));
#140467=CARTESIAN_POINT('Origin',(-15.5,-10.3,-15.5));
#140468=CARTESIAN_POINT('Origin',(15.1,-10.3,-15.1));
#140469=CARTESIAN_POINT('',(10.9,-7.5,-15.1));
#140470=CARTESIAN_POINT('Origin',(15.1,-7.5,-15.1));
#140471=CARTESIAN_POINT('',(10.9,-10.3,-15.1));
#140472=CARTESIAN_POINT('Origin',(13.1,-7.5,-1.80000000000345));
#140473=CARTESIAN_POINT('',(15.1,-7.5,-19.1));
#140474=CARTESIAN_POINT('',(-1.2,-7.5,-19.1));
#140475=CARTESIAN_POINT('',(19.1,-7.5,-15.1));
#140476=CARTESIAN_POINT('Origin',(15.1,-7.5,-15.1));
#140477=CARTESIAN_POINT('',(19.1,-7.5,-10.9813708499319));
#140478=CARTESIAN_POINT('',(19.1,-7.5,-10.4500000000017));
#140479=CARTESIAN_POINT('',(18.8656854249492,-7.5,-10.4156854249827));
#140480=CARTESIAN_POINT('Origin',(18.3,-7.5,-10.9813708499319));
#140481=CARTESIAN_POINT('',(16.734314575042,-7.5,-8.28431457507544));
#140482=CARTESIAN_POINT('',(16.4999999999906,-7.5,-8.05000000002406));
#140483=CARTESIAN_POINT('',(16.4999999999912,-7.5,-7.7186291501247));
#140484=CARTESIAN_POINT('Origin',(17.2999999999912,-7.5,-7.71862915012621));
#140485=CARTESIAN_POINT('',(16.4999999999931,-7.5,-6.72119489704348));
#140486=CARTESIAN_POINT('',(16.5000000000094,-7.5,1.94999999997594));
#140487=CARTESIAN_POINT('',(11.3899837160979,-7.5,-7.45800064600289));
#140488=CARTESIAN_POINT('Origin',(15.1,-7.5,-15.1));
#140489=CARTESIAN_POINT('Origin',(9.25,-7.5,-3.05000000003699));
#140490=CARTESIAN_POINT('Origin',(0.00380023450634622,-7.5,-9.29999922356006));
#140491=CARTESIAN_POINT('',(1.32237339244619,-7.5,-9.60943957263028));
#140492=CARTESIAN_POINT('Origin',(1.4041696846368,-7.5,-10.2038378957974));
#140493=CARTESIAN_POINT('',(5.41419360512517,-7.5,-8.0483854216423));
#140494=CARTESIAN_POINT('Origin',(-5.6920614055489E-17,-7.5,-1.53860044684792E-15));
#140495=CARTESIAN_POINT('',(6.14689326954821,-7.5,-8.09705302340923));
#140496=CARTESIAN_POINT('Origin',(5.74909217812359,-7.5,-8.54622369438117));
#140497=CARTESIAN_POINT('',(7.33287671232876,-7.5,-8.80342937459372));
#140498=CARTESIAN_POINT('Origin',(8.6,-7.5,-5.32716721908225));
#140499=CARTESIAN_POINT('Origin',(6.1,-7.5,-12.1857384988752));
#140500=CARTESIAN_POINT('',(10.5,-7.5,-13.400000000037));
#140501=CARTESIAN_POINT('',(9.25,-7.5,-13.400000000037));
#140502=CARTESIAN_POINT('',(10.9,-7.5,-13.800000000037));
#140503=CARTESIAN_POINT('Origin',(10.5,-7.5,-13.800000000037));
#140504=CARTESIAN_POINT('',(10.9,-7.5,-8.45000000000173));
#140505=CARTESIAN_POINT('',(15.1343145750407,-7.5,-8.94705627487115));
#140506=CARTESIAN_POINT('',(14.89999999999,-7.5,-8.3813708499204));
#140507=CARTESIAN_POINT('Origin',(15.69999999999,-7.5,-8.38137084992191));
#140508=CARTESIAN_POINT('',(14.8999999999893,-7.5,-8.71274169981976));
#140509=CARTESIAN_POINT('',(10.2965705850743,-7.5,-8.34761172707562));
#140510=CARTESIAN_POINT('Origin',(10.4128562056381,-7.5,-8.93623525230213));
#140511=CARTESIAN_POINT('',(11.608349401414,-7.5,-7.90779663028513));
#140512=CARTESIAN_POINT('Origin',(9.25,-7.5,-3.05000000003699));
#140513=CARTESIAN_POINT('',(13.9888110834979,-7.5,-7.18263475607025));
#140514=CARTESIAN_POINT('Origin',(15.1,-7.5,-15.1));
#140515=CARTESIAN_POINT('',(14.8999999999907,-7.5,-7.9748702165563));
#140516=CARTESIAN_POINT('Origin',(14.0999999999907,-7.5,-7.97487021655479));
#140517=CARTESIAN_POINT('',(14.9000000000107,-7.5,2.61274169977414));
#140518=CARTESIAN_POINT('',(13.55,-7.5,-15.1));
#140519=CARTESIAN_POINT('Origin',(15.1,-7.5,-15.1));
#140520=CARTESIAN_POINT('Origin',(-15.5,4.2410519540681E-15,-19.1));
#140521=CARTESIAN_POINT('',(-15.5,4.24105195407812E-15,-19.1000000000451));
#140522=CARTESIAN_POINT('',(-15.5,4.24105195407812E-15,-19.1000000000451));
#140523=CARTESIAN_POINT('',(15.1,4.2410519540681E-15,-19.1));
#140524=CARTESIAN_POINT('',(-69.9000013262034,4.2410519540681E-15,-19.1));
#140525=CARTESIAN_POINT('',(15.1,4.2410519540681E-15,-19.1));
#140526=CARTESIAN_POINT('Origin',(18.3,-12.2,-10.9813708499319));
#140527=CARTESIAN_POINT('',(19.1,2.43835415190839E-15,-10.9813708499319));
#140528=CARTESIAN_POINT('',(19.1,-12.2,-10.9813708499319));
#140529=CARTESIAN_POINT('',(18.8656854249492,1.57444844383239E-15,-10.4156854249827));
#140530=CARTESIAN_POINT('Origin',(18.3,2.22044604925031E-15,-10.9813708499319));
#140531=CARTESIAN_POINT('',(18.8656854249492,-12.2,-10.4156854249827));
#140532=CARTESIAN_POINT('Origin',(19.1,-24.4,-10.6500000000335));
#140533=CARTESIAN_POINT('',(16.734314575042,1.101189045516E-15,-8.28431457507544));
#140534=CARTESIAN_POINT('',(11.7749999999916,0.,-3.3250000000251));
#140535=CARTESIAN_POINT('',(16.734314575042,-24.4,-8.28431457507545));
#140536=CARTESIAN_POINT('Origin',(-2.25752749827279E-11,9.99200722212761E-17,
-0.450000000022572));
#140537=CARTESIAN_POINT('',(19.1,3.35287353436797E-15,-15.1));
#140538=CARTESIAN_POINT('',(19.1,4.2410519540681E-15,-19.1));
#140539=CARTESIAN_POINT('Origin',(15.1,3.35287353436797E-15,-15.1));
#140540=CARTESIAN_POINT('',(-19.1,4.33378681544358E-15,-15.5));
#140541=CARTESIAN_POINT('Origin',(-15.5,3.44169137633798E-15,-15.5));
#140542=CARTESIAN_POINT('',(-19.1,3.33044959100488E-15,-10.9813708498909));
#140543=CARTESIAN_POINT('',(-19.1,0.,4.0176406871349));
#140544=CARTESIAN_POINT('',(-18.8656854249492,1.86310643022669E-15,-10.4156854249416));
#140545=CARTESIAN_POINT('Origin',(-18.3,4.44089209850063E-15,-10.9813708498909));
#140546=CARTESIAN_POINT('',(-16.7343145750813,1.38984703191903E-15,-8.28431457507367));
#140547=CARTESIAN_POINT('',(-10.4750000000288,0.,-2.02500000002115));
#140548=CARTESIAN_POINT('Origin',(-17.3000000000305,0.,-7.71862915012443));
#140549=CARTESIAN_POINT('',(-16.2656854249441,-5.7894794125451E-15,11.4343145750533));
#140550=CARTESIAN_POINT('Origin',(-15.6999999999955,0.,10.8686291501034));
#140551=CARTESIAN_POINT('',(-9.73431457503237,-7.23973507252925E-15,17.9656854249499));
#140552=CARTESIAN_POINT('',(-12.3391827499422,-6.66133814775094E-15,15.3608172500461));
#140553=CARTESIAN_POINT('',(-9.16862915008379,-4.04121180963557E-15,18.2));
#140554=CARTESIAN_POINT('Origin',(-9.16862915008379,-4.44089209850063E-15,
17.4));
#140555=CARTESIAN_POINT('',(11.5427649064299,-4.04121180963557E-15,18.2));
#140556=CARTESIAN_POINT('',(-11.2907461519216,-4.04121180963557E-15,18.2));
#140557=CARTESIAN_POINT('',(12.6059538781827,-4.13252265231712E-15,18.6112274770755));
#140558=CARTESIAN_POINT('Origin',(11.5427649064299,-4.39204228541712E-15,
19.78));
#140559=CARTESIAN_POINT('',(17.0909902576697,-4.10898067127859E-15,18.5052038200428));
#140560=CARTESIAN_POINT('Origin',(14.7928932188134,-3.59870062220636E-15,
16.2071067811865));
#140561=CARTESIAN_POINT('',(18.5052038200428,-3.79496217954183E-15,17.0909902576697));
#140562=CARTESIAN_POINT('',(18.5052038200428,-3.79496217954183E-15,17.0909902576697));
#140563=CARTESIAN_POINT('',(19.3750857890412,-3.1235797785265E-15,14.067352726634));
#140564=CARTESIAN_POINT('Origin',(16.2071067811865,-3.28468213046961E-15,
14.7928932188135));
#140565=CARTESIAN_POINT('',(19.1,-2.58326727508653E-15,11.6340015374781));
#140566=CARTESIAN_POINT('Origin',(30.,-2.58326727508653E-15,11.6340015374781));
#140567=CARTESIAN_POINT('',(19.1,-1.08388206185084E-15,4.88137084986501));
#140568=CARTESIAN_POINT('',(19.1,4.2410519540681E-15,-19.1));
#140569=CARTESIAN_POINT('',(18.8656854249492,-1.57444844383014E-15,4.31568542491578));
#140570=CARTESIAN_POINT('Origin',(18.3,-2.22044604925031E-15,4.88137084986501));
#140571=CARTESIAN_POINT('',(16.7343145750595,-1.10118904551765E-15,2.18431457502608));
#140572=CARTESIAN_POINT('',(11.7750000000018,0.,-2.77500000003168));
#140573=CARTESIAN_POINT('',(16.5000000000088,-1.30309744108929E-15,1.61862915007835));
#140574=CARTESIAN_POINT('Origin',(17.3000000000088,0.,1.61862915007684));
#140575=CARTESIAN_POINT('',(16.4999999999912,7.70190389262261E-16,-7.7186291501247));
#140576=CARTESIAN_POINT('',(16.4999999999977,0.,-4.25000000003884));
#140577=CARTESIAN_POINT('Origin',(17.2999999999912,0.,-7.7186291501262));
#140578=CARTESIAN_POINT('',(17.338477631085,-3.53589692385901E-15,15.9242640687119));
#140579=CARTESIAN_POINT('',(15.9242640687119,-3.84991541559577E-15,17.338477631085));
#140580=CARTESIAN_POINT('',(16.3903174593052,-3.74643077460751E-15,16.8724242404918));
#140581=CARTESIAN_POINT('',(13.661522368915,-3.34748582881696E-15,15.0757359312881));
#140582=CARTESIAN_POINT('Origin',(14.7928932188134,-3.59870062220636E-15,
16.2071067811865));
#140583=CARTESIAN_POINT('',(15.0757359312881,-3.0334673370802E-15,13.661522368915));
#140584=CARTESIAN_POINT('',(14.8346825406948,-3.08699194196033E-15,13.9025757595082));
#140585=CARTESIAN_POINT('Origin',(16.2071067811865,-3.28468213046961E-15,
14.7928932188135));
#140586=CARTESIAN_POINT('',(-17.1,3.44169137633798E-15,-15.5));
#140587=CARTESIAN_POINT('Origin',(-15.5,3.44169137633798E-15,-15.5));
#140588=CARTESIAN_POINT('',(13.55,3.35287353436797E-15,-15.1));
#140589=CARTESIAN_POINT('Origin',(15.1,3.35287353436797E-15,-15.1));
#140590=CARTESIAN_POINT('',(-11.5275012782661,-2.33286334807598E-15,10.5062825051013));
#140591=CARTESIAN_POINT('Origin',(-8.47750127826606,-2.33286334807598E-15,
10.5062825051013));
#140592=CARTESIAN_POINT('Origin',(17.2999999999912,-24.4,-7.71862915012621));
#140593=CARTESIAN_POINT('',(16.4999999999912,-24.4,-7.7186291501247));
#140594=CARTESIAN_POINT('Origin',(16.4999999999906,-24.4,-8.05000000002406));
#140595=CARTESIAN_POINT('',(16.5000000000088,-6.6,1.61862915007835));
#140596=CARTESIAN_POINT('',(16.5000000000088,-24.4,1.61862915007834));
#140597=CARTESIAN_POINT('',(16.4999999999948,-6.6,-5.80993508719201));
#140598=CARTESIAN_POINT('',(16.5000000000094,-6.6,1.94999999997594));
#140599=CARTESIAN_POINT('Ctrl Pts',(16.4999999999931,-7.50000000000005,
-6.72119489704353));
#140600=CARTESIAN_POINT('Ctrl Pts',(16.4999999999939,-7.0732084403293,-6.28848666173585));
#140601=CARTESIAN_POINT('Ctrl Pts',(16.4999999999948,-6.6,-5.809935087192));
#140602=CARTESIAN_POINT('Origin',(17.3000000000088,-24.4,1.61862915007684));
#140603=CARTESIAN_POINT('',(16.7343145750595,-6.6,2.18431457502608));
#140604=CARTESIAN_POINT('Origin',(17.3000000000088,-6.6,1.61862915007684));
#140605=CARTESIAN_POINT('',(16.7343145750595,-24.4,2.18431457502608));
#140606=CARTESIAN_POINT('Origin',(18.3,-12.2,4.88137084986501));
#140607=CARTESIAN_POINT('',(19.1,-7.5,4.88137084986501));
#140608=CARTESIAN_POINT('',(19.1,-12.2,4.88137084986501));
#140609=CARTESIAN_POINT('',(18.8656854249492,-7.5,4.31568542491577));
#140610=CARTESIAN_POINT('Origin',(18.3,-7.5,4.88137084986501));
#140611=CARTESIAN_POINT('',(18.8656854249492,-12.2,4.31568542491577));
#140612=CARTESIAN_POINT('Origin',(16.5000000000094,-24.4,1.94999999997594));
#140613=CARTESIAN_POINT('',(17.5765623826223,-7.5,3.02656238258888));
#140614=CARTESIAN_POINT('',(14.7125000000122,-7.5,0.162499999978742));
#140615=CARTESIAN_POINT('',(16.7650854557587,-6.6,2.2150854557252));
#140616=CARTESIAN_POINT('Ctrl Pts',(16.7650854557587,-6.6,2.2150854557252));
#140617=CARTESIAN_POINT('Ctrl Pts',(17.1605923305092,-7.03154955968907,
2.61059233047575));
#140618=CARTESIAN_POINT('Ctrl Pts',(17.5765623826223,-7.5,3.02656238258888));
#140619=CARTESIAN_POINT('',(19.1,-6.6,4.54999999996654));
#140620=CARTESIAN_POINT('Origin',(13.1,-7.5,-1.80000000000345));
#140621=CARTESIAN_POINT('',(19.1,-7.5,10.5927097051057));
#140622=CARTESIAN_POINT('',(19.1,-7.5,1.1207142142697));
#140623=CARTESIAN_POINT('',(18.0728653213373,-7.5,11.5923414919222));
#140624=CARTESIAN_POINT('Origin',(18.1,-7.5,10.5927097051057));
#140625=CARTESIAN_POINT('',(14.7581088559379,-7.5,11.502363509309));
#140626=CARTESIAN_POINT('',(14.5178464431778,-7.5,11.4958416645148));
#140627=CARTESIAN_POINT('',(13.2896259362394,-7.5,12.0874135205689));
#140628=CARTESIAN_POINT('Origin',(14.7038394986125,-7.5,13.501627082942));
#140629=CARTESIAN_POINT('',(13.8999999999996,-7.5,11.4770394568086));
#140630=CARTESIAN_POINT('',(15.5737177837348,-7.5,9.80332167307343));
#140631=CARTESIAN_POINT('',(13.8999999999997,-7.5,9.24999999996345));
#140632=CARTESIAN_POINT('',(13.8999999999997,-7.5,6.29999983906575));
#140633=CARTESIAN_POINT('',(13.8988113452808,-7.5,9.11383245348325));
#140634=CARTESIAN_POINT('Origin',(6.09999999999969,-7.5,9.2499999999633));
#140635=CARTESIAN_POINT('',(14.6769816890462,-7.5,9.89957198073334));
#140636=CARTESIAN_POINT('Origin',(14.6986894319763,-7.5,9.09986655128017));
#140637=CARTESIAN_POINT('',(16.8837191928024,-7.5,9.959473150191));
#140638=CARTESIAN_POINT('',(13.3419069426877,-7.5,9.86333181239245));
#140639=CARTESIAN_POINT('',(17.5,-7.5,9.35969407810112));
#140640=CARTESIAN_POINT('Origin',(16.9,-7.5,9.35969407810112));
#140641=CARTESIAN_POINT('',(17.5,-7.5,4.08810094579999));
#140642=CARTESIAN_POINT('',(5.47101535039538,-7.5,6.69083194173083));
#140643=CARTESIAN_POINT('Origin',(0.213371879229554,-7.49999999999998,-93.1708583360234));
#140644=CARTESIAN_POINT('Origin',(5.5130764981647,-7.5,7.48972546395287));
#140645=CARTESIAN_POINT('Origin',(15.1,-7.5,-15.1));
#140646=CARTESIAN_POINT('Origin',(-9.16862915008379,-12.2,17.4));
#140647=CARTESIAN_POINT('',(-9.73431457503237,-2.60000000000001,17.9656854249499));
#140648=CARTESIAN_POINT('',(-9.73431457503237,-12.2,17.9656854249499));
#140649=CARTESIAN_POINT('',(-9.16862915008379,-2.6,18.2));
#140650=CARTESIAN_POINT('Origin',(-9.16862915008379,-2.6,17.4));
#140651=CARTESIAN_POINT('',(-9.16862915008379,-12.2,18.2));
#140652=CARTESIAN_POINT('Origin',(-10.6033654998821,-24.4,17.0966345001022));
#140653=CARTESIAN_POINT('',(-16.2656854249441,-2.60000000000001,11.4343145750533));
#140654=CARTESIAN_POINT('',(-16.2656854249441,-24.4,11.4343145750533));
#140655=CARTESIAN_POINT('',(-12.3391827499422,-2.60000000000001,15.3608172500461));
#140656=CARTESIAN_POINT('Origin',(-15.6999999999955,-24.4,10.8686291501034));
#140657=CARTESIAN_POINT('Origin',(-15.6999999999955,-2.6,10.8686291501034));
#140658=CARTESIAN_POINT('Origin',(-2.25752749827279E-11,-2.6,-0.450000000022573));
#140659=CARTESIAN_POINT('',(-13.1262499063287,-2.6,10.398411317633));
#140660=CARTESIAN_POINT('Origin',(-13.926034616533,-2.6,10.3798528337675));
#140661=CARTESIAN_POINT('',(-9.43078548284916,-2.6,5.95504649437932));
#140662=CARTESIAN_POINT('Origin',(-8.47750127826606,-2.6,10.5062825051013));
#140663=CARTESIAN_POINT('',(-8.89058649647473,-2.6,4.79243901829667));
#140664=CARTESIAN_POINT('Origin',(-9.59479136750862,-2.6,5.17203814844866));
#140665=CARTESIAN_POINT('',(-10.0921204701253,-2.6,-0.398878940274963));
#140666=CARTESIAN_POINT('Origin',(9.00768359641396E-11,-2.6,2.56054600265843E-10));
#140667=CARTESIAN_POINT('Origin',(-10.8914963489756,-2.6,-0.430473311803018));
#140668=CARTESIAN_POINT('Origin',(7.25952771151622,-2.6,9.86720616009051));
#140669=CARTESIAN_POINT('',(-6.85606479211595,-2.6,16.4647218026392));
#140670=CARTESIAN_POINT('Origin',(-6.74267665483338,-2.6,15.6727981129294));
#140671=CARTESIAN_POINT('',(-4.95681349263295,-2.6,16.6));
#140672=CARTESIAN_POINT('Origin',(-4.95681349263295,-2.6,3.2));
#140673=CARTESIAN_POINT('',(1.39248124878044,-2.6,16.6));
#140674=CARTESIAN_POINT('',(-2.47840674632776,-2.6,16.6));
#140675=CARTESIAN_POINT('Origin',(1.39248124878044,-2.6,15.8));
#140676=CARTESIAN_POINT('',(1.55054365106131,-2.6,18.2));
#140677=CARTESIAN_POINT('Origin',(1.55054365106131,-2.6,17.8));
#140678=CARTESIAN_POINT('',(19.1,-2.6,18.2));
#140679=CARTESIAN_POINT('',(-11.5275012782661,-2.6,10.5062825051013));
#140680=CARTESIAN_POINT('Origin',(-8.47750127826606,-2.6,10.5062825051013));
#140681=CARTESIAN_POINT('Origin',(-17.3000000000305,-24.4,-7.71862915012444));
#140682=CARTESIAN_POINT('',(-16.7343145750813,-24.4,-8.28431457507368));
#140683=CARTESIAN_POINT('Origin',(-18.3,-24.4,-10.9813708498909));
#140684=CARTESIAN_POINT('',(-19.1,-24.4,-10.9813708498909));
#140685=CARTESIAN_POINT('',(-18.8656854249492,-24.4,-10.4156854249417));
#140686=CARTESIAN_POINT('Origin',(-16.5000000000311,-24.4,-8.05000000002354));
#140687=CARTESIAN_POINT('',(-17.8000000000336,-17.35,-9.35000000002598));
#140688=CARTESIAN_POINT('Origin',(-16.6686291501351,-10.3,-10.4813708499245));
#140689=CARTESIAN_POINT('',(-16.6686291501351,-5.95,-10.4813708499245));
#140690=CARTESIAN_POINT('Origin',(9.25,-7.5,-3.05000000003699));
#140691=CARTESIAN_POINT('',(11.608349401414,-7.5,-7.90779663028513));
#140692=CARTESIAN_POINT('',(10.2965705850743,-8.9,-8.34761172707562));
#140693=CARTESIAN_POINT('Origin',(15.1,-7.5,-15.1));
#140694=CARTESIAN_POINT('',(13.9888110834979,-7.5,-7.18263475607025));
#140695=CARTESIAN_POINT('Origin',(14.0999999999907,-7.5,-7.97487021655479));
#140696=CARTESIAN_POINT('',(14.8999999999907,-7.5,-7.9748702165563));
#140697=CARTESIAN_POINT('Origin',(14.8999999999924,-1.6,-7.10754022756819));
#140698=CARTESIAN_POINT('',(14.89999999999,-1.6,-8.3813708499204));
#140699=CARTESIAN_POINT('Origin',(15.69999999999,-1.6,-8.38137084992191));
#140700=CARTESIAN_POINT('',(15.1343145750407,-1.6,-8.94705627487115));
#140701=CARTESIAN_POINT('Origin',(14.8999999999893,-1.6,-8.71274169981976));
#140702=CARTESIAN_POINT('Origin',(8.16898488501357,-7.5,-6.27357043065748));
#140703=CARTESIAN_POINT('',(7.69312168782831,-6.6,-5.90811972595898));
#140704=CARTESIAN_POINT('',(7.69312168782831,-7.5,-5.90811972595898));
#140705=CARTESIAN_POINT('',(7.97821751178067,-6.6,-6.84243580076698));
#140706=CARTESIAN_POINT('Origin',(8.16898488501357,-6.6,-6.27357043065748));
#140707=CARTESIAN_POINT('',(7.97821751178067,-7.5,-6.84243580076698));
#140708=CARTESIAN_POINT('Origin',(-2.12720466293355E-17,-7.5,-1.66578428666901E-15));
#140709=CARTESIAN_POINT('',(9.65595769539761,-6.6,0.923298968206738));
#140710=CARTESIAN_POINT('',(9.65595769539761,-7.5,0.923298968206738));
#140711=CARTESIAN_POINT('Origin',(-2.12720466293355E-17,-6.6,-1.48411142809398E-15));
#140712=CARTESIAN_POINT('Origin',(10.2532334291335,-7.5,0.98041024459066));
#140713=CARTESIAN_POINT('Origin',(10.2532334291335,-6.6,0.98041024459066));
#140714=CARTESIAN_POINT('Origin',(15.1,-10.3,-15.1));
#140715=CARTESIAN_POINT('',(13.5220680886962,-10.3,8.5924743090986));
#140716=CARTESIAN_POINT('',(13.5220680886962,-10.3,8.5924743090986));
#140717=CARTESIAN_POINT('',(10.3106112119491,-10.3,8.1569336551683));
#140718=CARTESIAN_POINT('Origin',(15.1,-10.3,-15.1));
#140719=CARTESIAN_POINT('',(10.3106112119491,-10.3,8.1569336551683));
#140720=CARTESIAN_POINT('Origin',(13.4954867544557,-10.3,8.99159012270412));
#140721=CARTESIAN_POINT('',(13.8952427952371,-10.3,8.97762202123065));
#140722=CARTESIAN_POINT('',(13.8952427952371,-10.3,8.97762202123065));
#140723=CARTESIAN_POINT('Origin',(13.4954867544557,-10.3,8.99159012270412));
#140724=CARTESIAN_POINT('Origin',(6.09999999999969,-7.5,9.2499999999633));
#140725=CARTESIAN_POINT('',(13.8988113452808,-7.5,9.11383245348325));
#140726=CARTESIAN_POINT('',(13.8999999999997,-10.3,9.24999999996345));
#140727=CARTESIAN_POINT('',(13.8999999999997,-7.5,9.24999999996345));
#140728=CARTESIAN_POINT('Origin',(6.09999999999969,-10.3,9.2499999999633));
#140729=CARTESIAN_POINT('Origin',(14.6986894319763,-7.5,9.09986655128017));
#140730=CARTESIAN_POINT('',(14.6769816890462,-7.5,9.89957198073334));
#140731=CARTESIAN_POINT('Origin',(13.8999999999997,-7.5,9.87848106632152));
#140732=CARTESIAN_POINT('',(16.8837191928024,-7.5,9.959473150191));
#140733=CARTESIAN_POINT('Origin',(16.9,-7.5,9.35969407810112));
#140734=CARTESIAN_POINT('',(17.5,-7.5,9.35969407810112));
#140735=CARTESIAN_POINT('Origin',(17.5,-7.5,9.97620189160342));
#140736=CARTESIAN_POINT('Origin',(15.8325427278768,-6.6,-1.75748667391245));
#140737=CARTESIAN_POINT('Origin',(15.1,-6.6,-15.1));
#140738=CARTESIAN_POINT('Origin',(15.1,-6.6,-15.1));
#140739=CARTESIAN_POINT('Origin',(-15.5,-10.3,-15.5));
#140740=CARTESIAN_POINT('',(-16.4600000000227,-10.3,-12.4473945554729));
#140741=CARTESIAN_POINT('',(-15.0612959521201,-10.3,-12.3302147141527));
#140742=CARTESIAN_POINT('Origin',(-16.7000000000283,-10.3,-11.6842431943411));
#140743=CARTESIAN_POINT('',(-17.5000000000283,-10.3,-11.6842431943471));
#140744=CARTESIAN_POINT('Origin',(-17.5,-1.6,-15.4999999999881));
#140745=CARTESIAN_POINT('',(-17.5000000000286,-1.6,-11.6441125497224));
#140746=CARTESIAN_POINT('Origin',(-16.7000000000286,-1.6,-11.6441125497165));
#140747=CARTESIAN_POINT('',(-17.2656854249779,-1.6,-11.0784271247672));
#140748=CARTESIAN_POINT('Origin',(-17.5000000000311,-1.6,-11.3127416998205));
#140749=CARTESIAN_POINT('',(-15.1343145750825,-1.6,-8.94705627487187));
#140750=CARTESIAN_POINT('Origin',(-15.7000000000318,-1.6,-8.38137084992263));
#140751=CARTESIAN_POINT('Origin',(-9.59479136750862,-2.6,5.17203814844866));
#140752=CARTESIAN_POINT('',(-8.89058649647473,-2.6,4.79243901829667));
#140753=CARTESIAN_POINT('',(-9.43078548284916,-2.6,5.95504649437932));
#140754=CARTESIAN_POINT('Origin',(9.00768359641396E-11,-2.6,2.56054600265843E-10));
#140755=CARTESIAN_POINT('',(-10.0921204701253,-2.6,-0.398878940274965));
#140756=CARTESIAN_POINT('Origin',(-10.8914963489756,-2.6,-0.430473311803018));
#140757=CARTESIAN_POINT('Origin',(-13.926034616533,-2.6,10.3798528337675));
#140758=CARTESIAN_POINT('',(-13.1262499063287,-2.6,10.398411317633));
#140759=CARTESIAN_POINT('Origin',(-8.47750127826606,-2.6,10.5062825051013));
#140760=CARTESIAN_POINT('Origin',(-19.1,-24.4,8.48528137429235));
#140761=CARTESIAN_POINT('',(-19.1,4.88334721263554E-15,-15.5));
#140762=CARTESIAN_POINT('Origin',(15.1,-7.05,-15.1));
#140763=CARTESIAN_POINT('Origin',(15.1,-6.6,-15.1));
#140764=CARTESIAN_POINT('Origin',(19.1,4.2410519540681E-15,-19.1));
#140765=CARTESIAN_POINT('',(19.1,3.35287353436797E-15,-15.1));
#140766=CARTESIAN_POINT('Origin',(19.1,4.2410519540681E-15,-19.1));
#140767=CARTESIAN_POINT('',(19.1,-5.,11.6340015374781));
#140768=CARTESIAN_POINT('',(19.1,-5.5,11.6340015374781));
#140769=CARTESIAN_POINT('',(19.1,-5.,10.5927097051057));
#140770=CARTESIAN_POINT('',(19.1,-5.,-1.9375));
#140771=CARTESIAN_POINT('',(19.1,-2.75,10.5927097051057));
#140772=CARTESIAN_POINT('Origin',(-15.5,3.44169137633798E-15,-15.5));
#140773=CARTESIAN_POINT('Origin',(-4.21607216363254,-10.1,-7.2584996763473));
#140774=CARTESIAN_POINT('',(-0.796199698700571,-10.1,-9.30032612545083));
#140775=CARTESIAN_POINT('Origin',(0.00380023450634744,-10.1,-9.29999922356006));
#140776=CARTESIAN_POINT('Origin',(-6.1338854524033,-10.1,-4.97849869506814));
#140777=CARTESIAN_POINT('',(-0.795830131689239,-10.1,-10.2047368760032));
#140778=CARTESIAN_POINT('Origin',(-1.39583008159634,-10.1,-10.204982052423));
#140779=CARTESIAN_POINT('',(-0.795830131689239,-10.1,-10.2047368760032));
#140780=CARTESIAN_POINT('Origin',(-1.39583008159634,-10.3,-10.204982052423));
#140781=CARTESIAN_POINT('',(-0.795830131689239,-10.3,-10.2047368760032));
#140782=CARTESIAN_POINT('Origin',(-6.1338854524033,-10.3,-4.97849869506814));
#140783=CARTESIAN_POINT('Origin',(-11.9533418970136,-2.6,-0.350905528319926));
#140784=CARTESIAN_POINT('Origin',(-2.25730545366787E-11,-10.4,-0.450000000022575));
#140785=CARTESIAN_POINT('',(-7.8,-10.4,-3.05000000003699));
#140786=CARTESIAN_POINT('Origin',(-9.35,-10.4,-3.05000000003699));
#140787=CARTESIAN_POINT('Origin',(-15.5,-10.3,-15.5));
#140788=CARTESIAN_POINT('',(-13.9781746176887,-10.1,-12.419231543135));
#140789=CARTESIAN_POINT('',(-13.9781746176887,-10.3,-12.419231543135));
#140790=CARTESIAN_POINT('',(-14.5846229736965,-10.1,-12.1880260147795));
#140791=CARTESIAN_POINT('Origin',(-15.5,-10.1,-15.5));
#140792=CARTESIAN_POINT('',(-14.5846229736965,-10.3,-12.1880260147795));
#140793=CARTESIAN_POINT('Origin',(-9.35,-10.3,-3.05000000003699));
#140794=CARTESIAN_POINT('Origin',(-9.35,-10.1,-3.05000000003699));
#140795=CARTESIAN_POINT('Origin',(-12.176305656554,-10.1,-9.1169160676784));
#140796=CARTESIAN_POINT('Origin',(-14.9790389431426,-10.1,-11.7358799730564));
#140797=CARTESIAN_POINT('Origin',(-14.9790389431426,-10.3,-11.7358799730564));
#140798=CARTESIAN_POINT('Origin',(0.213371879229554,-4.4814254252597E-16,
-93.1708583360234));
#140799=CARTESIAN_POINT('',(5.47101535039538,-10.3,6.69083194173083));
#140800=CARTESIAN_POINT('Origin',(0.213371879229554,-10.3,-93.1708583360234));
#140801=CARTESIAN_POINT('',(5.47101535039538,-2.26218921073957E-14,6.69083194173083));
#140802=CARTESIAN_POINT('Origin',(5.5130764981647,-1.91165057187814E-16,
7.48972546395287));
#140803=CARTESIAN_POINT('Origin',(5.5130764981647,-10.3,7.48972546395286));
#140804=CARTESIAN_POINT('Origin',(9.94289321881345,-10.3,16.2));
#140805=CARTESIAN_POINT('',(9.94289321881345,-10.3,13.7509759234611));
#140806=CARTESIAN_POINT('',(9.94289321881345,-10.3,13.7509759234611));
#140807=CARTESIAN_POINT('',(9.94289321881345,-10.3,15.6));
#140808=CARTESIAN_POINT('',(9.94289321881345,-10.3,7.87499999998871));
#140809=CARTESIAN_POINT('',(9.94289321881345,-10.3,15.6));
#140810=CARTESIAN_POINT('Origin',(9.34289321881345,-10.3,13.7509759234611));
#140811=CARTESIAN_POINT('',(9.0224799018401,-10.3,13.243693648681));
#140812=CARTESIAN_POINT('',(9.0224799018401,-10.3,13.243693648681));
#140813=CARTESIAN_POINT('Origin',(9.34289321881345,-10.3,13.7509759234611));
#140814=CARTESIAN_POINT('Origin',(7.1,-10.3,10.2));
#140815=CARTESIAN_POINT('Origin',(7.1,-10.3,10.2));
#140816=CARTESIAN_POINT('Origin',(5.74909217812359,-10.3,-8.54622369438117));
#140817=CARTESIAN_POINT('',(6.14689326954821,-10.3,-8.09705302340923));
#140818=CARTESIAN_POINT('',(5.41419360512517,-10.3,-8.0483854216423));
#140819=CARTESIAN_POINT('Origin',(8.6,-10.3,-5.32716721908225));
#140820=CARTESIAN_POINT('',(7.33287671232876,-10.3,-8.80342937459372));
#140821=CARTESIAN_POINT('Origin',(6.1,-10.3,-12.1857384988752));
#140822=CARTESIAN_POINT('Origin',(-0.796152266589922,-10.3,-9.41640280839959));
#140823=CARTESIAN_POINT('',(-0.79309436390975,-10.3,-16.899754823607));
#140824=CARTESIAN_POINT('',(-0.796199698700571,-10.3,-9.30032612545083));
#140825=CARTESIAN_POINT('Origin',(-1.39309431381685,-10.3,-16.9000000000267));
#140826=CARTESIAN_POINT('',(-1.39309431381607,-10.3,-17.5000000000267));
#140827=CARTESIAN_POINT('Origin',(-0.792849087283714,-10.3,-17.500000000026));
#140828=CARTESIAN_POINT('',(-11.9672956534841,-10.3,-17.5000000000405));
#140829=CARTESIAN_POINT('Origin',(-11.9672956534849,-10.3,-16.9000000000405));
#140830=CARTESIAN_POINT('',(-12.5250910766189,-10.3,-16.6789473684552));
#140831=CARTESIAN_POINT('Origin',(-15.5,-10.3,-15.5));
#140832=CARTESIAN_POINT('Origin',(-6.74267665483338,-2.6,15.6727981129294));
#140833=CARTESIAN_POINT('',(-6.85606479211595,-2.6,16.4647218026392));
#140834=CARTESIAN_POINT('Origin',(-4.95681349263295,-2.6,3.2));
#140835=CARTESIAN_POINT('',(-4.95681349263295,-2.6,16.6));
#140836=CARTESIAN_POINT('Origin',(-4.95681349263295,-2.6,16.6));
#140837=CARTESIAN_POINT('',(1.39248124878044,-2.6,16.6));
#140838=CARTESIAN_POINT('Origin',(1.39248124878044,-2.6,15.8));
#140839=CARTESIAN_POINT('Origin',(9.34289321881345,-10.3,15.6));
#140840=CARTESIAN_POINT('Origin',(9.34289321881345,-10.3,15.6));
#140841=CARTESIAN_POINT('Origin',(10.4128562056381,-8.9,-8.93623525230213));
#140842=CARTESIAN_POINT('Origin',(-5.6920614055489E-17,-10.3,-2.28766658394441E-15));
#140843=CARTESIAN_POINT('',(1.32237339244619,-10.3,-9.60943957263029));
#140844=CARTESIAN_POINT('Origin',(1.4041696846368,-10.3,-10.2038378957974));
#140845=CARTESIAN_POINT('Origin',(0.00380023450634744,-10.3,-9.29999922356006));
#140846=CARTESIAN_POINT('Origin',(-2.25730545366787E-11,-10.3,-0.450000000022575));
#140847=CARTESIAN_POINT('Origin',(10.4719722228657,-10.3,7.37337598393027));
#140848=CARTESIAN_POINT('',(13.8999999999996,-10.3,11.4770394568086));
#140849=CARTESIAN_POINT('',(13.8999999999997,-10.3,6.97499983905631));
#140850=CARTESIAN_POINT('',(12.1286796564404,-10.3,13.2483598003679));
#140851=CARTESIAN_POINT('',(11.961217783734,-10.3,13.4158216730743));
#140852=CARTESIAN_POINT('',(11.5428932188134,-10.3,14.662573362741));
#140853=CARTESIAN_POINT('Origin',(13.5428932188134,-10.3,14.662573362741));
#140854=CARTESIAN_POINT('',(11.5428932188134,-10.3,17.2));
#140855=CARTESIAN_POINT('',(11.5428932188134,-10.3,8.87499999998871));
#140856=CARTESIAN_POINT('',(10.5428932188134,-10.3,18.2));
#140857=CARTESIAN_POINT('Origin',(10.5428932188134,-10.3,17.2));
#140858=CARTESIAN_POINT('',(1.55054365106132,-10.3,18.2));
#140859=CARTESIAN_POINT('',(19.1,-10.3,18.2));
#140860=CARTESIAN_POINT('Origin',(1.55054365106131,-10.3,17.8));
#140861=CARTESIAN_POINT('Origin',(7.25952771151622,-10.3,9.86720616009051));
#140862=CARTESIAN_POINT('',(9.4,-10.3,10.2));
#140863=CARTESIAN_POINT('Origin',(7.1,-10.3,10.2));
#140864=CARTESIAN_POINT('Origin',(9.25,-7.05,-3.05000000003699));
#140865=CARTESIAN_POINT('Origin',(9.24999999999998,-6.6,-3.05000000003696));
#140866=CARTESIAN_POINT('Origin',(9.25,-6.6,-3.05000000003699));
#140867=CARTESIAN_POINT('',(10.9969254825289,-6.6,-6.64836787429487));
#140868=CARTESIAN_POINT('Origin',(9.24999999999998,-7.5,-3.05000000003696));
#140869=CARTESIAN_POINT('Origin',(7.25952771151622,-2.6,9.86720616009051));
#140870=CARTESIAN_POINT('Origin',(10.5,-10.3,-13.400000000037));
#140871=CARTESIAN_POINT('',(10.5,-10.3,-13.400000000037));
#140872=CARTESIAN_POINT('Origin',(10.5,-10.3,-13.800000000037));
#140873=CARTESIAN_POINT('',(10.9,-10.3,-13.800000000037));
#140874=CARTESIAN_POINT('Origin',(10.9,-10.3,-15.1));
#140875=CARTESIAN_POINT('Origin',(10.4719722228657,-10.3,7.37337598393027));
#140876=CARTESIAN_POINT('Origin',(18.4241839371104,-6.6,-4.3509818715809));
#140877=CARTESIAN_POINT('Origin',(7.1,-1.00000000000001,10.2));
#140878=CARTESIAN_POINT('',(8.7,-1.00000000000001,10.2));
#140879=CARTESIAN_POINT('Origin',(7.1,-1.00000000000001,10.2));
#140880=CARTESIAN_POINT('Origin',(7.1,-24.4,10.2));
#140881=CARTESIAN_POINT('',(8.7,-4.9,10.2));
#140882=CARTESIAN_POINT('Origin',(7.1,-4.9,10.2));
#140883=CARTESIAN_POINT('',(8.7,-24.4,10.2));
#140884=CARTESIAN_POINT('Origin',(7.1,-4.9,10.2));
#140885=CARTESIAN_POINT('',(9.1,-4.9,10.2));
#140886=CARTESIAN_POINT('Origin',(7.1,-4.9,10.2));
#140887=CARTESIAN_POINT('Origin',(15.1,3.35287353436797E-15,-15.1));
#140888=CARTESIAN_POINT('',(13.55,3.35287353436797E-15,-15.1));
#140889=CARTESIAN_POINT('Origin',(14.7928932188134,-5.5,16.2071067811865));
#140890=CARTESIAN_POINT('',(12.6059538781827,-5.,18.6112274770755));
#140891=CARTESIAN_POINT('',(12.6059538781827,-5.50000000000001,18.6112274770755));
#140892=CARTESIAN_POINT('',(17.0909902576697,-5.,18.5052038200428));
#140893=CARTESIAN_POINT('Origin',(14.7928932188134,-5.,16.2071067811865));
#140894=CARTESIAN_POINT('',(17.0909902576697,-5.50000000000001,18.5052038200428));
#140895=CARTESIAN_POINT('Origin',(17.0909902576697,-5.50000000000001,18.5052038200428));
#140896=CARTESIAN_POINT('',(18.5052038200428,-5.,17.0909902576697));
#140897=CARTESIAN_POINT('',(18.5052038200428,-5.5,17.0909902576697));
#140898=CARTESIAN_POINT('',(17.557043648263,-5.,18.0391504294495));
#140899=CARTESIAN_POINT('Origin',(16.2071067811865,-5.5,14.7928932188135));
#140900=CARTESIAN_POINT('',(19.3750857890412,-5.,14.0673527266339));
#140901=CARTESIAN_POINT('',(19.3750857890412,-5.5,14.0673527266339));
#140902=CARTESIAN_POINT('Origin',(16.2071067811865,-5.,14.7928932188135));
#140903=CARTESIAN_POINT('Origin',(14.7928932188134,-5.5,16.2071067811865));
#140904=CARTESIAN_POINT('',(13.661522368915,-5.,15.0757359312881));
#140905=CARTESIAN_POINT('',(15.9242640687119,-5.,17.338477631085));
#140906=CARTESIAN_POINT('Origin',(14.7928932188134,-5.,16.2071067811865));
#140907=CARTESIAN_POINT('',(13.661522368915,-5.5,15.0757359312881));
#140908=CARTESIAN_POINT('',(15.9242640687119,-5.5,17.338477631085));
#140909=CARTESIAN_POINT('Origin',(15.0757359312881,-5.5,13.661522368915));
#140910=CARTESIAN_POINT('',(15.0757359312881,-5.,13.661522368915));
#140911=CARTESIAN_POINT('',(14.8346825406948,-5.,13.9025757595082));
#140912=CARTESIAN_POINT('',(15.0757359312881,-5.5,13.661522368915));
#140913=CARTESIAN_POINT('Origin',(16.2071067811865,-5.5,14.7928932188135));
#140914=CARTESIAN_POINT('',(17.338477631085,-5.,15.9242640687119));
#140915=CARTESIAN_POINT('Origin',(16.2071067811865,-5.,14.7928932188135));
#140916=CARTESIAN_POINT('',(17.338477631085,-5.5,15.9242640687119));
#140917=CARTESIAN_POINT('Origin',(15.9242640687119,-5.5,17.338477631085));
#140918=CARTESIAN_POINT('',(16.3903174593052,-5.,16.8724242404917));
#140919=CARTESIAN_POINT('Origin',(-9.25,-7.2,-3.05000000003699));
#140920=CARTESIAN_POINT('',(-7.8,-7.2,-3.05000000003699));
#140921=CARTESIAN_POINT('Origin',(-9.35,-7.2,-3.05000000003699));
#140922=CARTESIAN_POINT('Origin',(-8.47750127826606,-2.33286334807598E-15,
10.5062825051013));
#140923=CARTESIAN_POINT('',(-11.5275012782661,-2.33286334807598E-15,10.5062825051013));
#140924=CARTESIAN_POINT('Origin',(7.1,-10.3,10.2));
#140925=CARTESIAN_POINT('',(9.1,-10.,10.2));
#140926=CARTESIAN_POINT('Origin',(7.1,-10.,10.2));
#140927=CARTESIAN_POINT('',(9.1,-10.3,10.2));
#140928=CARTESIAN_POINT('Origin',(11.5427649064299,-5.50000000000001,19.78));
#140929=CARTESIAN_POINT('',(11.5427649064299,-5.,18.2));
#140930=CARTESIAN_POINT('Origin',(11.5427649064299,-5.,19.78));
#140931=CARTESIAN_POINT('',(11.5427649064299,-5.50000000000001,18.2));
#140932=CARTESIAN_POINT('Origin',(14.7038394986125,-5.5,13.501627082942));
#140933=CARTESIAN_POINT('',(13.2896259362394,-5.,12.0874135205689));
#140934=CARTESIAN_POINT('',(14.7581088559379,-5.,11.502363509309));
#140935=CARTESIAN_POINT('Origin',(14.7038394986125,-5.,13.501627082942));
#140936=CARTESIAN_POINT('',(13.2896259362394,-5.5,12.0874135205689));
#140937=CARTESIAN_POINT('',(14.7581088559379,-5.5,11.502363509309));
#140938=CARTESIAN_POINT('Origin',(16.2952944868403,-5.5,11.5440899116599));
#140939=CARTESIAN_POINT('',(18.0728653213373,-5.,11.5923414919222));
#140940=CARTESIAN_POINT('',(18.0728653213373,-2.75,11.5923414919222));
#140941=CARTESIAN_POINT('',(16.0352973695706,-5.,11.5370323747515));
#140942=CARTESIAN_POINT('Origin',(30.,-5.5,11.6340015374781));
#140943=CARTESIAN_POINT('Origin',(30.,-5.,11.6340015374781));
#140944=CARTESIAN_POINT('Origin',(15.1,3.35287353436797E-15,-15.1));
#140945=CARTESIAN_POINT('Origin',(18.1,-2.75,10.5927097051057));
#140946=CARTESIAN_POINT('Origin',(18.1,-5.,10.5927097051057));
#140947=CARTESIAN_POINT('Origin',(15.675,-5.,15.225));
#140948=CARTESIAN_POINT('',(11.5428932188134,-5.,14.662573362741));
#140949=CARTESIAN_POINT('',(12.1286796564404,-5.,13.2483598003679));
#140950=CARTESIAN_POINT('Origin',(13.5428932188134,-5.,14.662573362741));
#140951=CARTESIAN_POINT('',(12.2043420607724,-5.,13.1726973960359));
#140952=CARTESIAN_POINT('',(10.5428932188134,-5.,18.2));
#140953=CARTESIAN_POINT('',(17.3875,-5.,18.2));
#140954=CARTESIAN_POINT('',(11.5428932188134,-5.,17.2));
#140955=CARTESIAN_POINT('Origin',(10.5428932188134,-5.,17.2));
#140956=CARTESIAN_POINT('',(11.5428932188134,-5.,16.7125));
#140957=CARTESIAN_POINT('Origin',(15.1,-7.05,-15.1));
#140958=CARTESIAN_POINT('Origin',(-15.5,3.44169137633798E-15,-15.5));
#140959=CARTESIAN_POINT('',(-17.1,3.44169137633798E-15,-15.5));
#140960=CARTESIAN_POINT('Origin',(-9.35,-10.3,-3.05000000003699));
#140961=CARTESIAN_POINT('',(-7.8,-10.3,-3.05000000003699));
#140962=CARTESIAN_POINT('Origin',(7.1,-10.15,10.2));
#140963=CARTESIAN_POINT('',(9.25,-10.15,10.2));
#140964=CARTESIAN_POINT('Origin',(1.55054365106131,-2.6,17.8));
#140965=CARTESIAN_POINT('',(1.55054365106131,-2.6,18.2));
#140966=CARTESIAN_POINT('Origin',(19.1,-4.04121180963557E-15,18.2));
#140967=CARTESIAN_POINT('',(10.5428932188134,-2.75,18.2));
#140968=CARTESIAN_POINT('Origin',(10.5428932188134,-2.75,17.2));
#140969=CARTESIAN_POINT('',(11.5428932188134,-2.75,17.2));
#140970=CARTESIAN_POINT('Origin',(11.5428932188134,-5.50000000000001,18.2));
#140971=CARTESIAN_POINT('',(11.5428932188134,-5.50000000000001,14.662573362741));
#140972=CARTESIAN_POINT('Origin',(13.5428932188134,-5.50000000000001,14.662573362741));
#140973=CARTESIAN_POINT('',(12.1286796564404,-5.50000000000001,13.2483598003679));
#140974=CARTESIAN_POINT('Origin',(11.4951643931407,-5.5,13.8818750636676));
#140975=CARTESIAN_POINT('',(13.8999999999996,-6.5,11.4770394568086));
#140976=CARTESIAN_POINT('Origin',(13.8999999999996,-7.5,14.3999996781349));
#140977=CARTESIAN_POINT('Origin',(3.56597033699713E-16,-18.2,11.6));
#140978=CARTESIAN_POINT('',(-3.17746460160488,-19.0909089210171,6.83040013131191));
#140979=CARTESIAN_POINT('',(-2.3,-20.5664319132398,8.65129518522849));
#140980=CARTESIAN_POINT('Ctrl Pts',(-3.17746460160488,-19.0909089210171,
6.83040013131191));
#140981=CARTESIAN_POINT('Ctrl Pts',(-3.13315640143359,-19.248936003566,
6.89428549599595));
#140982=CARTESIAN_POINT('Ctrl Pts',(-3.07905321107781,-19.3953385241206,
6.97496500901045));
#140983=CARTESIAN_POINT('Ctrl Pts',(-2.91283443393186,-19.7751825843832,
7.23829491707707));
#140984=CARTESIAN_POINT('Ctrl Pts',(-2.78681144529922,-19.9793063971522,
7.45724834891686));
#140985=CARTESIAN_POINT('Ctrl Pts',(-2.54447355256091,-20.3113748120439,
7.96074874984413));
#140986=CARTESIAN_POINT('Ctrl Pts',(-2.42818675997411,-20.4389117240242,
8.24557800636064));
#140987=CARTESIAN_POINT('Ctrl Pts',(-2.32051730171903,-20.5463637099844,
8.58397368821829));
#140988=CARTESIAN_POINT('Ctrl Pts',(-2.31014109346683,-20.5565755067051,
8.6175231927284));
#140989=CARTESIAN_POINT('Ctrl Pts',(-2.3,-20.5664319132398,8.65129518522849));
#140990=CARTESIAN_POINT('',(-2.3,-20.5664319132398,6.22469676050457));
#140991=CARTESIAN_POINT('Ctrl Pts',(-2.3,-20.5664319132398,6.22469676050457));
#140992=CARTESIAN_POINT('Ctrl Pts',(-2.48457597975064,-20.3870374624419,
6.36499899257086));
#140993=CARTESIAN_POINT('Ctrl Pts',(-2.65218676613499,-20.1805459930308,
6.48360541114717));
#140994=CARTESIAN_POINT('Ctrl Pts',(-2.94119052469523,-19.7229874823135,
6.68052442957258));
#140995=CARTESIAN_POINT('Ctrl Pts',(-3.07628642332023,-19.4360520008276,
6.76703831626945));
#140996=CARTESIAN_POINT('Ctrl Pts',(-3.16994744110375,-19.1173998416605,
6.82570105370662));
#140997=CARTESIAN_POINT('Ctrl Pts',(-3.17374660773455,-19.1041693044674,
6.82807740667823));
#140998=CARTESIAN_POINT('Ctrl Pts',(-3.17746460160488,-19.0909089210171,
6.83040013131191));
#140999=CARTESIAN_POINT('',(-2.3,-20.5664319132398,11.6));
#141000=CARTESIAN_POINT('Origin',(-2.3,-22.8,6.19999999999999));
#141001=CARTESIAN_POINT('',(-2.3,-22.8,8.65129518522849));
#141002=CARTESIAN_POINT('',(-2.3,-10.3,8.65129518522849));
#141003=CARTESIAN_POINT('',(-2.3,-22.8,6.22469676050457));
#141004=CARTESIAN_POINT('',(-2.3,-10.3,6.22469676050457));
#141005=CARTESIAN_POINT('',(-2.3,-22.8,8.2207882501999));
#141006=CARTESIAN_POINT('Origin',(3.04851216033843,-22.8,10.2415765003998));
#141007=CARTESIAN_POINT('',(-3.17746460160488,-22.8,6.8304001313119));
#141008=CARTESIAN_POINT('Origin',(-9.35000000000002,-22.8,-3.05000000003702));
#141009=CARTESIAN_POINT('Origin',(-8.4775012782713,-22.8,10.5062825050979));
#141010=CARTESIAN_POINT('Origin',(-8.4775012782713,-10.3,10.5062825050979));
#141011=CARTESIAN_POINT('',(-3.17746460160488,-10.3,6.83040013131191));
#141012=CARTESIAN_POINT('Origin',(-9.35,-10.3,-3.05000000003699));
#141013=CARTESIAN_POINT('Origin',(-10.7086647932826,-22.8,15.8599643568047));
#141014=CARTESIAN_POINT('',(-10.4009181015562,-6.3,15.1215254807077));
#141015=CARTESIAN_POINT('',(-10.1429793683341,-6.3,15.2942789318548));
#141016=CARTESIAN_POINT('Origin',(-10.7086647932826,-6.3,15.8599643568047));
#141017=CARTESIAN_POINT('',(-10.1429793683341,-15.7,15.2942789318548));
#141018=CARTESIAN_POINT('',(-10.1429793683341,-22.8,15.2942789318548));
#141019=CARTESIAN_POINT('',(-10.4009181015562,-15.7,15.1215254807077));
#141020=CARTESIAN_POINT('Origin',(-10.7086647932826,-15.7,15.8599643568047));
#141021=CARTESIAN_POINT('',(-10.4009181015562,-22.8,15.1215254807077));
#141022=CARTESIAN_POINT('Origin',(-9.46958677130784,-6.3,12.0780860478535));
#141023=CARTESIAN_POINT('',(-13.0927442538679,-6.3,12.4296993284023));
#141024=CARTESIAN_POINT('Origin',(-8.47750127826595,-6.3,10.5062825051013));
#141025=CARTESIAN_POINT('',(-13.2654977050156,-6.3,12.1717605951805));
#141026=CARTESIAN_POINT('Origin',(-13.8311831299642,-6.3,12.7374460201304));
#141027=CARTESIAN_POINT('',(-14.6656854249453,-6.3,10.771572875254));
#141028=CARTESIAN_POINT('',(-11.8753061227997,-6.3,13.5619521773932));
#141029=CARTESIAN_POINT('',(-14.8999999999968,-6.3,10.2058874503057));
#141030=CARTESIAN_POINT('Origin',(-14.0999999999968,-6.3,10.2058874503041));
#141031=CARTESIAN_POINT('',(-14.9000000000043,-6.3,6.20189169841771));
#141032=CARTESIAN_POINT('',(-14.8999999999947,-6.3,11.3076721740337));
#141033=CARTESIAN_POINT('',(-15.0836363636405,-6.3,5.86545927302009));
#141034=CARTESIAN_POINT('Origin',(-15.3000000000043,-6.3,6.20189169841847));
#141035=CARTESIAN_POINT('',(-15.8545454545506,-6.3,5.31964087814201));
#141036=CARTESIAN_POINT('Origin',(-9.35,-6.3,-3.05000000003698));
#141037=CARTESIAN_POINT('',(-16.5000000000054,-6.3,5.63547638297971));
#141038=CARTESIAN_POINT('Origin',(-16.1000000000054,-6.3,5.63547638297895));
#141039=CARTESIAN_POINT('',(-16.4999999999955,-6.3,10.8686291501049));
#141040=CARTESIAN_POINT('',(-16.5000000000028,-6.3,7.01404302392158));
#141041=CARTESIAN_POINT('',(-16.2656854249441,-6.3,11.4343145750533));
#141042=CARTESIAN_POINT('Origin',(-15.6999999999955,-6.3,10.8686291501034));
#141043=CARTESIAN_POINT('',(-9.73431457503237,-6.30000000000001,17.9656854249499));
#141044=CARTESIAN_POINT('',(-11.5745579308,-6.3,16.1254420691865));
#141045=CARTESIAN_POINT('',(-9.16862915008378,-6.30000000000001,18.2));
#141046=CARTESIAN_POINT('Origin',(-9.16862915008378,-6.30000000000001,17.4));
#141047=CARTESIAN_POINT('',(0.550543651061315,-6.30000000000001,18.2));
#141048=CARTESIAN_POINT('',(-4.73479338565392,-6.30000000000001,18.2));
#141049=CARTESIAN_POINT('',(0.748897957688963,-6.30000000000001,17.4526448948953));
#141050=CARTESIAN_POINT('Origin',(0.550543651061315,-6.30000000000001,17.8));
#141051=CARTESIAN_POINT('',(-0.459727007153423,-6.30000000000001,16.7624694423079));
#141052=CARTESIAN_POINT('',(-4.26116725349562,-6.3,14.5916879188221));
#141053=CARTESIAN_POINT('',(-0.755737525613271,-6.30000000000001,16.6));
#141054=CARTESIAN_POINT('Origin',(-5.41858467284464,-6.30000000000001,25.4463470699242));
#141055=CARTESIAN_POINT('',(-8.50588745028793,-6.30000000000001,16.6));
#141056=CARTESIAN_POINT('',(-7.2132001319704,-6.3,16.6));
#141057=CARTESIAN_POINT('',(-9.07157287523651,-6.30000000000001,16.3656854249499));
#141058=CARTESIAN_POINT('Origin',(-8.50588745028793,-6.3,15.8));
#141059=CARTESIAN_POINT('',(-9.32581890600149,-6.3,16.1114393941855));
#141060=CARTESIAN_POINT('Origin',(-8.47750127826595,-22.8,10.5062825051013));
#141061=CARTESIAN_POINT('',(-13.0927442538679,-15.7,12.4296993284023));
#141062=CARTESIAN_POINT('Origin',(-8.47750127826595,-15.7,10.5062825051013));
#141063=CARTESIAN_POINT('',(-13.0927442538679,-22.8,12.4296993284023));
#141064=CARTESIAN_POINT('Origin',(-13.8311831299642,-22.8,12.7374460201304));
#141065=CARTESIAN_POINT('',(-13.2654977050156,-15.7,12.1717605951805));
#141066=CARTESIAN_POINT('Origin',(-13.8311831299642,-15.7,12.7374460201304));
#141067=CARTESIAN_POINT('',(-13.2654977050156,-22.8,12.1717605951805));
#141068=CARTESIAN_POINT('Origin',(-12.3362327337785,-22.8,13.1010255664155));
#141069=CARTESIAN_POINT('',(-14.4917200414815,-15.7,10.9455382587175));
#141070=CARTESIAN_POINT('',(-14.4917200414815,-15.7,10.9455382587175));
#141071=CARTESIAN_POINT('',(-14.4917200414815,-24.,10.9455382587175));
#141072=CARTESIAN_POINT('',(-14.4917200414815,-15.9,10.9455382587175));
#141073=CARTESIAN_POINT('',(-14.6656854249453,-24.,10.771572875254));
#141074=CARTESIAN_POINT('',(-14.5858675678007,-24.,10.8513907323985));
#141075=CARTESIAN_POINT('',(-14.6656854249453,-22.8,10.771572875254));
#141076=CARTESIAN_POINT('Origin',(-8.47750127826595,-24.,10.5062825051013));
#141077=CARTESIAN_POINT('',(-12.344773048718,-24.,7.92428539947466));
#141078=CARTESIAN_POINT('',(-12.6774415881118,-24.4,7.7021781215713));
#141079=CARTESIAN_POINT('Origin',(-12.6774415881118,-24.,7.7021781215713));
#141080=CARTESIAN_POINT('',(-13.5261422614307,-24.4,10.3891320757003));
#141081=CARTESIAN_POINT('Origin',(-8.47750127826595,-24.4,10.5062825051013));
#141082=CARTESIAN_POINT('',(-13.1262499063286,-24.,10.3984113176331));
#141083=CARTESIAN_POINT('Origin',(-13.5261422614307,-24.,10.3891320757003));
#141084=CARTESIAN_POINT('Origin',(-8.47750127826595,-24.,10.5062825051013));
#141085=CARTESIAN_POINT('Ctrl Pts',(-13.1262499063286,-24.,10.3984113176331));
#141086=CARTESIAN_POINT('Ctrl Pts',(-13.138495190793,-24.,10.9261263700982));
#141087=CARTESIAN_POINT('Ctrl Pts',(-13.6284819468181,-24.,11.1224579837266));
#141088=CARTESIAN_POINT('Ctrl Pts',(-14.1184687028432,-24.,11.3187895973549));
#141089=CARTESIAN_POINT('Ctrl Pts',(-14.4917200414815,-24.,10.9455382587175));
#141090=CARTESIAN_POINT('Ctrl Pts',(-13.1262499063286,-24.4,10.3984113176331));
#141091=CARTESIAN_POINT('Ctrl Pts',(-13.138495190793,-24.4,10.9261263700982));
#141092=CARTESIAN_POINT('Ctrl Pts',(-13.6284819468181,-24.4,11.1224579837266));
#141093=CARTESIAN_POINT('Ctrl Pts',(-14.1184687028432,-24.4,11.3187895973549));
#141094=CARTESIAN_POINT('Ctrl Pts',(-14.4917200414815,-24.4,10.9455382587175));
#141095=CARTESIAN_POINT('Ctrl Pts',(-13.5261422614307,-24.4,10.3891320757003));
#141096=CARTESIAN_POINT('Ctrl Pts',(-13.532264903663,-24.4,10.6529896019329));
#141097=CARTESIAN_POINT('Ctrl Pts',(-13.7772582816755,-24.4,10.7511554087471));
#141098=CARTESIAN_POINT('Ctrl Pts',(-14.022251659688,-24.4,10.8493212155613));
#141099=CARTESIAN_POINT('Ctrl Pts',(-14.2088773290072,-24.4,10.6626955462425));
#141100=CARTESIAN_POINT('',(-14.2088773290072,-24.4,10.6626955462425));
#141101=CARTESIAN_POINT('Origin',(-14.2088773290072,-24.,10.6626955462425));
#141102=CARTESIAN_POINT('Origin',(-13.9260346165329,-24.,10.3798528337676));
#141103=CARTESIAN_POINT('Origin',(-13.9260346165329,-24.4,10.3798528337676));
#141104=CARTESIAN_POINT('Origin',(-14.3030248553264,-24.,10.5685480199236));
#141105=CARTESIAN_POINT('',(-14.3828427124711,-24.4,10.4887301627791));
#141106=CARTESIAN_POINT('Origin',(-14.3828427124711,-24.,10.4887301627791));
#141107=CARTESIAN_POINT('',(-14.3030248553264,-24.4,10.5685480199236));
#141108=CARTESIAN_POINT('Ctrl Pts',(-14.6656854249453,-24.,10.771572875254));
#141109=CARTESIAN_POINT('Ctrl Pts',(-14.8999999999965,-24.,10.537258300203));
#141110=CARTESIAN_POINT('Ctrl Pts',(-14.8999999999968,-24.,10.2058874503041));
#141111=CARTESIAN_POINT('Ctrl Pts',(-14.6656854249453,-24.4,10.771572875254));
#141112=CARTESIAN_POINT('Ctrl Pts',(-14.8999999999965,-24.4,10.537258300203));
#141113=CARTESIAN_POINT('Ctrl Pts',(-14.8999999999968,-24.4,10.2058874503041));
#141114=CARTESIAN_POINT('Ctrl Pts',(-14.3828427124711,-24.4,10.4887301627791));
#141115=CARTESIAN_POINT('Ctrl Pts',(-14.4999999999966,-24.4,10.3715728752536));
#141116=CARTESIAN_POINT('Ctrl Pts',(-14.4999999999968,-24.4,10.2058874503041));
#141117=CARTESIAN_POINT('',(-14.4999999999968,-24.4,10.2058874503049));
#141118=CARTESIAN_POINT('',(-14.8999999999968,-24.,10.2058874503056));
#141119=CARTESIAN_POINT('Origin',(-14.4999999999968,-24.,10.2058874503049));
#141120=CARTESIAN_POINT('Origin',(-14.0999999999968,-24.,10.2058874503041));
#141121=CARTESIAN_POINT('Origin',(-14.0999999999968,-24.4,10.2058874503041));
#141122=CARTESIAN_POINT('Origin',(-14.4999999999983,-24.,9.40207938827399));
#141123=CARTESIAN_POINT('',(-14.5000000000022,-24.4,7.31327650886668));
#141124=CARTESIAN_POINT('',(-14.9000000000022,-24.,7.31327650886744));
#141125=CARTESIAN_POINT('Origin',(-14.5000000000022,-24.,7.31327650886668));
#141126=CARTESIAN_POINT('',(-14.8999999999983,-24.,9.40207938827475));
#141127=CARTESIAN_POINT('',(-14.4999999999983,-24.4,9.40207938827399));
#141128=CARTESIAN_POINT('Ctrl Pts',(-14.9000000000022,-24.,7.31327650886593));
#141129=CARTESIAN_POINT('Ctrl Pts',(-14.9000000000026,-24.,6.87608602594433));
#141130=CARTESIAN_POINT('Ctrl Pts',(-14.5320493798966,-24.,6.63997617964215));
#141131=CARTESIAN_POINT('Ctrl Pts',(-14.1640987597902,-24.,6.40386633333922));
#141132=CARTESIAN_POINT('Ctrl Pts',(-13.7666666666687,-24.,6.58602903455695));
#141133=CARTESIAN_POINT('Ctrl Pts',(-14.9000000000022,-24.4,7.31327650886593));
#141134=CARTESIAN_POINT('Ctrl Pts',(-14.9000000000026,-24.4,6.87608602594433));
#141135=CARTESIAN_POINT('Ctrl Pts',(-14.5320493798966,-24.4,6.63997617964215));
#141136=CARTESIAN_POINT('Ctrl Pts',(-14.1640987597902,-24.4,6.40386633333922));
#141137=CARTESIAN_POINT('Ctrl Pts',(-13.7666666666687,-24.4,6.58602903455695));
#141138=CARTESIAN_POINT('Ctrl Pts',(-14.5000000000022,-24.4,7.31327650886593));
#141139=CARTESIAN_POINT('Ctrl Pts',(-14.5000000000024,-24.4,7.09468126740513));
#141140=CARTESIAN_POINT('Ctrl Pts',(-14.3160246899494,-24.4,6.97662634425404));
#141141=CARTESIAN_POINT('Ctrl Pts',(-14.1320493798962,-24.4,6.85857142110258));
#141142=CARTESIAN_POINT('Ctrl Pts',(-13.9333333333355,-24.4,6.94965277171144));
#141143=CARTESIAN_POINT('',(-13.9333333333355,-24.4,6.94965277171144));
#141144=CARTESIAN_POINT('',(-13.7666666666687,-24.,6.58602903455695));
#141145=CARTESIAN_POINT('Origin',(-13.9333333333355,-24.,6.94965277171144));
#141146=CARTESIAN_POINT('Origin',(-14.1000000000022,-24.,7.31327650886593));
#141147=CARTESIAN_POINT('Origin',(-14.1000000000022,-24.4,7.31327650886593));
#141148=CARTESIAN_POINT('Origin',(-9.35,-24.,-3.05000000003699));
#141149=CARTESIAN_POINT('',(-12.7813870032049,-24.4,7.40110440257217));
#141150=CARTESIAN_POINT('',(-12.6566092939974,-24.,7.02106424247729));
#141151=CARTESIAN_POINT('Origin',(-12.7813870032049,-24.,7.40110440257217));
#141152=CARTESIAN_POINT('Origin',(-9.35,-24.,-3.05000000003699));
#141153=CARTESIAN_POINT('Origin',(-9.35,-24.4,-3.05000000003699));
#141154=CARTESIAN_POINT('Ctrl Pts',(-12.6566092939974,-24.,7.02106424247729));
#141155=CARTESIAN_POINT('Ctrl Pts',(-12.3737754104109,-24.,7.11392643912346));
#141156=CARTESIAN_POINT('Ctrl Pts',(-12.2766257747715,-24.,7.39531645594302));
#141157=CARTESIAN_POINT('Ctrl Pts',(-12.1794761391321,-24.,7.67670647276257));
#141158=CARTESIAN_POINT('Ctrl Pts',(-12.344773048718,-24.,7.92428539947466));
#141159=CARTESIAN_POINT('Ctrl Pts',(-12.6566092939974,-24.4,7.02106424247729));
#141160=CARTESIAN_POINT('Ctrl Pts',(-12.3737754104109,-24.4,7.11392643912346));
#141161=CARTESIAN_POINT('Ctrl Pts',(-12.2766257747715,-24.4,7.39531645594302));
#141162=CARTESIAN_POINT('Ctrl Pts',(-12.1794761391321,-24.4,7.67670647276257));
#141163=CARTESIAN_POINT('Ctrl Pts',(-12.344773048718,-24.4,7.92428539947466));
#141164=CARTESIAN_POINT('Ctrl Pts',(-12.7813870032049,-24.4,7.40110440257217));
#141165=CARTESIAN_POINT('Ctrl Pts',(-12.6871090420094,-24.4,7.4320584681209));
#141166=CARTESIAN_POINT('Ctrl Pts',(-12.6547258301296,-24.4,7.52585514039408));
#141167=CARTESIAN_POINT('Ctrl Pts',(-12.6223426182498,-24.4,7.61965181266726));
#141168=CARTESIAN_POINT('Ctrl Pts',(-12.6774415881118,-24.4,7.7021781215713));
#141169=CARTESIAN_POINT('Origin',(-12.8437758578086,-24.,7.59112448261961));
#141170=CARTESIAN_POINT('Origin',(-12.8437758578086,-24.4,7.59112448261961));
#141171=CARTESIAN_POINT('Origin',(-14.1000000000022,-15.9,7.31327650886593));
#141172=CARTESIAN_POINT('',(-13.7666666666687,-15.9,6.58602903455695));
#141173=CARTESIAN_POINT('',(-13.7666666666687,-15.9,6.58602903455696));
#141174=CARTESIAN_POINT('',(-14.9000000000022,-15.9,7.31327650886744));
#141175=CARTESIAN_POINT('Origin',(-14.1000000000022,-15.9,7.31327650886593));
#141176=CARTESIAN_POINT('',(-14.9000000000022,-15.9,7.31327650886744));
#141177=CARTESIAN_POINT('Origin',(-9.35,-15.9,-3.05000000003699));
#141178=CARTESIAN_POINT('',(-12.6566092939974,-15.9,7.02106424247729));
#141179=CARTESIAN_POINT('',(-12.6566092939974,-15.9,7.02106424247729));
#141180=CARTESIAN_POINT('Origin',(-9.35,-15.9,-3.05000000003699));
#141181=CARTESIAN_POINT('Origin',(-12.8437758578086,-15.9,7.59112448261961));
#141182=CARTESIAN_POINT('',(-12.344773048718,-15.9,7.92428539947466));
#141183=CARTESIAN_POINT('',(-12.344773048718,-15.9,7.92428539947466));
#141184=CARTESIAN_POINT('Origin',(-12.8437758578086,-15.9,7.59112448261961));
#141185=CARTESIAN_POINT('Origin',(-8.47750127826595,-15.9,10.5062825051013));
#141186=CARTESIAN_POINT('',(-13.1262499063286,-15.7,10.3984113176331));
#141187=CARTESIAN_POINT('',(-13.1262499063286,-15.9,10.3984113176331));
#141188=CARTESIAN_POINT('',(-11.8432759364864,-15.7,7.29784660110059));
#141189=CARTESIAN_POINT('Origin',(-8.47750127826606,-15.7,10.5062825051013));
#141190=CARTESIAN_POINT('',(-11.8432759364864,-15.9,7.29784660110059));
#141191=CARTESIAN_POINT('',(-11.8432759364864,-15.7,7.29784660110059));
#141192=CARTESIAN_POINT('Origin',(-8.47750127826606,-15.9,10.5062825051013));
#141193=CARTESIAN_POINT('Origin',(-16.5006469797908,-24.4,8.26690047634872));
#141194=CARTESIAN_POINT('Origin',(9.25,-24.,-3.05000000003699));
#141195=CARTESIAN_POINT('',(6.50051930977378,-24.4,-5.37386659131824));
#141196=CARTESIAN_POINT('',(10.822232934276,-24.4,-6.28853108686909));
#141197=CARTESIAN_POINT('Origin',(9.25,-24.4,-3.05000000003699));
#141198=CARTESIAN_POINT('',(10.9969254825289,-24.,-6.64836787429488));
#141199=CARTESIAN_POINT('Origin',(10.822232934276,-24.,-6.28853108686909));
#141200=CARTESIAN_POINT('',(6.10786135295693,-24.,-5.52527063630252));
#141201=CARTESIAN_POINT('Origin',(9.25,-24.,-3.05000000003699));
#141202=CARTESIAN_POINT('Ctrl Pts',(6.10786135295693,-24.,-5.52527063630252));
#141203=CARTESIAN_POINT('Ctrl Pts',(6.10786135295693,-24.0499820482805,
-5.52527063630252));
#141204=CARTESIAN_POINT('Ctrl Pts',(6.11697130800671,-24.0993789543098,
-5.52169964929554));
#141205=CARTESIAN_POINT('Ctrl Pts',(6.15258459790043,-24.1929052251116,
-5.50777794808829));
#141206=CARTESIAN_POINT('Ctrl Pts',(6.17903125593076,-24.2358257575373,
-5.49745098428682));
#141207=CARTESIAN_POINT('Ctrl Pts',(6.24702590778167,-24.310651122957,-5.47102267386603));
#141208=CARTESIAN_POINT('Ctrl Pts',(6.28847953134104,-24.3411725421678,
-5.45496465532731));
#141209=CARTESIAN_POINT('Ctrl Pts',(6.35969905795551,-24.374843044091,-5.42755871292796));
#141210=CARTESIAN_POINT('Ctrl Pts',(6.3863963541329,-24.3840391504725,-5.41731874741856));
#141211=CARTESIAN_POINT('Ctrl Pts',(6.44133303396774,-24.3965469939097,
-5.39633290753587));
#141212=CARTESIAN_POINT('Ctrl Pts',(6.46946853864456,-24.3997869203202,
-5.38562749022657));
#141213=CARTESIAN_POINT('Ctrl Pts',(6.49863348682723,-24.3999966111496,
-5.3745807206615));
#141214=CARTESIAN_POINT('Ctrl Pts',(6.49957638848971,-24.4,-5.37422363275274));
#141215=CARTESIAN_POINT('Ctrl Pts',(6.50051930977378,-24.4,-5.37386659131824));
#141216=CARTESIAN_POINT('Origin',(8.6,-24.,-0.741996797474058));
#141217=CARTESIAN_POINT('',(6.50005584528697,-24.4,-0.726681867288135));
#141218=CARTESIAN_POINT('',(6.5,-24.4,-0.741996797474059));
#141219=CARTESIAN_POINT('Origin',(8.6,-24.4,-0.741996797474058));
#141220=CARTESIAN_POINT('',(6.09999999999987,-24.,-0.741996797474059));
#141221=CARTESIAN_POINT('Origin',(6.5,-24.,-0.741996797474058));
#141222=CARTESIAN_POINT('',(6.10539366127889,-24.,-0.57786509787753));
#141223=CARTESIAN_POINT('Origin',(8.6,-24.,-0.741996797474058));
#141224=CARTESIAN_POINT('Ctrl Pts',(6.10539366127889,-24.,-0.57786509787753));
#141225=CARTESIAN_POINT('Ctrl Pts',(6.10539366127889,-24.0498896942439,
-0.57786509787753));
#141226=CARTESIAN_POINT('Ctrl Pts',(6.11451322581987,-24.0991909205108,
-0.581363208838736));
#141227=CARTESIAN_POINT('Ctrl Pts',(6.15017006506992,-24.1925840562392,
-0.59500177188774));
#141228=CARTESIAN_POINT('Ctrl Pts',(6.17666097503203,-24.2354570848239,
-0.605122847790428));
#141229=CARTESIAN_POINT('Ctrl Pts',(6.24481762949856,-24.3102959529889,
-0.631038317531357));
#141230=CARTESIAN_POINT('Ctrl Pts',(6.286411708346,-24.3408530312395,-0.6467985164514));
#141231=CARTESIAN_POINT('Ctrl Pts',(6.35799432343061,-24.374663196465,-0.673735247695183));
#141232=CARTESIAN_POINT('Ctrl Pts',(6.38491858000175,-24.3839243701463,
-0.683832560852813));
#141233=CARTESIAN_POINT('Ctrl Pts',(6.44032696159033,-24.3965207054082,
-0.704524093670561));
#141234=CARTESIAN_POINT('Ctrl Pts',(6.46870751806677,-24.3997833674192,
-0.715078832732869));
#141235=CARTESIAN_POINT('Ctrl Pts',(6.49813509433547,-24.3999965227155,
-0.725971094000813));
#141236=CARTESIAN_POINT('Ctrl Pts',(6.49909545970173,-24.4,-0.726326505204189));
#141237=CARTESIAN_POINT('Ctrl Pts',(6.50005584528697,-24.4,-0.726681867288135));
#141238=CARTESIAN_POINT('Origin',(6.5,-24.,-0.875559616590781));
#141239=CARTESIAN_POINT('',(6.5,-24.4,-5.32716721908225));
#141240=CARTESIAN_POINT('',(6.09999999999996,-24.,-5.32716721908225));
#141241=CARTESIAN_POINT('Origin',(6.5,-24.,-5.32716721908225));
#141242=CARTESIAN_POINT('',(6.1,-24.,-0.875559616590781));
#141243=CARTESIAN_POINT('',(6.5,-24.4,-0.875559616590781));
#141244=CARTESIAN_POINT('Origin',(8.6,-24.,-5.32716721908225));
#141245=CARTESIAN_POINT('Origin',(8.6,-24.,-5.32716721908225));
#141246=CARTESIAN_POINT('Origin',(8.6,-24.4,-5.32716721908225));
#141247=CARTESIAN_POINT('Origin',(15.1,-24.,-15.1));
#141248=CARTESIAN_POINT('',(14.5000000000093,-24.4,1.88436706275989));
#141249=CARTESIAN_POINT('',(7.67776706572399,-24.4,0.188531086795103));
#141250=CARTESIAN_POINT('Origin',(15.1,-24.4,-15.1));
#141251=CARTESIAN_POINT('',(7.5030745174711,-24.,0.548367874220887));
#141252=CARTESIAN_POINT('Origin',(7.67776706572399,-24.,0.188531086795103));
#141253=CARTESIAN_POINT('',(14.9000000000101,-24.,2.29381194316097));
#141254=CARTESIAN_POINT('Origin',(15.1,-24.,-15.1));
#141255=CARTESIAN_POINT('Ctrl Pts',(14.9000000000101,-24.,2.29381194316097));
#141256=CARTESIAN_POINT('Ctrl Pts',(14.9000000000101,-24.0372063911278,
2.29381194316097));
#141257=CARTESIAN_POINT('Ctrl Pts',(14.8948129067846,-24.0735699191394,
2.28856685120141));
#141258=CARTESIAN_POINT('Ctrl Pts',(14.8740024198881,-24.1476753497927,
2.26749744126914));
#141259=CARTESIAN_POINT('Ctrl Pts',(14.8573938075257,-24.1834986088516,
2.25067154531768));
#141260=CARTESIAN_POINT('Ctrl Pts',(14.8103292966639,-24.2573026498551,
2.20288809341834));
#141261=CARTESIAN_POINT('Ctrl Pts',(14.7773043663909,-24.2916813383689,
2.16928922247749));
#141262=CARTESIAN_POINT('Ctrl Pts',(14.7064030541314,-24.3455212572614,
2.09689931539744));
#141263=CARTESIAN_POINT('Ctrl Pts',(14.6680189554609,-24.3653387142152,
2.05759047151054));
#141264=CARTESIAN_POINT('Ctrl Pts',(14.5877079846584,-24.3926910207608,
1.97503908071189));
#141265=CARTESIAN_POINT('Ctrl Pts',(14.5450918954055,-24.3996912357087,
1.93107222774991));
#141266=CARTESIAN_POINT('Ctrl Pts',(14.5018850095481,-24.3999966689777,
1.88631975494096));
#141267=CARTESIAN_POINT('Ctrl Pts',(14.5009424821723,-24.4,1.88534342752733));
#141268=CARTESIAN_POINT('Ctrl Pts',(14.5000000000093,-24.4,1.88436706275988));
#141269=CARTESIAN_POINT('Origin',(9.25,-24.,-3.05000000003699));
#141270=CARTESIAN_POINT('Origin',(9.25,-24.,-3.05000000003699));
#141271=CARTESIAN_POINT('Origin',(9.25,-24.4,-3.05000000003699));
#141272=CARTESIAN_POINT('Origin',(15.1,-24.,-15.1));
#141273=CARTESIAN_POINT('',(14.899999999995,-24.,-5.70716730244972));
#141274=CARTESIAN_POINT('Origin',(15.1,-24.,-15.1));
#141275=CARTESIAN_POINT('',(14.4999999999957,-24.4,-5.32343232644195));
#141276=CARTESIAN_POINT('Origin',(15.1,-24.4,-15.1));
#141277=CARTESIAN_POINT('Ctrl Pts',(14.4999999999947,-24.4,-5.32343232644195));
#141278=CARTESIAN_POINT('Ctrl Pts',(14.5009421725839,-24.4,-5.32431844938398));
#141279=CARTESIAN_POINT('Ctrl Pts',(14.5018842876012,-24.3999966711656,
-5.32520463865279));
#141280=CARTESIAN_POINT('Ctrl Pts',(14.5439766889831,-24.3996992464686,
-5.36480374024527));
#141281=CARTESIAN_POINT('Ctrl Pts',(14.585204113278,-24.3930574770938,-5.40382483561486));
#141282=CARTESIAN_POINT('Ctrl Pts',(14.6632392768287,-24.3673887589727,
-5.47811640684428));
#141283=CARTESIAN_POINT('Ctrl Pts',(14.7005942801588,-24.3486989590473,
-5.51389178275807));
#141284=CARTESIAN_POINT('Ctrl Pts',(14.7720840023387,-24.2967337204839,
-5.58270349652219));
#141285=CARTESIAN_POINT('Ctrl Pts',(14.8063215119823,-24.2621974509716,
-5.61586680033281));
#141286=CARTESIAN_POINT('Ctrl Pts',(14.8552444363892,-24.1877890402947,
-5.66343415251741));
#141287=CARTESIAN_POINT('Ctrl Pts',(14.8725660409886,-24.1514550547615,
-5.68034270422849));
#141288=CARTESIAN_POINT('Ctrl Pts',(14.8943560092086,-24.0762686187014,
-5.70163858223181));
#141289=CARTESIAN_POINT('Ctrl Pts',(14.8998530362039,-24.0393411392285,
-5.70702343466547));
#141290=CARTESIAN_POINT('Ctrl Pts',(14.899999033164,-24.0010156783502,-5.70716635598636));
#141291=CARTESIAN_POINT('Ctrl Pts',(14.899999999995,-24.0005077614335,-5.70716730244972));
#141292=CARTESIAN_POINT('Ctrl Pts',(14.899999999995,-24.,-5.70716730244972));
#141293=CARTESIAN_POINT('Origin',(14.4999999999963,-24.,-5.02907458701124));
#141294=CARTESIAN_POINT('',(14.8999999999963,-24.,-5.02907458701199));
#141295=CARTESIAN_POINT('',(14.4999999999963,-24.4,-5.02907458701124));
#141296=CARTESIAN_POINT('Origin',(9.25,-23.,-3.05000000003699));
#141297=CARTESIAN_POINT('',(10.9969254825289,-23.,-6.64836787429488));
#141298=CARTESIAN_POINT('',(10.9969254825289,-23.,-6.64836787429488));
#141299=CARTESIAN_POINT('',(6.10786135295693,-23.,-5.52527063630252));
#141300=CARTESIAN_POINT('Origin',(9.25,-23.,-3.05000000003699));
#141301=CARTESIAN_POINT('',(6.10786135295693,-23.,-5.52527063630252));
#141302=CARTESIAN_POINT('Origin',(15.1,-23.,-15.1));
#141303=CARTESIAN_POINT('',(14.899999999995,-23.,-5.70716730244972));
#141304=CARTESIAN_POINT('',(14.899999999995,-23.,-5.70716730244972));
#141305=CARTESIAN_POINT('Origin',(15.1,-23.,-15.1));
#141306=CARTESIAN_POINT('Origin',(14.899999999995,-24.,-5.70716730244972));
#141307=CARTESIAN_POINT('',(14.9000000000101,-23.,2.29381194316097));
#141308=CARTESIAN_POINT('',(14.9000000000101,-23.,2.29381194316097));
#141309=CARTESIAN_POINT('',(14.9000000000101,-23.,2.29381194316097));
#141310=CARTESIAN_POINT('Origin',(15.1,-23.,-15.1));
#141311=CARTESIAN_POINT('',(7.5030745174711,-23.,0.548367874220887));
#141312=CARTESIAN_POINT('',(7.5030745174711,-23.,0.548367874220887));
#141313=CARTESIAN_POINT('Origin',(15.1,-23.,-15.1));
#141314=CARTESIAN_POINT('Origin',(18.4241839371104,-24.4,-4.3509818715809));
#141315=CARTESIAN_POINT('Origin',(9.25,-24.,-3.05000000003698));
#141316=CARTESIAN_POINT('',(2.7,-24.4,6.94499874933762));
#141317=CARTESIAN_POINT('',(2.34026510098007,-24.1749022653573,6.25536451384759));
#141318=CARTESIAN_POINT('Ctrl Pts',(2.69999999999885,-24.4,6.94499874933762));
#141319=CARTESIAN_POINT('Ctrl Pts',(2.69938450726401,-24.4,6.94385951802002));
#141320=CARTESIAN_POINT('Ctrl Pts',(2.69876909427848,-24.3999985793826,
6.94272023953584));
#141321=CARTESIAN_POINT('Ctrl Pts',(2.64677346130994,-24.3997585865573,
6.84644726556242));
#141322=CARTESIAN_POINT('Ctrl Pts',(2.59493609531246,-24.3896208822043,
6.74905244702875));
#141323=CARTESIAN_POINT('Ctrl Pts',(2.49299662506508,-24.3470125596353,
6.55473757267498));
#141324=CARTESIAN_POINT('Ctrl Pts',(2.44575302778059,-24.3139777797754,
6.46307557893406));
#141325=CARTESIAN_POINT('Ctrl Pts',(2.38360876150232,-24.2471543612356,
6.34125351739879));
#141326=CARTESIAN_POINT('Ctrl Pts',(2.36029692449435,-24.2155260551564,
6.2951814529358));
#141327=CARTESIAN_POINT('Ctrl Pts',(2.34093461680916,-24.1762742976837,
6.2566955074144));
#141328=CARTESIAN_POINT('Ctrl Pts',(2.34059937404234,-24.1755897903934,
6.25602908229548));
#141329=CARTESIAN_POINT('Ctrl Pts',(2.34026510098007,-24.1749022653573,
6.2553645138476));
#141330=CARTESIAN_POINT('',(3.60315794694916,-24.4,7.48165109691342));
#141331=CARTESIAN_POINT('Origin',(9.25,-24.4,-3.05000000003698));
#141332=CARTESIAN_POINT('',(3.79217358052409,-24.,7.12912721082302));
#141333=CARTESIAN_POINT('Origin',(3.60315794694916,-24.,7.48165109691342));
#141334=CARTESIAN_POINT('',(2.2595024242038,-24.,6.14431583328021));
#141335=CARTESIAN_POINT('Origin',(9.25,-24.,-3.05000000003698));
#141336=CARTESIAN_POINT('Ctrl Pts',(2.34026510098008,-24.1749022653573,
6.2553645138476));
#141337=CARTESIAN_POINT('Ctrl Pts',(2.3186515458434,-24.1523299103811,6.22564587553467));
#141338=CARTESIAN_POINT('Ctrl Pts',(2.29829947779473,-24.1261400525693,
6.19766178196775));
#141339=CARTESIAN_POINT('Ctrl Pts',(2.27605378247541,-24.081552511153,6.16707395090368));
#141340=CARTESIAN_POINT('Ctrl Pts',(2.26879935823777,-24.0627177020031,
6.15709911757692));
#141341=CARTESIAN_POINT('Ctrl Pts',(2.26159865293807,-24.0317064411739,
6.14719814778983));
#141342=CARTESIAN_POINT('Ctrl Pts',(2.25950242420381,-24.0145787786788,
6.14431583328023));
#141343=CARTESIAN_POINT('Ctrl Pts',(2.2595024242038,-24.,6.14431583328023));
#141344=CARTESIAN_POINT('Ctrl Pts',(3.79217358052409,-24.,7.12912721082302));
#141345=CARTESIAN_POINT('Ctrl Pts',(4.03063238157239,-24.,7.25698362889877));
#141346=CARTESIAN_POINT('Ctrl Pts',(4.09266745560454,-24.,7.52034936894553));
#141347=CARTESIAN_POINT('Ctrl Pts',(4.15470252963669,-24.,7.7837151089923));
#141348=CARTESIAN_POINT('Ctrl Pts',(3.99837965786692,-24.,8.00456126178243));
#141349=CARTESIAN_POINT('Ctrl Pts',(3.79217358052409,-24.4,7.12912721082302));
#141350=CARTESIAN_POINT('Ctrl Pts',(4.03063238157239,-24.4,7.25698362889877));
#141351=CARTESIAN_POINT('Ctrl Pts',(4.09266745560454,-24.4,7.52034936894553));
#141352=CARTESIAN_POINT('Ctrl Pts',(4.15470252963669,-24.4,7.7837151089923));
#141353=CARTESIAN_POINT('Ctrl Pts',(3.99837965786692,-24.4,8.00456126178243));
#141354=CARTESIAN_POINT('Ctrl Pts',(3.60315794694916,-24.4,7.48165109691342));
#141355=CARTESIAN_POINT('Ctrl Pts',(3.68264421396526,-24.4,7.52426990293866));
#141356=CARTESIAN_POINT('Ctrl Pts',(3.70332257197598,-24.4,7.61205848295425));
#141357=CARTESIAN_POINT('Ctrl Pts',(3.7240009299867,-24.4,7.69984706296984));
#141358=CARTESIAN_POINT('Ctrl Pts',(3.67189330606344,-24.4,7.77346244723322));
#141359=CARTESIAN_POINT('',(3.67189330606344,-24.4,7.77346244723322));
#141360=CARTESIAN_POINT('',(3.99837965786692,-24.,8.00456126178243));
#141361=CARTESIAN_POINT('Origin',(3.67189330606344,-24.,7.77346244723322));
#141362=CARTESIAN_POINT('Origin',(3.5086501301617,-24.,7.65791303995861));
#141363=CARTESIAN_POINT('Origin',(3.5086501301617,-24.4,7.65791303995861));
#141364=CARTESIAN_POINT('Origin',(7.1,-24.,10.2));
#141365=CARTESIAN_POINT('',(2.99999999999999,-24.4,11.1110433579144));
#141366=CARTESIAN_POINT('',(2.99999999999999,-24.3874411221899,10.2674423504838));
#141367=CARTESIAN_POINT('Ctrl Pts',(2.99999999999999,-24.4,11.1110433579144));
#141368=CARTESIAN_POINT('Ctrl Pts',(2.99999999999999,-24.4,11.0262276390181));
#141369=CARTESIAN_POINT('Ctrl Pts',(2.99999999999999,-24.3984722201137,
10.9244602435706));
#141370=CARTESIAN_POINT('Ctrl Pts',(2.99999999999999,-24.3933294319036,
10.6618000221546));
#141371=CARTESIAN_POINT('Ctrl Pts',(2.99999999999999,-24.3882215189204,
10.4523039043015));
#141372=CARTESIAN_POINT('Ctrl Pts',(2.99999999999999,-24.3874411221899,
10.2674423504838));
#141373=CARTESIAN_POINT('',(5.0999999999996,-24.4,13.8932370625237));
#141374=CARTESIAN_POINT('Origin',(7.1,-24.4,10.2));
#141375=CARTESIAN_POINT('',(5.4999999999996,-24.,13.6467375879226));
#141376=CARTESIAN_POINT('Ctrl Pts',(5.4999999999996,-24.,13.6467375879226));
#141377=CARTESIAN_POINT('Ctrl Pts',(5.4999999999996,-24.043623376554,13.6467375879226));
#141378=CARTESIAN_POINT('Ctrl Pts',(5.49287202409357,-24.0865043128084,
13.6512950950102));
#141379=CARTESIAN_POINT('Ctrl Pts',(5.46477408706084,-24.170362369205,13.6691611438001));
#141380=CARTESIAN_POINT('Ctrl Pts',(5.4433360290039,-24.2097990038533,13.6827576452369));
#141381=CARTESIAN_POINT('Ctrl Pts',(5.38582695891643,-24.2843713974945,
13.7189116659061));
#141382=CARTESIAN_POINT('Ctrl Pts',(5.34841009281781,-24.3171808215248,
13.7422645921124));
#141383=CARTESIAN_POINT('Ctrl Pts',(5.27605644800346,-24.3610238413703,
13.7868820291226));
#141384=CARTESIAN_POINT('Ctrl Pts',(5.2427453790336,-24.3753624648512,13.8072640754931));
#141385=CARTESIAN_POINT('Ctrl Pts',(5.17389448060471,-24.3947460974665,
13.8490138439509));
#141386=CARTESIAN_POINT('Ctrl Pts',(5.13833439111214,-24.3997525395457,
13.8703923861214));
#141387=CARTESIAN_POINT('Ctrl Pts',(5.10178368010527,-24.3999970171617,
13.8921744392635));
#141388=CARTESIAN_POINT('Ctrl Pts',(5.10089186521198,-24.4,13.8927057932241));
#141389=CARTESIAN_POINT('Ctrl Pts',(5.0999999999996,-24.4,13.8932370625237));
#141390=CARTESIAN_POINT('Origin',(7.1,-24.,10.2));
#141391=CARTESIAN_POINT('',(2.92511356012264,-24.4,9.74138991056875));
#141392=CARTESIAN_POINT('Origin',(7.1,-24.4,10.2));
#141393=CARTESIAN_POINT('Ctrl Pts',(2.99999999999999,-24.3874411221899,
10.2674423504838));
#141394=CARTESIAN_POINT('Ctrl Pts',(2.96910221504019,-24.3946244822332,
10.0906889153863));
#141395=CARTESIAN_POINT('Ctrl Pts',(2.94468295018221,-24.3998756487825,
9.91725158038943));
#141396=CARTESIAN_POINT('Ctrl Pts',(2.92555818538903,-24.3999992746164,
9.74540441364033));
#141397=CARTESIAN_POINT('Ctrl Pts',(2.9253355193279,-24.4,9.74339719961947));
#141398=CARTESIAN_POINT('Ctrl Pts',(2.92511356012264,-24.4,9.74138991056876));
#141399=CARTESIAN_POINT('Origin',(9.25,-10.3,-3.05000000003698));
#141400=CARTESIAN_POINT('',(3.79217358052409,-19.450790764769,7.12912721082303));
#141401=CARTESIAN_POINT('',(3.79217358052409,-10.3,7.12912721082302));
#141402=CARTESIAN_POINT('',(4.20575266919785,-19.0059957824439,7.34028723688267));
#141403=CARTESIAN_POINT('Ctrl Pts',(3.79217358052409,-19.450790764769,7.12912721082303));
#141404=CARTESIAN_POINT('Ctrl Pts',(3.92894707189985,-19.3006588374492,
7.20246217945552));
#141405=CARTESIAN_POINT('Ctrl Pts',(4.06689863056173,-19.152147384955,7.27287676999272));
#141406=CARTESIAN_POINT('Ctrl Pts',(4.20575266919785,-19.0059957824439,
7.34028723688266));
#141407=CARTESIAN_POINT('',(4.20575266919785,-10.8312625177592,7.34028723688267));
#141408=CARTESIAN_POINT('',(4.20575266919785,-10.3,7.34028723688267));
#141409=CARTESIAN_POINT('',(3.96202237101811,-10.5713843344211,7.218388023182));
#141410=CARTESIAN_POINT('Ctrl Pts',(3.96202237101812,-10.5713843344211,
7.218388023182));
#141411=CARTESIAN_POINT('Ctrl Pts',(4.04291734656614,-10.658723483699,7.26004702749969));
#141412=CARTESIAN_POINT('Ctrl Pts',(4.12417858841689,-10.7454012583632,
7.30068488231253));
#141413=CARTESIAN_POINT('Ctrl Pts',(4.20575266919785,-10.8312625177592,
7.34028723688266));
#141414=CARTESIAN_POINT('',(3.96202237101811,-10.3,7.218388023182));
#141415=CARTESIAN_POINT('',(3.96202237101811,-10.3,7.218388023182));
#141416=CARTESIAN_POINT('',(0.753380028274003,-10.3,4.77367874183802));
#141417=CARTESIAN_POINT('Origin',(9.25,-10.3,-3.05000000003698));
#141418=CARTESIAN_POINT('',(0.753380028239878,-16.1330170457644,4.77367874180096));
#141419=CARTESIAN_POINT('',(0.753380028274003,-10.3,4.77367874183802));
#141420=CARTESIAN_POINT('',(1.06586901379278,-16.2754420649312,5.09999999999999));
#141421=CARTESIAN_POINT('Ctrl Pts',(0.753380028237917,-16.1330170457761,
4.77367874179883));
#141422=CARTESIAN_POINT('Ctrl Pts',(0.827841722403025,-16.1601570631323,
4.85454513964712));
#141423=CARTESIAN_POINT('Ctrl Pts',(0.902862648270401,-16.1920729653029,
4.9336847969506));
#141424=CARTESIAN_POINT('Ctrl Pts',(1.00701139399119,-16.2437237651945,
5.04057678208364));
#141425=CARTESIAN_POINT('Ctrl Pts',(1.03650440201479,-16.2591791978977,
5.07051241360133));
#141426=CARTESIAN_POINT('Ctrl Pts',(1.06586901379278,-16.2754420649312,
5.09999999999999));
#141427=CARTESIAN_POINT('',(2.33335341373322,-15.866448662099,6.19999999999999));
#141428=CARTESIAN_POINT('Ctrl Pts',(1.06586901379278,-16.2754420649312,
5.09999999999999));
#141429=CARTESIAN_POINT('Ctrl Pts',(1.08669238122262,-16.2630712876422,
5.12091057259128));
#141430=CARTESIAN_POINT('Ctrl Pts',(1.10765038033297,-16.25092019906,5.14179603489229));
#141431=CARTESIAN_POINT('Ctrl Pts',(1.497746484828,-16.0303633776365,5.52755122732));
#141432=CARTESIAN_POINT('Ctrl Pts',(1.90762157781984,-15.8909333123056,
5.88166090275419));
#141433=CARTESIAN_POINT('Ctrl Pts',(2.33335341373322,-15.866448662099,6.19999999999999));
#141434=CARTESIAN_POINT('',(2.33335341373322,-20.533551337901,6.19999999999999));
#141435=CARTESIAN_POINT('Ctrl Pts',(2.33335341373322,-15.866448662099,6.19999999999999));
#141436=CARTESIAN_POINT('Ctrl Pts',(2.50458376491819,-16.0376644900874,
6.328036737728));
#141437=CARTESIAN_POINT('Ctrl Pts',(2.6600024453182,-16.2320241427132,6.43676776431048));
#141438=CARTESIAN_POINT('Ctrl Pts',(2.94074307716937,-16.6760756161761,
6.62621602757801));
#141439=CARTESIAN_POINT('Ctrl Pts',(3.07603900473761,-16.9632728375209,
6.71196137328473));
#141440=CARTESIAN_POINT('Ctrl Pts',(3.25582314080075,-17.5745988720813,
6.82337466030348));
#141441=CARTESIAN_POINT('Ctrl Pts',(3.3,-17.8987366888933,6.84949493657468));
#141442=CARTESIAN_POINT('Ctrl Pts',(3.3,-18.5012633111067,6.84949493657468));
#141443=CARTESIAN_POINT('Ctrl Pts',(3.25582314080075,-18.8254011279188,
6.82337466030348));
#141444=CARTESIAN_POINT('Ctrl Pts',(3.07603900473761,-19.4367271624791,
6.71196137328473));
#141445=CARTESIAN_POINT('Ctrl Pts',(2.94074307716937,-19.7239243838239,
6.62621602757801));
#141446=CARTESIAN_POINT('Ctrl Pts',(2.6600024453182,-20.1679758572868,6.43676776431048));
#141447=CARTESIAN_POINT('Ctrl Pts',(2.50458376491819,-20.3623355099126,
6.328036737728));
#141448=CARTESIAN_POINT('Ctrl Pts',(2.33335341373322,-20.533551337901,6.19999999999999));
#141449=CARTESIAN_POINT('',(2.2595024242038,-20.5281396051547,6.14431583328021));
#141450=CARTESIAN_POINT('Ctrl Pts',(2.33335341373322,-20.533551337901,6.19999999999999));
#141451=CARTESIAN_POINT('Ctrl Pts',(2.30868348710064,-20.5321325233486,
6.18155317147826));
#141452=CARTESIAN_POINT('Ctrl Pts',(2.28406566649289,-20.530325389613,6.16299142467695));
#141453=CARTESIAN_POINT('Ctrl Pts',(2.2595024242038,-20.5281396051547,6.14431583328021));
#141454=CARTESIAN_POINT('',(2.2595024242038,-10.3,6.14431583328021));
#141455=CARTESIAN_POINT('Origin',(3.5086501301617,-10.3,7.65791303995861));
#141456=CARTESIAN_POINT('',(3.99837965786692,-18.7372583002031,8.00456126178243));
#141457=CARTESIAN_POINT('',(3.99837965786692,-10.3,8.00456126178243));
#141458=CARTESIAN_POINT('Ctrl Pts',(3.99837965786692,-18.7372583002031,
8.00456126178243));
#141459=CARTESIAN_POINT('Ctrl Pts',(4.03732967732535,-18.7372583002031,
7.94953436871739));
#141460=CARTESIAN_POINT('Ctrl Pts',(4.06767008908906,-18.7513211403521,
7.88573623665628));
#141461=CARTESIAN_POINT('Ctrl Pts',(4.10395213346578,-18.8019424520368,
7.75802399444114));
#141462=CARTESIAN_POINT('Ctrl Pts',(4.11016145474904,-18.8381784329961,
7.69405845595038));
#141463=CARTESIAN_POINT('Ctrl Pts',(4.10559496170999,-18.9320481917235,
7.5550706062975));
#141464=CARTESIAN_POINT('Ctrl Pts',(4.0852693413741,-19.0015084112899,7.47411890040826));
#141465=CARTESIAN_POINT('Ctrl Pts',(4.01784669559515,-19.1480722446802,
7.33082157667108));
#141466=CARTESIAN_POINT('Ctrl Pts',(3.97063386025383,-19.2251902002209,
7.26854514914513));
#141467=CARTESIAN_POINT('Ctrl Pts',(3.88247112583277,-19.3459928754066,
7.18595811268406));
#141468=CARTESIAN_POINT('Ctrl Pts',(3.83978846512759,-19.3985254147898,
7.15465727541167));
#141469=CARTESIAN_POINT('Ctrl Pts',(3.79217358052409,-19.450790764769,7.12912721082302));
#141470=CARTESIAN_POINT('Origin',(7.1,-24.4,10.2));
#141471=CARTESIAN_POINT('',(5.4999999999996,-18.7372583002031,13.6467375879226));
#141472=CARTESIAN_POINT('',(5.4999999999996,-24.4,13.6467375879226));
#141473=CARTESIAN_POINT('',(5.32295533693765,-18.7372583001967,13.5588855689756));
#141474=CARTESIAN_POINT('Origin',(7.1,-18.7372583002031,10.2));
#141475=CARTESIAN_POINT('',(3.43393944403533,-22.3025065380446,11.2));
#141476=CARTESIAN_POINT('Ctrl Pts',(5.32295533692251,-18.7372583001948,
13.5588855689689));
#141477=CARTESIAN_POINT('Ctrl Pts',(5.31543781191846,-18.8117391408375,
13.5549083636091));
#141478=CARTESIAN_POINT('Ctrl Pts',(5.30636187833369,-18.88600809146,13.5500757822301));
#141479=CARTESIAN_POINT('Ctrl Pts',(5.24790374924743,-19.2933639529239,
13.5185380397245));
#141480=CARTESIAN_POINT('Ctrl Pts',(5.16846423487534,-19.6208923989795,
13.4749524190562));
#141481=CARTESIAN_POINT('Ctrl Pts',(4.92922830421624,-20.319228523667,13.3228547377802));
#141482=CARTESIAN_POINT('Ctrl Pts',(4.75571610594006,-20.6793655488159,
13.2024143398389));
#141483=CARTESIAN_POINT('Ctrl Pts',(4.55878273226527,-21.,13.0252813661947));
#141484=CARTESIAN_POINT('Ctrl Pts',(4.41276324398597,-21.2377396863364,
12.8939432101154));
#141485=CARTESIAN_POINT('Ctrl Pts',(4.24917117087481,-21.4582044314781,
12.7230082485295));
#141486=CARTESIAN_POINT('Ctrl Pts',(3.8930603371699,-21.8849218960272,12.2680071579846));
#141487=CARTESIAN_POINT('Ctrl Pts',(3.67726565735291,-22.0909313543125,
11.9071305384491));
#141488=CARTESIAN_POINT('Ctrl Pts',(3.49330913993195,-22.2523441140072,
11.4010209787851));
#141489=CARTESIAN_POINT('Ctrl Pts',(3.46159216327806,-22.2793602584562,
11.301376543281));
#141490=CARTESIAN_POINT('Ctrl Pts',(3.43393944403533,-22.3025065380446,
11.2));
#141491=CARTESIAN_POINT('',(3.40807692379814,-18.7372583002031,9.30016445979934));
#141492=CARTESIAN_POINT('Ctrl Pts',(3.43393944403533,-22.3025065380446,
11.2));
#141493=CARTESIAN_POINT('Ctrl Pts',(3.38538330748545,-22.1110106189331,
11.0219902630444));
#141494=CARTESIAN_POINT('Ctrl Pts',(3.35318020866045,-21.9134486134528,
10.8519898266241));
#141495=CARTESIAN_POINT('Ctrl Pts',(3.31274055197059,-21.5315989463264,
10.546834566985));
#141496=CARTESIAN_POINT('Ctrl Pts',(3.30151522006465,-21.2950143493326,
10.3728117862555));
#141497=CARTESIAN_POINT('Ctrl Pts',(3.29999012118781,-21.0613145694522,
10.2176726278714));
#141498=CARTESIAN_POINT('Ctrl Pts',(3.29994830585796,-21.0309600750686,
10.1978078267685));
#141499=CARTESIAN_POINT('Ctrl Pts',(3.30006446200803,-21.,10.1778661547474));
#141500=CARTESIAN_POINT('Ctrl Pts',(3.30178228928965,-20.5421330548263,
9.88294980103293));
#141501=CARTESIAN_POINT('Ctrl Pts',(3.33837991246433,-20.0541154947359,
9.63659924188226));
#141502=CARTESIAN_POINT('Ctrl Pts',(3.38373137758155,-19.3064142028621,
9.40336523861826));
#141503=CARTESIAN_POINT('Ctrl Pts',(3.39632541877288,-19.0737391684594,
9.34905336737836));
#141504=CARTESIAN_POINT('Ctrl Pts',(3.4059639616169,-18.8035071049694,9.30886402172908));
#141505=CARTESIAN_POINT('Ctrl Pts',(3.40706313605649,-18.7704004107024,
9.30432391582275));
#141506=CARTESIAN_POINT('Ctrl Pts',(3.40807692379814,-18.7372583002031,
9.30016445979934));
#141507=CARTESIAN_POINT('Origin',(7.1,-18.7372583002031,10.2));
#141508=CARTESIAN_POINT('Origin',(5.09999999999967,-24.,10.2414572515418));
#141509=CARTESIAN_POINT('',(5.09999999999956,-24.4,16.));
#141510=CARTESIAN_POINT('',(5.09999999999967,-24.4,10.2414572515418));
#141511=CARTESIAN_POINT('',(5.49999999999956,-24.,16.));
#141512=CARTESIAN_POINT('Origin',(5.09999999999956,-24.,16.));
#141513=CARTESIAN_POINT('',(5.49999999999967,-24.,10.2414572515418));
#141514=CARTESIAN_POINT('Origin',(3.04851216033843,-24.4,10.2415765003998));
#141515=CARTESIAN_POINT('',(2.99999999999999,-24.4,16.2));
#141516=CARTESIAN_POINT('',(2.99999999999999,-24.4,14.2207882501964));
#141517=CARTESIAN_POINT('',(4.89999999999956,-24.4,16.2));
#141518=CARTESIAN_POINT('',(-0.954150666147262,-24.4,16.2));
#141519=CARTESIAN_POINT('Origin',(4.89999999999956,-24.4,16.));
#141520=CARTESIAN_POINT('Origin',(2.99999999999999,-22.8,18.199999999993));
#141521=CARTESIAN_POINT('',(2.99999999999999,-24.,11.1958530281318));
#141522=CARTESIAN_POINT('Origin',(2.99999999999999,-24.,9.96025655312461));
#141523=CARTESIAN_POINT('',(2.99999999999999,-22.6247197197547,11.1958530281318));
#141524=CARTESIAN_POINT('',(2.99999999999999,-22.8,11.1958530281318));
#141525=CARTESIAN_POINT('',(2.99999999999999,-22.6297291113566,11.2));
#141526=CARTESIAN_POINT('Ctrl Pts',(2.99999999999999,-22.6297291113566,
11.2));
#141527=CARTESIAN_POINT('Ctrl Pts',(2.99999999999999,-22.6272234444407,
11.1979253409942));
#141528=CARTESIAN_POINT('Ctrl Pts',(2.99999999999999,-22.6247197197547,
11.1958530281318));
#141529=CARTESIAN_POINT('',(3.00000000000928,-22.629729097456,14.395853022084));
#141530=CARTESIAN_POINT('',(2.99999999999999,-22.6297291113566,11.6));
#141531=CARTESIAN_POINT('',(2.99999999999999,-21.2805843601499,16.3958530281318));
#141532=CARTESIAN_POINT('Ctrl Pts',(2.99999999999999,-21.2805843601499,
16.3958530281318));
#141533=CARTESIAN_POINT('Ctrl Pts',(2.99999999999999,-21.8817576684837,
15.5754919688216));
#141534=CARTESIAN_POINT('Ctrl Pts',(2.99999999999999,-22.6297291101028,
14.3958530301092));
#141535=CARTESIAN_POINT('',(2.99999999999999,-21.7512078069108,16.6));
#141536=CARTESIAN_POINT('Ctrl Pts',(2.99999999999999,-21.2805843601499,
16.3958530281318));
#141537=CARTESIAN_POINT('Ctrl Pts',(2.99999999999999,-21.3068354153031,
16.4293435697378));
#141538=CARTESIAN_POINT('Ctrl Pts',(2.99999999999999,-21.3399515768309,
16.4595872648773));
#141539=CARTESIAN_POINT('Ctrl Pts',(2.99999999999999,-21.4209067702055,
16.5184033153281));
#141540=CARTESIAN_POINT('Ctrl Pts',(2.99999999999999,-21.4862885611465,
16.549963078009));
#141541=CARTESIAN_POINT('Ctrl Pts',(2.99999999999999,-21.6069095263048,
16.5880803850168));
#141542=CARTESIAN_POINT('Ctrl Pts',(2.99999999999999,-21.6852076397025,
16.6));
#141543=CARTESIAN_POINT('Ctrl Pts',(2.99999999999999,-21.7512078069108,
16.6));
#141544=CARTESIAN_POINT('',(2.99999999999999,-24.,16.6));
#141545=CARTESIAN_POINT('',(2.99999999999999,-16.55,16.6));
#141546=CARTESIAN_POINT('Origin',(3.,-24.,16.2));
#141547=CARTESIAN_POINT('Ctrl Pts',(5.49999999999956,-24.,16.));
#141548=CARTESIAN_POINT('Ctrl Pts',(5.49999999999955,-24.,16.6));
#141549=CARTESIAN_POINT('Ctrl Pts',(4.89999999999956,-24.,16.6));
#141550=CARTESIAN_POINT('Ctrl Pts',(5.49999999999956,-24.4,16.));
#141551=CARTESIAN_POINT('Ctrl Pts',(5.49999999999955,-24.4,16.6));
#141552=CARTESIAN_POINT('Ctrl Pts',(4.89999999999956,-24.4,16.6));
#141553=CARTESIAN_POINT('Ctrl Pts',(5.09999999999956,-24.4,16.));
#141554=CARTESIAN_POINT('Ctrl Pts',(5.09999999999956,-24.4,16.2));
#141555=CARTESIAN_POINT('Ctrl Pts',(4.89999999999956,-24.4,16.2));
#141556=CARTESIAN_POINT('',(4.89999999999956,-24.,16.6));
#141557=CARTESIAN_POINT('Origin',(4.89999999999956,-24.,16.2));
#141558=CARTESIAN_POINT('Origin',(4.89999999999956,-24.,16.));
#141559=CARTESIAN_POINT('Origin',(-0.954150666147262,-24.,16.2));
#141560=CARTESIAN_POINT('',(-0.954150666147262,-24.,16.6));
#141561=CARTESIAN_POINT('Origin',(5.49999999999967,-16.5524667901538,10.2413380026838));
#141562=CARTESIAN_POINT('',(5.49999999999956,-12.5846724700528,16.));
#141563=CARTESIAN_POINT('',(5.49999999999956,-13.4262333950769,16.));
#141564=CARTESIAN_POINT('',(5.49999999999956,-12.5535531013342,15.9538461538416));
#141565=CARTESIAN_POINT('Origin',(5.49999999999956,-12.238262308539,16.1999999999999));
#141566=CARTESIAN_POINT('',(5.49999999999963,-12.5141521334422,12.4978250586149));
#141567=CARTESIAN_POINT('Origin',(5.49999999999959,-14.8,14.199999999963));
#141568=CARTESIAN_POINT('',(5.4999999999996,-17.7372583002031,12.4978250586149));
#141569=CARTESIAN_POINT('',(5.4999999999996,-24.4,12.4978250586149));
#141570=CARTESIAN_POINT('Ctrl Pts',(5.4999999999996,-18.737258300203,13.6467375879226));
#141571=CARTESIAN_POINT('Ctrl Pts',(5.49999999999962,-18.1372583002031,
12.985242495291));
#141572=CARTESIAN_POINT('Ctrl Pts',(5.49999999999962,-17.7372583002032,
12.4978250586151));
#141573=CARTESIAN_POINT('',(5.49999999999962,-14.8,12.549999999963));
#141574=CARTESIAN_POINT('Origin',(5.49999999999959,-14.8,14.199999999963));
#141575=CARTESIAN_POINT('Origin',(4.89999999999956,-13.4262333950769,16.));
#141576=CARTESIAN_POINT('',(4.89999999999956,-12.238262308539,16.6));
#141577=CARTESIAN_POINT('',(4.89999999999956,-13.4262333950769,16.6));
#141578=CARTESIAN_POINT('Ctrl Pts',(5.49999999999956,-12.5846724700528,
16.));
#141579=CARTESIAN_POINT('Ctrl Pts',(5.49999999999956,-12.5940887807114,
16.0163095284805));
#141580=CARTESIAN_POINT('Ctrl Pts',(5.49932802856564,-12.6023867107517,
16.0333635630483));
#141581=CARTESIAN_POINT('Ctrl Pts',(5.49367232615558,-12.629123862268,16.0998863384286));
#141582=CARTESIAN_POINT('Ctrl Pts',(5.48249827863786,-12.638262308539,16.1524460685814));
#141583=CARTESIAN_POINT('Ctrl Pts',(5.44738870998965,-12.638262308539,16.2517509248842));
#141584=CARTESIAN_POINT('Ctrl Pts',(5.42063930011652,-12.6277423449409,
16.3033655674568));
#141585=CARTESIAN_POINT('Ctrl Pts',(5.35597524083088,-12.5914895471395,
16.3939321009808));
#141586=CARTESIAN_POINT('Ctrl Pts',(5.31811815076933,-12.56591478853,16.4329882568349));
#141587=CARTESIAN_POINT('Ctrl Pts',(5.22634454907965,-12.4998649350384,
16.5084457181327));
#141588=CARTESIAN_POINT('Ctrl Pts',(5.16276007011936,-12.4504558640288,
16.5438950744375));
#141589=CARTESIAN_POINT('Ctrl Pts',(5.03098863695038,-12.3452667223669,
16.5896665496838));
#141590=CARTESIAN_POINT('Ctrl Pts',(4.96277844627394,-12.289520695278,16.5999999999999));
#141591=CARTESIAN_POINT('Ctrl Pts',(4.89999999999955,-12.238262308539,16.5999999999999));
#141592=CARTESIAN_POINT('Origin',(-4.95681349263295,-10.3,16.6));
#141593=CARTESIAN_POINT('',(-3.65042002992564,-15.3215437309242,16.6));
#141594=CARTESIAN_POINT('Origin',(1.12776416393948E-15,-18.2,16.6));
#141595=CARTESIAN_POINT('',(-3.65042002992564,-10.3,16.6));
#141596=CARTESIAN_POINT('',(-3.65042002992564,-10.3,16.6));
#141597=CARTESIAN_POINT('',(-7.62176460923847,-10.3,16.6));
#141598=CARTESIAN_POINT('',(-1.35407769578341,-10.3,16.6));
#141599=CARTESIAN_POINT('',(-7.62176460923847,-15.7,16.6));
#141600=CARTESIAN_POINT('',(-7.62176460923847,-10.3,16.6));
#141601=CARTESIAN_POINT('',(-8.50588745028793,-15.7,16.6));
#141602=CARTESIAN_POINT('',(-8.50588745028793,-15.7,16.6));
#141603=CARTESIAN_POINT('',(-8.50588745028793,-16.55,16.6));
#141604=CARTESIAN_POINT('',(-0.755737525613271,-10.3,16.6));
#141605=CARTESIAN_POINT('',(-0.755737525613271,-21.1,16.6));
#141606=CARTESIAN_POINT('',(10.8999999999996,-10.3,16.6));
#141607=CARTESIAN_POINT('',(7.27432905053284,-10.3,16.6));
#141608=CARTESIAN_POINT('',(10.8999999999996,-11.8066740906056,16.6));
#141609=CARTESIAN_POINT('',(10.8999999999996,-10.3,16.6));
#141610=CARTESIAN_POINT('',(8.28666521865374,-11.8066740906056,16.6));
#141611=CARTESIAN_POINT('',(13.8999999999996,-11.8066740906056,16.6));
#141612=CARTESIAN_POINT('',(7.96034186369749,-12.238262308539,16.6));
#141613=CARTESIAN_POINT('Ctrl Pts',(8.28666521865374,-11.8066740906056,
16.6));
#141614=CARTESIAN_POINT('Ctrl Pts',(8.1108270602786,-12.0320528721918,16.6));
#141615=CARTESIAN_POINT('Ctrl Pts',(7.96034186369749,-12.238262308539,16.6));
#141616=CARTESIAN_POINT('',(8.49999999999956,-12.238262308539,16.6));
#141617=CARTESIAN_POINT('Origin',(3.234855708905,-24.,10.646656929178));
#141618=CARTESIAN_POINT('',(2.7,-24.4,9.08346239821099));
#141619=CARTESIAN_POINT('',(3.234855708905,-24.4,10.646656929178));
#141620=CARTESIAN_POINT('',(2.3,-24.,9.14999999999999));
#141621=CARTESIAN_POINT('Origin',(2.7,-24.,9.08346239821099));
#141622=CARTESIAN_POINT('',(2.85639594574927,-24.,10.776149043502));
#141623=CARTESIAN_POINT('Origin',(2.7,-24.,9.6957882501999));
#141624=CARTESIAN_POINT('',(2.3,-24.,6.19999999999999));
#141625=CARTESIAN_POINT('Origin',(2.7,-24.,6.74999999999999));
#141626=CARTESIAN_POINT('',(2.3,-24.,9.6957882501999));
#141627=CARTESIAN_POINT('',(2.7,-24.4,9.6957882501999));
#141628=CARTESIAN_POINT('Origin',(2.99999999999999,-22.8,11.1958530281318));
#141629=CARTESIAN_POINT('',(2.3,-20.5664319132398,9.14999999999999));
#141630=CARTESIAN_POINT('',(2.3,-22.8,9.14999999999999));
#141631=CARTESIAN_POINT('Ctrl Pts',(2.99999999999999,-22.6247197197547,
11.1958530281318));
#141632=CARTESIAN_POINT('Ctrl Pts',(2.54392068220353,-21.3234927580979,
9.86289409472867));
#141633=CARTESIAN_POINT('Ctrl Pts',(2.3,-20.5664319132398,9.14999999999999));
#141634=CARTESIAN_POINT('Origin',(2.3,-22.8,9.14999999999999));
#141635=CARTESIAN_POINT('',(2.3,-20.5664319132398,6.19999999999997));
#141636=CARTESIAN_POINT('',(2.3,-22.8,6.19999999999999));
#141637=CARTESIAN_POINT('',(2.3,-20.5664319132399,11.6));
#141638=CARTESIAN_POINT('Origin',(7.1,-24.,10.2));
#141639=CARTESIAN_POINT('',(11.0937451095552,-24.4,11.499999999963));
#141640=CARTESIAN_POINT('',(11.2999891909638,-24.4,10.1904713176424));
#141641=CARTESIAN_POINT('Origin',(7.1,-24.4,10.2));
#141642=CARTESIAN_POINT('',(10.8999902203958,-24.,10.1913788112003));
#141643=CARTESIAN_POINT('Origin',(11.2999891909638,-24.,10.1904713176424));
#141644=CARTESIAN_POINT('',(10.4985290936118,-24.,11.899999999963));
#141645=CARTESIAN_POINT('Origin',(7.1,-24.,10.2));
#141646=CARTESIAN_POINT('Ctrl Pts',(11.0937451095552,-24.4,11.499999999963));
#141647=CARTESIAN_POINT('Ctrl Pts',(11.0924567483356,-24.4,11.5009355247485));
#141648=CARTESIAN_POINT('Ctrl Pts',(11.0911681658151,-24.3999967179757,
11.5018707575305));
#141649=CARTESIAN_POINT('Ctrl Pts',(11.0231542191183,-24.3996506319442,
11.5512102927633));
#141650=CARTESIAN_POINT('Ctrl Pts',(10.9549864097868,-24.3905292179535,
11.5994056955316));
#141651=CARTESIAN_POINT('Ctrl Pts',(10.8262909213129,-24.3560435733156,
11.6880601135325));
#141652=CARTESIAN_POINT('Ctrl Pts',(10.7632529694956,-24.3309943848462,
11.730357597492));
#141653=CARTESIAN_POINT('Ctrl Pts',(10.6545605129792,-24.2665454594411,
11.8016069437028));
#141654=CARTESIAN_POINT('Ctrl Pts',(10.6108433428765,-24.2311087701909,
11.8295581358754));
#141655=CARTESIAN_POINT('Ctrl Pts',(10.5541231913578,-24.1654279391003,
11.8654132910912));
#141656=CARTESIAN_POINT('Ctrl Pts',(10.5340339349874,-24.1354346237366,
11.8779647727759));
#141657=CARTESIAN_POINT('Ctrl Pts',(10.5089740421432,-24.0763110214604,
11.8935467247689));
#141658=CARTESIAN_POINT('Ctrl Pts',(10.5017642773951,-24.049084401109,11.8980004953156));
#141659=CARTESIAN_POINT('Ctrl Pts',(10.4988131157112,-24.0137087622167,
11.8998245213102));
#141660=CARTESIAN_POINT('Ctrl Pts',(10.4985290936118,-24.006841140788,11.899999999963));
#141661=CARTESIAN_POINT('Ctrl Pts',(10.4985290936118,-24.,11.899999999963));
#141662=CARTESIAN_POINT('Ctrl Pts',(10.8999902203958,-24.,10.1913788112003));
#141663=CARTESIAN_POINT('Ctrl Pts',(10.8993682056462,-24.,9.91721128970292));
#141664=CARTESIAN_POINT('Ctrl Pts',(11.1062409847674,-24.,9.73728944554553));
#141665=CARTESIAN_POINT('Ctrl Pts',(11.3131137638887,-24.,9.55736760138814));
#141666=CARTESIAN_POINT('Ctrl Pts',(11.5845457335763,-24.,9.59600569888118));
#141667=CARTESIAN_POINT('Ctrl Pts',(10.8999902203958,-24.4,10.1913788112003));
#141668=CARTESIAN_POINT('Ctrl Pts',(10.8993682056462,-24.4,9.91721128970292));
#141669=CARTESIAN_POINT('Ctrl Pts',(11.1062409847674,-24.4,9.73728944554553));
#141670=CARTESIAN_POINT('Ctrl Pts',(11.3131137638887,-24.4,9.55736760138814));
#141671=CARTESIAN_POINT('Ctrl Pts',(11.5845457335763,-24.4,9.59600569888118));
#141672=CARTESIAN_POINT('Ctrl Pts',(11.2999891909638,-24.4,10.1904713176424));
#141673=CARTESIAN_POINT('Ctrl Pts',(11.2997818527139,-24.4,10.09908214381));
#141674=CARTESIAN_POINT('Ctrl Pts',(11.3687394457543,-24.4,10.0391081957575));
#141675=CARTESIAN_POINT('Ctrl Pts',(11.4376970387948,-24.4,9.97913424770505));
#141676=CARTESIAN_POINT('Ctrl Pts',(11.5281743620239,-24.4,9.99201361353606));
#141677=CARTESIAN_POINT('',(11.5281743620239,-24.4,9.99201361353606));
#141678=CARTESIAN_POINT('',(11.5845457335763,-24.,9.59600569888119));
#141679=CARTESIAN_POINT('Origin',(11.5281743620239,-24.,9.99201361353606));
#141680=CARTESIAN_POINT('Origin',(11.4999886762478,-24.,10.1900175708635));
#141681=CARTESIAN_POINT('Origin',(11.4999886762478,-24.4,10.1900175708635));
#141682=CARTESIAN_POINT('Origin',(15.1,-24.,-15.1000000000002));
#141683=CARTESIAN_POINT('',(11.7266197306119,-24.4,10.0194623972745));
#141684=CARTESIAN_POINT('',(11.7798591918362,-24.,9.62302127961819));
#141685=CARTESIAN_POINT('Origin',(11.7266197306119,-24.,10.0194623972745));
#141686=CARTESIAN_POINT('Origin',(15.1,-24.,-15.1000000000002));
#141687=CARTESIAN_POINT('Origin',(15.1,-24.4,-15.1000000000002));
#141688=CARTESIAN_POINT('Ctrl Pts',(11.7798591918362,-24.,9.62302127961819));
#141689=CARTESIAN_POINT('Ctrl Pts',(12.2999999999997,-24.,9.69287280397854));
#141690=CARTESIAN_POINT('Ctrl Pts',(12.2999999999997,-24.,10.2176829561026));
#141691=CARTESIAN_POINT('Ctrl Pts',(11.7798591918362,-24.4,9.62302127961819));
#141692=CARTESIAN_POINT('Ctrl Pts',(12.2999999999997,-24.4,9.69287280397853));
#141693=CARTESIAN_POINT('Ctrl Pts',(12.2999999999997,-24.4,10.2176829561026));
#141694=CARTESIAN_POINT('Ctrl Pts',(11.7266197306119,-24.4,10.0194623972745));
#141695=CARTESIAN_POINT('Ctrl Pts',(11.8999999999997,-24.4,10.0427462387279));
#141696=CARTESIAN_POINT('Ctrl Pts',(11.8999999999997,-24.4,10.2176829561026));
#141697=CARTESIAN_POINT('',(11.8999999999997,-24.4,10.2176829561026));
#141698=CARTESIAN_POINT('',(12.2999999999997,-24.,10.2176829561026));
#141699=CARTESIAN_POINT('Origin',(11.8999999999997,-24.,10.2176829561026));
#141700=CARTESIAN_POINT('Origin',(11.6999999999997,-24.,10.2176829561026));
#141701=CARTESIAN_POINT('Origin',(11.6999999999997,-24.4,10.2176829561026));
#141702=CARTESIAN_POINT('Origin',(11.8999999999997,-24.,9.96444707415598));
#141703=CARTESIAN_POINT('',(12.2999999999997,-24.,11.899999999963));
#141704=CARTESIAN_POINT('',(12.2999999999997,-24.,9.96444707415599));
#141705=CARTESIAN_POINT('',(11.8999999999997,-24.4,11.499999999963));
#141706=CARTESIAN_POINT('',(11.8999999999997,-24.4,9.96444707415598));
#141707=CARTESIAN_POINT('Origin',(11.8999999999997,-24.,11.499999999963));
#141708=CARTESIAN_POINT('Origin',(8.47425608016909,-24.,11.499999999963));
#141709=CARTESIAN_POINT('',(8.47425608016909,-24.,11.899999999963));
#141710=CARTESIAN_POINT('',(8.47425608016909,-24.4,11.499999999963));
#141711=CARTESIAN_POINT('Origin',(12.2999999999997,-10.3,9.68731764791195));
#141712=CARTESIAN_POINT('',(12.2999999999997,-17.5694764848252,11.899999999963));
#141713=CARTESIAN_POINT('',(12.2999999999997,-16.55,11.899999999963));
#141714=CARTESIAN_POINT('',(12.2999999999997,-11.8066740905561,12.2));
#141715=CARTESIAN_POINT('Origin',(12.2999999999996,-14.8,14.199999999963));
#141716=CARTESIAN_POINT('',(12.2999999999997,-10.3,12.2));
#141717=CARTESIAN_POINT('',(12.2999999999997,-10.3,12.2));
#141718=CARTESIAN_POINT('',(12.2999999999997,-10.3,10.2176829561026));
#141719=CARTESIAN_POINT('',(12.2999999999997,-10.3,9.67578794473567));
#141720=CARTESIAN_POINT('',(12.2999999999997,-10.3,10.2176829561026));
#141721=CARTESIAN_POINT('Origin',(13.8999999999998,-22.8,11.899999999963));
#141722=CARTESIAN_POINT('',(10.4985290936118,-18.7372583002031,11.899999999963));
#141723=CARTESIAN_POINT('',(10.4985290936118,-24.4,11.899999999963));
#141724=CARTESIAN_POINT('',(9.32485954615698,-17.7372583002031,11.899999999963));
#141725=CARTESIAN_POINT('Ctrl Pts',(10.4985290936118,-18.7372583002031,
11.899999999963));
#141726=CARTESIAN_POINT('Ctrl Pts',(9.83672072559501,-18.1453701441239,
11.899999999963));
#141727=CARTESIAN_POINT('Ctrl Pts',(9.33545999193445,-17.7456813369822,
11.899999999963));
#141728=CARTESIAN_POINT('Ctrl Pts',(9.32485954615698,-17.7372583002031,
11.899999999963));
#141729=CARTESIAN_POINT('',(9.32485954615879,-17.0248595461262,11.8999999999606));
#141730=CARTESIAN_POINT('',(9.32485954615698,-24.4,11.899999999963));
#141731=CARTESIAN_POINT('',(11.8999999999998,-17.0248595461287,11.899999999963));
#141732=CARTESIAN_POINT('',(13.8999999999996,-17.0248595461287,11.899999999963));
#141733=CARTESIAN_POINT('Ctrl Pts',(11.8999999999998,-17.0248595461287,
11.899999999963));
#141734=CARTESIAN_POINT('Ctrl Pts',(11.9442850147497,-17.0248595461287,
11.899999999963));
#141735=CARTESIAN_POINT('Ctrl Pts',(11.9956860440864,-17.0383505886509,
11.899999999963));
#141736=CARTESIAN_POINT('Ctrl Pts',(12.0829656062854,-17.0830517207412,
11.899999999963));
#141737=CARTESIAN_POINT('Ctrl Pts',(12.13151199187,-17.1255662498947,11.899999999963));
#141738=CARTESIAN_POINT('Ctrl Pts',(12.2060204418464,-17.2176526173486,
11.899999999963));
#141739=CARTESIAN_POINT('Ctrl Pts',(12.2421146765233,-17.28636338603,11.899999999963));
#141740=CARTESIAN_POINT('Ctrl Pts',(12.2861083322068,-17.4146162004345,
11.899999999963));
#141741=CARTESIAN_POINT('Ctrl Pts',(12.2999999999998,-17.4985665379817,
11.899999999963));
#141742=CARTESIAN_POINT('Ctrl Pts',(12.2999999999998,-17.5694764848252,
11.899999999963));
#141743=CARTESIAN_POINT('Origin',(7.1,-24.4,10.2));
#141744=CARTESIAN_POINT('',(10.8999902203958,-18.7372583002031,10.1913788112003));
#141745=CARTESIAN_POINT('',(10.8999902203958,-10.3,10.1913788112003));
#141746=CARTESIAN_POINT('Origin',(7.1,-18.7372583002031,10.2));
#141747=CARTESIAN_POINT('Origin',(3.04851216033843,-24.4,10.2415765003998));
#141748=CARTESIAN_POINT('Origin',(5.65685424949238,-24.,-12.8999999999999));
#141749=CARTESIAN_POINT('',(9.28759150877464,-23.9860345618388,-12.1992436937665));
#141750=CARTESIAN_POINT('',(9.28736209575136,-24.,-12.1993418985011));
#141751=CARTESIAN_POINT('Ctrl Pts',(9.28759150880459,-23.98603456184,-12.1992436937537));
#141752=CARTESIAN_POINT('Ctrl Pts',(9.28743869432123,-23.9906846184834,
-12.1993091465896));
#141753=CARTESIAN_POINT('Ctrl Pts',(9.28736209575136,-23.9953405449403,
-12.1993418985011));
#141754=CARTESIAN_POINT('Ctrl Pts',(9.28736209575136,-24.,-12.1993418985011));
#141755=CARTESIAN_POINT('',(3.29032212515741,-23.9860345609289,-10.0587259632996));
#141756=CARTESIAN_POINT('Origin',(5.65685424949238,-23.9860345609261,-12.8999999999999));
#141757=CARTESIAN_POINT('',(3.29051067971883,-24.,-10.0588862911288));
#141758=CARTESIAN_POINT('Ctrl Pts',(3.29051067971883,-24.,-10.0588862911288));
#141759=CARTESIAN_POINT('Ctrl Pts',(3.29051067971883,-23.9953398535192,
-10.0588862911288));
#141760=CARTESIAN_POINT('Ctrl Pts',(3.29044771115612,-23.9906840233497,
-10.0588327519088));
#141761=CARTESIAN_POINT('Ctrl Pts',(3.29032212515734,-23.9860345609289,
-10.0587259632996));
#141762=CARTESIAN_POINT('',(3.3089883286316,-24.4,-9.54187032534883));
#141763=CARTESIAN_POINT('Ctrl Pts',(3.30898832863159,-24.4,-9.54187032534883));
#141764=CARTESIAN_POINT('Ctrl Pts',(3.3089127945394,-24.4,-9.54302222643878));
#141765=CARTESIAN_POINT('Ctrl Pts',(3.30883748342679,-24.399996957327,-9.54417414390669));
#141766=CARTESIAN_POINT('Ctrl Pts',(3.30550334651522,-24.399726789429,-9.59532351692953));
#141767=CARTESIAN_POINT('Ctrl Pts',(3.30266654088576,-24.3937324334157,
-9.6454638152666));
#141768=CARTESIAN_POINT('Ctrl Pts',(3.29802761162445,-24.3705240815341,
-9.74158961799118));
#141769=CARTESIAN_POINT('Ctrl Pts',(3.29619025535583,-24.3535039951622,
-9.78793108463616));
#141770=CARTESIAN_POINT('Ctrl Pts',(3.29317220178152,-24.3044744324752,
-9.88126024765772));
#141771=CARTESIAN_POINT('Ctrl Pts',(3.29213934109232,-24.2703518742144,
-9.92746145303948));
#141772=CARTESIAN_POINT('Ctrl Pts',(3.29102336292671,-24.1952991262786,
-9.99546731421881));
#141773=CARTESIAN_POINT('Ctrl Pts',(3.29078368451477,-24.1574693504857,
-10.0200507383762));
#141774=CARTESIAN_POINT('Ctrl Pts',(3.29054076369835,-24.0787815416442,
-10.0511334347581));
#141775=CARTESIAN_POINT('Ctrl Pts',(3.29051067971883,-24.0397880746094,
-10.0588862911288));
#141776=CARTESIAN_POINT('Ctrl Pts',(3.29051067971883,-24.,-10.0588862911288));
#141777=CARTESIAN_POINT('',(6.61977032797715,-24.4,-8.91724945296497));
#141778=CARTESIAN_POINT('Origin',(5.65685424949238,-24.4,-12.8999999999999));
#141779=CARTESIAN_POINT('',(7.20805405049754,-24.3984199843545,-9.1458714239949));
#141780=CARTESIAN_POINT('Ctrl Pts',(7.20805405049754,-24.3984199843545,
-9.1458714239949));
#141781=CARTESIAN_POINT('Ctrl Pts',(6.90636576576306,-24.397809874008,-9.02861943572731));
#141782=CARTESIAN_POINT('Ctrl Pts',(6.7786421819491,-24.39962955605,-8.97898757769515));
#141783=CARTESIAN_POINT('Ctrl Pts',(6.67099081608409,-24.399947062377,-8.93715374025662));
#141784=CARTESIAN_POINT('Ctrl Pts',(6.64964997085853,-24.3999890424235,
-8.92886064780516));
#141785=CARTESIAN_POINT('Ctrl Pts',(6.62551569595268,-24.3999993697358,
-8.91948209361555));
#141786=CARTESIAN_POINT('Ctrl Pts',(6.62264293759876,-24.4,-8.91836574382844));
#141787=CARTESIAN_POINT('Ctrl Pts',(6.61977032797715,-24.4,-8.91724945296497));
#141788=CARTESIAN_POINT('',(9.38783269785609,-24.3739393224439,-11.5863664642257));
#141789=CARTESIAN_POINT('Ctrl Pts',(9.38783269785609,-24.3739393224439,
-11.5863664642257));
#141790=CARTESIAN_POINT('Ctrl Pts',(9.26990225756709,-24.3877368249567,
-11.1420300359286));
#141791=CARTESIAN_POINT('Ctrl Pts',(9.068557708432,-24.3930188075499,-10.7236304265978));
#141792=CARTESIAN_POINT('Ctrl Pts',(8.58163711558267,-24.3980317489178,
-10.0688695190312));
#141793=CARTESIAN_POINT('Ctrl Pts',(8.32848943789226,-24.3986403983757,
-9.81649678623844));
#141794=CARTESIAN_POINT('Ctrl Pts',(7.78572548264438,-24.3991085362301,
-9.41576798370814));
#141795=CARTESIAN_POINT('Ctrl Pts',(7.50514199796396,-24.3990207913455,
-9.26133547842921));
#141796=CARTESIAN_POINT('Ctrl Pts',(7.20805405049754,-24.3984199843545,
-9.1458714239949));
#141797=CARTESIAN_POINT('Ctrl Pts',(9.28736209575136,-24.,-12.1993418985011));
#141798=CARTESIAN_POINT('Ctrl Pts',(9.28736209575136,-24.0226784817566,
-12.1993418985011));
#141799=CARTESIAN_POINT('Ctrl Pts',(9.2888110615892,-24.0451292520319,-12.1966331561604));
#141800=CARTESIAN_POINT('Ctrl Pts',(9.29445398178838,-24.0898867003991,
-12.1858228852564));
#141801=CARTESIAN_POINT('Ctrl Pts',(9.29870760508546,-24.1117158371081,
-12.1775929804491));
#141802=CARTESIAN_POINT('Ctrl Pts',(9.31367063881442,-24.1705623930577,
-12.1473840540648));
#141803=CARTESIAN_POINT('Ctrl Pts',(9.32706218188048,-24.2053291077597,
-12.1192924667623));
#141804=CARTESIAN_POINT('Ctrl Pts',(9.36003187846609,-24.2738464175524,
-12.0372926322239));
#141805=CARTESIAN_POINT('Ctrl Pts',(9.37926713369123,-24.3028996833776,
-11.9809172492032));
#141806=CARTESIAN_POINT('Ctrl Pts',(9.40700119469152,-24.3468831586282,
-11.847323417685));
#141807=CARTESIAN_POINT('Ctrl Pts',(9.41407362988669,-24.360132393681,-11.7709710919796));
#141808=CARTESIAN_POINT('Ctrl Pts',(9.40317973190691,-24.3708302579929,
-11.6559864908138));
#141809=CARTESIAN_POINT('Ctrl Pts',(9.39697144103178,-24.3728701173123,
-11.6207992747186));
#141810=CARTESIAN_POINT('Ctrl Pts',(9.38783269785609,-24.3739393224439,
-11.5863664642257));
#141811=CARTESIAN_POINT('Ctrl Pts',(9.28736209575136,-24.,-12.1993418985011));
#141812=CARTESIAN_POINT('Ctrl Pts',(9.72748477929187,-24.,-12.0110470586274));
#141813=CARTESIAN_POINT('Ctrl Pts',(9.64163093544796,-24.,-11.540099035182));
#141814=CARTESIAN_POINT('Ctrl Pts',(9.28736209575136,-24.2759603294941,
-12.1993418985011));
#141815=CARTESIAN_POINT('Ctrl Pts',(9.72748477929187,-24.2759603294941,
-12.0110470586274));
#141816=CARTESIAN_POINT('Ctrl Pts',(9.64163093544796,-24.2759603294941,
-11.540099035182));
#141817=CARTESIAN_POINT('Ctrl Pts',(9.18588826821947,-24.3739393224439,
-11.9621557211613));
#141818=CARTESIAN_POINT('Ctrl Pts',(9.4367721008869,-24.3739393224439,-11.8548217143816));
#141819=CARTESIAN_POINT('Ctrl Pts',(9.38783269785609,-24.3739393224439,
-11.5863664642257));
#141820=CARTESIAN_POINT('',(9.64163093544796,-24.,-11.540099035182));
#141821=CARTESIAN_POINT('Origin',(9.24811638706485,-24.,-11.6118367533701));
#141822=CARTESIAN_POINT('Origin',(9.0513591128733,-24.,-11.6477056124642));
#141823=CARTESIAN_POINT('Origin',(6.1,-24.,-12.1857384988752));
#141824=CARTESIAN_POINT('',(7.33287671232877,-24.,-8.80342937459372));
#141825=CARTESIAN_POINT('Origin',(7.1958904109589,-24.,-9.17924149951388));
#141826=CARTESIAN_POINT('Origin',(6.1,-24.,-12.1857384988752));
#141827=CARTESIAN_POINT('Origin',(8.6,-24.,-5.32716721908225));
#141828=CARTESIAN_POINT('',(4.5,-24.4,-5.32716721908225));
#141829=CARTESIAN_POINT('Origin',(8.6,-24.4,-5.32716721908225));
#141830=CARTESIAN_POINT('',(4.9,-24.,-5.32716721908225));
#141831=CARTESIAN_POINT('Origin',(4.5,-24.,-5.32716721908225));
#141832=CARTESIAN_POINT('Origin',(8.6,-24.,-5.32716721908225));
#141833=CARTESIAN_POINT('Origin',(-3.45175358661618,-24.4,-3.05000000003699));
#141834=CARTESIAN_POINT('',(1.01279069686664,-24.4,-6.14651140747171));
#141835=CARTESIAN_POINT('Origin',(9.25,-24.4,-3.05000000003699));
#141836=CARTESIAN_POINT('',(0.999999999210583,-24.4,-6.07613614821183));
#141837=CARTESIAN_POINT('Origin',(1.19999999921058,-24.4,-6.07613614821183));
#141838=CARTESIAN_POINT('',(0.999999999210583,-24.4,-4.25000000003699));
#141839=CARTESIAN_POINT('',(0.999999999210583,-24.4,-4.75788611936281));
#141840=CARTESIAN_POINT('',(1.19999999921058,-24.4,-4.05000000003699));
#141841=CARTESIAN_POINT('Origin',(1.19999999921058,-24.4,-4.25000000003699));
#141842=CARTESIAN_POINT('',(4.3,-24.4,-4.05000000003699));
#141843=CARTESIAN_POINT('',(-1.71792900372085,-24.4,-4.05000000003699));
#141844=CARTESIAN_POINT('',(4.5,-24.4,-4.25000000003699));
#141845=CARTESIAN_POINT('Origin',(4.3,-24.4,-4.25000000003699));
#141846=CARTESIAN_POINT('',(4.5,-24.4,-4.18858360955962));
#141847=CARTESIAN_POINT('Origin',(4.5,-24.,-4.18858360955962));
#141848=CARTESIAN_POINT('',(4.9,-24.,-4.25000000003699));
#141849=CARTESIAN_POINT('Origin',(4.5,-24.,-4.25000000003699));
#141850=CARTESIAN_POINT('',(4.9,-24.,-4.18858360955962));
#141851=CARTESIAN_POINT('Ctrl Pts',(4.9,-24.,-4.25000000003699));
#141852=CARTESIAN_POINT('Ctrl Pts',(4.9,-24.,-3.65000000003699));
#141853=CARTESIAN_POINT('Ctrl Pts',(4.3,-24.,-3.65000000003699));
#141854=CARTESIAN_POINT('Ctrl Pts',(4.9,-24.4,-4.25000000003699));
#141855=CARTESIAN_POINT('Ctrl Pts',(4.9,-24.4,-3.65000000003699));
#141856=CARTESIAN_POINT('Ctrl Pts',(4.3,-24.4,-3.65000000003699));
#141857=CARTESIAN_POINT('Ctrl Pts',(4.5,-24.4,-4.25000000003699));
#141858=CARTESIAN_POINT('Ctrl Pts',(4.5,-24.4,-4.05000000003699));
#141859=CARTESIAN_POINT('Ctrl Pts',(4.3,-24.4,-4.05000000003699));
#141860=CARTESIAN_POINT('',(4.3,-24.,-3.65000000003699));
#141861=CARTESIAN_POINT('Origin',(4.3,-24.,-4.05000000003699));
#141862=CARTESIAN_POINT('Origin',(4.3,-24.,-4.25000000003699));
#141863=CARTESIAN_POINT('Origin',(-1.71792900372085,-24.,-4.05000000003699));
#141864=CARTESIAN_POINT('',(1.19999999921058,-24.,-3.65000000003699));
#141865=CARTESIAN_POINT('Origin',(1.19999999921058,-24.,-4.05000000003699));
#141866=CARTESIAN_POINT('',(-1.71792900372085,-24.,-3.65000000003699));
#141867=CARTESIAN_POINT('Ctrl Pts',(1.19999999921058,-24.,-3.65000000003699));
#141868=CARTESIAN_POINT('Ctrl Pts',(0.599999999210583,-24.,-3.65000000003699));
#141869=CARTESIAN_POINT('Ctrl Pts',(0.599999999210583,-24.,-4.25000000003699));
#141870=CARTESIAN_POINT('Ctrl Pts',(1.19999999921058,-24.4,-3.65000000003699));
#141871=CARTESIAN_POINT('Ctrl Pts',(0.599999999210583,-24.4,-3.65000000003699));
#141872=CARTESIAN_POINT('Ctrl Pts',(0.599999999210583,-24.4,-4.25000000003699));
#141873=CARTESIAN_POINT('Ctrl Pts',(1.19999999921058,-24.4,-4.05000000003699));
#141874=CARTESIAN_POINT('Ctrl Pts',(0.999999999210583,-24.4,-4.05000000003699));
#141875=CARTESIAN_POINT('Ctrl Pts',(0.999999999210583,-24.4,-4.25000000003699));
#141876=CARTESIAN_POINT('',(0.599999999210583,-24.,-4.25000000003699));
#141877=CARTESIAN_POINT('Origin',(0.999999999210583,-24.,-4.25000000003699));
#141878=CARTESIAN_POINT('Origin',(1.19999999921058,-24.,-4.25000000003699));
#141879=CARTESIAN_POINT('Origin',(0.999999999210583,-24.,-4.75788611936281));
#141880=CARTESIAN_POINT('',(0.599999999210583,-24.,-6.07613614821183));
#141881=CARTESIAN_POINT('Origin',(0.999999999210583,-24.,-6.07613614821183));
#141882=CARTESIAN_POINT('',(0.599999999210583,-24.,-4.75788611936281));
#141883=CARTESIAN_POINT('Ctrl Pts',(0.599999999210582,-24.,-6.07613614821183));
#141884=CARTESIAN_POINT('Ctrl Pts',(0.599999999210582,-24.,-6.18518609949224));
#141885=CARTESIAN_POINT('Ctrl Pts',(0.638372092178763,-24.,-6.28726192599147));
#141886=CARTESIAN_POINT('Ctrl Pts',(0.599999999210582,-24.4,-6.07613614821183));
#141887=CARTESIAN_POINT('Ctrl Pts',(0.599999999210582,-24.4,-6.18518609949224));
#141888=CARTESIAN_POINT('Ctrl Pts',(0.638372092178763,-24.4,-6.28726192599147));
#141889=CARTESIAN_POINT('Ctrl Pts',(0.999999999210582,-24.4,-6.07613614821183));
#141890=CARTESIAN_POINT('Ctrl Pts',(0.999999999210582,-24.4,-6.11248613197196));
#141891=CARTESIAN_POINT('Ctrl Pts',(1.01279069686664,-24.4,-6.14651140747171));
#141892=CARTESIAN_POINT('',(0.638372092178764,-24.,-6.28726192599147));
#141893=CARTESIAN_POINT('Origin',(1.01279069686664,-24.,-6.14651140747171));
#141894=CARTESIAN_POINT('Origin',(1.19999999921058,-24.,-6.07613614821183));
#141895=CARTESIAN_POINT('Origin',(9.25,-24.,-3.05000000003699));
#141896=CARTESIAN_POINT('Origin',(9.25,-24.,-3.05000000003699));
#141897=CARTESIAN_POINT('Origin',(9.0513591128733,-19.9,-11.6477056124642));
#141898=CARTESIAN_POINT('',(9.64163093544796,-20.,-11.540099035182));
#141899=CARTESIAN_POINT('',(9.64163093544796,-19.9,-11.540099035182));
#141900=CARTESIAN_POINT('',(9.03750044632957,-20.,-12.2475455389126));
#141901=CARTESIAN_POINT('Origin',(9.0513591128733,-20.,-11.6477056124642));
#141902=CARTESIAN_POINT('',(9.03750044632957,-22.5020352696956,-12.2475455389126));
#141903=CARTESIAN_POINT('',(9.03750044632957,-19.9,-12.2475455389126));
#141904=CARTESIAN_POINT('Ctrl Pts',(9.03750044632957,-22.5020352696956,
-12.2475455389126));
#141905=CARTESIAN_POINT('Ctrl Pts',(9.09123412340781,-22.6355177185059,
-12.248786998642));
#141906=CARTESIAN_POINT('Ctrl Pts',(9.13679223934425,-22.7752399470139,
-12.2427744067466));
#141907=CARTESIAN_POINT('Ctrl Pts',(9.24836945479761,-23.2096289940093,
-12.2195751234883));
#141908=CARTESIAN_POINT('Ctrl Pts',(9.28517493986822,-23.5143240465938,
-12.2002907823841));
#141909=CARTESIAN_POINT('Ctrl Pts',(9.28930197413971,-23.8000000000006,
-12.1985079316063));
#141910=CARTESIAN_POINT('Ctrl Pts',(9.2901945404804,-23.8617840133094,-12.1981223490087));
#141911=CARTESIAN_POINT('Ctrl Pts',(9.28963512742458,-23.9238484297288,
-12.1983683799008));
#141912=CARTESIAN_POINT('Ctrl Pts',(9.28759150880459,-23.98603456184,-12.1992436937537));
#141913=CARTESIAN_POINT('Origin',(6.1,-19.9,-12.1857384988752));
#141914=CARTESIAN_POINT('',(7.33287671232877,-20.,-8.80342937459372));
#141915=CARTESIAN_POINT('',(7.33287671232877,-19.9,-8.80342937459372));
#141916=CARTESIAN_POINT('Origin',(6.1,-20.,-12.1857384988752));
#141917=CARTESIAN_POINT('Origin',(8.6,-19.9,-5.32716721908225));
#141918=CARTESIAN_POINT('',(4.9,-20.,-5.32716721908225));
#141919=CARTESIAN_POINT('',(4.9,-19.9,-5.32716721908225));
#141920=CARTESIAN_POINT('Origin',(8.6,-20.,-5.32716721908225));
#141921=CARTESIAN_POINT('Origin',(4.9,-19.9,-5.32716721908225));
#141922=CARTESIAN_POINT('',(4.9,-20.,-4.25000000003699));
#141923=CARTESIAN_POINT('',(4.9,-19.9,-4.25000000003699));
#141924=CARTESIAN_POINT('',(4.9,-20.,-2.88858360955241));
#141925=CARTESIAN_POINT('Origin',(4.3,-19.9,-4.25000000003699));
#141926=CARTESIAN_POINT('',(4.3,-20.,-3.65000000003699));
#141927=CARTESIAN_POINT('',(4.3,-19.9,-3.65000000003699));
#141928=CARTESIAN_POINT('Origin',(4.3,-20.,-4.25000000003699));
#141929=CARTESIAN_POINT('Origin',(0.0158955791744741,-19.9,-3.65000000003699));
#141930=CARTESIAN_POINT('',(1.19999999921058,-20.,-3.65000000003699));
#141931=CARTESIAN_POINT('',(1.19999999921058,-19.9,-3.65000000003699));
#141932=CARTESIAN_POINT('',(-1.31220842229031,-20.,-3.65000000003699));
#141933=CARTESIAN_POINT('Origin',(1.19999999921058,-19.9,-4.25000000003699));
#141934=CARTESIAN_POINT('',(0.599999999210583,-20.,-4.25000000003699));
#141935=CARTESIAN_POINT('',(0.599999999210583,-19.9,-4.25000000003699));
#141936=CARTESIAN_POINT('Origin',(1.19999999921058,-20.,-4.25000000003699));
#141937=CARTESIAN_POINT('Origin',(0.599999999210582,-19.9,-6.46577223868862));
#141938=CARTESIAN_POINT('',(0.599999999210583,-20.,-6.07613614821183));
#141939=CARTESIAN_POINT('',(0.599999999210583,-21.1,-6.07613614821183));
#141940=CARTESIAN_POINT('',(0.599999999210583,-20.,-3.4578861193556));
#141941=CARTESIAN_POINT('Origin',(1.19999999921058,-21.1,-6.07613614821183));
#141942=CARTESIAN_POINT('',(0.638372092178764,-20.,-6.28726192599147));
#141943=CARTESIAN_POINT('',(0.638372092178764,-21.1,-6.28726192599147));
#141944=CARTESIAN_POINT('Origin',(1.19999999921058,-20.,-6.07613614821183));
#141945=CARTESIAN_POINT('Origin',(9.25,-21.1,-3.05000000003699));
#141946=CARTESIAN_POINT('Ctrl Pts',(9.03750044632957,-22.5020352696956,
-12.2475455389126));
#141947=CARTESIAN_POINT('Ctrl Pts',(8.98537162787598,-22.3725395284934,
-12.2463411577428));
#141948=CARTESIAN_POINT('Ctrl Pts',(8.92564846760114,-22.2460178877848,
-12.2445240024109));
#141949=CARTESIAN_POINT('Ctrl Pts',(8.71336297104777,-21.8572772044711,
-12.2354893007256));
#141950=CARTESIAN_POINT('Ctrl Pts',(8.53368079632539,-21.610148441077,-12.2244104567008));
#141951=CARTESIAN_POINT('Ctrl Pts',(8.12142382370261,-21.1750909413994,
-12.1828657208104));
#141952=CARTESIAN_POINT('Ctrl Pts',(7.88887334972075,-20.9871548429568,
-12.1522357203516));
#141953=CARTESIAN_POINT('Ctrl Pts',(7.41647976391155,-20.6988748539929,
-12.0683269172958));
#141954=CARTESIAN_POINT('Ctrl Pts',(7.15662707779066,-20.5802100071682,
-12.0129405712226));
#141955=CARTESIAN_POINT('Ctrl Pts',(6.62192580066298,-20.4243112646203,
-11.8709829857734));
#141956=CARTESIAN_POINT('Ctrl Pts',(6.34714997371524,-20.3871246330873,
-11.784085965654));
#141957=CARTESIAN_POINT('Ctrl Pts',(5.84722372089706,-20.3871246330873,
-11.6017196823151));
#141958=CARTESIAN_POINT('Ctrl Pts',(5.58103575919986,-20.4243112646203,
-11.4912804853426));
#141959=CARTESIAN_POINT('Ctrl Pts',(5.08052131739254,-20.5802100071682,
-11.2556054858818));
#141960=CARTESIAN_POINT('Ctrl Pts',(4.84604074311545,-20.6988748539929,
-11.130665796022));
#141961=CARTESIAN_POINT('Ctrl Pts',(4.43057607697443,-20.9871548429568,
-10.8906960097316));
#141962=CARTESIAN_POINT('Ctrl Pts',(4.23292528343976,-21.1750909413994,
-10.7643944511806));
#141963=CARTESIAN_POINT('Ctrl Pts',(3.89075001978357,-21.610148441077,-10.5307325897267));
#141964=CARTESIAN_POINT('Ctrl Pts',(3.74613849230621,-21.8572772044711,
-10.423513511114));
#141965=CARTESIAN_POINT('Ctrl Pts',(3.40776601711932,-22.6391281658009,
-10.1625026467189));
#141966=CARTESIAN_POINT('Ctrl Pts',(3.29568612325364,-23.2300913446515,
-10.0632891899245));
#141967=CARTESIAN_POINT('Ctrl Pts',(3.2889159286883,-23.8,-10.0575299995985));
#141968=CARTESIAN_POINT('Ctrl Pts',(3.28817872204094,-23.8620573670452,
-10.0569028812268));
#141969=CARTESIAN_POINT('Ctrl Pts',(3.2886489655866,-23.9240906131805,-10.057303237953));
#141970=CARTESIAN_POINT('Ctrl Pts',(3.29032212515734,-23.9860345609289,
-10.0587259632996));
#141971=CARTESIAN_POINT('',(9.25,-20.,-12.250000000037));
#141972=CARTESIAN_POINT('Origin',(9.25,-20.,-3.05000000003699));
#141973=CARTESIAN_POINT('',(9.25,-15.9,-12.250000000037));
#141974=CARTESIAN_POINT('',(9.25,-21.1,-12.250000000037));
#141975=CARTESIAN_POINT('',(0.194290142826891,-15.9,-4.67299691398904));
#141976=CARTESIAN_POINT('Origin',(9.25,-15.9,-3.05000000003699));
#141977=CARTESIAN_POINT('',(0.194290142826895,-16.4303892440217,-4.67299691398904));
#141978=CARTESIAN_POINT('',(0.194290142826893,-21.1,-4.67299691398904));
#141979=CARTESIAN_POINT('',(0.47847834656078,-17.2370030965064,-5.82496087962556));
#141980=CARTESIAN_POINT('Origin',(9.25,-15.2939545703814,-3.05000000003699));
#141981=CARTESIAN_POINT('',(0.644705633055379,-17.4355690700213,-6.30406036490954));
#141982=CARTESIAN_POINT('Ctrl Pts',(0.644705633059486,-17.4355690700257,
-6.3040603649199));
#141983=CARTESIAN_POINT('Ctrl Pts',(0.603246655335933,-17.4006034041543,
-6.19442296811137));
#141984=CARTESIAN_POINT('Ctrl Pts',(0.565483129929027,-17.368112123324,
-6.08802112521124));
#141985=CARTESIAN_POINT('Ctrl Pts',(0.513579180401821,-17.3023542725618,
-5.93419691137546));
#141986=CARTESIAN_POINT('Ctrl Pts',(0.494843565862922,-17.2732246177677,
-5.87669057301615));
#141987=CARTESIAN_POINT('Ctrl Pts',(0.478478346560781,-17.2370030965064,
-5.82496087962556));
#141988=CARTESIAN_POINT('',(0.227169467729596,-19.1738552422879,-4.84681083758479));
#141989=CARTESIAN_POINT('Ctrl Pts',(0.227169467729604,-19.1738552422878,
-4.84681083758478));
#141990=CARTESIAN_POINT('Ctrl Pts',(0.288341103269117,-19.1595858444531,
-5.15398913889562));
#141991=CARTESIAN_POINT('Ctrl Pts',(0.364344206904044,-19.1359275310739,
-5.45154142969646));
#141992=CARTESIAN_POINT('Ctrl Pts',(0.531373163443829,-19.0522811885239,
-6.00095643599083));
#141993=CARTESIAN_POINT('Ctrl Pts',(0.64706147259344,-18.9778030839297,
-6.32116532630702));
#141994=CARTESIAN_POINT('Ctrl Pts',(0.792548014213962,-18.813342562401,
-6.67277297469914));
#141995=CARTESIAN_POINT('Ctrl Pts',(0.845006682143811,-18.7418056498301,
-6.79239746305243));
#141996=CARTESIAN_POINT('Ctrl Pts',(0.914713320592898,-18.6089688816776,
-6.94460170106634));
#141997=CARTESIAN_POINT('Ctrl Pts',(0.944350360166487,-18.5391485007925,
-7.00709614019699));
#141998=CARTESIAN_POINT('Ctrl Pts',(0.976481807510859,-18.4195181965843,
-7.07361815041777));
#141999=CARTESIAN_POINT('Ctrl Pts',(0.985172457114319,-18.3771538424934,
-7.09138547440372));
#142000=CARTESIAN_POINT('Ctrl Pts',(0.996932135198067,-18.2897944712841,
-7.11534824541121));
#142001=CARTESIAN_POINT('Ctrl Pts',(1.,-18.2448003741776,-7.12154761734421));
#142002=CARTESIAN_POINT('Ctrl Pts',(1.,-18.1551996258224,-7.12154761734421));
#142003=CARTESIAN_POINT('Ctrl Pts',(0.996932135198067,-18.1102055287159,
-7.11534824541121));
#142004=CARTESIAN_POINT('Ctrl Pts',(0.98517245711432,-18.0228461575066,
-7.09138547440372));
#142005=CARTESIAN_POINT('Ctrl Pts',(0.97648180751086,-17.9804818034157,
-7.07361815041777));
#142006=CARTESIAN_POINT('Ctrl Pts',(0.944350360166488,-17.8608514992075,
-7.00709614019699));
#142007=CARTESIAN_POINT('Ctrl Pts',(0.914713320592898,-17.7910311183224,
-6.94460170106634));
#142008=CARTESIAN_POINT('Ctrl Pts',(0.845006682143811,-17.6581943501699,
-6.79239746305243));
#142009=CARTESIAN_POINT('Ctrl Pts',(0.792548014213962,-17.586657437599,
-6.67277297469914));
#142010=CARTESIAN_POINT('Ctrl Pts',(0.715345229333762,-17.4993860644298,
-6.48619152641746));
#142011=CARTESIAN_POINT('Ctrl Pts',(0.679882242726209,-17.4652363133496,
-6.39708417120235));
#142012=CARTESIAN_POINT('Ctrl Pts',(0.644705633055442,-17.4355690700223,
-6.30406036490921));
#142013=CARTESIAN_POINT('',(0.194290142826893,-19.2201728349062,-4.67299691398903));
#142014=CARTESIAN_POINT('Ctrl Pts',(0.194292330138919,-19.2200994892544,
-4.67313792326464));
#142015=CARTESIAN_POINT('Ctrl Pts',(0.196951382332334,-19.2121899859122,
-4.68795556951401));
#142016=CARTESIAN_POINT('Ctrl Pts',(0.19974428037187,-19.2053433257718,
-4.70328228986047));
#142017=CARTESIAN_POINT('Ctrl Pts',(0.202641290095105,-19.1995065588509,
-4.71897015143785));
#142018=CARTESIAN_POINT('Ctrl Pts',(0.204743381693374,-19.195271357772,
-4.73035337937532));
#142019=CARTESIAN_POINT('Ctrl Pts',(0.20690081470169,-19.1915680174414,
-4.74192775747502));
#142020=CARTESIAN_POINT('Ctrl Pts',(0.209112002429709,-19.1883798624547,
-4.75365040315691));
#142021=CARTESIAN_POINT('Ctrl Pts',(0.212120691938237,-19.1840418461306,
-4.76960101676983));
#142022=CARTESIAN_POINT('Ctrl Pts',(0.215230415767539,-19.1806621755999,
-4.78580553951459));
#142023=CARTESIAN_POINT('Ctrl Pts',(0.21839854029795,-19.1782166203877,
-4.80213822120128));
#142024=CARTESIAN_POINT('Ctrl Pts',(0.221271933531467,-19.1759985756955,
-4.81695147004717));
#142025=CARTESIAN_POINT('Ctrl Pts',(0.224194281023603,-19.1745492587607,
-4.83187069759389));
#142026=CARTESIAN_POINT('Ctrl Pts',(0.227169467729732,-19.1738552422878,
-4.84681083758542));
#142027=CARTESIAN_POINT('',(0.194290142826891,-20.,-4.67299691398904));
#142028=CARTESIAN_POINT('',(0.194290142826893,-21.1,-4.67299691398904));
#142029=CARTESIAN_POINT('Origin',(9.25,-20.,-3.05000000003699));
#142030=CARTESIAN_POINT('Origin',(5.65685424949238,-23.8568542494924,-12.8999999999999));
#142031=CARTESIAN_POINT('Origin',(15.1,-24.,-15.1));
#142032=CARTESIAN_POINT('',(11.6304347826087,-24.,-12.7331207884076));
#142033=CARTESIAN_POINT('',(11.3,-24.4,-12.5077037206369));
#142034=CARTESIAN_POINT('Origin',(11.3,-24.,-12.5077037206369));
#142035=CARTESIAN_POINT('',(15.1517070744679,-24.4,-10.5002906202185));
#142036=CARTESIAN_POINT('Origin',(15.1,-24.4,-15.1));
#142037=CARTESIAN_POINT('',(15.1472108071229,-24.,-10.9002653488952));
#142038=CARTESIAN_POINT('Origin',(15.1517070744679,-24.,-10.5002906202185));
#142039=CARTESIAN_POINT('Origin',(15.1,-24.,-15.1));
#142040=CARTESIAN_POINT('Ctrl Pts',(15.1472108071229,-24.,-10.9002653488952));
#142041=CARTESIAN_POINT('Ctrl Pts',(15.6849777763716,-24.,-10.906310590981));
#142042=CARTESIAN_POINT('Ctrl Pts',(15.8935746197026,-24.,-10.4106118769225));
#142043=CARTESIAN_POINT('Ctrl Pts',(16.1021714630336,-24.,-9.91491316286401));
#142044=CARTESIAN_POINT('Ctrl Pts',(15.7218887667622,-24.,-9.53463046659261));
#142045=CARTESIAN_POINT('Ctrl Pts',(15.1472108071229,-24.4,-10.9002653488952));
#142046=CARTESIAN_POINT('Ctrl Pts',(15.6849777763716,-24.4,-10.906310590981));
#142047=CARTESIAN_POINT('Ctrl Pts',(15.8935746197026,-24.4,-10.4106118769225));
#142048=CARTESIAN_POINT('Ctrl Pts',(16.1021714630336,-24.4,-9.91491316286401));
#142049=CARTESIAN_POINT('Ctrl Pts',(15.7218887667622,-24.4,-9.53463046659261));
#142050=CARTESIAN_POINT('Ctrl Pts',(15.1517070744679,-24.4,-10.5002906202185));
#142051=CARTESIAN_POINT('Ctrl Pts',(15.4205905590923,-24.4,-10.5033132412614));
#142052=CARTESIAN_POINT('Ctrl Pts',(15.5248889807578,-24.4,-10.2554638842322));
#142053=CARTESIAN_POINT('Ctrl Pts',(15.6291874024233,-24.4,-10.0076145272029));
#142054=CARTESIAN_POINT('Ctrl Pts',(15.4390460542876,-24.4,-9.81747317906723));
#142055=CARTESIAN_POINT('',(15.4390460542876,-24.4,-9.81747317906723));
#142056=CARTESIAN_POINT('',(15.7218887667622,-24.,-9.53463046659261));
#142057=CARTESIAN_POINT('Origin',(15.4390460542876,-24.,-9.81747317906723));
#142058=CARTESIAN_POINT('Origin',(15.1562033418129,-24.,-10.1003158915419));
#142059=CARTESIAN_POINT('Origin',(15.1562033418129,-24.4,-10.1003158915419));
#142060=CARTESIAN_POINT('Origin',(10.1478480409737,-24.,-4.5262751657534));
#142061=CARTESIAN_POINT('',(14.8514718625661,-24.4,-9.22989898734577));
#142062=CARTESIAN_POINT('',(15.1343145750407,-24.,-8.94705627487115));
#142063=CARTESIAN_POINT('Origin',(14.8514718625661,-24.,-9.22989898734577));
#142064=CARTESIAN_POINT('',(10.4306907534484,-24.,-4.24343245327878));
#142065=CARTESIAN_POINT('',(10.1478480409737,-24.4,-4.5262751657534));
#142066=CARTESIAN_POINT('Origin',(15.69999999999,-24.,-8.38137084992192));
#142067=CARTESIAN_POINT('',(14.49999999999,-24.4,-8.38137084991966));
#142068=CARTESIAN_POINT('',(14.89999999999,-24.,-8.38137084992041));
#142069=CARTESIAN_POINT('Origin',(14.49999999999,-24.,-8.38137084991966));
#142070=CARTESIAN_POINT('Origin',(15.69999999999,-24.,-8.38137084992192));
#142071=CARTESIAN_POINT('Origin',(15.69999999999,-24.4,-8.38137084992192));
#142072=CARTESIAN_POINT('Origin',(14.4999999999975,-24.,-4.37858365125987));
#142073=CARTESIAN_POINT('',(14.4999999999902,-24.4,-8.27794038524243));
#142074=CARTESIAN_POINT('',(14.8999999999902,-24.,-8.27794038524318));
#142075=CARTESIAN_POINT('Origin',(14.4999999999902,-24.,-8.27794038524243));
#142076=CARTESIAN_POINT('',(14.8999999999975,-24.,-4.37858365126063));
#142077=CARTESIAN_POINT('',(14.4999999999975,-24.4,-4.37858365125987));
#142078=CARTESIAN_POINT('Ctrl Pts',(14.8999999999902,-24.,-8.27794038524318));
#142079=CARTESIAN_POINT('Ctrl Pts',(14.8999999999908,-24.,-7.91192841075916));
#142080=CARTESIAN_POINT('Ctrl Pts',(14.6230576451076,-24.,-7.67262170893618));
#142081=CARTESIAN_POINT('Ctrl Pts',(14.3461152902243,-24.,-7.4333150071132));
#142082=CARTESIAN_POINT('Ctrl Pts',(13.9839732502781,-24.,-7.48639898180705));
#142083=CARTESIAN_POINT('Ctrl Pts',(14.8999999999902,-24.4,-8.27794038524318));
#142084=CARTESIAN_POINT('Ctrl Pts',(14.8999999999908,-24.4,-7.91192841075916));
#142085=CARTESIAN_POINT('Ctrl Pts',(14.6230576451076,-24.4,-7.67262170893618));
#142086=CARTESIAN_POINT('Ctrl Pts',(14.3461152902243,-24.4,-7.4333150071132));
#142087=CARTESIAN_POINT('Ctrl Pts',(13.9839732502781,-24.4,-7.48639898180705));
#142088=CARTESIAN_POINT('Ctrl Pts',(14.4999999999902,-24.4,-8.27794038524243));
#142089=CARTESIAN_POINT('Ctrl Pts',(14.4999999999905,-24.4,-8.09493439800042));
#142090=CARTESIAN_POINT('Ctrl Pts',(14.3615288225489,-24.4,-7.97528104708893));
#142091=CARTESIAN_POINT('Ctrl Pts',(14.2230576451072,-24.4,-7.85562769617744));
#142092=CARTESIAN_POINT('Ctrl Pts',(14.0419866251341,-24.4,-7.88216968352437));
#142093=CARTESIAN_POINT('',(14.0419866251341,-24.4,-7.88216968352437));
#142094=CARTESIAN_POINT('',(13.9839732502781,-24.,-7.48639898180705));
#142095=CARTESIAN_POINT('Origin',(14.0419866251341,-24.,-7.88216968352437));
#142096=CARTESIAN_POINT('Origin',(14.0999999999902,-24.,-8.27794038524168));
#142097=CARTESIAN_POINT('Origin',(14.0999999999902,-24.4,-8.27794038524168));
#142098=CARTESIAN_POINT('Origin',(9.25,-24.,-3.05000000003699));
#142099=CARTESIAN_POINT('',(11.7393688126037,-24.,-8.17767422085447));
#142100=CARTESIAN_POINT('',(11.9140613608566,-24.4,-8.53751100828026));
#142101=CARTESIAN_POINT('Origin',(11.9140613608566,-24.,-8.53751100828026));
#142102=CARTESIAN_POINT('',(10.5587573250099,-24.4,-9.00794883031683));
#142103=CARTESIAN_POINT('Origin',(9.25,-24.4,-3.05000000003699));
#142104=CARTESIAN_POINT('',(10.4729371725502,-24.,-8.61726366111815));
#142105=CARTESIAN_POINT('Origin',(10.5587573250099,-24.,-9.00794883031683));
#142106=CARTESIAN_POINT('Origin',(9.25,-24.,-3.05000000003699));
#142107=CARTESIAN_POINT('Ctrl Pts',(10.4729371725502,-24.,-8.61726366111815));
#142108=CARTESIAN_POINT('Ctrl Pts',(10.1641684413763,-24.,-8.68508957741407));
#142109=CARTESIAN_POINT('Ctrl Pts',(10.0455250613722,-24.,-8.97811215786373));
#142110=CARTESIAN_POINT('Ctrl Pts',(9.92688168136818,-24.,-9.27113473831338));
#142111=CARTESIAN_POINT('Ctrl Pts',(10.1014821344353,-24.,-9.53467442424495));
#142112=CARTESIAN_POINT('Ctrl Pts',(10.4729371725502,-24.4,-8.61726366111815));
#142113=CARTESIAN_POINT('Ctrl Pts',(10.1641684413763,-24.4,-8.68508957741407));
#142114=CARTESIAN_POINT('Ctrl Pts',(10.0455250613722,-24.4,-8.97811215786373));
#142115=CARTESIAN_POINT('Ctrl Pts',(9.92688168136818,-24.4,-9.27113473831338));
#142116=CARTESIAN_POINT('Ctrl Pts',(10.1014821344353,-24.4,-9.53467442424495));
#142117=CARTESIAN_POINT('Ctrl Pts',(10.5587573250099,-24.4,-9.00794883031683));
#142118=CARTESIAN_POINT('Ctrl Pts',(10.4558344146186,-24.4,-9.03055746908214));
#142119=CARTESIAN_POINT('Ctrl Pts',(10.4162866212839,-24.4,-9.12823166256536));
#142120=CARTESIAN_POINT('Ctrl Pts',(10.3767388279492,-24.4,-9.22590585604857));
#142121=CARTESIAN_POINT('Ctrl Pts',(10.4349389789716,-24.4,-9.31375241802576));
#142122=CARTESIAN_POINT('',(10.4349389789716,-24.4,-9.31375241802576));
#142123=CARTESIAN_POINT('',(10.1014821344353,-24.,-9.53467442424495));
#142124=CARTESIAN_POINT('Origin',(10.4349389789716,-24.,-9.31375241802576));
#142125=CARTESIAN_POINT('Origin',(10.6016674012397,-24.,-9.20329141491617));
#142126=CARTESIAN_POINT('Origin',(10.6016674012397,-24.4,-9.20329141491617));
#142127=CARTESIAN_POINT('Origin',(6.1,-24.,-12.1857384988752));
#142128=CARTESIAN_POINT('',(11.3,-24.4,-12.1857384988752));
#142129=CARTESIAN_POINT('',(10.9,-24.,-12.1857384988752));
#142130=CARTESIAN_POINT('Origin',(11.3,-24.,-12.1857384988752));
#142131=CARTESIAN_POINT('Origin',(6.1,-24.,-12.1857384988752));
#142132=CARTESIAN_POINT('Origin',(6.1,-24.4,-12.1857384988752));
#142133=CARTESIAN_POINT('Origin',(11.3,-24.,-7.32500000002662));
#142134=CARTESIAN_POINT('',(10.9,-24.,-12.5077037206369));
#142135=CARTESIAN_POINT('Origin',(11.3,-24.,-12.5077037206369));
#142136=CARTESIAN_POINT('',(10.9,-24.,-7.32500000002662));
#142137=CARTESIAN_POINT('',(11.3,-24.4,-7.32500000002662));
#142138=CARTESIAN_POINT('Origin',(15.1,-24.,-15.1));
#142139=CARTESIAN_POINT('Origin',(15.1,-24.,-15.1));
#142140=CARTESIAN_POINT('Origin',(15.1,-24.4,-15.1));
#142141=CARTESIAN_POINT('Origin',(11.3,-24.,-12.5077037206369));
#142142=CARTESIAN_POINT('Origin',(11.3,-24.,-12.5077037206369));
#142143=CARTESIAN_POINT('Origin',(17.9686291501015,-23.,-11.7813708499319));
#142144=CARTESIAN_POINT('',(15.1343145750407,-22.1,-8.94705627487116));
#142145=CARTESIAN_POINT('',(15.1343145750407,-23.,-8.94705627487115));
#142146=CARTESIAN_POINT('',(15.7218887667622,-22.1,-9.53463046659261));
#142147=CARTESIAN_POINT('',(17.9686291501015,-22.1,-11.7813708499319));
#142148=CARTESIAN_POINT('',(15.7218887667622,-22.1,-9.53463046659261));
#142149=CARTESIAN_POINT('Origin',(15.69999999999,-23.,-8.38137084992192));
#142150=CARTESIAN_POINT('',(14.89999999999,-22.1,-8.38137084992041));
#142151=CARTESIAN_POINT('',(14.89999999999,-23.,-8.38137084992041));
#142152=CARTESIAN_POINT('Origin',(15.69999999999,-22.1,-8.38137084992192));
#142153=CARTESIAN_POINT('Origin',(14.899999999995,-24.,-5.70716730244972));
#142154=CARTESIAN_POINT('',(14.8999999999902,-22.1,-8.27794038524318));
#142155=CARTESIAN_POINT('',(14.8999999999902,-22.1,-8.27794038524318));
#142156=CARTESIAN_POINT('',(14.8999999999893,-22.1,-8.71274169981977));
#142157=CARTESIAN_POINT('Origin',(14.0999999999902,-22.1,-8.27794038524168));
#142158=CARTESIAN_POINT('',(13.9839732502781,-22.1,-7.48639898180705));
#142159=CARTESIAN_POINT('',(13.9839732502781,-22.1,-7.48639898180705));
#142160=CARTESIAN_POINT('Origin',(14.0999999999902,-22.1,-8.27794038524168));
#142161=CARTESIAN_POINT('Origin',(15.1,-22.1,-15.1));
#142162=CARTESIAN_POINT('',(11.7393688126037,-22.1,-8.17767422085447));
#142163=CARTESIAN_POINT('',(11.7393688126037,-22.1,-8.17767422085447));
#142164=CARTESIAN_POINT('Origin',(15.1,-22.1,-15.1));
#142165=CARTESIAN_POINT('Origin',(9.25,-22.1,-3.05000000003699));
#142166=CARTESIAN_POINT('',(10.4729371725502,-22.1,-8.61726366111815));
#142167=CARTESIAN_POINT('',(10.4729371725502,-22.1,-8.61726366111815));
#142168=CARTESIAN_POINT('Origin',(9.25,-22.1,-3.05000000003699));
#142169=CARTESIAN_POINT('Origin',(-3.45175358661618,-24.4,-3.05000000003699));
#142170=CARTESIAN_POINT('Origin',(17.1,-24.,0.396768100868128));
#142171=CARTESIAN_POINT('',(17.5,-24.,5.54411254966196));
#142172=CARTESIAN_POINT('',(17.1,-24.4,5.54411254966196));
#142173=CARTESIAN_POINT('Origin',(17.1,-24.,5.54411254966196));
#142174=CARTESIAN_POINT('',(17.1,-24.4,11.));
#142175=CARTESIAN_POINT('',(17.1,-24.4,0.396768100868128));
#142176=CARTESIAN_POINT('',(17.5,-24.,11.));
#142177=CARTESIAN_POINT('Origin',(17.1,-24.,11.));
#142178=CARTESIAN_POINT('',(17.5,-24.,0.396768100868128));
#142179=CARTESIAN_POINT('Ctrl Pts',(17.5,-24.,11.));
#142180=CARTESIAN_POINT('Ctrl Pts',(17.5,-24.,11.6));
#142181=CARTESIAN_POINT('Ctrl Pts',(16.9,-24.,11.6));
#142182=CARTESIAN_POINT('Ctrl Pts',(17.5,-24.4,11.));
#142183=CARTESIAN_POINT('Ctrl Pts',(17.5,-24.4,11.6));
#142184=CARTESIAN_POINT('Ctrl Pts',(16.9,-24.4,11.6));
#142185=CARTESIAN_POINT('Ctrl Pts',(17.1,-24.4,11.));
#142186=CARTESIAN_POINT('Ctrl Pts',(17.1,-24.4,11.2));
#142187=CARTESIAN_POINT('Ctrl Pts',(16.9,-24.4,11.2));
#142188=CARTESIAN_POINT('',(16.9,-24.4,11.2));
#142189=CARTESIAN_POINT('',(16.9,-24.,11.6));
#142190=CARTESIAN_POINT('Origin',(16.9,-24.,11.2));
#142191=CARTESIAN_POINT('Origin',(16.9,-24.,11.));
#142192=CARTESIAN_POINT('Origin',(16.9,-24.4,11.));
#142193=CARTESIAN_POINT('Origin',(7.02412320669191,-24.,11.2));
#142194=CARTESIAN_POINT('',(16.3999999999996,-24.4,11.2));
#142195=CARTESIAN_POINT('',(16.3999999999996,-24.,11.6));
#142196=CARTESIAN_POINT('Origin',(16.3999999999996,-24.,11.2));
#142197=CARTESIAN_POINT('',(7.02412320669191,-24.,11.6));
#142198=CARTESIAN_POINT('',(7.02412320669191,-24.4,11.2));
#142199=CARTESIAN_POINT('Origin',(16.3999999999996,-24.,15.7));
#142200=CARTESIAN_POINT('',(14.5808510638294,-24.4,11.5840921842161));
#142201=CARTESIAN_POINT('',(14.742553191489,-24.,11.9499506567302));
#142202=CARTESIAN_POINT('Origin',(14.5808510638294,-24.,11.5840921842161));
#142203=CARTESIAN_POINT('Origin',(16.3999999999996,-24.,15.7));
#142204=CARTESIAN_POINT('Origin',(16.3999999999996,-24.4,15.7));
#142205=CARTESIAN_POINT('Ctrl Pts',(14.742553191489,-24.,11.9499506567302));
#142206=CARTESIAN_POINT('Ctrl Pts',(14.4450678125079,-24.,12.0814332445142));
#142207=CARTESIAN_POINT('Ctrl Pts',(14.1725339062537,-24.,11.9039212969169));
#142208=CARTESIAN_POINT('Ctrl Pts',(13.8999999999996,-24.,11.7264093493195));
#142209=CARTESIAN_POINT('Ctrl Pts',(13.8999999999996,-24.,11.401162947959));
#142210=CARTESIAN_POINT('Ctrl Pts',(14.742553191489,-24.4,11.9499506567302));
#142211=CARTESIAN_POINT('Ctrl Pts',(14.4450678125079,-24.4,12.0814332445142));
#142212=CARTESIAN_POINT('Ctrl Pts',(14.1725339062537,-24.4,11.9039212969169));
#142213=CARTESIAN_POINT('Ctrl Pts',(13.8999999999996,-24.4,11.7264093493195));
#142214=CARTESIAN_POINT('Ctrl Pts',(13.8999999999996,-24.4,11.401162947959));
#142215=CARTESIAN_POINT('Ctrl Pts',(14.5808510638294,-24.4,11.5840921842161));
#142216=CARTESIAN_POINT('Ctrl Pts',(14.4816892708357,-24.4,11.6279197134774));
#142217=CARTESIAN_POINT('Ctrl Pts',(14.3908446354177,-24.4,11.5687490642783));
#142218=CARTESIAN_POINT('Ctrl Pts',(14.2999999999996,-24.4,11.5095784150792));
#142219=CARTESIAN_POINT('Ctrl Pts',(14.2999999999996,-24.4,11.401162947959));
#142220=CARTESIAN_POINT('',(14.2999999999996,-24.4,11.401162947959));
#142221=CARTESIAN_POINT('',(13.8999999999996,-24.,11.401162947959));
#142222=CARTESIAN_POINT('Origin',(14.2999999999996,-24.,11.401162947959));
#142223=CARTESIAN_POINT('Origin',(14.4999999999996,-24.,11.401162947959));
#142224=CARTESIAN_POINT('Origin',(14.4999999999996,-24.4,11.401162947959));
#142225=CARTESIAN_POINT('Origin',(14.2999999999999,-24.,-0.800000000036603));
#142226=CARTESIAN_POINT('',(14.2999999999997,-24.4,9.24999999996345));
#142227=CARTESIAN_POINT('',(13.8999999999997,-24.,9.24999999996345));
#142228=CARTESIAN_POINT('Origin',(14.2999999999997,-24.,9.24999999996345));
#142229=CARTESIAN_POINT('',(13.8999999999999,-24.,-0.80000000003661));
#142230=CARTESIAN_POINT('',(14.2999999999999,-24.4,-0.800000000036603));
#142231=CARTESIAN_POINT('Origin',(6.09999999999969,-24.,9.2499999999633));
#142232=CARTESIAN_POINT('',(12.8526992139868,-24.4,4.59800544650364));
#142233=CARTESIAN_POINT('',(12.5232992523289,-24.,4.82493201008704));
#142234=CARTESIAN_POINT('Origin',(12.8526992139868,-24.,4.59800544650364));
#142235=CARTESIAN_POINT('Origin',(6.09999999999969,-24.,9.2499999999633));
#142236=CARTESIAN_POINT('Origin',(6.09999999999969,-24.4,9.2499999999633));
#142237=CARTESIAN_POINT('Ctrl Pts',(12.5232992523289,-24.,4.82493201008704));
#142238=CARTESIAN_POINT('Ctrl Pts',(12.3051223920045,-24.,4.50823286173429));
#142239=CARTESIAN_POINT('Ctrl Pts',(12.5017731872981,-24.,4.17773632974227));
#142240=CARTESIAN_POINT('Ctrl Pts',(12.6984239825917,-24.,3.84723979775026));
#142241=CARTESIAN_POINT('Ctrl Pts',(13.080844887153,-24.,3.88790605775575));
#142242=CARTESIAN_POINT('Ctrl Pts',(12.5232992523289,-24.4,4.82493201008704));
#142243=CARTESIAN_POINT('Ctrl Pts',(12.3051223920045,-24.4,4.50823286173429));
#142244=CARTESIAN_POINT('Ctrl Pts',(12.5017731872981,-24.4,4.17773632974227));
#142245=CARTESIAN_POINT('Ctrl Pts',(12.6984239825917,-24.4,3.84723979775026));
#142246=CARTESIAN_POINT('Ctrl Pts',(13.080844887153,-24.4,3.88790605775575));
#142247=CARTESIAN_POINT('Ctrl Pts',(12.8526992139868,-24.4,4.59800544650365));
#142248=CARTESIAN_POINT('Ctrl Pts',(12.7799735938787,-24.4,4.49243906371939));
#142249=CARTESIAN_POINT('Ctrl Pts',(12.8455238589765,-24.4,4.38227355305539));
#142250=CARTESIAN_POINT('Ctrl Pts',(12.9110741240744,-24.4,4.27210804239138));
#142251=CARTESIAN_POINT('Ctrl Pts',(13.0385477589281,-24.4,4.28566346239322));
#142252=CARTESIAN_POINT('',(13.0385477589281,-24.4,4.28566346239322));
#142253=CARTESIAN_POINT('',(13.080844887153,-24.,3.88790605775575));
#142254=CARTESIAN_POINT('Origin',(13.0385477589281,-24.,4.28566346239322));
#142255=CARTESIAN_POINT('Origin',(13.0173991948157,-24.,4.48454216471195));
#142256=CARTESIAN_POINT('Origin',(13.0173991948157,-24.4,4.48454216471195));
#142257=CARTESIAN_POINT('Origin',(15.1,-24.,-15.1));
#142258=CARTESIAN_POINT('',(15.9166307959896,-24.4,4.37785017301522));
#142259=CARTESIAN_POINT('',(15.899875065829,-24.,3.97820127021829));
#142260=CARTESIAN_POINT('Origin',(15.9166307959896,-24.,4.37785017301522));
#142261=CARTESIAN_POINT('Origin',(15.1,-24.,-15.1));
#142262=CARTESIAN_POINT('Origin',(15.1,-24.4,-15.1));
#142263=CARTESIAN_POINT('Ctrl Pts',(15.899875065829,-24.,3.97820127021829));
#142264=CARTESIAN_POINT('Ctrl Pts',(16.2507487943837,-24.,3.9634904941472));
#142265=CARTESIAN_POINT('Ctrl Pts',(16.4990719510994,-24.,4.2118136508629));
#142266=CARTESIAN_POINT('Ctrl Pts',(15.899875065829,-24.4,3.97820127021829));
#142267=CARTESIAN_POINT('Ctrl Pts',(16.2507487943837,-24.4,3.9634904941472));
#142268=CARTESIAN_POINT('Ctrl Pts',(16.4990719510994,-24.4,4.2118136508629));
#142269=CARTESIAN_POINT('Ctrl Pts',(15.9166307959896,-24.4,4.37785017301522));
#142270=CARTESIAN_POINT('Ctrl Pts',(16.0920676602669,-24.4,4.37049478497967));
#142271=CARTESIAN_POINT('Ctrl Pts',(16.2162292386248,-24.4,4.49465636333752));
#142272=CARTESIAN_POINT('',(16.2162292386248,-24.4,4.49465636333752));
#142273=CARTESIAN_POINT('',(16.4990719510994,-24.,4.2118136508629));
#142274=CARTESIAN_POINT('Origin',(16.2162292386248,-24.,4.49465636333752));
#142275=CARTESIAN_POINT('Origin',(15.9333865261502,-24.,4.77749907581214));
#142276=CARTESIAN_POINT('Origin',(15.9333865261502,-24.4,4.77749907581214));
#142277=CARTESIAN_POINT('Origin',(8.90268758620957,-24.,-2.81888528907772));
#142278=CARTESIAN_POINT('',(16.9828427124746,-24.4,5.26126983718734));
#142279=CARTESIAN_POINT('',(17.2656854249492,-24.,4.97842712471272));
#142280=CARTESIAN_POINT('Origin',(16.9828427124746,-24.,5.26126983718734));
#142281=CARTESIAN_POINT('',(9.18553029868418,-24.,-3.10172800155234));
#142282=CARTESIAN_POINT('',(8.90268758620957,-24.4,-2.81888528907772));
#142283=CARTESIAN_POINT('Ctrl Pts',(17.2656854249492,-24.,4.97842712471272));
#142284=CARTESIAN_POINT('Ctrl Pts',(17.5,-24.,5.21274169976348));
#142285=CARTESIAN_POINT('Ctrl Pts',(17.5,-24.,5.54411254966196));
#142286=CARTESIAN_POINT('Ctrl Pts',(17.2656854249492,-24.4,4.97842712471272));
#142287=CARTESIAN_POINT('Ctrl Pts',(17.5,-24.4,5.21274169976348));
#142288=CARTESIAN_POINT('Ctrl Pts',(17.5,-24.4,5.54411254966196));
#142289=CARTESIAN_POINT('Ctrl Pts',(16.9828427124746,-24.4,5.26126983718734));
#142290=CARTESIAN_POINT('Ctrl Pts',(17.1,-24.4,5.37842712471272));
#142291=CARTESIAN_POINT('Ctrl Pts',(17.1,-24.4,5.54411254966196));
#142292=CARTESIAN_POINT('Origin',(16.7,-24.,5.54411254966196));
#142293=CARTESIAN_POINT('Origin',(16.7,-24.4,5.54411254966196));
#142294=CARTESIAN_POINT('Origin',(13.0173991948157,-22.1,4.48454216471195));
#142295=CARTESIAN_POINT('',(13.080844887153,-22.1,3.88790605775575));
#142296=CARTESIAN_POINT('',(13.080844887153,-22.1,3.88790605775575));
#142297=CARTESIAN_POINT('',(12.5232992523289,-22.1,4.82493201008704));
#142298=CARTESIAN_POINT('Origin',(13.0173991948157,-22.1,4.48454216471195));
#142299=CARTESIAN_POINT('',(12.5232992523289,-22.1,4.82493201008704));
#142300=CARTESIAN_POINT('Origin',(15.1,-22.1,-15.1));
#142301=CARTESIAN_POINT('',(15.899875065829,-22.1,3.97820127021829));
#142302=CARTESIAN_POINT('',(15.899875065829,-22.1,3.97820127021829));
#142303=CARTESIAN_POINT('Origin',(15.1,-22.1,-15.1));
#142304=CARTESIAN_POINT('Origin',(15.9333865261502,-22.1,4.77749907581214));
#142305=CARTESIAN_POINT('',(16.4990719510994,-22.1,4.2118136508629));
#142306=CARTESIAN_POINT('',(16.4990719510994,-22.1,4.2118136508629));
#142307=CARTESIAN_POINT('Origin',(15.9333865261502,-22.1,4.77749907581214));
#142308=CARTESIAN_POINT('Origin',(15.4783082405767,-23.,3.19104994034017));
#142309=CARTESIAN_POINT('',(17.2656854249492,-22.1,4.97842712471272));
#142310=CARTESIAN_POINT('',(17.2656854249492,-22.55,4.97842712471272));
#142311=CARTESIAN_POINT('',(14.9000000000107,-22.1,2.61274169977414));
#142312=CARTESIAN_POINT('Origin',(16.7,-22.55,5.54411254966196));
#142313=CARTESIAN_POINT('',(17.5,-22.1,5.54411254966196));
#142314=CARTESIAN_POINT('',(17.5,-22.55,5.54411254966196));
#142315=CARTESIAN_POINT('Origin',(16.7,-22.1,5.54411254966196));
#142316=CARTESIAN_POINT('Origin',(17.5,-22.1,3.84353620177326));
#142317=CARTESIAN_POINT('',(17.5,-22.1,11.));
#142318=CARTESIAN_POINT('',(17.5,-22.1,11.));
#142319=CARTESIAN_POINT('',(17.5,-22.1,1.69676810087534));
#142320=CARTESIAN_POINT('Origin',(-3.45175358661618,-24.4,-3.05000000003699));
#142321=CARTESIAN_POINT('Origin',(0.999999999210583,-24.,-4.75788611936281));
#142322=CARTESIAN_POINT('',(0.599999999210584,-24.,-0.0238638518621566));
#142323=CARTESIAN_POINT('',(0.999999999210584,-24.4,-0.0238638518621564));
#142324=CARTESIAN_POINT('Origin',(0.999999999210584,-24.,-0.0238638518621564));
#142325=CARTESIAN_POINT('',(0.999999999210583,-24.4,-1.85000000003699));
#142326=CARTESIAN_POINT('',(0.999999999210583,-24.4,-4.75788611936281));
#142327=CARTESIAN_POINT('',(0.599999999210584,-24.,-1.85000000003699));
#142328=CARTESIAN_POINT('Origin',(0.999999999210583,-24.,-1.85000000003699));
#142329=CARTESIAN_POINT('',(0.599999999210583,-24.,-4.75788611936281));
#142330=CARTESIAN_POINT('Ctrl Pts',(0.599999999210584,-24.,-1.85000000003699));
#142331=CARTESIAN_POINT('Ctrl Pts',(0.599999999210584,-24.,-2.45000000003699));
#142332=CARTESIAN_POINT('Ctrl Pts',(1.19999999921058,-24.,-2.45000000003699));
#142333=CARTESIAN_POINT('Ctrl Pts',(0.599999999210584,-24.4,-1.85000000003699));
#142334=CARTESIAN_POINT('Ctrl Pts',(0.599999999210584,-24.4,-2.45000000003699));
#142335=CARTESIAN_POINT('Ctrl Pts',(1.19999999921058,-24.4,-2.45000000003699));
#142336=CARTESIAN_POINT('Ctrl Pts',(0.999999999210584,-24.4,-1.85000000003699));
#142337=CARTESIAN_POINT('Ctrl Pts',(0.999999999210584,-24.4,-2.05000000003699));
#142338=CARTESIAN_POINT('Ctrl Pts',(1.19999999921058,-24.4,-2.05000000003699));
#142339=CARTESIAN_POINT('',(1.19999999921058,-24.4,-2.05000000003699));
#142340=CARTESIAN_POINT('',(1.19999999921058,-24.,-2.45000000003699));
#142341=CARTESIAN_POINT('Origin',(1.19999999921058,-24.,-2.05000000003699));
#142342=CARTESIAN_POINT('Origin',(1.19999999921058,-24.,-1.85000000003699));
#142343=CARTESIAN_POINT('Origin',(1.19999999921058,-24.4,-1.85000000003699));
#142344=CARTESIAN_POINT('Origin',(-4.69720428956801,-24.,-2.05000000003699));
#142345=CARTESIAN_POINT('',(4.3,-24.4,-2.05000000003699));
#142346=CARTESIAN_POINT('',(4.3,-24.,-2.45000000003699));
#142347=CARTESIAN_POINT('Origin',(4.3,-24.,-2.05000000003699));
#142348=CARTESIAN_POINT('',(-4.69720428956801,-24.,-2.45000000003699));
#142349=CARTESIAN_POINT('',(-4.69720428956801,-24.4,-2.05000000003699));
#142350=CARTESIAN_POINT('Ctrl Pts',(4.3,-24.,-2.45000000003699));
#142351=CARTESIAN_POINT('Ctrl Pts',(4.9,-24.,-2.45000000003699));
#142352=CARTESIAN_POINT('Ctrl Pts',(4.9,-24.,-1.85000000003699));
#142353=CARTESIAN_POINT('Ctrl Pts',(4.3,-24.4,-2.45000000003699));
#142354=CARTESIAN_POINT('Ctrl Pts',(4.9,-24.4,-2.45000000003699));
#142355=CARTESIAN_POINT('Ctrl Pts',(4.9,-24.4,-1.85000000003699));
#142356=CARTESIAN_POINT('Ctrl Pts',(4.3,-24.4,-2.05000000003699));
#142357=CARTESIAN_POINT('Ctrl Pts',(4.5,-24.4,-2.05000000003699));
#142358=CARTESIAN_POINT('Ctrl Pts',(4.5,-24.4,-1.85000000003699));
#142359=CARTESIAN_POINT('',(4.5,-24.4,-1.85000000003699));
#142360=CARTESIAN_POINT('',(4.9,-24.,-1.85000000003699));
#142361=CARTESIAN_POINT('Origin',(4.5,-24.,-1.85000000003699));
#142362=CARTESIAN_POINT('Origin',(4.3,-24.,-1.85000000003699));
#142363=CARTESIAN_POINT('Origin',(4.3,-24.4,-1.85000000003699));
#142364=CARTESIAN_POINT('Origin',(4.5,-24.,-4.18858360955962));
#142365=CARTESIAN_POINT('',(4.5,-24.4,-0.74199679747406));
#142366=CARTESIAN_POINT('',(4.9,-24.,-0.74199679747406));
#142367=CARTESIAN_POINT('Origin',(4.5,-24.,-0.74199679747406));
#142368=CARTESIAN_POINT('',(4.9,-24.,-4.18858360955962));
#142369=CARTESIAN_POINT('',(4.5,-24.4,-4.18858360955962));
#142370=CARTESIAN_POINT('Origin',(8.6,-24.,-0.741996797474058));
#142371=CARTESIAN_POINT('',(7.60485436893191,-24.4,3.23539998597188));
#142372=CARTESIAN_POINT('',(7.7019417475727,-24.,2.84736127539179));
#142373=CARTESIAN_POINT('Origin',(7.60485436893191,-24.,3.23539998597188));
#142374=CARTESIAN_POINT('Origin',(8.6,-24.,-0.741996797474058));
#142375=CARTESIAN_POINT('Origin',(8.6,-24.4,-0.741996797474058));
#142376=CARTESIAN_POINT('Origin',(6.09999999999969,-24.,9.2499999999633));
#142377=CARTESIAN_POINT('',(11.6600331084108,-24.4,6.50663858859724));
#142378=CARTESIAN_POINT('',(12.0187449218567,-24.,6.32964752979943));
#142379=CARTESIAN_POINT('Origin',(11.6600331084108,-24.,6.50663858859724));
#142380=CARTESIAN_POINT('Origin',(6.09999999999969,-24.,9.2499999999633));
#142381=CARTESIAN_POINT('Origin',(6.09999999999969,-24.4,9.2499999999633));
#142382=CARTESIAN_POINT('Ctrl Pts',(12.0187449218567,-24.,6.32964752979943));
#142383=CARTESIAN_POINT('Ctrl Pts',(12.1810106563356,-24.,6.65851519277877));
#142384=CARTESIAN_POINT('Ctrl Pts',(11.9623390923243,-24.,6.9529075422587));
#142385=CARTESIAN_POINT('Ctrl Pts',(11.7436675283129,-24.,7.24729989173863));
#142386=CARTESIAN_POINT('Ctrl Pts',(11.381945787434,-24.,7.18695512796406));
#142387=CARTESIAN_POINT('Ctrl Pts',(12.0187449218567,-24.4,6.32964752979943));
#142388=CARTESIAN_POINT('Ctrl Pts',(12.1810106563356,-24.4,6.65851519277877));
#142389=CARTESIAN_POINT('Ctrl Pts',(11.9623390923243,-24.4,6.9529075422587));
#142390=CARTESIAN_POINT('Ctrl Pts',(11.7436675283129,-24.4,7.24729989173863));
#142391=CARTESIAN_POINT('Ctrl Pts',(11.381945787434,-24.4,7.18695512796406));
#142392=CARTESIAN_POINT('Ctrl Pts',(11.6600331084108,-24.4,6.50663858859724));
#142393=CARTESIAN_POINT('Ctrl Pts',(11.7141216865704,-24.4,6.61626114292369));
#142394=CARTESIAN_POINT('Ctrl Pts',(11.6412311652333,-24.4,6.71439192608367));
#142395=CARTESIAN_POINT('Ctrl Pts',(11.5683406438962,-24.4,6.81252270924365));
#142396=CARTESIAN_POINT('Ctrl Pts',(11.4477667302699,-24.4,6.79240778798545));
#142397=CARTESIAN_POINT('',(11.4477667302699,-24.4,6.79240778798545));
#142398=CARTESIAN_POINT('',(11.381945787434,-24.,7.18695512796406));
#142399=CARTESIAN_POINT('Origin',(11.4477667302699,-24.,6.79240778798545));
#142400=CARTESIAN_POINT('Origin',(11.4806772016879,-24.,6.59513411799615));
#142401=CARTESIAN_POINT('Origin',(11.4806772016879,-24.4,6.59513411799615));
#142402=CARTESIAN_POINT('Origin',(15.1,-24.,-15.1));
#142403=CARTESIAN_POINT('',(5.40676393843642,-24.4,4.86640932333035));
#142404=CARTESIAN_POINT('',(5.23207139018353,-24.,5.22624611075613));
#142405=CARTESIAN_POINT('Origin',(5.40676393843642,-24.,4.86640932333035));
#142406=CARTESIAN_POINT('Origin',(15.1,-24.,-15.1));
#142407=CARTESIAN_POINT('Origin',(15.1,-24.4,-15.1));
#142408=CARTESIAN_POINT('Origin',(9.25,-24.,-3.05000000003699));
#142409=CARTESIAN_POINT('',(1.01279069686664,-24.4,0.0465114073977232));
#142410=CARTESIAN_POINT('',(0.638372092178764,-24.,0.187261925917483));
#142411=CARTESIAN_POINT('Origin',(1.01279069686664,-24.,0.0465114073977232));
#142412=CARTESIAN_POINT('Origin',(9.25,-24.,-3.05000000003699));
#142413=CARTESIAN_POINT('Origin',(9.25,-24.4,-3.05000000003699));
#142414=CARTESIAN_POINT('Ctrl Pts',(0.638372092178765,-24.,0.187261925917483));
#142415=CARTESIAN_POINT('Ctrl Pts',(0.599999999210585,-24.,0.0851860994182524));
#142416=CARTESIAN_POINT('Ctrl Pts',(0.599999999210585,-24.,-0.0238638518621567));
#142417=CARTESIAN_POINT('Ctrl Pts',(0.638372092178765,-24.4,0.187261925917482));
#142418=CARTESIAN_POINT('Ctrl Pts',(0.599999999210585,-24.4,0.0851860994182523));
#142419=CARTESIAN_POINT('Ctrl Pts',(0.599999999210585,-24.4,-0.0238638518621568));
#142420=CARTESIAN_POINT('Ctrl Pts',(1.01279069686665,-24.4,0.0465114073977229));
#142421=CARTESIAN_POINT('Ctrl Pts',(0.999999999210585,-24.4,0.0124861318979795));
#142422=CARTESIAN_POINT('Ctrl Pts',(0.999999999210585,-24.4,-0.0238638518621568));
#142423=CARTESIAN_POINT('Origin',(1.19999999921058,-24.,-0.0238638518621567));
#142424=CARTESIAN_POINT('Origin',(1.19999999921058,-24.4,-0.0238638518621568));
#142425=CARTESIAN_POINT('Origin',(6.09999999999969,-19.9,9.2499999999633));
#142426=CARTESIAN_POINT('',(12.0187449218567,-20.,6.32964752979944));
#142427=CARTESIAN_POINT('',(12.0187449218567,-19.9,6.32964752979943));
#142428=CARTESIAN_POINT('',(7.7019417475727,-20.,2.84736127539179));
#142429=CARTESIAN_POINT('Origin',(6.09999999999969,-20.,9.2499999999633));
#142430=CARTESIAN_POINT('',(7.7019417475727,-19.9,2.84736127539179));
#142431=CARTESIAN_POINT('Origin',(11.4806772016879,-19.9,6.59513411799615));
#142432=CARTESIAN_POINT('',(11.381945787434,-20.,7.18695512796406));
#142433=CARTESIAN_POINT('',(11.381945787434,-19.9,7.18695512796406));
#142434=CARTESIAN_POINT('Origin',(11.4806772016879,-20.,6.59513411799615));
#142435=CARTESIAN_POINT('Origin',(15.1,-19.9,-15.1));
#142436=CARTESIAN_POINT('',(5.23207139018353,-15.9,5.22624611075614));
#142437=CARTESIAN_POINT('',(5.23207139018353,-19.9,5.22624611075614));
#142438=CARTESIAN_POINT('',(13.3925518029794,-15.9,7.43035544899269));
#142439=CARTESIAN_POINT('Origin',(15.1,-15.9,-15.1));
#142440=CARTESIAN_POINT('',(13.3925518029794,-20.,7.43035544899269));
#142441=CARTESIAN_POINT('',(13.3925518029795,-19.9,7.43035544899269));
#142442=CARTESIAN_POINT('Origin',(15.1,-20.,-15.1));
#142443=CARTESIAN_POINT('Origin',(9.25,-21.1,-3.05000000003699));
#142444=CARTESIAN_POINT('',(0.638372092178764,-20.,0.187261925917484));
#142445=CARTESIAN_POINT('',(0.638372092178764,-21.1,0.187261925917483));
#142446=CARTESIAN_POINT('',(0.159697928570087,-20.,-1.63352259105473));
#142447=CARTESIAN_POINT('Origin',(9.25,-20.,-3.05000000003699));
#142448=CARTESIAN_POINT('',(0.159697928570086,-19.2185290786118,-1.63352259105473));
#142449=CARTESIAN_POINT('',(0.159697928570086,-21.1,-1.63352259105473));
#142450=CARTESIAN_POINT('',(0.184164224908069,-19.1828954869493,-1.48455383390278));
#142451=CARTESIAN_POINT('Ctrl Pts',(0.184164224908773,-19.1828954869485,
-1.48455383389902));
#142452=CARTESIAN_POINT('Ctrl Pts',(0.181353760516264,-19.1834220810812,
-1.50082983826466));
#142453=CARTESIAN_POINT('Ctrl Pts',(0.178601777697792,-19.1849707452015,
-1.51707236850617));
#142454=CARTESIAN_POINT('Ctrl Pts',(0.175910270632949,-19.1875443857133,
-1.53316372260399));
#142455=CARTESIAN_POINT('Ctrl Pts',(0.174241610022826,-19.1891399722911,
-1.54313992110531));
#142456=CARTESIAN_POINT('Ctrl Pts',(0.172597130274316,-19.1911297373904,
-1.55305778148705));
#142457=CARTESIAN_POINT('Ctrl Pts',(0.170986625987962,-19.1935166139609,
-1.56288598586302));
#142458=CARTESIAN_POINT('Ctrl Pts',(0.16828963437131,-19.1975137384361,
-1.57934454796268));
#142459=CARTESIAN_POINT('Ctrl Pts',(0.165686978366581,-19.2026151899126,
-1.59551812123727));
#142460=CARTESIAN_POINT('Ctrl Pts',(0.163189474647243,-19.2088472856758,
-1.61127304108951));
#142461=CARTESIAN_POINT('Ctrl Pts',(0.162001044626545,-19.2118128106676,
-1.61876997476017));
#142462=CARTESIAN_POINT('Ctrl Pts',(0.16083686547626,-19.2150346144176,
-1.62617154830696));
#142463=CARTESIAN_POINT('Ctrl Pts',(0.159700282405873,-19.2185167914062,
-1.63346006998121));
#142464=CARTESIAN_POINT('',(0.506210580792261,-17.3375900928828,-0.188855719761902));
#142465=CARTESIAN_POINT('Ctrl Pts',(0.506210580792261,-17.3375900928828,
-0.188855719761907));
#142466=CARTESIAN_POINT('Ctrl Pts',(0.580278907014156,-17.381066136149,
0.0375005152529757));
#142467=CARTESIAN_POINT('Ctrl Pts',(0.669274719311132,-17.4473071571919,
0.274849655756337));
#142468=CARTESIAN_POINT('Ctrl Pts',(0.792548014213962,-17.586657437599,
0.572772974625153));
#142469=CARTESIAN_POINT('Ctrl Pts',(0.845006682143812,-17.6581943501699,
0.692397462978445));
#142470=CARTESIAN_POINT('Ctrl Pts',(0.914713320592898,-17.7910311183224,
0.844601700992352));
#142471=CARTESIAN_POINT('Ctrl Pts',(0.944350360166487,-17.8608514992075,
0.907096140123004));
#142472=CARTESIAN_POINT('Ctrl Pts',(0.976481807510859,-17.9804818034157,
0.973618150343783));
#142473=CARTESIAN_POINT('Ctrl Pts',(0.985172457114319,-18.0228461575066,
0.991385474329735));
#142474=CARTESIAN_POINT('Ctrl Pts',(0.996932135198067,-18.1102055287159,
1.01534824533723));
#142475=CARTESIAN_POINT('Ctrl Pts',(1.,-18.1551996258224,1.02154761727023));
#142476=CARTESIAN_POINT('Ctrl Pts',(1.,-18.2,1.02154761727023));
#142477=CARTESIAN_POINT('Ctrl Pts',(1.,-18.2593850884882,1.02154761727022));
#142478=CARTESIAN_POINT('Ctrl Pts',(0.994695748169923,-18.3171214241364,
1.01084158300733));
#142479=CARTESIAN_POINT('Ctrl Pts',(0.972999971362076,-18.4411618339318,
0.966468917575704));
#142480=CARTESIAN_POINT('Ctrl Pts',(0.954670937162076,-18.5034679387583,
0.928689483412159));
#142481=CARTESIAN_POINT('Ctrl Pts',(0.8978478687292,-18.6513824418007,0.808562130066912));
#142482=CARTESIAN_POINT('Ctrl Pts',(0.853199148505529,-18.7268262065284,
0.711075214280202));
#142483=CARTESIAN_POINT('Ctrl Pts',(0.703337160928647,-18.9335978311899,
0.365553184470413));
#142484=CARTESIAN_POINT('Ctrl Pts',(0.584646620624056,-19.0181565122869,
0.055144231507496));
#142485=CARTESIAN_POINT('Ctrl Pts',(0.475205795724452,-19.0801011465358,
-0.284823424914531));
#142486=CARTESIAN_POINT('Ctrl Pts',(0.458257453044452,-19.0890086151428,
-0.339186673888201));
#142487=CARTESIAN_POINT('Ctrl Pts',(0.441807997660264,-19.0971096327671,
-0.393733136576476));
#142488=CARTESIAN_POINT('Ctrl Pts',(0.377329500084536,-19.1288639634147,
-0.607544103570025));
#142489=CARTESIAN_POINT('Ctrl Pts',(0.319510142661645,-19.1489487401334,
-0.828054390322394));
#142490=CARTESIAN_POINT('Ctrl Pts',(0.23834220554392,-19.1717559114687,
-1.19207823060078));
#142491=CARTESIAN_POINT('Ctrl Pts',(0.209486143478189,-19.1781509423164,
-1.33790915187365));
#142492=CARTESIAN_POINT('Ctrl Pts',(0.184164224908118,-19.1828954869486,
-1.48455383390281));
#142493=CARTESIAN_POINT('',(0.40335604954683,-17.2099042410653,-0.524749356257178));
#142494=CARTESIAN_POINT('Ctrl Pts',(0.403130429600274,-17.2100443552713,
-0.524549252433244));
#142495=CARTESIAN_POINT('Ctrl Pts',(0.407548590591942,-17.2208124362877,
-0.509132289531301));
#142496=CARTESIAN_POINT('Ctrl Pts',(0.412172338640691,-17.2307118184428,
-0.493157767087332));
#142497=CARTESIAN_POINT('Ctrl Pts',(0.416951623028926,-17.2398480136672,
-0.476819041514874));
#142498=CARTESIAN_POINT('Ctrl Pts',(0.418225874816477,-17.2422839040956,
-0.472462813976238));
#142499=CARTESIAN_POINT('Ctrl Pts',(0.419511363141136,-17.2446655122957,
-0.468080466407649));
#142500=CARTESIAN_POINT('Ctrl Pts',(0.420807513383204,-17.2469947858434,
-0.463675204646474));
#142501=CARTESIAN_POINT('Ctrl Pts',(0.426291621896912,-17.2568501162514,
-0.445036213003789));
#142502=CARTESIAN_POINT('Ctrl Pts',(0.43198280701597,-17.2658022765771,
-0.425926953399594));
#142503=CARTESIAN_POINT('Ctrl Pts',(0.437814431480213,-17.2739660976529,
-0.406566899304107));
#142504=CARTESIAN_POINT('Ctrl Pts',(0.439452911598933,-17.2762598424932,
-0.401127409171076));
#142505=CARTESIAN_POINT('Ctrl Pts',(0.441102768804601,-17.2784913221943,
-0.395667966425912));
#142506=CARTESIAN_POINT('Ctrl Pts',(0.442763141978182,-17.2806630452537,
-0.390193150631224));
#142507=CARTESIAN_POINT('Ctrl Pts',(0.449381559241047,-17.2893197554528,
-0.368369975008351));
#142508=CARTESIAN_POINT('Ctrl Pts',(0.456211562902522,-17.2970896099185,
-0.346146242590313));
#142509=CARTESIAN_POINT('Ctrl Pts',(0.463166341463394,-17.304076867005,
-0.323783362358173));
#142510=CARTESIAN_POINT('Ctrl Pts',(0.465562880074469,-17.3064845973513,
-0.316077364897278));
#142511=CARTESIAN_POINT('Ctrl Pts',(0.467974715975203,-17.3087993719827,
-0.308354963529586));
#142512=CARTESIAN_POINT('Ctrl Pts',(0.470399514304154,-17.3110254971623,
-0.300627410446533));
#142513=CARTESIAN_POINT('Ctrl Pts',(0.477253100275757,-17.3173175422038,
-0.27878582107703));
#142514=CARTESIAN_POINT('Ctrl Pts',(0.484291111603266,-17.322976955946,
-0.256640895596778));
#142515=CARTESIAN_POINT('Ctrl Pts',(0.491434018931853,-17.3280382086754,
-0.234423871949092));
#142516=CARTESIAN_POINT('Ctrl Pts',(0.496316244720445,-17.3314976093734,
-0.219238385030569));
#142517=CARTESIAN_POINT('Ctrl Pts',(0.501248496234294,-17.3346774875366,
-0.204020079963621));
#142518=CARTESIAN_POINT('Ctrl Pts',(0.506210580792283,-17.3375900928828,
-0.188855719761839));
#142519=CARTESIAN_POINT('',(0.159697928570089,-16.4335328638949,-1.63352259105473));
#142520=CARTESIAN_POINT('Origin',(9.25,-15.4417047044218,-3.05000000003699));
#142521=CARTESIAN_POINT('',(0.159697928570088,-15.9,-1.63352259105473));
#142522=CARTESIAN_POINT('',(0.159697928570087,-21.1,-1.63352259105473));
#142523=CARTESIAN_POINT('Origin',(9.25,-15.9,-3.05000000003699));
#142524=CARTESIAN_POINT('Origin',(1.19999999921058,-21.1,-0.0238638518621564));
#142525=CARTESIAN_POINT('',(0.599999999210584,-20.,-0.0238638518621564));
#142526=CARTESIAN_POINT('',(0.599999999210584,-21.1,-0.0238638518621563));
#142527=CARTESIAN_POINT('Origin',(1.19999999921058,-20.,-0.0238638518621563));
#142528=CARTESIAN_POINT('Origin',(0.599999999210582,-19.9,-6.46577223868862));
#142529=CARTESIAN_POINT('',(0.599999999210583,-20.,-1.85000000003699));
#142530=CARTESIAN_POINT('',(0.599999999210583,-19.9,-1.85000000003699));
#142531=CARTESIAN_POINT('',(0.599999999210583,-20.,-3.4578861193556));
#142532=CARTESIAN_POINT('Origin',(-3.45175358661618,-24.4,-3.05000000003699));
#142533=CARTESIAN_POINT('Origin',(-9.35,-24.,-3.05000000003699));
#142534=CARTESIAN_POINT('',(-9.75435462095199,-24.4,-15.093213746397));
#142535=CARTESIAN_POINT('',(-11.6859078763815,-24.4,-14.8714226890816));
#142536=CARTESIAN_POINT('Origin',(-9.35,-24.4,-3.05000000003699));
#142537=CARTESIAN_POINT('',(-11.6083673659622,-24.,-14.479010317661));
#142538=CARTESIAN_POINT('Origin',(-11.6859078763815,-24.,-14.8714226890816));
#142539=CARTESIAN_POINT('',(-9.354354620952,-24.,-14.6999991861862));
#142540=CARTESIAN_POINT('Origin',(-9.35,-24.,-3.05000000003699));
#142541=CARTESIAN_POINT('Ctrl Pts',(-9.35435462095199,-24.,-14.6999991861862));
#142542=CARTESIAN_POINT('Ctrl Pts',(-9.35435462095199,-24.037424083604,
-14.6999991861862));
#142543=CARTESIAN_POINT('Ctrl Pts',(-9.35960040832283,-24.0739958314266,
-14.7052459637971));
#142544=CARTESIAN_POINT('Ctrl Pts',(-9.38066945411349,-24.1485527620938,
-14.7262799468246));
#142545=CARTESIAN_POINT('Ctrl Pts',(-9.39750274952949,-24.1846222324459,
-14.7430693141688));
#142546=CARTESIAN_POINT('Ctrl Pts',(-9.4452457342648,-24.2588372562424,
-14.7905361348673));
#142547=CARTESIAN_POINT('Ctrl Pts',(-9.47880473566812,-24.2934419877695,
-14.8237995352573));
#142548=CARTESIAN_POINT('Ctrl Pts',(-9.5500240810494,-24.3466490845449,
-14.8940310481549));
#142549=CARTESIAN_POINT('Ctrl Pts',(-9.58800870687269,-24.3660751179944,
-14.9313311053489));
#142550=CARTESIAN_POINT('Ctrl Pts',(-9.66746480896846,-24.392789111755,
-15.0089629008643));
#142551=CARTESIAN_POINT('Ctrl Pts',(-9.70955513466183,-24.3996933673943,
-15.0498836464634));
#142552=CARTESIAN_POINT('Ctrl Pts',(-9.75246992778725,-24.399996669763,
-15.0913911669504));
#142553=CARTESIAN_POINT('Ctrl Pts',(-9.75341224988955,-24.4,-15.0923024847155));
#142554=CARTESIAN_POINT('Ctrl Pts',(-9.75435462095199,-24.4,-15.093213746397));
#142555=CARTESIAN_POINT('Ctrl Pts',(-11.6083673659622,-24.,-14.479010317661));
#142556=CARTESIAN_POINT('Ctrl Pts',(-11.9073491418757,-24.,-14.4199316514445));
#142557=CARTESIAN_POINT('Ctrl Pts',(-12.1314036071098,-24.,-14.6265230059077));
#142558=CARTESIAN_POINT('Ctrl Pts',(-12.355458072344,-24.,-14.8331143603709));
#142559=CARTESIAN_POINT('Ctrl Pts',(-12.3207815844978,-24.,-15.1358979998248));
#142560=CARTESIAN_POINT('Ctrl Pts',(-11.6083673659622,-24.4,-14.479010317661));
#142561=CARTESIAN_POINT('Ctrl Pts',(-11.9073491418757,-24.4,-14.4199316514445));
#142562=CARTESIAN_POINT('Ctrl Pts',(-12.1314036071098,-24.4,-14.6265230059077));
#142563=CARTESIAN_POINT('Ctrl Pts',(-12.355458072344,-24.4,-14.8331143603709));
#142564=CARTESIAN_POINT('Ctrl Pts',(-12.3207815844978,-24.4,-15.1358979998248));
#142565=CARTESIAN_POINT('Ctrl Pts',(-11.6859078763815,-24.4,-14.8714226890816));
#142566=CARTESIAN_POINT('Ctrl Pts',(-11.7855684683526,-24.4,-14.8517298003428));
#142567=CARTESIAN_POINT('Ctrl Pts',(-11.8602532900974,-24.4,-14.9205935851638));
#142568=CARTESIAN_POINT('Ctrl Pts',(-11.9349381118421,-24.4,-14.9894573699849));
#142569=CARTESIAN_POINT('Ctrl Pts',(-11.92337928256,-24.4,-15.0903852498028));
#142570=CARTESIAN_POINT('',(-11.92337928256,-24.4,-15.0903852498028));
#142571=CARTESIAN_POINT('',(-12.3207815844978,-24.,-15.1358979998248));
#142572=CARTESIAN_POINT('Origin',(-11.92337928256,-24.,-15.0903852498028));
#142573=CARTESIAN_POINT('Origin',(-11.7246781315911,-24.,-15.0676288747919));
#142574=CARTESIAN_POINT('Origin',(-11.7246781315911,-24.4,-15.0676288747919));
#142575=CARTESIAN_POINT('Origin',(-15.5,-24.,-15.5));
#142576=CARTESIAN_POINT('',(-12.1532274611957,-24.4,-16.8263157895108));
#142577=CARTESIAN_POINT('',(-12.5250910766184,-24.,-16.6789473684541));
#142578=CARTESIAN_POINT('Origin',(-12.1532274611957,-24.,-16.8263157895108));
#142579=CARTESIAN_POINT('Origin',(-15.5,-24.,-15.5));
#142580=CARTESIAN_POINT('Origin',(-15.5,-24.4,-15.5));
#142581=CARTESIAN_POINT('Ctrl Pts',(-12.5250910766184,-24.,-16.6789473684541));
#142582=CARTESIAN_POINT('Ctrl Pts',(-12.642154986228,-24.,-16.9743417843728));
#142583=CARTESIAN_POINT('Ctrl Pts',(-12.4635977686071,-24.,-17.2371708922063));
#142584=CARTESIAN_POINT('Ctrl Pts',(-12.2850405509867,-24.,-17.5000000000395));
#142585=CARTESIAN_POINT('Ctrl Pts',(-11.9672956534844,-24.,-17.5000000000392));
#142586=CARTESIAN_POINT('Ctrl Pts',(-12.5250910766184,-24.4,-16.6789473684541));
#142587=CARTESIAN_POINT('Ctrl Pts',(-12.642154986228,-24.4,-16.9743417843728));
#142588=CARTESIAN_POINT('Ctrl Pts',(-12.4635977686071,-24.4,-17.2371708922063));
#142589=CARTESIAN_POINT('Ctrl Pts',(-12.2850405509867,-24.4,-17.5000000000395));
#142590=CARTESIAN_POINT('Ctrl Pts',(-11.9672956534844,-24.4,-17.5000000000392));
#142591=CARTESIAN_POINT('Ctrl Pts',(-12.1532274611957,-24.4,-16.8263157895108));
#142592=CARTESIAN_POINT('Ctrl Pts',(-12.1922487643989,-24.4,-16.9247805948171));
#142593=CARTESIAN_POINT('Ctrl Pts',(-12.1327296918586,-24.4,-17.0123902974282));
#142594=CARTESIAN_POINT('Ctrl Pts',(-12.0732106193185,-24.4,-17.1000000000393));
#142595=CARTESIAN_POINT('Ctrl Pts',(-11.9672956534844,-24.4,-17.1000000000392));
#142596=CARTESIAN_POINT('',(-11.9672956534841,-24.4,-17.1000000000392));
#142597=CARTESIAN_POINT('',(-11.9672956534834,-24.,-17.5000000000392));
#142598=CARTESIAN_POINT('Origin',(-11.9672956534841,-24.,-17.1000000000392));
#142599=CARTESIAN_POINT('Origin',(-11.9672956534844,-24.,-16.9000000000392));
#142600=CARTESIAN_POINT('Origin',(-11.9672956534844,-24.4,-16.9000000000392));
#142601=CARTESIAN_POINT('Origin',(-11.8235138411924,-24.,-17.1000000000389));
#142602=CARTESIAN_POINT('',(-9.35435462095199,-24.,-17.5000000000348));
#142603=CARTESIAN_POINT('',(-11.8235138411917,-24.,-17.5000000000389));
#142604=CARTESIAN_POINT('',(-9.75435462095199,-24.4,-17.1000000000355));
#142605=CARTESIAN_POINT('',(-11.8235138411924,-24.4,-17.1000000000389));
#142606=CARTESIAN_POINT('Origin',(-9.75435462095199,-24.,-17.1000000000355));
#142607=CARTESIAN_POINT('Origin',(-9.75435462095199,-24.,-15.8999999999905));
#142608=CARTESIAN_POINT('',(-9.75435462095199,-24.4,-15.8999999999905));
#142609=CARTESIAN_POINT('',(-9.35459848714994,-23.9860345609578,-14.6999990924797));
#142610=CARTESIAN_POINT('Ctrl Pts',(-9.35459848714994,-23.9860345609578,
-14.6999990924797));
#142611=CARTESIAN_POINT('Ctrl Pts',(-9.35443500229638,-23.9907142615241,
-14.6999991570104));
#142612=CARTESIAN_POINT('Ctrl Pts',(-9.35435462095199,-23.9953714378489,
-14.6999991861862));
#142613=CARTESIAN_POINT('Ctrl Pts',(-9.35435462095199,-24.,-14.6999991861862));
#142614=CARTESIAN_POINT('',(-9.35459848714835,-23.986034560926,-17.5000000000348));
#142615=CARTESIAN_POINT('',(-9.35459848715105,-23.9860345609261,-15.8999999999905));
#142616=CARTESIAN_POINT('Origin',(-9.75435462095199,-24.,-17.5000000000409));
#142617=CARTESIAN_POINT('Origin',(-11.9672956534844,-10.3,-16.9000000000392));
#142618=CARTESIAN_POINT('',(-11.9672956534834,-10.3,-17.5000000000392));
#142619=CARTESIAN_POINT('',(-11.9672956534834,-10.3,-17.5000000000392));
#142620=CARTESIAN_POINT('',(-12.5250910766184,-10.3,-16.6789473684541));
#142621=CARTESIAN_POINT('Origin',(-11.9672956534844,-10.3,-16.9000000000392));
#142622=CARTESIAN_POINT('',(-12.5250910766184,-10.3,-16.6789473684541));
#142623=CARTESIAN_POINT('Origin',(-13.0020008006734,-10.3,-17.5000000000409));
#142624=CARTESIAN_POINT('',(-3.59005376343034,-20.7879235316574,-17.5000000000251));
#142625=CARTESIAN_POINT('Origin',(-5.65685424948968,-23.8568542494924,-17.5000000000285));
#142626=CARTESIAN_POINT('',(-3.59005376342686,-18.4674209709515,-17.5000000000251));
#142627=CARTESIAN_POINT('',(-3.59005376342686,-10.3,-17.5000000000251));
#142628=CARTESIAN_POINT('',(-1.39005376342686,-14.8791942943342,-17.5000000000433));
#142629=CARTESIAN_POINT('Origin',(-1.26287869055635E-16,-18.2,-17.5000000000409));
#142630=CARTESIAN_POINT('',(-1.39005376342686,-10.3,-17.5000000000213));
#142631=CARTESIAN_POINT('',(-1.39005376342686,-10.3,-17.5000000000213));
#142632=CARTESIAN_POINT('',(-2.22490186899551,-10.3,-17.5000000000227));
#142633=CARTESIAN_POINT('',(-0.170697831157441,-10.3,-17.5000000000193));
#142634=CARTESIAN_POINT('',(-9.08880662998386,-10.3,-17.5000000000343));
#142635=CARTESIAN_POINT('Origin',(-5.65685424948968,-12.5431457505076,-17.5000000000285));
#142636=CARTESIAN_POINT('',(-0.170697831157441,-10.3,-17.5000000000193));
#142637=CARTESIAN_POINT('Origin',(-5.65685424949238,-23.8568542494924,-15.8999999999905));
#142638=CARTESIAN_POINT('',(-3.59005376343416,-20.7879235316642,-13.1764761567201));
#142639=CARTESIAN_POINT('Ctrl Pts',(-9.35459848714994,-23.9860345609578,
-14.6999990924797));
#142640=CARTESIAN_POINT('Ctrl Pts',(-9.35676177374305,-23.9241111885544,
-14.6999982385873));
#142641=CARTESIAN_POINT('Ctrl Pts',(-9.35737145099148,-23.8620802493589,
-14.6999977069853));
#142642=CARTESIAN_POINT('Ctrl Pts',(-9.35641741186418,-23.799999982972,
-14.6999982325186));
#142643=CARTESIAN_POINT('Ctrl Pts',(-9.34952807250257,-23.3517038800543,
-14.7000020275173));
#142644=CARTESIAN_POINT('Ctrl Pts',(-9.25618380964402,-22.8776101099329,
-14.7010327279702));
#142645=CARTESIAN_POINT('Ctrl Pts',(-8.8860287285298,-21.9844435897398,
-14.6922910406182));
#142646=CARTESIAN_POINT('Ctrl Pts',(-8.60117160618611,-21.5685814254056,
-14.6805753032666));
#142647=CARTESIAN_POINT('Ctrl Pts',(-7.93807194307344,-20.905481762293,
-14.6190191278397));
#142648=CARTESIAN_POINT('Ctrl Pts',(-7.51415814075371,-20.6187964801274,
-14.5639150424745));
#142649=CARTESIAN_POINT('Ctrl Pts',(-6.59851020504296,-20.2446694117715,
-14.3800423269859));
#142650=CARTESIAN_POINT('Ctrl Pts',(-6.10725151442864,-20.1568542494924,
-14.2496697959988));
#142651=CARTESIAN_POINT('Ctrl Pts',(-5.16315899376981,-20.1568542494924,
-13.9341089601114));
#142652=CARTESIAN_POINT('Ctrl Pts',(-4.65119667500065,-20.2605684182922,
-13.7228927256965));
#142653=CARTESIAN_POINT('Ctrl Pts',(-3.97775061505936,-20.5518405627531,
-13.3900421583534));
#142654=CARTESIAN_POINT('Ctrl Pts',(-3.77693263646862,-20.6620681829664,
-13.2827729814766));
#142655=CARTESIAN_POINT('Ctrl Pts',(-3.59005376343416,-20.7879235316642,
-13.1764761567201));
#142656=CARTESIAN_POINT('',(-3.59005376342956,-20.7879235316673,-15.8999999999905));
#142657=CARTESIAN_POINT('Origin',(-10.6450268817134,-24.4,-15.5));
#142658=CARTESIAN_POINT('Origin',(-9.35,-10.3,-3.05000000003699));
#142659=CARTESIAN_POINT('',(-11.6083673659622,-10.3,-14.479010317661));
#142660=CARTESIAN_POINT('',(-11.6083673659622,-10.3,-14.479010317661));
#142661=CARTESIAN_POINT('',(-9.15685424949238,-10.3,-14.6983988049827));
#142662=CARTESIAN_POINT('Origin',(-9.35,-10.3,-3.05000000003699));
#142663=CARTESIAN_POINT('',(-8.15685424949238,-11.3,-14.6387403637713));
#142664=CARTESIAN_POINT('Ctrl Pts',(-8.15685424949238,-11.3,-14.6387403637713));
#142665=CARTESIAN_POINT('Ctrl Pts',(-8.15685424949238,-11.1743649985927,
-14.6387403637713));
#142666=CARTESIAN_POINT('Ctrl Pts',(-8.18197680776031,-11.0404139596789,
-14.641412739057));
#142667=CARTESIAN_POINT('Ctrl Pts',(-8.28402198897147,-10.7941000141912,
-14.6512421030957));
#142668=CARTESIAN_POINT('Ctrl Pts',(-8.36093991003168,-10.6817304364779,
-14.6582803730457));
#142669=CARTESIAN_POINT('Ctrl Pts',(-8.53837619979829,-10.5042348482132,
-14.6720346815212));
#142670=CARTESIAN_POINT('Ctrl Pts',(-8.65077495464815,-10.427264453842,
-14.6796516718487));
#142671=CARTESIAN_POINT('Ctrl Pts',(-8.89716064669893,-10.3251447177429,
-14.6918490881968));
#142672=CARTESIAN_POINT('Ctrl Pts',(-9.03115517829841,-10.3,-14.6963145492965));
#142673=CARTESIAN_POINT('Ctrl Pts',(-9.15685424949238,-10.3,-14.6983988049827));
#142674=CARTESIAN_POINT('',(-8.15685424949238,-12.5431457505076,-14.6387403637713));
#142675=CARTESIAN_POINT('',(-8.15685424949238,-10.3,-14.6387403637713));
#142676=CARTESIAN_POINT('',(-3.15685424949238,-12.5431457505076,-12.9174943989697));
#142677=CARTESIAN_POINT('Ctrl Pts',(-8.15685424949238,-12.5431457505076,
-14.6387403637713));
#142678=CARTESIAN_POINT('Ctrl Pts',(-8.15685424949238,-12.8564022173972,
-14.6387403637713));
#142679=CARTESIAN_POINT('Ctrl Pts',(-8.09433479998511,-13.190466093178,
-14.6328369794813));
#142680=CARTESIAN_POINT('Ctrl Pts',(-7.84073632742103,-13.8044918157331,
-14.6025292016044));
#142681=CARTESIAN_POINT('Ctrl Pts',(-7.64965844750753,-14.0844177261518,
-14.5773916287323));
#142682=CARTESIAN_POINT('Ctrl Pts',(-7.20376387556559,-14.5332382695204,
-14.5029020140874));
#142683=CARTESIAN_POINT('Ctrl Pts',(-6.91723165226354,-14.7280486885119,
-14.4476267125339));
#142684=CARTESIAN_POINT('Ctrl Pts',(-6.29717897630526,-14.9828867355091,
-14.2974237235192));
#142685=CARTESIAN_POINT('Ctrl Pts',(-5.96393092697842,-15.0431457505076,
-14.2017652067917));
#142686=CARTESIAN_POINT('Ctrl Pts',(-5.33066040655443,-15.0431457505076,
-13.9900959366778));
#142687=CARTESIAN_POINT('Ctrl Pts',(-4.98833212718866,-14.9759248056554,
-13.8580828066145));
#142688=CARTESIAN_POINT('Ctrl Pts',(-4.363575736342,-14.7094251062448,-13.5844375087381));
#142689=CARTESIAN_POINT('Ctrl Pts',(-4.08079555119357,-14.5103803575851,
-13.4433817276104));
#142690=CARTESIAN_POINT('Ctrl Pts',(-3.65133920193737,-14.064895460083,
-13.2137667708102));
#142691=CARTESIAN_POINT('Ctrl Pts',(-3.46785847818632,-13.7938980371273,
-13.1070248812659));
#142692=CARTESIAN_POINT('Ctrl Pts',(-3.22046675563909,-13.1912956863282,
-12.9581865955658));
#142693=CARTESIAN_POINT('Ctrl Pts',(-3.15685424949238,-12.8592223348356,
-12.9174943989697));
#142694=CARTESIAN_POINT('Ctrl Pts',(-3.15685424949238,-12.5431457505076,
-12.9174943989697));
#142695=CARTESIAN_POINT('',(-3.15685424949238,-11.3,-12.9174943989697));
#142696=CARTESIAN_POINT('',(-3.15685424949238,-10.3,-12.9174943989697));
#142697=CARTESIAN_POINT('',(-2.15685424949238,-10.3,-12.2141232102494));
#142698=CARTESIAN_POINT('Ctrl Pts',(-2.15685424949238,-10.3,-12.2141232102494));
#142699=CARTESIAN_POINT('Ctrl Pts',(-2.28026220008018,-10.3,-12.3109891465738));
#142700=CARTESIAN_POINT('Ctrl Pts',(-2.41580651903231,-10.3241114437069,
-12.4129327889492));
#142701=CARTESIAN_POINT('Ctrl Pts',(-2.67271826515926,-10.4320719373805,
-12.5978509719696));
#142702=CARTESIAN_POINT('Ctrl Pts',(-2.79395836511785,-10.5160800083143,
-12.680909505094));
#142703=CARTESIAN_POINT('Ctrl Pts',(-2.96758654966608,-10.7038187238232,
-12.7965770599196));
#142704=CARTESIAN_POINT('Ctrl Pts',(-3.03762609498192,-10.8096646825789,
-12.8418124725612));
#142705=CARTESIAN_POINT('Ctrl Pts',(-3.13234930878862,-11.0458400668001,
-12.9022320096932));
#142706=CARTESIAN_POINT('Ctrl Pts',(-3.15685424949238,-11.1762211096894,
-12.9174943989697));
#142707=CARTESIAN_POINT('Ctrl Pts',(-3.15685424949238,-11.3,-12.9174943989697));
#142708=CARTESIAN_POINT('',(-1.77992868114481,-10.3,-11.9053102841234));
#142709=CARTESIAN_POINT('Origin',(-9.35,-10.3,-3.05000000003699));
#142710=CARTESIAN_POINT('',(-1.77992868114481,-15.0708061916784,-11.9053102841234));
#142711=CARTESIAN_POINT('',(-1.77992868114481,-10.3,-11.9053102841234));
#142712=CARTESIAN_POINT('',(-3.59005376343415,-18.4674209708535,-13.1764761567201));
#142713=CARTESIAN_POINT('Ctrl Pts',(-3.59005376343416,-18.4674209708535,
-13.1764761567201));
#142714=CARTESIAN_POINT('Ctrl Pts',(-3.59678968275853,-18.3769930868941,
-13.1803075520211));
#142715=CARTESIAN_POINT('Ctrl Pts',(-3.6,-18.2875463035025,-13.1821271212293));
#142716=CARTESIAN_POINT('Ctrl Pts',(-3.6,-17.8815466224465,-13.1821271212293));
#142717=CARTESIAN_POINT('Ctrl Pts',(-3.55476999791657,-17.5382077727571,
-13.1568963520113));
#142718=CARTESIAN_POINT('Ctrl Pts',(-3.36933995170902,-16.8877857922236,
-13.0482873955818));
#142719=CARTESIAN_POINT('Ctrl Pts',(-3.22941756244032,-16.5807035365666,
-12.964430626659));
#142720=CARTESIAN_POINT('Ctrl Pts',(-2.88197413954814,-16.0120984149223,
-12.7421606660272));
#142721=CARTESIAN_POINT('Ctrl Pts',(-2.63436410033982,-15.720213086085,
-12.5756271636011));
#142722=CARTESIAN_POINT('Ctrl Pts',(-2.17431453454083,-15.3198884370908,
-12.2308360831179));
#142723=CARTESIAN_POINT('Ctrl Pts',(-1.97456413725502,-15.1815175288212,
-12.0716968066352));
#142724=CARTESIAN_POINT('Ctrl Pts',(-1.77992868114481,-15.0708061916784,
-11.9053102841234));
#142725=CARTESIAN_POINT('',(-3.59005376343416,-10.3,-13.1764761567201));
#142726=CARTESIAN_POINT('Origin',(-14.5000000000146,-24.,0.715147871306033));
#142727=CARTESIAN_POINT('',(-14.9000000000115,-24.,2.37724133593659));
#142728=CARTESIAN_POINT('',(-14.5000000000115,-24.4,2.37724133593584));
#142729=CARTESIAN_POINT('Origin',(-14.5000000000115,-24.,2.37724133593584));
#142730=CARTESIAN_POINT('',(-14.5000000000318,-24.4,-8.3813708499249));
#142731=CARTESIAN_POINT('',(-14.5000000000146,-24.4,0.715147871306033));
#142732=CARTESIAN_POINT('',(-14.9000000000318,-24.,-8.38137084992414));
#142733=CARTESIAN_POINT('Origin',(-14.5000000000318,-24.,-8.3813708499249));
#142734=CARTESIAN_POINT('',(-14.9000000000146,-24.,0.715147871306786));
#142735=CARTESIAN_POINT('Origin',(-15.7000000000318,-24.,-8.38137084992264));
#142736=CARTESIAN_POINT('',(-14.8514718626079,-24.4,-9.2298989873465));
#142737=CARTESIAN_POINT('',(-15.1343145750825,-24.,-8.94705627487188));
#142738=CARTESIAN_POINT('Origin',(-14.8514718626079,-24.,-9.2298989873465));
#142739=CARTESIAN_POINT('Origin',(-15.7000000000318,-24.,-8.38137084992264));
#142740=CARTESIAN_POINT('Origin',(-15.7000000000318,-24.4,-8.38137084992264));
#142741=CARTESIAN_POINT('Origin',(-10.3394102592575,-24.,-4.71783738399612));
#142742=CARTESIAN_POINT('',(-15.0728809663607,-24.4,-9.45130809109928));
#142743=CARTESIAN_POINT('',(-15.3557236788353,-24.,-9.16846537862467));
#142744=CARTESIAN_POINT('Origin',(-15.0728809663607,-24.,-9.45130809109928));
#142745=CARTESIAN_POINT('',(-10.6222529717321,-24.,-4.4349946715215));
#142746=CARTESIAN_POINT('',(-10.3394102592575,-24.4,-4.71783738399612));
#142747=CARTESIAN_POINT('Ctrl Pts',(-15.3557236788353,-24.,-9.16846537862466));
#142748=CARTESIAN_POINT('Ctrl Pts',(-15.54137387769,-24.,-9.35411557747933));
#142749=CARTESIAN_POINT('Ctrl Pts',(-15.5309901758822,-24.,-9.61645919071648));
#142750=CARTESIAN_POINT('Ctrl Pts',(-15.5206064740745,-24.,-9.87880280395362));
#142751=CARTESIAN_POINT('Ctrl Pts',(-15.3208637689692,-24.,-10.0491989436598));
#142752=CARTESIAN_POINT('Ctrl Pts',(-15.3557236788353,-24.4,-9.16846537862466));
#142753=CARTESIAN_POINT('Ctrl Pts',(-15.54137387769,-24.4,-9.35411557747933));
#142754=CARTESIAN_POINT('Ctrl Pts',(-15.5309901758822,-24.4,-9.61645919071648));
#142755=CARTESIAN_POINT('Ctrl Pts',(-15.5206064740745,-24.4,-9.87880280395362));
#142756=CARTESIAN_POINT('Ctrl Pts',(-15.3208637689692,-24.4,-10.0491989436598));
#142757=CARTESIAN_POINT('Ctrl Pts',(-15.0728809663607,-24.4,-9.45130809109929));
#142758=CARTESIAN_POINT('Ctrl Pts',(-15.1347643659789,-24.4,-9.51319149071751));
#142759=CARTESIAN_POINT('Ctrl Pts',(-15.131303132043,-24.4,-9.60063936179656));
#142760=CARTESIAN_POINT('Ctrl Pts',(-15.1278418981071,-24.4,-9.68808723287561));
#142761=CARTESIAN_POINT('Ctrl Pts',(-15.0612609964053,-24.4,-9.74488594611101));
#142762=CARTESIAN_POINT('',(-15.0612609964053,-24.4,-9.74488594611101));
#142763=CARTESIAN_POINT('',(-15.3208637689692,-24.,-10.0491989436598));
#142764=CARTESIAN_POINT('Origin',(-15.0612609964053,-24.,-9.74488594611101));
#142765=CARTESIAN_POINT('Origin',(-14.9314596101234,-24.,-9.5927294473366));
#142766=CARTESIAN_POINT('Origin',(-14.9314596101234,-24.4,-9.5927294473366));
#142767=CARTESIAN_POINT('Origin',(-9.35,-24.,-3.05000000003699));
#142768=CARTESIAN_POINT('',(-14.7703541221629,-24.4,-9.98251478115012));
#142769=CARTESIAN_POINT('',(-15.0167338549885,-24.,-10.2976290893825));
#142770=CARTESIAN_POINT('Origin',(-14.7703541221629,-24.,-9.98251478115012));
#142771=CARTESIAN_POINT('Origin',(-9.35,-24.,-3.05000000003699));
#142772=CARTESIAN_POINT('Origin',(-9.35,-24.4,-3.05000000003699));
#142773=CARTESIAN_POINT('Ctrl Pts',(-15.0167338549885,-24.,-10.2976290893825));
#142774=CARTESIAN_POINT('Ctrl Pts',(-14.8012729185294,-24.,-10.4660924265662));
#142775=CARTESIAN_POINT('Ctrl Pts',(-14.5327864509729,-24.,-10.4139548407577));
#142776=CARTESIAN_POINT('Ctrl Pts',(-14.2642999834165,-24.,-10.3618172549492));
#142777=CARTESIAN_POINT('Ctrl Pts',(-14.1275490134794,-24.,-10.1249576270339));
#142778=CARTESIAN_POINT('Ctrl Pts',(-15.0167338549885,-24.4,-10.2976290893825));
#142779=CARTESIAN_POINT('Ctrl Pts',(-14.8012729185294,-24.4,-10.4660924265662));
#142780=CARTESIAN_POINT('Ctrl Pts',(-14.5327864509729,-24.4,-10.4139548407577));
#142781=CARTESIAN_POINT('Ctrl Pts',(-14.2642999834165,-24.4,-10.3618172549492));
#142782=CARTESIAN_POINT('Ctrl Pts',(-14.1275490134794,-24.4,-10.1249576270339));
#142783=CARTESIAN_POINT('Ctrl Pts',(-14.7703541221629,-24.4,-9.98251478115011));
#142784=CARTESIAN_POINT('Ctrl Pts',(-14.6985338100098,-24.4,-10.038669226878));
#142785=CARTESIAN_POINT('Ctrl Pts',(-14.6090383208244,-24.4,-10.0212900316085));
#142786=CARTESIAN_POINT('Ctrl Pts',(-14.5195428316389,-24.4,-10.003910836339));
#142787=CARTESIAN_POINT('Ctrl Pts',(-14.4739591749932,-24.4,-9.92495762703391));
#142788=CARTESIAN_POINT('',(-14.4739591749932,-24.4,-9.92495762703391));
#142789=CARTESIAN_POINT('',(-14.1275490134794,-24.,-10.1249576270339));
#142790=CARTESIAN_POINT('Origin',(-14.4739591749932,-24.,-9.92495762703391));
#142791=CARTESIAN_POINT('Origin',(-14.6471642557501,-24.,-9.82495762703391));
#142792=CARTESIAN_POINT('Origin',(-14.6471642557501,-24.4,-9.82495762703391));
#142793=CARTESIAN_POINT('Origin',(-11.8202184969051,-24.,-5.32854394247302));
#142794=CARTESIAN_POINT('',(-12.1762549821757,-24.4,-5.94521722430999));
#142795=CARTESIAN_POINT('',(-11.8298448206619,-24.,-6.14521722430999));
#142796=CARTESIAN_POINT('Origin',(-12.1762549821757,-24.,-5.94521722430999));
#142797=CARTESIAN_POINT('',(-11.4738083353913,-24.,-5.52854394247302));
#142798=CARTESIAN_POINT('',(-11.8202184969051,-24.4,-5.32854394247302));
#142799=CARTESIAN_POINT('Ctrl Pts',(-11.8298448206619,-24.,-6.14521722430999));
#142800=CARTESIAN_POINT('Ctrl Pts',(-11.6079320382025,-24.,-5.76085301024134));
#142801=CARTESIAN_POINT('Ctrl Pts',(-11.9105146878693,-24.,-5.43616104514808));
#142802=CARTESIAN_POINT('Ctrl Pts',(-11.8298448206619,-24.4,-6.14521722430999));
#142803=CARTESIAN_POINT('Ctrl Pts',(-11.6079320382025,-24.4,-5.76085301024134));
#142804=CARTESIAN_POINT('Ctrl Pts',(-11.9105146878693,-24.4,-5.43616104514808));
#142805=CARTESIAN_POINT('Ctrl Pts',(-12.1762549821757,-24.4,-5.94521722430999));
#142806=CARTESIAN_POINT('Ctrl Pts',(-12.1022840546892,-24.4,-5.81709581962044));
#142807=CARTESIAN_POINT('Ctrl Pts',(-12.2031449379115,-24.4,-5.70886516458935));
#142808=CARTESIAN_POINT('',(-12.2031449379115,-24.4,-5.70886516458935));
#142809=CARTESIAN_POINT('',(-11.9105146878693,-24.,-5.43616104514808));
#142810=CARTESIAN_POINT('Origin',(-12.2031449379115,-24.,-5.70886516458935));
#142811=CARTESIAN_POINT('Origin',(-12.3494600629326,-24.,-5.84521722430999));
#142812=CARTESIAN_POINT('Origin',(-12.3494600629326,-24.4,-5.84521722430999));
#142813=CARTESIAN_POINT('Origin',(-9.35,-24.,-3.05000000003699));
#142814=CARTESIAN_POINT('',(-12.2031449379115,-24.4,-0.391134835484633));
#142815=CARTESIAN_POINT('',(-11.9105146878693,-24.,-0.663838954925902));
#142816=CARTESIAN_POINT('Origin',(-12.2031449379115,-24.,-0.391134835484633));
#142817=CARTESIAN_POINT('',(-12.85,-24.,-3.05000000003699));
#142818=CARTESIAN_POINT('Origin',(-9.35,-24.,-3.05000000003699));
#142819=CARTESIAN_POINT('Origin',(-9.35,-24.,-3.05000000003699));
#142820=CARTESIAN_POINT('Origin',(-9.35,-24.4,-3.05000000003699));
#142821=CARTESIAN_POINT('Ctrl Pts',(-11.9105146878693,-24.,-0.663838954925902));
#142822=CARTESIAN_POINT('Ctrl Pts',(-11.6079320382025,-24.,-0.339146989832641));
#142823=CARTESIAN_POINT('Ctrl Pts',(-11.8298448206619,-24.,0.0452172242359999));
#142824=CARTESIAN_POINT('Ctrl Pts',(-11.9105146878693,-24.4,-0.663838954925903));
#142825=CARTESIAN_POINT('Ctrl Pts',(-11.6079320382025,-24.4,-0.339146989832641));
#142826=CARTESIAN_POINT('Ctrl Pts',(-11.8298448206619,-24.4,0.0452172242359998));
#142827=CARTESIAN_POINT('Ctrl Pts',(-12.2031449379115,-24.4,-0.391134835484634));
#142828=CARTESIAN_POINT('Ctrl Pts',(-12.1022840546892,-24.4,-0.282904180453547));
#142829=CARTESIAN_POINT('Ctrl Pts',(-12.1762549821757,-24.4,-0.154782775764001));
#142830=CARTESIAN_POINT('',(-12.1762549821757,-24.4,-0.154782775764));
#142831=CARTESIAN_POINT('',(-11.8298448206619,-24.,0.0452172242359991));
#142832=CARTESIAN_POINT('Origin',(-12.1762549821757,-24.,-0.154782775764));
#142833=CARTESIAN_POINT('Origin',(-12.3494600629326,-24.,-0.254782775764));
#142834=CARTESIAN_POINT('Origin',(-12.3494600629326,-24.4,-0.254782775764001));
#142835=CARTESIAN_POINT('Origin',(-10.3305808539815,-24.,-3.35158414001175));
#142836=CARTESIAN_POINT('',(-13.7535898384977,-24.4,2.57724133593509));
#142837=CARTESIAN_POINT('',(-13.4071796769839,-24.,2.77724133593509));
#142838=CARTESIAN_POINT('Origin',(-13.7535898384977,-24.,2.57724133593509));
#142839=CARTESIAN_POINT('',(-9.98417069246773,-24.,-3.15158414001175));
#142840=CARTESIAN_POINT('',(-10.3305808539815,-24.4,-3.35158414001175));
#142841=CARTESIAN_POINT('Ctrl Pts',(-13.4071796769839,-24.,2.77724133593509));
#142842=CARTESIAN_POINT('Ctrl Pts',(-13.7141104721752,-24.,3.30886106761391));
#142843=CARTESIAN_POINT('Ctrl Pts',(-14.3070552360928,-24.,3.14998199696654));
#142844=CARTESIAN_POINT('Ctrl Pts',(-14.9000000000103,-24.,2.99110292631917));
#142845=CARTESIAN_POINT('Ctrl Pts',(-14.9000000000115,-24.,2.37724133593659));
#142846=CARTESIAN_POINT('Ctrl Pts',(-13.4071796769839,-24.4,2.77724133593509));
#142847=CARTESIAN_POINT('Ctrl Pts',(-13.7141104721752,-24.4,3.30886106761391));
#142848=CARTESIAN_POINT('Ctrl Pts',(-14.3070552360928,-24.4,3.14998199696654));
#142849=CARTESIAN_POINT('Ctrl Pts',(-14.9000000000103,-24.4,2.99110292631917));
#142850=CARTESIAN_POINT('Ctrl Pts',(-14.9000000000115,-24.4,2.37724133593659));
#142851=CARTESIAN_POINT('Ctrl Pts',(-13.7535898384977,-24.4,2.57724133593509));
#142852=CARTESIAN_POINT('Ctrl Pts',(-13.9070552360934,-24.4,2.8430512017745));
#142853=CARTESIAN_POINT('Ctrl Pts',(-14.2035276180521,-24.4,2.76361166645081));
#142854=CARTESIAN_POINT('Ctrl Pts',(-14.5000000000109,-24.4,2.68417213112713));
#142855=CARTESIAN_POINT('Ctrl Pts',(-14.5000000000115,-24.4,2.37724133593584));
#142856=CARTESIAN_POINT('Origin',(-14.1000000000115,-24.,2.37724133593509));
#142857=CARTESIAN_POINT('Origin',(-14.1000000000115,-24.4,2.37724133593509));
#142858=CARTESIAN_POINT('Origin',(-12.3494600629326,-21.1,-5.84521722430998));
#142859=CARTESIAN_POINT('',(-11.9105146878693,-20.,-5.43616104514808));
#142860=CARTESIAN_POINT('',(-11.9105146878693,-21.1,-5.43616104514808));
#142861=CARTESIAN_POINT('',(-11.8298448206619,-20.,-6.14521722430999));
#142862=CARTESIAN_POINT('Origin',(-12.3494600629326,-20.,-5.84521722430998));
#142863=CARTESIAN_POINT('',(-11.8298448206619,-21.1,-6.14521722430999));
#142864=CARTESIAN_POINT('Origin',(-9.35,-21.1,-3.05000000003699));
#142865=CARTESIAN_POINT('',(-12.85,-19.7,-3.05000000003699));
#142866=CARTESIAN_POINT('Origin',(-9.35,-19.7,-3.05000000003699));
#142867=CARTESIAN_POINT('',(-12.85,-21.1,-3.05000000003699));
#142868=CARTESIAN_POINT('',(-11.9105146878693,-20.,-0.663838954925901));
#142869=CARTESIAN_POINT('',(-11.9105146878693,-21.1,-0.663838954925901));
#142870=CARTESIAN_POINT('',(-10.1362187386524,-20.,0.360551288976537));
#142871=CARTESIAN_POINT('Origin',(-9.35,-20.,-3.05000000003699));
#142872=CARTESIAN_POINT('',(-10.1362187386524,-24.,0.360551288976536));
#142873=CARTESIAN_POINT('',(-10.1362187386524,-21.1,0.360551288976537));
#142874=CARTESIAN_POINT('',(-6.00326657347833,-24.,-2.02560975613455));
#142875=CARTESIAN_POINT('Origin',(-9.35,-24.,-3.05000000003699));
#142876=CARTESIAN_POINT('',(-6.00326657347833,-20.,-2.02560975613455));
#142877=CARTESIAN_POINT('',(-6.00326657347833,-21.1,-2.02560975613455));
#142878=CARTESIAN_POINT('',(-6.00326657347833,-20.,-4.07439024393943));
#142879=CARTESIAN_POINT('Origin',(-9.35,-20.,-3.05000000003699));
#142880=CARTESIAN_POINT('',(-6.00326657347833,-24.,-4.07439024393943));
#142881=CARTESIAN_POINT('',(-6.00326657347833,-21.1,-4.07439024393943));
#142882=CARTESIAN_POINT('',(-10.1362187386524,-24.,-6.46055128905052));
#142883=CARTESIAN_POINT('Origin',(-9.35,-24.,-3.05000000003699));
#142884=CARTESIAN_POINT('',(-10.1362187386524,-20.,-6.46055128905052));
#142885=CARTESIAN_POINT('',(-10.1362187386524,-21.1,-6.46055128905052));
#142886=CARTESIAN_POINT('Origin',(-9.35,-20.,-3.05000000003699));
#142887=CARTESIAN_POINT('Origin',(-12.3494600629326,-21.1,-0.254782775764));
#142888=CARTESIAN_POINT('',(-11.8298448206619,-20.,0.0452172242360003));
#142889=CARTESIAN_POINT('',(-11.8298448206619,-21.1,0.0452172242359998));
#142890=CARTESIAN_POINT('Origin',(-12.3494600629326,-20.,-0.254782775764));
#142891=CARTESIAN_POINT('Origin',(-11.5732877460107,-19.9,-0.399152664101091));
#142892=CARTESIAN_POINT('',(-13.4071796769839,-20.,2.77724133593509));
#142893=CARTESIAN_POINT('',(-13.4071796769839,-19.9,2.77724133593509));
#142894=CARTESIAN_POINT('',(-10.9972459287083,-20.,-1.39688635895322));
#142895=CARTESIAN_POINT('Origin',(-14.1000000000115,-19.9,2.37724133593509));
#142896=CARTESIAN_POINT('',(-14.9000000000115,-20.,2.3772413359366));
#142897=CARTESIAN_POINT('',(-14.9000000000115,-19.9,2.3772413359366));
#142898=CARTESIAN_POINT('Origin',(-14.1000000000115,-20.,2.37724133593509));
#142899=CARTESIAN_POINT('Origin',(-14.9000000000075,-22.8,4.48029574262901));
#142900=CARTESIAN_POINT('',(-14.9000000000318,-20.,-8.38137084992414));
#142901=CARTESIAN_POINT('',(-14.9000000000318,-22.8,-8.38137084992414));
#142902=CARTESIAN_POINT('',(-14.9000000000171,-20.,-0.58485212871229));
#142903=CARTESIAN_POINT('Origin',(-3.45175358661618,-24.4,-3.05000000003699));
#142904=CARTESIAN_POINT('Origin',(-9.35,-24.,-3.05000000003699));
#142905=CARTESIAN_POINT('',(-3.36628450305284,-24.4,-9.50253042240576));
#142906=CARTESIAN_POINT('',(-1.01046511708684,-24.4,-5.85929847771334));
#142907=CARTESIAN_POINT('Origin',(-9.35,-24.4,-3.05000000003699));
#142908=CARTESIAN_POINT('',(-0.631395349681702,-24.,-5.98699386306226));
#142909=CARTESIAN_POINT('Origin',(-1.01046511708684,-24.,-5.85929847771334));
#142910=CARTESIAN_POINT('',(-3.34165888869613,-24.,-10.0170536879467));
#142911=CARTESIAN_POINT('Origin',(-9.35,-24.,-3.05000000003699));
#142912=CARTESIAN_POINT('Ctrl Pts',(-3.36628450305284,-24.4,-9.50253042240576));
#142913=CARTESIAN_POINT('Ctrl Pts',(-3.36619187924502,-24.4,-9.50372689824024));
#142914=CARTESIAN_POINT('Ctrl Pts',(-3.36609949462665,-24.3999966844721,
-9.50492339449873));
#142915=CARTESIAN_POINT('Ctrl Pts',(-3.36298725258202,-24.3997727516819,
-9.54533619308514));
#142916=CARTESIAN_POINT('Ctrl Pts',(-3.36022413301821,-24.3959947528393,
-9.58462112336526));
#142917=CARTESIAN_POINT('Ctrl Pts',(-3.35282072422976,-24.3739050476839,
-9.7007017752616));
#142918=CARTESIAN_POINT('Ctrl Pts',(-3.34928303606659,-24.3452366730688,
-9.77290486275007));
#142919=CARTESIAN_POINT('Ctrl Pts',(-3.34497556527484,-24.2733286996026,
-9.88229757161595));
#142920=CARTESIAN_POINT('Ctrl Pts',(-3.3437149391037,-24.2334157755877,
-9.92518249065517));
#142921=CARTESIAN_POINT('Ctrl Pts',(-3.34228518261157,-24.1483727618738,
-9.98306784206126));
#142922=CARTESIAN_POINT('Ctrl Pts',(-3.34194048879486,-24.1068706951224,
-10.0015273168103));
#142923=CARTESIAN_POINT('Ctrl Pts',(-3.34169547356203,-24.0418361742419,
-10.0149184217387));
#142924=CARTESIAN_POINT('Ctrl Pts',(-3.34165888869613,-24.0209215876749,
-10.0170536879467));
#142925=CARTESIAN_POINT('Ctrl Pts',(-3.34165888869614,-23.9999999999998,
-10.0170536879467));
#142926=CARTESIAN_POINT('Ctrl Pts',(-0.631395349681701,-24.,-5.98699386306226));
#142927=CARTESIAN_POINT('Ctrl Pts',(-0.600000000789416,-24.,-5.89379529077492));
#142928=CARTESIAN_POINT('Ctrl Pts',(-0.600000000789416,-24.,-5.79545078503888));
#142929=CARTESIAN_POINT('Ctrl Pts',(-0.631395349681701,-24.4,-5.98699386306226));
#142930=CARTESIAN_POINT('Ctrl Pts',(-0.600000000789416,-24.4,-5.89379529077492));
#142931=CARTESIAN_POINT('Ctrl Pts',(-0.600000000789416,-24.4,-5.79545078503888));
#142932=CARTESIAN_POINT('Ctrl Pts',(-1.01046511708684,-24.4,-5.85929847771334));
#142933=CARTESIAN_POINT('Ctrl Pts',(-1.00000000078942,-24.4,-5.82823228695089));
#142934=CARTESIAN_POINT('Ctrl Pts',(-1.00000000078942,-24.4,-5.79545078503888));
#142935=CARTESIAN_POINT('',(-1.00000000078942,-24.4,-5.79545078503888));
#142936=CARTESIAN_POINT('',(-0.600000000789416,-24.,-5.79545078503888));
#142937=CARTESIAN_POINT('Origin',(-1.00000000078942,-24.,-5.79545078503888));
#142938=CARTESIAN_POINT('Origin',(-1.20000000078942,-24.,-5.79545078503888));
#142939=CARTESIAN_POINT('Origin',(-1.20000000078942,-24.4,-5.79545078503888));
#142940=CARTESIAN_POINT('Origin',(-1.00000000078942,-24.,-1.33262554947194));
#142941=CARTESIAN_POINT('',(-1.00000000078942,-24.4,-4.25000000003699));
#142942=CARTESIAN_POINT('',(-0.600000000789417,-24.,-4.25000000003699));
#142943=CARTESIAN_POINT('Origin',(-1.00000000078942,-24.,-4.25000000003699));
#142944=CARTESIAN_POINT('',(-0.600000000789417,-24.,-1.33262554947194));
#142945=CARTESIAN_POINT('',(-1.00000000078942,-24.4,-1.33262554947194));
#142946=CARTESIAN_POINT('Ctrl Pts',(-0.600000000789416,-24.,-4.25000000003699));
#142947=CARTESIAN_POINT('Ctrl Pts',(-0.600000000789416,-24.,-3.65000000003699));
#142948=CARTESIAN_POINT('Ctrl Pts',(-1.20000000078942,-24.,-3.65000000003699));
#142949=CARTESIAN_POINT('Ctrl Pts',(-0.600000000789416,-24.4,-4.25000000003699));
#142950=CARTESIAN_POINT('Ctrl Pts',(-0.600000000789416,-24.4,-3.65000000003699));
#142951=CARTESIAN_POINT('Ctrl Pts',(-1.20000000078942,-24.4,-3.65000000003699));
#142952=CARTESIAN_POINT('Ctrl Pts',(-1.00000000078942,-24.4,-4.25000000003699));
#142953=CARTESIAN_POINT('Ctrl Pts',(-1.00000000078942,-24.4,-4.05000000003699));
#142954=CARTESIAN_POINT('Ctrl Pts',(-1.20000000078942,-24.4,-4.05000000003699));
#142955=CARTESIAN_POINT('',(-1.20000000078942,-24.4,-4.05000000003699));
#142956=CARTESIAN_POINT('',(-1.20000000078942,-24.,-3.65000000003699));
#142957=CARTESIAN_POINT('Origin',(-1.20000000078942,-24.,-4.05000000003699));
#142958=CARTESIAN_POINT('Origin',(-1.20000000078942,-24.,-4.25000000003699));
#142959=CARTESIAN_POINT('Origin',(-1.20000000078942,-24.4,-4.25000000003699));
#142960=CARTESIAN_POINT('Origin',(-1.71792900372085,-24.,-4.05000000003699));
#142961=CARTESIAN_POINT('',(-5.42954084321747,-24.4,-4.05000000003699));
#142962=CARTESIAN_POINT('',(-5.42954084321747,-24.,-3.65000000003699));
#142963=CARTESIAN_POINT('Origin',(-5.42954084321747,-24.,-4.05000000003699));
#142964=CARTESIAN_POINT('',(-1.71792900372085,-24.,-3.65000000003699));
#142965=CARTESIAN_POINT('',(-1.71792900372085,-24.4,-4.05000000003699));
#142966=CARTESIAN_POINT('Ctrl Pts',(-5.42954084321747,-24.,-3.65000000003699));
#142967=CARTESIAN_POINT('Ctrl Pts',(-5.87336640813625,-24.,-3.65000000003699));
#142968=CARTESIAN_POINT('Ctrl Pts',(-6.00326657347833,-24.,-4.07439024393943));
#142969=CARTESIAN_POINT('Ctrl Pts',(-5.42954084321747,-24.4,-3.65000000003699));
#142970=CARTESIAN_POINT('Ctrl Pts',(-5.87336640813625,-24.4,-3.65000000003699));
#142971=CARTESIAN_POINT('Ctrl Pts',(-6.00326657347833,-24.4,-4.07439024393943));
#142972=CARTESIAN_POINT('Ctrl Pts',(-5.42954084321747,-24.4,-4.05000000003699));
#142973=CARTESIAN_POINT('Ctrl Pts',(-5.57748269819039,-24.4,-4.05000000003699));
#142974=CARTESIAN_POINT('Ctrl Pts',(-5.62078275330442,-24.4,-4.19146341467114));
#142975=CARTESIAN_POINT('',(-5.62078275330442,-24.4,-4.19146341467114));
#142976=CARTESIAN_POINT('Origin',(-5.62078275330442,-24.,-4.19146341467114));
#142977=CARTESIAN_POINT('Origin',(-5.42954084321747,-24.,-4.25000000003699));
#142978=CARTESIAN_POINT('Origin',(-5.42954084321747,-24.4,-4.25000000003699));
#142979=CARTESIAN_POINT('Origin',(-9.35,-24.,-3.05000000003699));
#142980=CARTESIAN_POINT('',(-10.2260723087841,-24.4,-6.8503285792235));
#142981=CARTESIAN_POINT('Origin',(-10.2260723087841,-24.,-6.8503285792235));
#142982=CARTESIAN_POINT('Origin',(-9.35,-24.4,-3.05000000003699));
#142983=CARTESIAN_POINT('Ctrl Pts',(-10.1362187386524,-24.,-6.46055128905052));
#142984=CARTESIAN_POINT('Ctrl Pts',(-10.5687015536612,-24.,-6.36085301024134));
#142985=CARTESIAN_POINT('Ctrl Pts',(-10.7906143361206,-24.,-6.74521722430999));
#142986=CARTESIAN_POINT('Ctrl Pts',(-10.1362187386524,-24.4,-6.46055128905052));
#142987=CARTESIAN_POINT('Ctrl Pts',(-10.5687015536612,-24.4,-6.36085301024134));
#142988=CARTESIAN_POINT('Ctrl Pts',(-10.7906143361206,-24.4,-6.74521722430999));
#142989=CARTESIAN_POINT('Ctrl Pts',(-10.2260723087841,-24.4,-6.8503285792235));
#142990=CARTESIAN_POINT('Ctrl Pts',(-10.3702332471204,-24.4,-6.81709581962044));
#142991=CARTESIAN_POINT('Ctrl Pts',(-10.4442041746068,-24.4,-6.94521722430999));
#142992=CARTESIAN_POINT('',(-10.4442041746068,-24.4,-6.94521722430999));
#142993=CARTESIAN_POINT('',(-10.7906143361206,-24.,-6.74521722430999));
#142994=CARTESIAN_POINT('Origin',(-10.4442041746068,-24.,-6.94521722430999));
#142995=CARTESIAN_POINT('Origin',(-10.2709990938499,-24.,-7.04521722430998));
#142996=CARTESIAN_POINT('Origin',(-10.2709990938499,-24.4,-7.04521722430998));
#142997=CARTESIAN_POINT('Origin',(-8.59853004641263,-24.,-3.74841586006224));
#142998=CARTESIAN_POINT('',(-12.7419083674243,-24.4,-10.9249576270339));
#142999=CARTESIAN_POINT('',(-13.0883185289381,-24.,-10.7249576270339));
#143000=CARTESIAN_POINT('Origin',(-12.7419083674243,-24.,-10.9249576270339));
#143001=CARTESIAN_POINT('',(-8.9449402079264,-24.,-3.54841586006224));
#143002=CARTESIAN_POINT('',(-8.59853004641263,-24.4,-3.74841586006224));
#143003=CARTESIAN_POINT('Ctrl Pts',(-13.0883185289381,-24.,-10.7249576270339));
#143004=CARTESIAN_POINT('Ctrl Pts',(-13.2250694988751,-24.,-10.9618172549492));
#143005=CARTESIAN_POINT('Ctrl Pts',(-13.135978738899,-24.,-11.2204021493297));
#143006=CARTESIAN_POINT('Ctrl Pts',(-13.046887978923,-24.,-11.4789870437101));
#143007=CARTESIAN_POINT('Ctrl Pts',(-12.7932639810861,-24.,-11.5813500196151));
#143008=CARTESIAN_POINT('Ctrl Pts',(-13.0883185289381,-24.4,-10.7249576270339));
#143009=CARTESIAN_POINT('Ctrl Pts',(-13.2250694988751,-24.4,-10.9618172549492));
#143010=CARTESIAN_POINT('Ctrl Pts',(-13.135978738899,-24.4,-11.2204021493297));
#143011=CARTESIAN_POINT('Ctrl Pts',(-13.046887978923,-24.4,-11.4789870437101));
#143012=CARTESIAN_POINT('Ctrl Pts',(-12.7932639810861,-24.4,-11.5813500196151));
#143013=CARTESIAN_POINT('Ctrl Pts',(-12.7419083674243,-24.4,-10.9249576270339));
#143014=CARTESIAN_POINT('Ctrl Pts',(-12.78749202407,-24.4,-11.003910836339));
#143015=CARTESIAN_POINT('Ctrl Pts',(-12.757795104078,-24.4,-11.0901058011325));
#143016=CARTESIAN_POINT('Ctrl Pts',(-12.7280981840859,-24.4,-11.176300765926));
#143017=CARTESIAN_POINT('Ctrl Pts',(-12.6435568514736,-24.4,-11.2104217578943));
#143018=CARTESIAN_POINT('',(-12.6435568514736,-24.4,-11.2104217578943));
#143019=CARTESIAN_POINT('',(-12.7932639810861,-24.,-11.5813500196151));
#143020=CARTESIAN_POINT('Origin',(-12.6435568514736,-24.,-11.2104217578943));
#143021=CARTESIAN_POINT('Origin',(-12.5687032866674,-24.,-11.0249576270339));
#143022=CARTESIAN_POINT('Origin',(-12.5687032866674,-24.4,-11.0249576270339));
#143023=CARTESIAN_POINT('Origin',(-9.35,-24.,-3.05000000003699));
#143024=CARTESIAN_POINT('',(-9.29674553898285,-24.,-12.2498458662666));
#143025=CARTESIAN_POINT('Origin',(-9.35,-24.,-3.05000000003699));
#143026=CARTESIAN_POINT('',(-9.61646521955773,-24.4,-11.845964772975));
#143027=CARTESIAN_POINT('Origin',(-9.35,-24.4,-3.05000000003699));
#143028=CARTESIAN_POINT('Ctrl Pts',(-9.61646521955773,-24.4,-11.845964772975));
#143029=CARTESIAN_POINT('Ctrl Pts',(-9.61574684903454,-24.4,-11.8469292690866));
#143030=CARTESIAN_POINT('Ctrl Pts',(-9.61502828402677,-24.3999966702549,
-11.8478936227214));
#143031=CARTESIAN_POINT('Ctrl Pts',(-9.58516778418947,-24.3997200467267,
-11.887951279054));
#143032=CARTESIAN_POINT('Ctrl Pts',(-9.55564185868478,-24.3939779655324,
-11.9268827633724));
#143033=CARTESIAN_POINT('Ctrl Pts',(-9.49847236767601,-24.3718197176192,
-12.0010201299338));
#143034=CARTESIAN_POINT('Ctrl Pts',(-9.47064424094682,-24.3556254163147,
-12.0364970754362));
#143035=CARTESIAN_POINT('Ctrl Pts',(-9.41249687350933,-24.307908789952,
-12.1095546655319));
#143036=CARTESIAN_POINT('Ctrl Pts',(-9.38271825407688,-24.2737132836985,
-12.146203631867));
#143037=CARTESIAN_POINT('Ctrl Pts',(-9.33855412802582,-24.1981575036158,
-12.1998901428329));
#143038=CARTESIAN_POINT('Ctrl Pts',(-9.32244973805791,-24.1600118608394,
-12.2191999208178));
#143039=CARTESIAN_POINT('Ctrl Pts',(-9.30191813777489,-24.0802759631265,
-12.2437190437141));
#143040=CARTESIAN_POINT('Ctrl Pts',(-9.29674553898285,-24.0405572215704,
-12.2498458662666));
#143041=CARTESIAN_POINT('Ctrl Pts',(-9.29674553898285,-24.,-12.2498458662666));
#143042=CARTESIAN_POINT('Origin',(-5.65685424949238,-24.,-12.900000000019));
#143043=CARTESIAN_POINT('',(-3.34147109452317,-23.9860345655466,-10.0168917310781));
#143044=CARTESIAN_POINT('',(-9.29699352038222,-23.9860345613817,-12.2498472983957));
#143045=CARTESIAN_POINT('Origin',(-5.65685424949238,-23.9860345609261,-12.900000000019));
#143046=CARTESIAN_POINT('Ctrl Pts',(-9.29674553898285,-24.,-12.2498458662666));
#143047=CARTESIAN_POINT('Ctrl Pts',(-9.29674553898285,-23.9953402268027,
-12.2498458662666));
#143048=CARTESIAN_POINT('Ctrl Pts',(-9.29682833839145,-23.9906843935221,
-12.2498463466717));
#143049=CARTESIAN_POINT('Ctrl Pts',(-9.29699352039839,-23.9860345613823,
-12.2498472983958));
#143050=CARTESIAN_POINT('Origin',(-5.65685424949238,-24.4,-12.900000000019));
#143051=CARTESIAN_POINT('Ctrl Pts',(-3.34147109439903,-23.9860345655524,
-10.0168917309711));
#143052=CARTESIAN_POINT('Ctrl Pts',(-3.341509443135,-23.9874600657353,-10.0169248044703));
#143053=CARTESIAN_POINT('Ctrl Pts',(-3.34154193167206,-23.9888862421037,
-10.0169528233557));
#143054=CARTESIAN_POINT('Ctrl Pts',(-3.34162881025419,-23.9935434575362,
-10.0170277488358));
#143055=CARTESIAN_POINT('Ctrl Pts',(-3.34165888869614,-23.9967726737154,
-10.0170536879467));
#143056=CARTESIAN_POINT('Ctrl Pts',(-3.34165888869614,-24.,-10.0170536879467));
#143057=CARTESIAN_POINT('Origin',(-10.5340572614694,-19.9,-6.30084733597289));
#143058=CARTESIAN_POINT('',(-13.0883185289381,-20.,-10.7249576270339));
#143059=CARTESIAN_POINT('',(-13.0883185289381,-19.9,-10.7249576270339));
#143060=CARTESIAN_POINT('',(-10.7906143361206,-20.,-6.74521722430999));
#143061=CARTESIAN_POINT('',(-11.083848469093,-20.,-7.25311364113158));
#143062=CARTESIAN_POINT('',(-10.7906143361206,-21.1,-6.74521722430999));
#143063=CARTESIAN_POINT('Origin',(-12.5687032866674,-19.9,-11.0249576270339));
#143064=CARTESIAN_POINT('',(-12.7932639810861,-20.,-11.5813500196151));
#143065=CARTESIAN_POINT('',(-12.7932639810861,-19.9,-11.5813500196151));
#143066=CARTESIAN_POINT('Origin',(-12.5687032866674,-20.,-11.0249576270339));
#143067=CARTESIAN_POINT('Origin',(-5.65685424949238,-23.8568542494924,-12.900000000019));
#143068=CARTESIAN_POINT('Ctrl Pts',(-3.34147109439903,-23.9860345655524,
-10.0168917309711));
#143069=CARTESIAN_POINT('Ctrl Pts',(-3.33980474884187,-23.9240931491361,
-10.0154546072388));
#143070=CARTESIAN_POINT('Ctrl Pts',(-3.33933631565976,-23.8620596978386,
-10.0150501085589));
#143071=CARTESIAN_POINT('Ctrl Pts',(-3.34007057236773,-23.8,-10.0156836186691));
#143072=CARTESIAN_POINT('Ctrl Pts',(-3.34678531450252,-23.2324670603222,
-10.0214770380324));
#143073=CARTESIAN_POINT('Ctrl Pts',(-3.45749112478326,-22.6438394405351,
-10.1208452048344));
#143074=CARTESIAN_POINT('Ctrl Pts',(-3.79210650744726,-21.8648455084378,
-10.3828564688412));
#143075=CARTESIAN_POINT('Ctrl Pts',(-3.93516684582503,-21.6185652596727,
-10.4905697000702));
#143076=CARTESIAN_POINT('Ctrl Pts',(-4.27387597232643,-21.1849574912198,
-10.7256407182475));
#143077=CARTESIAN_POINT('Ctrl Pts',(-4.46961146676767,-20.9976223772148,
-10.8528595348611));
#143078=CARTESIAN_POINT('Ctrl Pts',(-4.88103383123282,-20.7104988261178,
-11.0948576110964));
#143079=CARTESIAN_POINT('Ctrl Pts',(-5.11310773771486,-20.5923839396418,
-11.2209466582962));
#143080=CARTESIAN_POINT('Ctrl Pts',(-5.60871935569803,-20.4371939821691,
-11.4594259875479));
#143081=CARTESIAN_POINT('Ctrl Pts',(-5.87241302260401,-20.4001685914811,
-11.5715243725022));
#143082=CARTESIAN_POINT('Ctrl Pts',(-6.36784226154627,-20.4001685914811,
-11.7572799449367));
#143083=CARTESIAN_POINT('Ctrl Pts',(-6.64023366360302,-20.4371939821691,
-11.8461805746377));
#143084=CARTESIAN_POINT('Ctrl Pts',(-7.17046372693134,-20.5923839396418,
-11.9923289454911));
#143085=CARTESIAN_POINT('Ctrl Pts',(-7.4282279911993,-20.7104988261178,
-12.0498991631386));
#143086=CARTESIAN_POINT('Ctrl Pts',(-7.89733525228042,-20.9976223772148,
-12.1380456802828));
#143087=CARTESIAN_POINT('Ctrl Pts',(-8.12846146141512,-21.1849574912198,
-12.1708738166254));
#143088=CARTESIAN_POINT('Ctrl Pts',(-8.53822541702071,-21.6185652596727,
-12.2164342890631));
#143089=CARTESIAN_POINT('Ctrl Pts',(-8.71683712981021,-21.8648455084378,
-12.2293283440095));
#143090=CARTESIAN_POINT('Ctrl Pts',(-9.14122841916257,-22.6438394405351,
-12.2518980206493));
#143091=CARTESIAN_POINT('Ctrl Pts',(-9.28997465514599,-23.2324670603222,
-12.2498084550781));
#143092=CARTESIAN_POINT('Ctrl Pts',(-9.29884308443129,-23.8,-12.2498577690457));
#143093=CARTESIAN_POINT('Ctrl Pts',(-9.299812397741,-23.8620309656229,-12.2498631590289));
#143094=CARTESIAN_POINT('Ctrl Pts',(-9.29919497128662,-23.9240642722867,
-12.2498599824283));
#143095=CARTESIAN_POINT('Ctrl Pts',(-9.29699352039839,-23.9860345613823,
-12.2498472983958));
#143096=CARTESIAN_POINT('Origin',(-9.35,-19.9,-3.05000000003699));
#143097=CARTESIAN_POINT('',(-15.0167338549885,-20.,-10.2976290893825));
#143098=CARTESIAN_POINT('',(-15.0167338549885,-19.9,-10.2976290893825));
#143099=CARTESIAN_POINT('Origin',(-9.35,-20.,-3.05000000003699));
#143100=CARTESIAN_POINT('',(-0.631395349681702,-20.,-5.98699386306226));
#143101=CARTESIAN_POINT('',(-0.631395349681702,-19.9,-5.98699386306226));
#143102=CARTESIAN_POINT('',(-0.294290142826895,-20.,-4.67299691398904));
#143103=CARTESIAN_POINT('Origin',(-9.35,-20.,-3.05000000003699));
#143104=CARTESIAN_POINT('',(-0.294290142826894,-19.2199531690376,-4.67299691398904));
#143105=CARTESIAN_POINT('',(-0.294290142826896,-19.9,-4.67299691398904));
#143106=CARTESIAN_POINT('',(-0.298851850326922,-19.2053752002609,-4.69824669658142));
#143107=CARTESIAN_POINT('Origin',(-9.35,-20.1569908742018,-3.05000000003699));
#143108=CARTESIAN_POINT('',(-0.342996093127177,-19.1393368299495,-4.92453477474183));
#143109=CARTESIAN_POINT('Ctrl Pts',(-0.342996093127217,-19.1393368299494,
-4.92453477474201));
#143110=CARTESIAN_POINT('Ctrl Pts',(-0.338919064412081,-19.1408255450474,
-4.90494494687582));
#143111=CARTESIAN_POINT('Ctrl Pts',(-0.334921557723668,-19.1432424146486,
-4.88531258691514));
#143112=CARTESIAN_POINT('Ctrl Pts',(-0.331000810775166,-19.1466300793749,
-4.8658317759892));
#143113=CARTESIAN_POINT('Ctrl Pts',(-0.327439080338206,-19.149707541074,
-4.84813479168418));
#143114=CARTESIAN_POINT('Ctrl Pts',(-0.323940103826726,-19.1535851808526,
-4.83056196821088));
#143115=CARTESIAN_POINT('Ctrl Pts',(-0.320545023409296,-19.1582941278276,
-4.81325056669589));
#143116=CARTESIAN_POINT('Ctrl Pts',(-0.319571527254381,-19.1596443585174,
-4.80828674235626));
#143117=CARTESIAN_POINT('Ctrl Pts',(-0.318606891114168,-19.1610629779184,
-4.8033444026678));
#143118=CARTESIAN_POINT('Ctrl Pts',(-0.317652896980343,-19.1625508569463,
-4.79842681298157));
#143119=CARTESIAN_POINT('Ctrl Pts',(-0.314288911428832,-19.1677974338119,
-4.78108634927618));
#143120=CARTESIAN_POINT('Ctrl Pts',(-0.311033236905911,-19.1739224599097,
-4.76399853811601));
#143121=CARTESIAN_POINT('Ctrl Pts',(-0.30788938154976,-19.1810057026344,
-4.7472968131946));
#143122=CARTESIAN_POINT('Ctrl Pts',(-0.304916277889118,-19.1877042343697,
-4.73150220629397));
#143123=CARTESIAN_POINT('Ctrl Pts',(-0.302043295501447,-19.1952595294941,
-4.71605245153));
#143124=CARTESIAN_POINT('Ctrl Pts',(-0.299306816945607,-19.2037448874674,
-4.70109451849818));
#143125=CARTESIAN_POINT('Ctrl Pts',(-0.299149655135435,-19.2042322197054,
-4.70023545244532));
#143126=CARTESIAN_POINT('Ctrl Pts',(-0.29899295283953,-19.2047226217816,
-4.69937801956356));
#143127=CARTESIAN_POINT('Ctrl Pts',(-0.298836720346318,-19.2052161083662,
-4.69852225182618));
#143128=CARTESIAN_POINT('',(-1.,-18.2,-6.91231795691211));
#143129=CARTESIAN_POINT('Ctrl Pts',(-0.342996093127179,-19.1393368299495,
-4.92453477474183));
#143130=CARTESIAN_POINT('Ctrl Pts',(-0.390027426021725,-19.1221634764483,
-5.15051692500272));
#143131=CARTESIAN_POINT('Ctrl Pts',(-0.444566627282946,-19.0983023390303,
-5.36921499635279));
#143132=CARTESIAN_POINT('Ctrl Pts',(-0.57830980171757,-19.020446191969,
-5.83793682181643));
#143133=CARTESIAN_POINT('Ctrl Pts',(-0.682583950067457,-18.9451070919295,
-6.14520550751075));
#143134=CARTESIAN_POINT('Ctrl Pts',(-0.813666835274515,-18.7846217981295,
-6.48259695343331));
#143135=CARTESIAN_POINT('Ctrl Pts',(-0.860880288003759,-18.7154616839175,
-6.59730399074034));
#143136=CARTESIAN_POINT('Ctrl Pts',(-0.923475479616496,-18.588207088439,
-6.7429762948862));
#143137=CARTESIAN_POINT('Ctrl Pts',(-0.950034610743345,-18.5217732832391,
-6.80269945385084));
#143138=CARTESIAN_POINT('Ctrl Pts',(-0.978869456157098,-18.408184197995,
-6.86637474789097));
#143139=CARTESIAN_POINT('Ctrl Pts',(-0.986675532106876,-18.3679906488546,
-6.8834002020665));
#143140=CARTESIAN_POINT('Ctrl Pts',(-0.997241481275889,-18.2851363950946,
-6.90637026654278));
#143141=CARTESIAN_POINT('Ctrl Pts',(-1.,-18.2424763716807,-6.91231795691211));
#143142=CARTESIAN_POINT('Ctrl Pts',(-1.,-18.2,-6.91231795691211));
#143143=CARTESIAN_POINT('',(-0.707045437301172,-17.4928318802494,-6.20267131609953));
#143144=CARTESIAN_POINT('Ctrl Pts',(-1.,-18.2,-6.91231795691211));
#143145=CARTESIAN_POINT('Ctrl Pts',(-1.,-18.1575236283193,-6.91231795691211));
#143146=CARTESIAN_POINT('Ctrl Pts',(-0.997241481275889,-18.1148636049054,
-6.90637026654278));
#143147=CARTESIAN_POINT('Ctrl Pts',(-0.986675532106877,-18.0320093511454,
-6.88340020206649));
#143148=CARTESIAN_POINT('Ctrl Pts',(-0.978869456157098,-17.991815802005,
-6.86637474789097));
#143149=CARTESIAN_POINT('Ctrl Pts',(-0.950034610743345,-17.8782267167609,
-6.80269945385084));
#143150=CARTESIAN_POINT('Ctrl Pts',(-0.923475479616496,-17.811792911561,
-6.7429762948862));
#143151=CARTESIAN_POINT('Ctrl Pts',(-0.860880288003759,-17.6845383160825,
-6.59730399074034));
#143152=CARTESIAN_POINT('Ctrl Pts',(-0.813666835274515,-17.6153782018705,
-6.48259695343331));
#143153=CARTESIAN_POINT('Ctrl Pts',(-0.75261478687592,-17.5406319380172,
-6.32545638658357));
#143154=CARTESIAN_POINT('Ctrl Pts',(-0.729894647720439,-17.5156771266932,
-6.2653117462773));
#143155=CARTESIAN_POINT('Ctrl Pts',(-0.707045437301173,-17.4928318802494,
-6.20267131609953));
#143156=CARTESIAN_POINT('',(-0.689573580943891,-17.4676466969021,-6.15435407779857));
#143157=CARTESIAN_POINT('Ctrl Pts',(-0.689576769163932,-17.4676488696199,
-6.15435513352118));
#143158=CARTESIAN_POINT('Ctrl Pts',(-0.692251029448898,-17.4728748513358,
-6.16181963780152));
#143159=CARTESIAN_POINT('Ctrl Pts',(-0.695047478275197,-17.4775916434185,
-6.16958981118521));
#143160=CARTESIAN_POINT('Ctrl Pts',(-0.697949233001934,-17.4817806390516,
-6.17760927298781));
#143161=CARTESIAN_POINT('Ctrl Pts',(-0.700891780631754,-17.4860285236359,
-6.18574147248153));
#143162=CARTESIAN_POINT('Ctrl Pts',(-0.70393704643326,-17.48972582708,-6.19411510571193));
#143163=CARTESIAN_POINT('Ctrl Pts',(-0.707067566378145,-17.4928576526749,
-6.20267384590877));
#143164=CARTESIAN_POINT('',(-0.605214914090966,-17.2952175137768,-5.90809968361399));
#143165=CARTESIAN_POINT('Origin',(-9.35,-15.2939545703814,-3.05000000003699));
#143166=CARTESIAN_POINT('',(-0.294290142826895,-16.4303892440217,-4.67299691398904));
#143167=CARTESIAN_POINT('Origin',(-9.35,-15.2939545703814,-3.05000000003699));
#143168=CARTESIAN_POINT('',(-0.294290142826895,-15.9,-4.67299691398904));
#143169=CARTESIAN_POINT('',(-0.294290142826896,-19.9,-4.67299691398904));
#143170=CARTESIAN_POINT('',(-16.5700864372805,-15.9,-8.75178496951782));
#143171=CARTESIAN_POINT('Origin',(-9.35,-15.9,-3.05000000003699));
#143172=CARTESIAN_POINT('',(-16.5700864372805,-20.,-8.75178496951782));
#143173=CARTESIAN_POINT('',(-16.5700864372805,-19.9,-8.75178496951782));
#143174=CARTESIAN_POINT('',(-15.3208637689692,-20.,-10.0491989436598));
#143175=CARTESIAN_POINT('Origin',(-9.35,-20.,-3.05000000003699));
#143176=CARTESIAN_POINT('',(-15.3208637689692,-19.9,-10.0491989436598));
#143177=CARTESIAN_POINT('Origin',(-3.45175358661618,-24.4,-3.05000000003699));
#143178=CARTESIAN_POINT('Origin',(-9.35,-24.,-3.05000000003699));
#143179=CARTESIAN_POINT('',(-0.631395349681703,-24.,-0.11300613701172));
#143180=CARTESIAN_POINT('',(-1.01046511708685,-24.4,-0.240701522360645));
#143181=CARTESIAN_POINT('Origin',(-1.01046511708685,-24.,-0.240701522360645));
#143182=CARTESIAN_POINT('',(-12.6435568514736,-24.4,5.11042175782032));
#143183=CARTESIAN_POINT('Origin',(-9.35,-24.4,-3.05000000003699));
#143184=CARTESIAN_POINT('',(-12.7932639810861,-24.,5.4813500195411));
#143185=CARTESIAN_POINT('Origin',(-12.6435568514736,-24.,5.11042175782032));
#143186=CARTESIAN_POINT('Origin',(-9.35,-24.,-3.05000000003699));
#143187=CARTESIAN_POINT('Ctrl Pts',(-12.7932639810861,-24.,5.4813500195411));
#143188=CARTESIAN_POINT('Ctrl Pts',(-13.046887978923,-24.,5.37898704363615));
#143189=CARTESIAN_POINT('Ctrl Pts',(-13.135978738899,-24.,5.12040214925567));
#143190=CARTESIAN_POINT('Ctrl Pts',(-13.2250694988751,-24.,4.86181725487519));
#143191=CARTESIAN_POINT('Ctrl Pts',(-13.0883185289381,-24.,4.62495762695992));
#143192=CARTESIAN_POINT('Ctrl Pts',(-12.7932639810861,-24.4,5.4813500195411));
#143193=CARTESIAN_POINT('Ctrl Pts',(-13.046887978923,-24.4,5.37898704363615));
#143194=CARTESIAN_POINT('Ctrl Pts',(-13.135978738899,-24.4,5.12040214925567));
#143195=CARTESIAN_POINT('Ctrl Pts',(-13.2250694988751,-24.4,4.86181725487519));
#143196=CARTESIAN_POINT('Ctrl Pts',(-13.0883185289381,-24.4,4.62495762695992));
#143197=CARTESIAN_POINT('Ctrl Pts',(-12.6435568514736,-24.4,5.11042175782032));
#143198=CARTESIAN_POINT('Ctrl Pts',(-12.7280981840859,-24.4,5.076300765852));
#143199=CARTESIAN_POINT('Ctrl Pts',(-12.757795104078,-24.4,4.99010580105851));
#143200=CARTESIAN_POINT('Ctrl Pts',(-12.78749202407,-24.4,4.90391083626501));
#143201=CARTESIAN_POINT('Ctrl Pts',(-12.7419083674243,-24.4,4.82495762695992));
#143202=CARTESIAN_POINT('',(-12.7419083674243,-24.4,4.82495762695992));
#143203=CARTESIAN_POINT('',(-13.0883185289381,-24.,4.62495762695992));
#143204=CARTESIAN_POINT('Origin',(-12.7419083674243,-24.,4.82495762695992));
#143205=CARTESIAN_POINT('Origin',(-12.5687032866674,-24.,4.92495762695992));
#143206=CARTESIAN_POINT('Origin',(-12.5687032866674,-24.4,4.92495762695992));
#143207=CARTESIAN_POINT('Origin',(-10.0881676893362,-24.,0.228543942399029));
#143208=CARTESIAN_POINT('',(-10.4442041746068,-24.4,0.845217224235998));
#143209=CARTESIAN_POINT('',(-10.7906143361206,-24.,0.645217224235999));
#143210=CARTESIAN_POINT('Origin',(-10.4442041746068,-24.,0.845217224235998));
#143211=CARTESIAN_POINT('',(-10.43457785085,-24.,0.0285439423990298));
#143212=CARTESIAN_POINT('',(-10.0881676893362,-24.4,0.228543942399029));
#143213=CARTESIAN_POINT('Ctrl Pts',(-10.7906143361206,-24.,0.645217224236));
#143214=CARTESIAN_POINT('Ctrl Pts',(-10.5687015536612,-24.,0.260853010167357));
#143215=CARTESIAN_POINT('Ctrl Pts',(-10.1362187386524,-24.,0.360551288976537));
#143216=CARTESIAN_POINT('Ctrl Pts',(-10.7906143361206,-24.4,0.645217224236));
#143217=CARTESIAN_POINT('Ctrl Pts',(-10.5687015536612,-24.4,0.260853010167357));
#143218=CARTESIAN_POINT('Ctrl Pts',(-10.1362187386524,-24.4,0.360551288976537));
#143219=CARTESIAN_POINT('Ctrl Pts',(-10.4442041746068,-24.4,0.845217224235999));
#143220=CARTESIAN_POINT('Ctrl Pts',(-10.3702332471204,-24.4,0.717095819546453));
#143221=CARTESIAN_POINT('Ctrl Pts',(-10.2260723087841,-24.4,0.750328579149512));
#143222=CARTESIAN_POINT('',(-10.2260723087841,-24.4,0.750328579149511));
#143223=CARTESIAN_POINT('Origin',(-10.2260723087841,-24.,0.750328579149511));
#143224=CARTESIAN_POINT('Origin',(-10.2709990938499,-24.,0.945217224235998));
#143225=CARTESIAN_POINT('Origin',(-10.2709990938499,-24.4,0.945217224235998));
#143226=CARTESIAN_POINT('Origin',(-9.35,-24.,-3.05000000003699));
#143227=CARTESIAN_POINT('',(-5.62078275330442,-24.4,-1.90853658540285));
#143228=CARTESIAN_POINT('Origin',(-5.62078275330442,-24.,-1.90853658540285));
#143229=CARTESIAN_POINT('Origin',(-9.35,-24.4,-3.05000000003699));
#143230=CARTESIAN_POINT('Ctrl Pts',(-6.00326657347833,-24.,-2.02560975613455));
#143231=CARTESIAN_POINT('Ctrl Pts',(-5.87336640813625,-24.,-2.45000000003699));
#143232=CARTESIAN_POINT('Ctrl Pts',(-5.42954084321747,-24.,-2.45000000003699));
#143233=CARTESIAN_POINT('Ctrl Pts',(-6.00326657347833,-24.4,-2.02560975613455));
#143234=CARTESIAN_POINT('Ctrl Pts',(-5.87336640813625,-24.4,-2.45000000003699));
#143235=CARTESIAN_POINT('Ctrl Pts',(-5.42954084321747,-24.4,-2.45000000003699));
#143236=CARTESIAN_POINT('Ctrl Pts',(-5.62078275330442,-24.4,-1.90853658540285));
#143237=CARTESIAN_POINT('Ctrl Pts',(-5.57748269819039,-24.4,-2.05000000003699));
#143238=CARTESIAN_POINT('Ctrl Pts',(-5.42954084321747,-24.4,-2.05000000003699));
#143239=CARTESIAN_POINT('',(-5.42954084321747,-24.4,-2.05000000003699));
#143240=CARTESIAN_POINT('',(-5.42954084321747,-24.,-2.45000000003699));
#143241=CARTESIAN_POINT('Origin',(-5.42954084321747,-24.,-2.05000000003699));
#143242=CARTESIAN_POINT('Origin',(-5.42954084321747,-24.,-1.85000000003699));
#143243=CARTESIAN_POINT('Origin',(-5.42954084321747,-24.4,-1.85000000003699));
#143244=CARTESIAN_POINT('Origin',(-4.69720428956801,-24.,-2.05000000003699));
#143245=CARTESIAN_POINT('',(-1.20000000078942,-24.4,-2.05000000003699));
#143246=CARTESIAN_POINT('',(-1.20000000078942,-24.,-2.45000000003699));
#143247=CARTESIAN_POINT('Origin',(-1.20000000078942,-24.,-2.05000000003699));
#143248=CARTESIAN_POINT('',(-4.69720428956801,-24.,-2.45000000003699));
#143249=CARTESIAN_POINT('',(-4.69720428956801,-24.4,-2.05000000003699));
#143250=CARTESIAN_POINT('Ctrl Pts',(-1.20000000078942,-24.,-2.45000000003699));
#143251=CARTESIAN_POINT('Ctrl Pts',(-0.600000000789417,-24.,-2.45000000003699));
#143252=CARTESIAN_POINT('Ctrl Pts',(-0.600000000789417,-24.,-1.85000000003699));
#143253=CARTESIAN_POINT('Ctrl Pts',(-1.20000000078942,-24.4,-2.45000000003699));
#143254=CARTESIAN_POINT('Ctrl Pts',(-0.600000000789417,-24.4,-2.45000000003699));
#143255=CARTESIAN_POINT('Ctrl Pts',(-0.600000000789417,-24.4,-1.85000000003699));
#143256=CARTESIAN_POINT('Ctrl Pts',(-1.20000000078942,-24.4,-2.05000000003699));
#143257=CARTESIAN_POINT('Ctrl Pts',(-1.00000000078942,-24.4,-2.05000000003699));
#143258=CARTESIAN_POINT('Ctrl Pts',(-1.00000000078942,-24.4,-1.85000000003699));
#143259=CARTESIAN_POINT('',(-1.00000000078942,-24.4,-1.85000000003699));
#143260=CARTESIAN_POINT('',(-0.600000000789417,-24.,-1.85000000003699));
#143261=CARTESIAN_POINT('Origin',(-1.00000000078942,-24.,-1.85000000003699));
#143262=CARTESIAN_POINT('Origin',(-1.20000000078942,-24.,-1.85000000003699));
#143263=CARTESIAN_POINT('Origin',(-1.20000000078942,-24.4,-1.85000000003699));
#143264=CARTESIAN_POINT('Origin',(-1.00000000078942,-24.,-1.33262554947194));
#143265=CARTESIAN_POINT('',(-1.00000000078942,-24.4,-0.304549215035108));
#143266=CARTESIAN_POINT('',(-0.600000000789418,-24.,-0.304549215035108));
#143267=CARTESIAN_POINT('Origin',(-1.00000000078942,-24.,-0.304549215035108));
#143268=CARTESIAN_POINT('',(-0.600000000789417,-24.,-1.33262554947194));
#143269=CARTESIAN_POINT('',(-1.00000000078942,-24.4,-1.33262554947194));
#143270=CARTESIAN_POINT('Ctrl Pts',(-0.600000000789417,-24.,-0.304549215035108));
#143271=CARTESIAN_POINT('Ctrl Pts',(-0.600000000789417,-24.,-0.206204709299061));
#143272=CARTESIAN_POINT('Ctrl Pts',(-0.631395349681703,-24.,-0.113006137011717));
#143273=CARTESIAN_POINT('Ctrl Pts',(-0.600000000789417,-24.4,-0.304549215035108));
#143274=CARTESIAN_POINT('Ctrl Pts',(-0.600000000789417,-24.4,-0.206204709299061));
#143275=CARTESIAN_POINT('Ctrl Pts',(-0.631395349681703,-24.4,-0.113006137011717));
#143276=CARTESIAN_POINT('Ctrl Pts',(-1.00000000078942,-24.4,-0.304549215035108));
#143277=CARTESIAN_POINT('Ctrl Pts',(-1.00000000078942,-24.4,-0.271767713123092));
#143278=CARTESIAN_POINT('Ctrl Pts',(-1.01046511708685,-24.4,-0.240701522360645));
#143279=CARTESIAN_POINT('Origin',(-1.20000000078942,-24.,-0.304549215035108));
#143280=CARTESIAN_POINT('Origin',(-1.20000000078942,-24.4,-0.304549215035108));
#143281=CARTESIAN_POINT('Origin',(-5.94265499251984,-19.9,-2.45000000003699));
#143282=CARTESIAN_POINT('',(-1.20000000078942,-20.,-2.45000000003699));
#143283=CARTESIAN_POINT('',(-1.20000000078942,-19.9,-2.45000000003699));
#143284=CARTESIAN_POINT('',(-5.42954084321747,-20.,-2.45000000003699));
#143285=CARTESIAN_POINT('',(-4.29148370813747,-20.,-2.45000000003699));
#143286=CARTESIAN_POINT('',(-5.42954084321747,-21.1,-2.45000000003699));
#143287=CARTESIAN_POINT('Origin',(-1.20000000078942,-19.9,-1.85000000003699));
#143288=CARTESIAN_POINT('',(-0.600000000789417,-20.,-1.85000000003699));
#143289=CARTESIAN_POINT('',(-0.600000000789418,-19.9,-1.85000000003699));
#143290=CARTESIAN_POINT('Origin',(-1.20000000078942,-20.,-1.85000000003699));
#143291=CARTESIAN_POINT('Origin',(-0.600000000789418,-19.9,0.384748901093117));
#143292=CARTESIAN_POINT('',(-0.600000000789418,-20.,-0.304549215035106));
#143293=CARTESIAN_POINT('',(-0.600000000789418,-19.9,-0.304549215035106));
#143294=CARTESIAN_POINT('',(-0.600000000789418,-20.,-0.0326255494647287));
#143295=CARTESIAN_POINT('Origin',(-1.20000000078942,-19.9,-0.304549215035106));
#143296=CARTESIAN_POINT('',(-0.631395349681703,-20.,-0.113006137011719));
#143297=CARTESIAN_POINT('',(-0.631395349681703,-19.9,-0.113006137011719));
#143298=CARTESIAN_POINT('Origin',(-1.20000000078942,-20.,-0.304549215035107));
#143299=CARTESIAN_POINT('Origin',(-9.35,-19.9,-3.05000000003699));
#143300=CARTESIAN_POINT('',(-12.7932639810861,-20.,5.4813500195411));
#143301=CARTESIAN_POINT('',(-12.7932639810861,-19.9,5.4813500195411));
#143302=CARTESIAN_POINT('',(-15.8187500000085,-20.,3.49180964541969));
#143303=CARTESIAN_POINT('Origin',(-9.35,-20.,-3.05000000003699));
#143304=CARTESIAN_POINT('',(-15.8187500000085,-15.9,3.49180964541969));
#143305=CARTESIAN_POINT('',(-15.8187500000085,-19.9,3.49180964541969));
#143306=CARTESIAN_POINT('',(-0.259697928570093,-15.9,-1.63352259105473));
#143307=CARTESIAN_POINT('Origin',(-9.35,-15.9,-3.05000000003699));
#143308=CARTESIAN_POINT('',(-0.259697928570093,-16.4335328638949,-1.63352259105473));
#143309=CARTESIAN_POINT('',(-0.259697928570092,-19.9,-1.63352259105473));
#143310=CARTESIAN_POINT('',(-0.522069917640389,-17.2551814608384,-0.460086785087467));
#143311=CARTESIAN_POINT('Origin',(-9.35,-15.4417047044218,-3.05000000003699));
#143312=CARTESIAN_POINT('',(-0.703370836441857,-17.4891769091775,0.092579212634288));
#143313=CARTESIAN_POINT('Ctrl Pts',(-0.703370836454029,-17.4891769091919,
0.0925792126665254));
#143314=CARTESIAN_POINT('Ctrl Pts',(-0.658863507426592,-17.4451361940672,
-0.0298801887081493));
#143315=CARTESIAN_POINT('Ctrl Pts',(-0.616842608901601,-17.4065266547297,
-0.154129592507691));
#143316=CARTESIAN_POINT('Ctrl Pts',(-0.560016497085532,-17.3303629754732,
-0.333206402781313));
#143317=CARTESIAN_POINT('Ctrl Pts',(-0.539569532605825,-17.2969480440437,
-0.400437922534331));
#143318=CARTESIAN_POINT('Ctrl Pts',(-0.522069917640389,-17.2551814608384,
-0.46008678508747));
#143319=CARTESIAN_POINT('',(-1.,-18.2,0.812317956838124));
#143320=CARTESIAN_POINT('Ctrl Pts',(-0.703370836441977,-17.48917690918,
0.092579212633367));
#143321=CARTESIAN_POINT('Ctrl Pts',(-0.727460088883102,-17.5130136104037,
0.158859429802102));
#143322=CARTESIAN_POINT('Ctrl Pts',(-0.751446619517419,-17.5392017461089,
0.222449665429705));
#143323=CARTESIAN_POINT('Ctrl Pts',(-0.813666835274514,-17.6153782018705,
0.382596953359324));
#143324=CARTESIAN_POINT('Ctrl Pts',(-0.860880288003759,-17.6845383160825,
0.497303990666353));
#143325=CARTESIAN_POINT('Ctrl Pts',(-0.923475479616496,-17.811792911561,
0.642976294812216));
#143326=CARTESIAN_POINT('Ctrl Pts',(-0.950034610743346,-17.8782267167609,
0.702699453776853));
#143327=CARTESIAN_POINT('Ctrl Pts',(-0.978869456157099,-17.991815802005,
0.766374747816984));
#143328=CARTESIAN_POINT('Ctrl Pts',(-0.986675532106877,-18.0320093511454,
0.783400201992511));
#143329=CARTESIAN_POINT('Ctrl Pts',(-0.997241481275889,-18.1148636049054,
0.806370266468799));
#143330=CARTESIAN_POINT('Ctrl Pts',(-1.,-18.1575236283193,0.812317956838124));
#143331=CARTESIAN_POINT('Ctrl Pts',(-1.,-18.2,0.812317956838124));
#143332=CARTESIAN_POINT('',(-0.2950380218237,-19.1554855130662,-1.42283572628271));
#143333=CARTESIAN_POINT('Ctrl Pts',(-1.,-18.2,0.812317956838124));
#143334=CARTESIAN_POINT('Ctrl Pts',(-1.,-18.2424763716807,0.812317956838124));
#143335=CARTESIAN_POINT('Ctrl Pts',(-0.997241481275889,-18.2851363950946,
0.806370266468801));
#143336=CARTESIAN_POINT('Ctrl Pts',(-0.986675532106876,-18.3679906488546,
0.783400201992511));
#143337=CARTESIAN_POINT('Ctrl Pts',(-0.978869456157098,-18.408184197995,
0.766374747816981));
#143338=CARTESIAN_POINT('Ctrl Pts',(-0.950034610743345,-18.5217732832391,
0.70269945377685));
#143339=CARTESIAN_POINT('Ctrl Pts',(-0.923475479616496,-18.588207088439,
0.642976294812216));
#143340=CARTESIAN_POINT('Ctrl Pts',(-0.860880288003759,-18.7154616839175,
0.497303990666353));
#143341=CARTESIAN_POINT('Ctrl Pts',(-0.813666835274514,-18.7846217981295,
0.382596953359324));
#143342=CARTESIAN_POINT('Ctrl Pts',(-0.682583950067456,-18.9451070919295,
0.0452055074367616));
#143343=CARTESIAN_POINT('Ctrl Pts',(-0.57830980171757,-19.020446191969,
-0.262063178257554));
#143344=CARTESIAN_POINT('Ctrl Pts',(-0.423429326492426,-19.1106070327523,
-0.804863656734993));
#143345=CARTESIAN_POINT('Ctrl Pts',(-0.351385643958767,-19.1380863052892,
-1.10926838448257));
#143346=CARTESIAN_POINT('Ctrl Pts',(-0.295038021823737,-19.1554855130657,
-1.42283572628275));
#143347=CARTESIAN_POINT('',(-0.260663520072962,-19.2137914246021,-1.62733969108494));
#143348=CARTESIAN_POINT('Ctrl Pts',(-0.260663520072961,-19.2137914246021,
-1.62733969108494));
#143349=CARTESIAN_POINT('Ctrl Pts',(-0.263049439156941,-19.2049905456179,
-1.61209612153309));
#143350=CARTESIAN_POINT('Ctrl Pts',(-0.26556279235318,-19.197231830287,
-1.5962907461053));
#143351=CARTESIAN_POINT('Ctrl Pts',(-0.276256418693354,-19.1697212655996,
-1.53022122955726));
#143352=CARTESIAN_POINT('Ctrl Pts',(-0.285408690980658,-19.1584588901442,
-1.47642172621256));
#143353=CARTESIAN_POINT('Ctrl Pts',(-0.295038021824301,-19.1554855130655,
-1.42283572627961));
#143354=CARTESIAN_POINT('',(-0.259697928570093,-19.217361123564,-1.63352259105473));
#143355=CARTESIAN_POINT('Origin',(-9.35,-20.0351647369409,-3.05000000003699));
#143356=CARTESIAN_POINT('',(-0.259697928570092,-20.,-1.63352259105473));
#143357=CARTESIAN_POINT('',(-0.259697928570092,-19.9,-1.63352259105473));
#143358=CARTESIAN_POINT('Origin',(-9.35,-20.,-3.05000000003699));
#143359=CARTESIAN_POINT('Origin',(-3.45175358661618,-24.4,-3.05000000003699));
#143360=CARTESIAN_POINT('Origin',(-15.7000000000318,-22.8,-8.38137084992264));
#143361=CARTESIAN_POINT('',(-15.1343145750825,-20.,-8.94705627487188));
#143362=CARTESIAN_POINT('',(-15.1343145750825,-22.8,-8.94705627487188));
#143363=CARTESIAN_POINT('Origin',(-15.7000000000318,-20.,-8.38137084992264));
#143364=CARTESIAN_POINT('Origin',(-14.9000000000324,-22.8,-8.71274169982174));
#143365=CARTESIAN_POINT('',(-15.3557236788353,-20.,-9.16846537862466));
#143366=CARTESIAN_POINT('',(-15.3557236788353,-19.9,-9.16846537862467));
#143367=CARTESIAN_POINT('',(-14.4242364691429,-20.,-8.23697816893229));
#143368=CARTESIAN_POINT('Origin',(-14.9314596101234,-19.9,-9.5927294473366));
#143369=CARTESIAN_POINT('Origin',(-14.9314596101234,-20.,-9.5927294473366));
#143370=CARTESIAN_POINT('Origin',(-11.7246781315911,-10.3,-15.0676288747919));
#143371=CARTESIAN_POINT('',(-12.3207815844978,-10.3,-15.1358979998248));
#143372=CARTESIAN_POINT('',(-12.3207815844978,-10.3,-15.1358979998248));
#143373=CARTESIAN_POINT('Origin',(-11.7246781315911,-10.3,-15.0676288747919));
#143374=CARTESIAN_POINT('Origin',(-15.5,-10.3,-15.5));
#143375=CARTESIAN_POINT('Origin',(-15.5,-10.3,-15.5));
#143376=CARTESIAN_POINT('Origin',(-17.9000000000407,-24.4,-10.0156854249824));
#143377=CARTESIAN_POINT('',(-18.1828427125153,-15.9,-9.73284271250775));
#143378=CARTESIAN_POINT('',(-17.5000000000407,-15.9,-10.0156854249794));
#143379=CARTESIAN_POINT('Origin',(-17.9000000000407,-15.9,-10.0156854249824));
#143380=CARTESIAN_POINT('',(-17.5000000000407,-10.3,-10.0156854249794));
#143381=CARTESIAN_POINT('',(-17.5000000000407,-24.4,-10.0156854249794));
#143382=CARTESIAN_POINT('',(-18.1828427125153,-10.3,-9.73284271250775));
#143383=CARTESIAN_POINT('Origin',(-17.9000000000407,-10.3,-10.0156854249824));
#143384=CARTESIAN_POINT('',(-18.1828427125153,-24.4,-9.73284271250775));
#143385=CARTESIAN_POINT('Origin',(-16.5000000000311,-24.4,-8.05000000002354));
#143386=CARTESIAN_POINT('',(-17.1668459513761,-15.9,-8.71684595136846));
#143387=CARTESIAN_POINT('',(-13.2927206125707,-15.9,-4.84272061256308));
#143388=CARTESIAN_POINT('',(-18.8656854249492,-10.3,-10.4156854249416));
#143389=CARTESIAN_POINT('',(-7.38427091436115,-10.3,1.06572908564645));
#143390=CARTESIAN_POINT('',(-18.8656854249492,-25.4,-10.4156854249417));
#143391=CARTESIAN_POINT('',(-18.8656854249492,-24.4,-10.4156854249417));
#143392=CARTESIAN_POINT('',(-16.7343145750813,-25.4,-8.28431457507368));
#143393=CARTESIAN_POINT('',(-10.4750000000288,-25.4,-2.02500000002116));
#143394=CARTESIAN_POINT('',(-16.7343145750813,-20.,-8.28431457507368));
#143395=CARTESIAN_POINT('',(-16.7343145750813,-24.4,-8.28431457507368));
#143396=CARTESIAN_POINT('',(-17.1668459513761,-20.,-8.71684595136846));
#143397=CARTESIAN_POINT('',(-15.7899218940915,-20.,-7.33992189408395));
#143398=CARTESIAN_POINT('',(-17.1668459513761,-19.9,-8.71684595136846));
#143399=CARTESIAN_POINT('Origin',(-17.5000000000421,-22.8,-9.82772085584933));
#143400=CARTESIAN_POINT('',(-17.5000000000302,-15.9,-11.4373755457745));
#143401=CARTESIAN_POINT('',(-17.5000000000467,-15.9,-9.21712743154979));
#143402=CARTESIAN_POINT('',(-17.5000000000302,-10.3,-11.4373755457745));
#143403=CARTESIAN_POINT('',(-17.5000000000302,-10.3,-11.4373755457745));
#143404=CARTESIAN_POINT('',(-17.500000000174,-10.3,7.93725830003194));
#143405=CARTESIAN_POINT('Origin',(-16.8840032389014,-19.9,-8.99968866384308));
#143406=CARTESIAN_POINT('Origin',(-16.8840032389014,-15.9,-8.99968866384308));
#143407=CARTESIAN_POINT('Origin',(-16.8840032389014,-20.,-8.99968866384308));
#143408=CARTESIAN_POINT('Origin',(-14.6471642557501,-19.9,-9.82495762703391));
#143409=CARTESIAN_POINT('',(-14.1275490134794,-20.,-10.1249576270339));
#143410=CARTESIAN_POINT('',(-14.1275490134794,-19.9,-10.1249576270339));
#143411=CARTESIAN_POINT('Origin',(-14.6471642557501,-20.,-9.82495762703391));
#143412=CARTESIAN_POINT('Origin',(-18.3,-24.4,-10.9813708498909));
#143413=CARTESIAN_POINT('',(-19.1,-10.3,-10.9813708498909));
#143414=CARTESIAN_POINT('Origin',(-18.3,-10.3,-10.9813708498909));
#143415=CARTESIAN_POINT('',(-19.1,-25.4,-10.9813708498909));
#143416=CARTESIAN_POINT('',(-19.1,-24.4,-10.9813708498909));
#143417=CARTESIAN_POINT('Origin',(-18.3,-25.4,-10.9813708498909));
#143418=CARTESIAN_POINT('Origin',(-16.7000000000302,-10.3,-11.4373755457685));
#143419=CARTESIAN_POINT('',(-16.4733788179429,-15.9,-12.2046061759114));
#143420=CARTESIAN_POINT('Origin',(-16.7000000000302,-15.9,-11.4373755457685));
#143421=CARTESIAN_POINT('',(-16.4733788179429,-10.3,-12.2046061759113));
#143422=CARTESIAN_POINT('',(-16.4733788179429,-10.3,-12.2046061759113));
#143423=CARTESIAN_POINT('Origin',(-16.7000000000302,-10.3,-11.4373755457685));
#143424=CARTESIAN_POINT('Origin',(-15.5,-10.3,-15.5));
#143425=CARTESIAN_POINT('',(-13.9781746176887,-15.9,-12.419231543135));
#143426=CARTESIAN_POINT('Origin',(-15.5,-15.9,-15.5));
#143427=CARTESIAN_POINT('',(-13.9781746176887,-10.3,-12.419231543135));
#143428=CARTESIAN_POINT('',(-13.9781746176887,-10.3,-12.419231543135));
#143429=CARTESIAN_POINT('Origin',(-15.5,-10.3,-15.5));
#143430=CARTESIAN_POINT('Origin',(-19.1,-24.4,8.48528137429235));
#143431=CARTESIAN_POINT('',(-19.1,-10.3,-15.5));
#143432=CARTESIAN_POINT('',(-19.1,-10.3,9.07476980792574));
#143433=CARTESIAN_POINT('',(-19.1,-25.4,-15.5));
#143434=CARTESIAN_POINT('',(-19.1,-24.4,-15.5));
#143435=CARTESIAN_POINT('',(-19.1,-25.4,4.01764068713489));
#143436=CARTESIAN_POINT('Origin',(-15.5,-24.4,-15.5));
#143437=CARTESIAN_POINT('',(-15.5,-25.4,-19.1000000000451));
#143438=CARTESIAN_POINT('Origin',(-15.5,-25.4,-15.5));
#143439=CARTESIAN_POINT('',(-15.5,-10.3,-19.1000000000451));
#143440=CARTESIAN_POINT('Origin',(-15.5,-10.3,-15.5));
#143441=CARTESIAN_POINT('',(-15.5,-24.4,-19.1000000000451));
#143442=CARTESIAN_POINT('Origin',(-15.5,-20.8,-15.5));
#143443=CARTESIAN_POINT('',(-12.7,-20.8,-15.5));
#143444=CARTESIAN_POINT('Origin',(-15.5,-20.8,-15.5));
#143445=CARTESIAN_POINT('',(-17.1,-20.8,-15.5));
#143446=CARTESIAN_POINT('Origin',(-15.5,-20.8,-15.5));
#143447=CARTESIAN_POINT('Origin',(-15.5,-24.4,-15.5));
#143448=CARTESIAN_POINT('',(-17.1,-10.3,-15.5));
#143449=CARTESIAN_POINT('Origin',(-15.5,-10.3,-15.5));
#143450=CARTESIAN_POINT('',(-17.1,-24.4,-15.5));
#143451=CARTESIAN_POINT('Origin',(-15.5,-24.4,-15.5));
#143452=CARTESIAN_POINT('',(-12.7,-25.4,-15.5));
#143453=CARTESIAN_POINT('Origin',(-15.5,-25.4,-15.5));
#143454=CARTESIAN_POINT('',(-12.7,-24.4,-15.5));
#143455=CARTESIAN_POINT('Origin',(10.9,-22.1,-11.6000000000162));
#143456=CARTESIAN_POINT('',(10.9,-22.1,-12.5077037206369));
#143457=CARTESIAN_POINT('',(10.9,-22.1,-12.5077037206369));
#143458=CARTESIAN_POINT('',(10.9,-22.1,-15.1));
#143459=CARTESIAN_POINT('',(10.9,-22.1,-6.02500000001941));
#143460=CARTESIAN_POINT('',(10.9,-10.3,-15.1));
#143461=CARTESIAN_POINT('',(10.9,-22.1,-15.1));
#143462=CARTESIAN_POINT('',(10.9,-10.3,-13.800000000037));
#143463=CARTESIAN_POINT('',(10.9,-10.3,-11.6000000000162));
#143464=CARTESIAN_POINT('',(10.9,-15.9,-13.800000000037));
#143465=CARTESIAN_POINT('',(10.9,-18.9,-13.800000000037));
#143466=CARTESIAN_POINT('',(10.9,-15.9,-12.650000000037));
#143467=CARTESIAN_POINT('',(10.9,-15.9,-10.1032670035799));
#143468=CARTESIAN_POINT('',(10.9,-20.,-12.650000000037));
#143469=CARTESIAN_POINT('',(10.9,-21.,-12.650000000037));
#143470=CARTESIAN_POINT('',(10.9,-20.,-12.1857384988752));
#143471=CARTESIAN_POINT('',(10.9,-20.,-6.02500000001941));
#143472=CARTESIAN_POINT('',(10.9,-21.,-12.1857384988752));
#143473=CARTESIAN_POINT('Origin',(11.3,-22.1,-12.5077037206369));
#143474=CARTESIAN_POINT('',(11.6304347826087,-22.1,-12.7331207884076));
#143475=CARTESIAN_POINT('',(11.6304347826087,-22.1,-12.7331207884076));
#143476=CARTESIAN_POINT('Origin',(11.3,-22.1,-12.5077037206369));
#143477=CARTESIAN_POINT('Origin',(15.1,-22.1,-15.1));
#143478=CARTESIAN_POINT('',(15.1472108071229,-22.1,-10.9002653488952));
#143479=CARTESIAN_POINT('',(15.1472108071229,-22.1,-10.9002653488952));
#143480=CARTESIAN_POINT('Origin',(15.1,-22.1,-15.1));
#143481=CARTESIAN_POINT('Origin',(15.1562033418129,-22.1,-10.1003158915419));
#143482=CARTESIAN_POINT('Origin',(15.1562033418129,-22.1,-10.1003158915419));
#143483=CARTESIAN_POINT('Origin',(10.5,-21.,-12.650000000037));
#143484=CARTESIAN_POINT('',(10.5,-15.9,-12.250000000037));
#143485=CARTESIAN_POINT('Origin',(10.5,-15.9,-12.650000000037));
#143486=CARTESIAN_POINT('',(10.5,-20.,-12.250000000037));
#143487=CARTESIAN_POINT('',(10.5,-21.,-12.250000000037));
#143488=CARTESIAN_POINT('Origin',(10.5,-20.,-12.650000000037));
#143489=CARTESIAN_POINT('Origin',(18.3,-24.4,-10.9813708499319));
#143490=CARTESIAN_POINT('',(18.8656854249492,-25.4,-10.4156854249827));
#143491=CARTESIAN_POINT('',(19.1,-25.4,-10.9813708499319));
#143492=CARTESIAN_POINT('Origin',(18.3,-25.4,-10.9813708499319));
#143493=CARTESIAN_POINT('',(19.1,-22.1,-10.9813708499319));
#143494=CARTESIAN_POINT('',(19.1,-24.4,-10.9813708499319));
#143495=CARTESIAN_POINT('',(18.8656854249492,-22.1,-10.4156854249827));
#143496=CARTESIAN_POINT('Origin',(18.3,-22.1,-10.9813708499319));
#143497=CARTESIAN_POINT('',(18.8656854249492,-24.4,-10.4156854249827));
#143498=CARTESIAN_POINT('Origin',(19.1,-24.4,-10.6500000000335));
#143499=CARTESIAN_POINT('',(16.734314575042,-22.1,-8.28431457507545));
#143500=CARTESIAN_POINT('',(19.1,-22.1,-10.6500000000335));
#143501=CARTESIAN_POINT('',(16.734314575042,-25.4,-8.28431457507545));
#143502=CARTESIAN_POINT('',(16.734314575042,-24.4,-8.28431457507545));
#143503=CARTESIAN_POINT('',(11.7749999999916,-25.4,-3.3250000000251));
#143504=CARTESIAN_POINT('Origin',(10.6016674012397,-21.,-9.20329141491617));
#143505=CARTESIAN_POINT('',(10.1014821344353,-22.1,-9.53467442424494));
#143506=CARTESIAN_POINT('',(10.1014821344353,-21.,-9.53467442424494));
#143507=CARTESIAN_POINT('Origin',(10.6016674012397,-22.1,-9.20329141491617));
#143508=CARTESIAN_POINT('Origin',(19.1,-24.4,18.2));
#143509=CARTESIAN_POINT('',(19.1,-25.4,-15.1));
#143510=CARTESIAN_POINT('',(19.1,-25.4,8.87499999998871));
#143511=CARTESIAN_POINT('',(19.1,-22.1,-15.1));
#143512=CARTESIAN_POINT('',(19.1,-24.4,-15.1));
#143513=CARTESIAN_POINT('',(19.1,-22.1,8.87499999998871));
#143514=CARTESIAN_POINT('Origin',(15.1,-24.4,-15.1));
#143515=CARTESIAN_POINT('',(15.1,-25.4,-19.1));
#143516=CARTESIAN_POINT('Origin',(15.1,-25.4,-15.1));
#143517=CARTESIAN_POINT('',(15.1,-22.1,-19.1));
#143518=CARTESIAN_POINT('',(15.1,-24.4,-19.1));
#143519=CARTESIAN_POINT('Origin',(15.1,-22.1,-15.1));
#143520=CARTESIAN_POINT('Origin',(11.2581254575403,-22.1,-18.3));
#143521=CARTESIAN_POINT('',(11.2581254575403,-10.3,-19.1000000000102));
#143522=CARTESIAN_POINT('',(11.8728253843338,-10.3,-17.788));
#143523=CARTESIAN_POINT('Origin',(11.2581254575403,-10.3,-18.3));
#143524=CARTESIAN_POINT('',(11.8728253843338,-22.1,-17.788));
#143525=CARTESIAN_POINT('',(11.8728253843338,-22.1,-17.788));
#143526=CARTESIAN_POINT('',(11.2581254575403,-22.1,-19.1));
#143527=CARTESIAN_POINT('Origin',(11.2581254575403,-22.1,-18.3));
#143528=CARTESIAN_POINT('',(11.2581254575403,-22.1,-19.1));
#143529=CARTESIAN_POINT('Origin',(15.1,-22.1,-15.1));
#143530=CARTESIAN_POINT('Origin',(15.1,-10.3,-15.1));
#143531=CARTESIAN_POINT('Origin',(15.1,-22.1,-15.1));
#143532=CARTESIAN_POINT('Origin',(15.1,-24.4,-15.1));
#143533=CARTESIAN_POINT('',(13.55,-22.1,-15.1));
#143534=CARTESIAN_POINT('Origin',(15.1,-22.1,-15.1));
#143535=CARTESIAN_POINT('',(13.55,-25.4,-15.1));
#143536=CARTESIAN_POINT('',(13.55,-24.4,-15.1));
#143537=CARTESIAN_POINT('Origin',(15.1,-25.4,-15.1));
#143538=CARTESIAN_POINT('Origin',(10.5,-18.9,-13.800000000037));
#143539=CARTESIAN_POINT('',(10.5,-10.3,-13.400000000037));
#143540=CARTESIAN_POINT('Origin',(10.5,-10.3,-13.800000000037));
#143541=CARTESIAN_POINT('',(10.5,-15.9,-13.400000000037));
#143542=CARTESIAN_POINT('',(10.5,-18.9,-13.400000000037));
#143543=CARTESIAN_POINT('Origin',(10.5,-15.9,-13.800000000037));
#143544=CARTESIAN_POINT('Origin',(0.0099462365591374,-15.7,-9.20072405893627));
#143545=CARTESIAN_POINT('',(0.634274193548385,-15.9,-8.78513459549712));
#143546=CARTESIAN_POINT('',(0.634274193548384,-10.3,-8.78513459549712));
#143547=CARTESIAN_POINT('',(0.634274193548385,-15.7,-8.78513459549712));
#143548=CARTESIAN_POINT('',(-0.616835877496162,-10.3,-8.7888452157064));
#143549=CARTESIAN_POINT('Origin',(0.0099462365591374,-10.3,-9.20072405893626));
#143550=CARTESIAN_POINT('',(-0.616835877496162,-15.9,-8.7888452157064));
#143551=CARTESIAN_POINT('',(-0.616835877496162,-15.7,-8.7888452157064));
#143552=CARTESIAN_POINT('Origin',(0.0099462365591374,-15.9,-9.20072405893627));
#143553=CARTESIAN_POINT('Origin',(5.65685424949238,-12.5431457505076,-17.500000000019));
#143554=CARTESIAN_POINT('',(3.15685424949238,-12.5431457505076,-12.8620372432944));
#143555=CARTESIAN_POINT('',(8.15685424949238,-12.5431457505076,-14.5481534330082));
#143556=CARTESIAN_POINT('Ctrl Pts',(3.15685424949238,-12.5431457505076,
-12.8620372432944));
#143557=CARTESIAN_POINT('Ctrl Pts',(3.15685424949238,-12.8592320850127,
-12.8620372432944));
#143558=CARTESIAN_POINT('Ctrl Pts',(3.22047042900536,-13.1914168687361,
-12.9023109536184));
#143559=CARTESIAN_POINT('Ctrl Pts',(3.46810331101024,-13.7943820582662,
-13.0496463732524));
#143560=CARTESIAN_POINT('Ctrl Pts',(3.65182681306313,-14.0656238936063,
-13.1553086621643));
#143561=CARTESIAN_POINT('Ctrl Pts',(4.08156538511786,-14.5109362958629,
-13.3821704208394));
#143562=CARTESIAN_POINT('Ctrl Pts',(4.36420178144363,-14.7097688956392,
-13.5212507616241));
#143563=CARTESIAN_POINT('Ctrl Pts',(4.98866328596235,-14.9759892088894,
-13.7905365871133));
#143564=CARTESIAN_POINT('Ctrl Pts',(5.33083836910257,-15.0431457505076,
-13.9201585567324));
#143565=CARTESIAN_POINT('Ctrl Pts',(5.96402984326142,-15.0431457505076,
-14.1274260237179));
#143566=CARTESIAN_POINT('Ctrl Pts',(6.29726352242101,-14.9828471682561,
-14.2207295472445));
#143567=CARTESIAN_POINT('Ctrl Pts',(6.91708557876398,-14.7281135426884,
-14.3664199959765));
#143568=CARTESIAN_POINT('Ctrl Pts',(7.20340848989777,-14.5334551117466,
-14.4195445895854));
#143569=CARTESIAN_POINT('Ctrl Pts',(7.64935577171109,-14.0848586172969,
-14.4907101386031));
#143570=CARTESIAN_POINT('Ctrl Pts',(7.84056457463014,-13.8048197236649,
-14.5143922650254));
#143571=CARTESIAN_POINT('Ctrl Pts',(8.09431374793703,-13.1906049475643,
-14.5427449864562));
#143572=CARTESIAN_POINT('Ctrl Pts',(8.15685424949238,-12.8564634012673,
-14.5481534330082));
#143573=CARTESIAN_POINT('Ctrl Pts',(8.15685424949238,-12.5431457505076,
-14.5481534330082));
#143574=CARTESIAN_POINT('',(3.15685424949238,-12.5431457505076,-11.4163656902917));
#143575=CARTESIAN_POINT('',(3.15685424949238,-12.5431457505076,-17.5000000000137));
#143576=CARTESIAN_POINT('',(8.15685424949238,-12.5431457505076,-13.3421101999983));
#143577=CARTESIAN_POINT('Ctrl Pts',(8.15685424949238,-12.5431457505076,
-13.3421101999983));
#143578=CARTESIAN_POINT('Ctrl Pts',(8.15685424949238,-12.8578774912135,
-13.3421101999983));
#143579=CARTESIAN_POINT('Ctrl Pts',(8.09374219603427,-13.1934037608601,
-13.3360182818923));
#143580=CARTESIAN_POINT('Ctrl Pts',(7.83801789221978,-13.8095513827507,
-13.3040436400873));
#143581=CARTESIAN_POINT('Ctrl Pts',(7.64540523586579,-14.0901286700669,
-13.2773205739759));
#143582=CARTESIAN_POINT('Ctrl Pts',(7.19727521652421,-14.5382586894085,
-13.1970274688756));
#143583=CARTESIAN_POINT('Ctrl Pts',(6.91043414045708,-14.7317662324076,
-13.1371819992974));
#143584=CARTESIAN_POINT('Ctrl Pts',(6.29202188533623,-14.9840644227757,
-12.9734658623863));
#143585=CARTESIAN_POINT('Ctrl Pts',(5.96078348705636,-15.0431457505076,
-12.8687874210152));
#143586=CARTESIAN_POINT('Ctrl Pts',(5.32706036423454,-15.0431457505076,
-12.6341908129028));
#143587=CARTESIAN_POINT('Ctrl Pts',(4.98261630817213,-14.9745611086902,
-12.4857870053569));
#143588=CARTESIAN_POINT('Ctrl Pts',(4.35583159298622,-14.7050239351627,
-12.1764316966991));
#143589=CARTESIAN_POINT('Ctrl Pts',(4.07305532958835,-14.50439870059,-12.0160781324946));
#143590=CARTESIAN_POINT('Ctrl Pts',(3.64746690731458,-14.0589639276313,
-11.755750359458));
#143591=CARTESIAN_POINT('Ctrl Pts',(3.46630265431125,-13.7906444571559,
-11.6345025681409));
#143592=CARTESIAN_POINT('Ctrl Pts',(3.22082631848395,-13.1916327737242,
-11.4639114195569));
#143593=CARTESIAN_POINT('Ctrl Pts',(3.15685424949238,-12.8602908531128,
-11.4163656902917));
#143594=CARTESIAN_POINT('Ctrl Pts',(3.15685424949238,-12.5431457505076,
-11.4163656902917));
#143595=CARTESIAN_POINT('',(8.15685424949238,-12.5431457505076,-17.5000000000052));
#143596=CARTESIAN_POINT('Origin',(-5.65685424949238,-12.5431457505076,-17.500000000019));
#143597=CARTESIAN_POINT('',(-8.15685424949239,-12.5431457505076,-13.4316618717243));
#143598=CARTESIAN_POINT('',(-8.15685424949238,-12.5431457505076,-17.5000000000328));
#143599=CARTESIAN_POINT('',(-3.15685424949238,-12.5431457505076,-11.4670924738648));
#143600=CARTESIAN_POINT('Ctrl Pts',(-3.15685424949238,-12.5431457505076,
-11.4670924738648));
#143601=CARTESIAN_POINT('Ctrl Pts',(-3.15685424949238,-12.8710195758623,
-11.4670924738648));
#143602=CARTESIAN_POINT('Ctrl Pts',(-3.22511540251142,-13.2121346615079,
-11.5183801889379));
#143603=CARTESIAN_POINT('Ctrl Pts',(-3.48502968752171,-13.8253626051227,
-11.7004217329402));
#143604=CARTESIAN_POINT('Ctrl Pts',(-3.6763649683173,-14.0981903752653,
-11.8292149981844));
#143605=CARTESIAN_POINT('Ctrl Pts',(-4.11108111624766,-14.5329065231956,
-12.0956632706648));
#143606=CARTESIAN_POINT('Ctrl Pts',(-4.38898639276768,-14.7231999641409,
-12.253689661289));
#143607=CARTESIAN_POINT('Ctrl Pts',(-5.00163457398632,-14.9784717317639,
-12.5584845046953));
#143608=CARTESIAN_POINT('Ctrl Pts',(-5.33677055768477,-15.0431457505076,
-12.7047172810065));
#143609=CARTESIAN_POINT('Ctrl Pts',(-5.9621407575736,-15.0431457505076,
-12.9409762725843));
#143610=CARTESIAN_POINT('Ctrl Pts',(-6.29493995959754,-14.9835365833956,
-13.0486345344632));
#143611=CARTESIAN_POINT('Ctrl Pts',(-6.9160341250112,-14.7288097484239,
-13.2176887423056));
#143612=CARTESIAN_POINT('Ctrl Pts',(-7.20398399968078,-14.5333922588975,
-13.2798994668974));
#143613=CARTESIAN_POINT('Ctrl Pts',(-7.65043593866441,-14.0832724915651,
-13.3632649111085));
#143614=CARTESIAN_POINT('Ctrl Pts',(-7.84118079530232,-13.8036434650245,
-13.3912900060078));
#143615=CARTESIAN_POINT('Ctrl Pts',(-8.09439086444467,-13.1901020782128,
-13.4250787866805));
#143616=CARTESIAN_POINT('Ctrl Pts',(-8.15685424949238,-12.85623436387,-13.4316618717243));
#143617=CARTESIAN_POINT('Ctrl Pts',(-8.15685424949238,-12.5431457505076,
-13.4316618717243));
#143618=CARTESIAN_POINT('',(-3.15685424949238,-12.5431457505076,-17.5000000000243));
#143619=CARTESIAN_POINT('Origin',(-5.65685424949238,-12.5431457505076,-19.1));
#143620=CARTESIAN_POINT('',(-6.95685424949238,-12.5431457505076,-19.1));
#143621=CARTESIAN_POINT('Origin',(-5.65685424949238,-12.5431457505076,-19.1));
#143622=CARTESIAN_POINT('',(-6.95685424949238,-12.5431457505076,-16.700000000013));
#143623=CARTESIAN_POINT('',(-6.95685424949238,-12.5431457505076,-19.1));
#143624=CARTESIAN_POINT('Origin',(-5.65685424949238,-12.5431457505076,-16.700000000013));
#143625=CARTESIAN_POINT('Origin',(-1.28238570254272E-15,-12.6715728752538,
-15.900000000019));
#143626=CARTESIAN_POINT('',(-4.55308926455237,-10.3,-15.9000000000267));
#143627=CARTESIAN_POINT('',(-6.76061923443239,-10.3,-15.9000000000304));
#143628=CARTESIAN_POINT('',(-2.27654463227754,-10.3,-15.9000000000228));
#143629=CARTESIAN_POINT('Origin',(-5.65685424949238,-12.5431457505076,-15.900000000019));
#143630=CARTESIAN_POINT('',(-7.75685424949508,-12.5431457505076,-15.9000000000321));
#143631=CARTESIAN_POINT('Origin',(-5.65685424949373,-12.5431457505076,-15.9000000000285));
#143632=CARTESIAN_POINT('Origin',(-5.65685424949306,-12.5431457505076,-16.3000000000208));
#143633=CARTESIAN_POINT('',(-7.35685424949373,-12.5431457505076,-16.3000000000225));
#143634=CARTESIAN_POINT('Origin',(5.65685424949238,-12.5431457505076,-19.1));
#143635=CARTESIAN_POINT('',(4.35685424949238,-12.5431457505076,-19.1));
#143636=CARTESIAN_POINT('Origin',(5.65685424949238,-12.5431457505076,-19.1));
#143637=CARTESIAN_POINT('',(4.35685424949238,-12.5431457505076,-16.7000000000321));
#143638=CARTESIAN_POINT('',(4.35685424949238,-12.5431457505076,-19.1));
#143639=CARTESIAN_POINT('Origin',(5.65685424949238,-12.5431457505076,-16.7000000000321));
#143640=CARTESIAN_POINT('Origin',(-1.28238570254272E-15,-12.6715728752538,
-15.900000000019));
#143641=CARTESIAN_POINT('',(6.76061923443239,-10.3,-15.9000000000076));
#143642=CARTESIAN_POINT('',(4.55308926455238,-10.3,-15.9000000000113));
#143643=CARTESIAN_POINT('',(3.38030961721484,-10.3,-15.9000000000133));
#143644=CARTESIAN_POINT('Origin',(5.65685424949238,-12.5431457505076,-15.900000000019));
#143645=CARTESIAN_POINT('',(3.55685424948968,-12.5431457505076,-15.900000000013));
#143646=CARTESIAN_POINT('Origin',(5.65685424949103,-12.5431457505076,-15.9000000000094));
#143647=CARTESIAN_POINT('Origin',(5.65685424949171,-12.5431457505076,-16.3000000000208));
#143648=CARTESIAN_POINT('',(3.95685424949103,-12.5431457505076,-16.3000000000225));
#143649=CARTESIAN_POINT('Origin',(-5.65685424949103,-12.5431457505076,-16.7000000000401));
#143650=CARTESIAN_POINT('Ctrl Pts',(-2.22490186897899,-10.3,-17.5000000000366));
#143651=CARTESIAN_POINT('Ctrl Pts',(-3.67120009961655,-10.3,-16.2893593523635));
#143652=CARTESIAN_POINT('Ctrl Pts',(-4.55308926462462,-10.3,-15.9000000000179));
#143653=CARTESIAN_POINT('Ctrl Pts',(-6.76061923434026,-10.3,-15.9000000000128));
#143654=CARTESIAN_POINT('Ctrl Pts',(-7.64250839935299,-10.3,-16.2893593523584));
#143655=CARTESIAN_POINT('Ctrl Pts',(-9.08880663000172,-10.3,-17.5000000000493));
#143656=CARTESIAN_POINT('Origin',(-1.72162677917566E-16,-23.3784271247462,
-15.900000000019));
#143657=CARTESIAN_POINT('',(-7.08117906942998,-25.4,-15.9));
#143658=CARTESIAN_POINT('',(-4.23252942955478,-25.4,-15.9));
#143659=CARTESIAN_POINT('Origin',(-5.65685424949238,-23.8568542494924,-15.900000000019));
#143660=CARTESIAN_POINT('',(-3.15685424949238,-25.3999994322658,-15.9000000000148));
#143661=CARTESIAN_POINT('',(1.74566039757947E-12,-25.4,-15.9000000000095));
#143662=CARTESIAN_POINT('',(-3.15685424949238,-23.8568542494924,-15.9000000000148));
#143663=CARTESIAN_POINT('',(-3.15685424949238,-24.389213278506,-15.9000000000148));
#143664=CARTESIAN_POINT('',(-8.15685424949238,-23.8568542494924,-15.9000000000232));
#143665=CARTESIAN_POINT('Origin',(-5.65685424949238,-23.8568542494924,-15.900000000019));
#143666=CARTESIAN_POINT('',(-8.15685424949238,-25.3999994322658,-15.9000000000232));
#143667=CARTESIAN_POINT('',(-8.15685424949238,-23.6176406871193,-15.9000000000232));
#143668=CARTESIAN_POINT('',(1.74566039757947E-12,-25.4,-15.9000000000095));
#143669=CARTESIAN_POINT('Origin',(-1.72162677917566E-16,-23.3784271247462,
-15.900000000019));
#143670=CARTESIAN_POINT('',(4.23252942955478,-25.4,-15.9));
#143671=CARTESIAN_POINT('',(7.08117906942998,-25.4,-15.9));
#143672=CARTESIAN_POINT('Origin',(5.65685424949238,-23.8568542494924,-15.900000000019));
#143673=CARTESIAN_POINT('',(8.15685424949238,-25.4,-15.8999999999957));
#143674=CARTESIAN_POINT('',(1.74566039757947E-12,-25.4,-15.9000000000095));
#143675=CARTESIAN_POINT('',(8.15685424949238,-23.8568542494924,-15.8999999999957));
#143676=CARTESIAN_POINT('',(8.15685424949238,-24.3892135623731,-15.8999999999957));
#143677=CARTESIAN_POINT('',(3.15685424949238,-23.8568542494924,-15.9000000000041));
#143678=CARTESIAN_POINT('Origin',(5.65685424949238,-23.8568542494924,-15.900000000019));
#143679=CARTESIAN_POINT('',(3.15685424949238,-25.4,-15.9000000000041));
#143680=CARTESIAN_POINT('',(3.15685424949238,-23.6176406871193,-15.9000000000041));
#143681=CARTESIAN_POINT('',(1.74566039757947E-12,-25.4,-15.9000000000095));
#143682=CARTESIAN_POINT('Origin',(-3.15685424949238,-25.3999994322658,-15.9000000000148));
#143683=CARTESIAN_POINT('',(-3.15685424949238,-25.3999994322658,-12.9000000000148));
#143684=CARTESIAN_POINT('',(-3.15685424949238,-25.4,-8.17500000001868));
#143685=CARTESIAN_POINT('',(-3.15685424949238,-23.8568542494924,-12.9000000000148));
#143686=CARTESIAN_POINT('',(-3.15685424949238,-24.389213278506,-12.9000000000148));
#143687=CARTESIAN_POINT('',(-3.15685424949238,-23.8568542494924,-15.9000000000148));
#143688=CARTESIAN_POINT('Origin',(-5.65685424949238,-23.8568542494924,-15.9000000000095));
#143689=CARTESIAN_POINT('',(-3.42078627199525,-22.7388202607371,-12.9000000000057));
#143690=CARTESIAN_POINT('Origin',(-5.65685424949238,-23.8568542494924,-12.9000000000095));
#143691=CARTESIAN_POINT('',(-8.15685424949238,-23.8568542494924,-12.9000000000232));
#143692=CARTESIAN_POINT('Origin',(-5.65685424949238,-23.8568542494924,-12.9000000000095));
#143693=CARTESIAN_POINT('',(-8.15685424949238,-23.8568542494924,-15.9000000000232));
#143694=CARTESIAN_POINT('Origin',(-8.15685424949238,-23.8568542494924,-15.9000000000232));
#143695=CARTESIAN_POINT('',(-8.15685424949238,-25.3999994322658,-12.9000000000232));
#143696=CARTESIAN_POINT('',(-8.15685424949238,-23.6176406871193,-12.9000000000232));
#143697=CARTESIAN_POINT('',(-8.15685424949238,-25.4,-8.1750000000229));
#143698=CARTESIAN_POINT('Origin',(8.15685424949238,-25.4,-15.8999999999957));
#143699=CARTESIAN_POINT('',(8.15685424949238,-25.4,-12.8999999999957));
#143700=CARTESIAN_POINT('',(8.15685424949238,-25.4,-8.17500000000913));
#143701=CARTESIAN_POINT('',(8.15685424949238,-23.8568542494924,-12.8999999999957));
#143702=CARTESIAN_POINT('',(8.15685424949238,-24.3892135623731,-12.8999999999957));
#143703=CARTESIAN_POINT('',(8.15685424949238,-23.8568542494924,-15.8999999999957));
#143704=CARTESIAN_POINT('Origin',(5.65685424949238,-23.8568542494924,-15.9000000000095));
#143705=CARTESIAN_POINT('',(7.89292222699332,-22.7388202607448,-12.9000000000057));
#143706=CARTESIAN_POINT('Origin',(5.65685424949238,-23.8568542494924,-12.9000000000095));
#143707=CARTESIAN_POINT('',(3.15685424949238,-23.8568542494924,-12.9000000000041));
#143708=CARTESIAN_POINT('Origin',(5.65685424949238,-23.8568542494924,-12.9000000000095));
#143709=CARTESIAN_POINT('',(3.15685424949238,-23.8568542494924,-15.9000000000041));
#143710=CARTESIAN_POINT('Origin',(3.15685424949238,-23.8568542494924,-15.9000000000041));
#143711=CARTESIAN_POINT('',(3.15685424949238,-25.4,-12.9000000000041));
#143712=CARTESIAN_POINT('',(3.15685424949238,-23.6176406871193,-12.9000000000041));
#143713=CARTESIAN_POINT('',(3.15685424949238,-25.4,-8.17500000001335));
#143714=CARTESIAN_POINT('Origin',(5.65685424949238,-23.8568542494924,-12.8999999999999));
#143715=CARTESIAN_POINT('Origin',(5.65685424949238,-23.8568542494924,-12.8999999999999));
#143716=CARTESIAN_POINT('',(7.10022992246644,-22.4134785765183,-11.4566243270258));
#143717=CARTESIAN_POINT('Origin',(5.65685424949238,-23.8568542494924,-12.8999999999999));
#143718=CARTESIAN_POINT('Origin',(5.65685424949238,-24.6284271247462,-12.8999999999999));
#143719=CARTESIAN_POINT('Origin',(5.65685424949238,-25.4,-12.8999999999999));
#143720=CARTESIAN_POINT('Origin',(-5.65685424949238,-23.8568542494924,-12.900000000019));
#143721=CARTESIAN_POINT('Origin',(-5.65685424949238,-23.8568542494924,-12.900000000019));
#143722=CARTESIAN_POINT('',(-4.21347857651832,-22.4134785765183,-11.4566243270449));
#143723=CARTESIAN_POINT('Origin',(-5.65685424949238,-23.8568542494924,-12.900000000019));
#143724=CARTESIAN_POINT('Origin',(-5.65685424949238,-24.6284268408791,-12.900000000019));
#143725=CARTESIAN_POINT('Origin',(-5.65685424949238,-25.4,-12.900000000019));
#143726=CARTESIAN_POINT('Origin',(4.35685424949238,-23.8568542494924,-19.1));
#143727=CARTESIAN_POINT('',(4.35685424949238,-23.8568542494924,-16.7));
#143728=CARTESIAN_POINT('',(4.35685424949238,-25.4,-15.9822540280527));
#143729=CARTESIAN_POINT('Ctrl Pts',(4.35685424949238,-23.8568542494924,
-16.7));
#143730=CARTESIAN_POINT('Ctrl Pts',(4.35685424949238,-24.461508581868,-16.7));
#143731=CARTESIAN_POINT('Ctrl Pts',(4.35685424949238,-25.4,-15.9822540280527));
#143732=CARTESIAN_POINT('',(4.35685424949238,-25.4,-19.1));
#143733=CARTESIAN_POINT('',(4.35685424949238,-25.4,-9.77500000001129));
#143734=CARTESIAN_POINT('',(4.35685424949238,-23.8568542494924,-19.1));
#143735=CARTESIAN_POINT('',(4.35685424949238,-24.1284271247462,-19.1));
#143736=CARTESIAN_POINT('',(4.35685424949238,-23.8568542494924,-19.1));
#143737=CARTESIAN_POINT('Origin',(5.65685424949238,-23.8568542494924,-19.1));
#143738=CARTESIAN_POINT('',(6.95685424949238,-23.8568542494924,-16.7));
#143739=CARTESIAN_POINT('Origin',(5.65685424949238,-23.8568542494924,-16.7));
#143740=CARTESIAN_POINT('',(6.95685424949238,-23.8568542494924,-19.1));
#143741=CARTESIAN_POINT('Origin',(5.65685424949238,-23.8568542494924,-19.1));
#143742=CARTESIAN_POINT('',(6.95685424949238,-23.8568542494924,-19.1));
#143743=CARTESIAN_POINT('Origin',(6.95685424949238,-25.4,-19.1));
#143744=CARTESIAN_POINT('',(6.95685424949238,-25.4,-15.9822540280527));
#143745=CARTESIAN_POINT('Ctrl Pts',(6.95685424949238,-25.4,-15.9822540280527));
#143746=CARTESIAN_POINT('Ctrl Pts',(6.95685424949238,-24.4615085818681,
-16.7));
#143747=CARTESIAN_POINT('Ctrl Pts',(6.95685424949238,-23.8568542494924,
-16.7));
#143748=CARTESIAN_POINT('',(6.95685424949238,-25.4,-19.1));
#143749=CARTESIAN_POINT('',(6.95685424949238,-24.9,-19.1));
#143750=CARTESIAN_POINT('',(6.95685424949238,-25.4,-9.77500000001129));
#143751=CARTESIAN_POINT('Origin',(5.65685424949238,-23.8568542494924,-16.3));
#143752=CARTESIAN_POINT('Ctrl Pts',(7.08117906942999,-25.4,-15.9));
#143753=CARTESIAN_POINT('Ctrl Pts',(7.01777493434072,-25.4,-15.9430038491878));
#143754=CARTESIAN_POINT('Ctrl Pts',(6.95685424949238,-25.4,-15.9822540280527));
#143755=CARTESIAN_POINT('Ctrl Pts',(4.35685424949238,-25.4,-15.9822540280527));
#143756=CARTESIAN_POINT('Ctrl Pts',(4.29593356464403,-25.4,-15.9430038491878));
#143757=CARTESIAN_POINT('Ctrl Pts',(4.23252942955477,-25.4,-15.9));
#143758=CARTESIAN_POINT('Origin',(-6.95685424949238,-23.8568542494924,-19.1));
#143759=CARTESIAN_POINT('',(-6.95685424949238,-23.8568542494924,-16.7));
#143760=CARTESIAN_POINT('',(-6.95685424949238,-25.4,-15.9822540280527));
#143761=CARTESIAN_POINT('Ctrl Pts',(-6.95685424949238,-23.8568542494924,
-16.7));
#143762=CARTESIAN_POINT('Ctrl Pts',(-6.95685424949238,-24.4615085818681,
-16.7));
#143763=CARTESIAN_POINT('Ctrl Pts',(-6.95685424949238,-25.4,-15.9822540280527));
#143764=CARTESIAN_POINT('',(-6.95685424949238,-25.3999994322658,-19.1));
#143765=CARTESIAN_POINT('',(-6.95685424949238,-25.4,-9.77500000001129));
#143766=CARTESIAN_POINT('',(-6.95685424949238,-23.8568542494924,-19.1));
#143767=CARTESIAN_POINT('',(-6.95685424949238,-24.1284271247462,-19.1));
#143768=CARTESIAN_POINT('',(-6.95685424949238,-23.8568542494924,-19.1));
#143769=CARTESIAN_POINT('Origin',(-5.65685424949238,-23.8568542494924,-19.1));
#143770=CARTESIAN_POINT('',(-4.35685424949238,-23.8568542494924,-16.7));
#143771=CARTESIAN_POINT('Origin',(-5.65685424949238,-23.8568542494924,-16.7));
#143772=CARTESIAN_POINT('',(-4.35685424949238,-23.8568542494924,-19.1));
#143773=CARTESIAN_POINT('Origin',(-5.65685424949238,-23.8568542494924,-19.1));
#143774=CARTESIAN_POINT('',(-4.35685424949238,-23.8568542494924,-19.1));
#143775=CARTESIAN_POINT('Origin',(-4.35685424949238,-25.3999994322658,-19.1));
#143776=CARTESIAN_POINT('',(-4.35685424949238,-25.4,-15.9822540280527));
#143777=CARTESIAN_POINT('Ctrl Pts',(-4.35685424949238,-25.4,-15.9822540280527));
#143778=CARTESIAN_POINT('Ctrl Pts',(-4.35685424949238,-24.4615085818681,
-16.7));
#143779=CARTESIAN_POINT('Ctrl Pts',(-4.35685424949238,-23.8568542494924,
-16.7));
#143780=CARTESIAN_POINT('',(-4.35685424949238,-25.3999994322658,-19.1));
#143781=CARTESIAN_POINT('',(-4.35685424949238,-24.8999997161328,-19.1));
#143782=CARTESIAN_POINT('',(-4.35685424949239,-25.4,-9.77500000001129));
#143783=CARTESIAN_POINT('Origin',(-5.65685424949238,-23.8568542494924,-16.3));
#143784=CARTESIAN_POINT('Ctrl Pts',(-4.23252942955477,-25.4,-15.9));
#143785=CARTESIAN_POINT('Ctrl Pts',(-4.29593356464405,-25.4,-15.9430038491878));
#143786=CARTESIAN_POINT('Ctrl Pts',(-4.35685424949239,-25.4,-15.9822540280527));
#143787=CARTESIAN_POINT('Ctrl Pts',(-6.95685424949238,-25.4,-15.9822540280527));
#143788=CARTESIAN_POINT('Ctrl Pts',(-7.01777493434072,-25.4,-15.9430038491878));
#143789=CARTESIAN_POINT('Ctrl Pts',(-7.08117906942999,-25.4,-15.9));
#143790=CARTESIAN_POINT('Origin',(10.9,-15.7,-13.400000000037));
#143791=CARTESIAN_POINT('',(9.25,-10.3,-13.400000000037));
#143792=CARTESIAN_POINT('',(4.12984378812245,-10.3,-13.400000000037));
#143793=CARTESIAN_POINT('',(9.25,-15.9,-13.400000000037));
#143794=CARTESIAN_POINT('',(9.25,-21.1,-13.400000000037));
#143795=CARTESIAN_POINT('',(3.8928257784653,-15.9,-13.400000000037));
#143796=CARTESIAN_POINT('Origin',(10.9,-19.9,-12.250000000037));
#143797=CARTESIAN_POINT('',(3.8928257784653,-15.9,-12.250000000037));
#143798=CARTESIAN_POINT('',(4.12984378812245,-20.,-12.250000000037));
#143799=CARTESIAN_POINT('Origin',(-1.26287869055635E-16,-18.2,-19.1));
#143800=CARTESIAN_POINT('',(-0.790053763424162,-14.6877621021777,-16.9000000000203));
#143801=CARTESIAN_POINT('Ctrl Pts',(-0.790053763427873,-14.6877621021785,
-16.9000000000213));
#143802=CARTESIAN_POINT('Ctrl Pts',(-0.790053763427873,-14.6877621021785,
-16.9749752755816));
#143803=CARTESIAN_POINT('Ctrl Pts',(-0.804989255950869,-14.6910185364364,
-17.0548386220574));
#143804=CARTESIAN_POINT('Ctrl Pts',(-0.865223395403298,-14.7053831241914,
-17.2013777360166));
#143805=CARTESIAN_POINT('Ctrl Pts',(-0.910511782222757,-14.7166346855472,
-17.2680436277885));
#143806=CARTESIAN_POINT('Ctrl Pts',(-1.01708168610465,-14.7461903939279,
-17.3764937169279));
#143807=CARTESIAN_POINT('Ctrl Pts',(-1.08648661407425,-14.7669551355699,
-17.4238310868093));
#143808=CARTESIAN_POINT('Ctrl Pts',(-1.23615012040654,-14.8179616954849,
-17.485547331143));
#143809=CARTESIAN_POINT('Ctrl Pts',(-1.31633318766185,-14.8483356495151,
-17.5000000000213));
#143810=CARTESIAN_POINT('Ctrl Pts',(-1.39005376342787,-14.8791942943346,
-17.5000000000213));
#143811=CARTESIAN_POINT('',(-3.59005376342416,-18.4674209709877,-19.1));
#143812=CARTESIAN_POINT('',(-0.790053763435527,-14.6877621021802,-12.3613777665646));
#143813=CARTESIAN_POINT('Ctrl Pts',(-0.79005376343553,-14.6877621021802,
-12.3613777665646));
#143814=CARTESIAN_POINT('Ctrl Pts',(-0.790053763435658,-14.6877621021803,
-12.2855065251448));
#143815=CARTESIAN_POINT('Ctrl Pts',(-0.805345661260487,-14.6910942468679,
-12.2047540470466));
#143816=CARTESIAN_POINT('Ctrl Pts',(-0.866899513458881,-14.7057924400671,
-12.0568713431911));
#143817=CARTESIAN_POINT('Ctrl Pts',(-0.913151482487876,-14.7173085072149,
-11.9897519100894));
#143818=CARTESIAN_POINT('Ctrl Pts',(-1.02061424285241,-14.7472351076383,
-11.8822891497248));
#143819=CARTESIAN_POINT('Ctrl Pts',(-1.08953284953172,-14.767936670379,
-11.8359268093953));
#143820=CARTESIAN_POINT('Ctrl Pts',(-1.2378422455355,-14.8185968721662,
-11.7755081825809));
#143821=CARTESIAN_POINT('Ctrl Pts',(-1.31715971249138,-14.8486816239716,
-11.7613777665656));
#143822=CARTESIAN_POINT('Ctrl Pts',(-1.46598670564076,-14.910979012095,
-11.7613777665656));
#143823=CARTESIAN_POINT('Ctrl Pts',(-1.54605981512051,-14.9478478813323,
-11.7765606781301));
#143824=CARTESIAN_POINT('Ctrl Pts',(-1.67832189315571,-15.0144783588798,
-11.8313482828004));
#143825=CARTESIAN_POINT('Ctrl Pts',(-1.73301170809371,-15.0441191690517,
-11.865202730501));
#143826=CARTESIAN_POINT('Ctrl Pts',(-1.77992868114481,-15.0708061916784,
-11.9053102841234));
#143827=CARTESIAN_POINT('',(-0.790053763424162,-14.6877621021777,-19.1));
#143828=CARTESIAN_POINT('Origin',(-3.59005376342686,-10.3,-17.5000000000251));
#143829=CARTESIAN_POINT('Origin',(-0.790053763426861,-10.3,-17.5000000000203));
#143830=CARTESIAN_POINT('',(-0.790053763427873,-10.3,-16.9000000000203));
#143831=CARTESIAN_POINT('',(-0.790053763427873,-10.3,-16.9000000000203));
#143832=CARTESIAN_POINT('',(-0.790053763435531,-10.3,-12.3613777665646));
#143833=CARTESIAN_POINT('',(-0.79005376343553,-10.3,-12.3613777665646));
#143834=CARTESIAN_POINT('',(-0.790053763449776,-10.3,-3.91787087923316));
#143835=CARTESIAN_POINT('Origin',(1.40994623656442,-10.3,-12.3320287107467));
#143836=CARTESIAN_POINT('',(0.809946236564421,-10.3,-12.3320287107477));
#143837=CARTESIAN_POINT('',(1.79710938537606,-10.3,-11.8736569225635));
#143838=CARTESIAN_POINT('Origin',(1.40994623656442,-10.3,-12.3320287107467));
#143839=CARTESIAN_POINT('',(1.79710938537606,-15.0806414350073,-11.8736569225635));
#143840=CARTESIAN_POINT('',(1.79710938537606,-10.3,-11.8736569225635));
#143841=CARTESIAN_POINT('',(0.809946236564415,-14.6922960367392,-12.3320287107477));
#143842=CARTESIAN_POINT('Ctrl Pts',(1.79710938537606,-15.0806414350073,
-11.8736569225635));
#143843=CARTESIAN_POINT('Ctrl Pts',(1.75079494773061,-15.0539589908968,
-11.8345374916201));
#143844=CARTESIAN_POINT('Ctrl Pts',(1.69707204519075,-15.0244494752567,
-11.8015240531292));
#143845=CARTESIAN_POINT('Ctrl Pts',(1.5659413296006,-14.9573677420981,-11.7472096227115));
#143846=CARTESIAN_POINT('Ctrl Pts',(1.48587960880272,-14.9199127536573,
-11.7320287107467));
#143847=CARTESIAN_POINT('Ctrl Pts',(1.33711320367574,-14.8565894593461,
-11.7320287107467));
#143848=CARTESIAN_POINT('Ctrl Pts',(1.25782749360031,-14.825976274775,-11.7461351698937));
#143849=CARTESIAN_POINT('Ctrl Pts',(1.10951031289533,-14.7743390479818,
-11.8065293086185));
#143850=CARTESIAN_POINT('Ctrl Pts',(1.04055362922102,-14.7531894409119,
-11.8528931806663));
#143851=CARTESIAN_POINT('Ctrl Pts',(0.933070797095156,-14.7225913145941,
-11.9603760127921));
#143852=CARTESIAN_POINT('Ctrl Pts',(0.8868166131236,-14.710793680294,-12.0274791631079));
#143853=CARTESIAN_POINT('Ctrl Pts',(0.825248988139974,-14.695721396081,
-12.1753628835624));
#143854=CARTESIAN_POINT('Ctrl Pts',(0.809946236564421,-14.6922960367393,
-12.2561325049032));
#143855=CARTESIAN_POINT('Ctrl Pts',(0.809946236564421,-14.6922960367393,
-12.3320287107467));
#143856=CARTESIAN_POINT('',(0.80994623656442,-10.3,-12.3320287107477));
#143857=CARTESIAN_POINT('Origin',(1.70994623656809,-18.2,-14.5048933931961));
#143858=CARTESIAN_POINT('',(3.6,-18.2,-17.5000000000129));
#143859=CARTESIAN_POINT('',(3.60994623657314,-18.2,-17.5000000000129));
#143860=CARTESIAN_POINT('',(-5.64602728205014,-18.2,-17.5000000000285));
#143861=CARTESIAN_POINT('',(3.60000000001663,-18.2,-13.1237282076557));
#143862=CARTESIAN_POINT('',(3.6,-18.2,-19.1));
#143863=CARTESIAN_POINT('',(3.60994623658205,-18.2,-13.1293002508741));
#143864=CARTESIAN_POINT('Origin',(9.25,-18.2,-3.05000000003699));
#143865=CARTESIAN_POINT('',(3.6099462365668,-18.2,-13.7451470201718));
#143866=CARTESIAN_POINT('Origin',(3.60994623656552,-10.3,-12.9854006471506));
#143867=CARTESIAN_POINT('',(3.60994623657554,-20.7746200619787,-17.5000000000129));
#143868=CARTESIAN_POINT('',(3.60994623657314,-10.3,-17.5000000000129));
#143869=CARTESIAN_POINT('',(3.60994623656576,-20.7746200619886,-13.1293002508268));
#143870=CARTESIAN_POINT('',(3.60994623656576,-10.3,-13.1293002508268));
#143871=CARTESIAN_POINT('',(3.60994623657044,-20.7746200619855,-15.8999999999905));
#143872=CARTESIAN_POINT('Origin',(-1.26287869055635E-16,-18.2,-19.1));
#143873=CARTESIAN_POINT('',(1.40994623657314,-14.8875912676765,-17.5000000000386));
#143874=CARTESIAN_POINT('',(0.809946236575839,-14.6922960367419,-16.9000000000176));
#143875=CARTESIAN_POINT('Ctrl Pts',(1.40994623657213,-14.887591267676,-17.5000000000166));
#143876=CARTESIAN_POINT('Ctrl Pts',(1.33625361239476,-14.8562235692673,
-17.5000000000166));
#143877=CARTESIAN_POINT('Ctrl Pts',(1.25606667560244,-14.8253033748672,
-17.4855585585683));
#143878=CARTESIAN_POINT('Ctrl Pts',(1.1063385789953,-14.7732966653415,-17.4238130856251));
#143879=CARTESIAN_POINT('Ctrl Pts',(1.03687453723727,-14.7520783114986,
-17.3764332109703));
#143880=CARTESIAN_POINT('Ctrl Pts',(0.930320256457108,-14.7218724492534,
-17.2679197801565));
#143881=CARTESIAN_POINT('Ctrl Pts',(0.885069824864685,-14.710356559554,
-17.2012887424176));
#143882=CARTESIAN_POINT('Ctrl Pts',(0.824877328391394,-14.6956402424863,
-17.0548048739472));
#143883=CARTESIAN_POINT('Ctrl Pts',(0.809946236572128,-14.692296036741,
-16.9749620143834));
#143884=CARTESIAN_POINT('Ctrl Pts',(0.809946236572128,-14.692296036741,
-16.9000000000166));
#143885=CARTESIAN_POINT('',(0.809946236575839,-14.6922960367419,-19.1));
#143886=CARTESIAN_POINT('Ctrl Pts',(1.79710938537606,-15.0806414350073,
-11.8736569225635));
#143887=CARTESIAN_POINT('Ctrl Pts',(1.98632462279995,-15.1896511791408,
-12.0334773325729));
#143888=CARTESIAN_POINT('Ctrl Pts',(2.17985487135821,-15.3247214343457,
-12.1860629633352));
#143889=CARTESIAN_POINT('Ctrl Pts',(2.63411012231677,-15.7199744539229,
-12.5234615495083));
#143890=CARTESIAN_POINT('Ctrl Pts',(2.88145248890814,-16.0115207345657,
-12.6881804314593));
#143891=CARTESIAN_POINT('Ctrl Pts',(3.22898189906331,-16.5797619219656,
-12.9082317714475));
#143892=CARTESIAN_POINT('Ctrl Pts',(3.36909827503896,-16.8871060729476,
-12.9912776188885));
#143893=CARTESIAN_POINT('Ctrl Pts',(3.5547431222469,-17.5379457491925,-13.0987837118773));
#143894=CARTESIAN_POINT('Ctrl Pts',(3.6,-17.8814386363522,-13.1237282076074));
#143895=CARTESIAN_POINT('Ctrl Pts',(3.6,-18.2,-13.1237282076074));
#143896=CARTESIAN_POINT('Origin',(-1.26287869055635E-16,-18.2,-17.5000000000409));
#143897=CARTESIAN_POINT('Origin',(0.,-18.2,-12.1));
#143898=CARTESIAN_POINT('',(-2.,-18.2,-12.1));
#143899=CARTESIAN_POINT('Origin',(0.,-18.2,-12.1));
#143900=CARTESIAN_POINT('',(-1.,-18.2,-12.1));
#143901=CARTESIAN_POINT('Origin',(0.,-18.2,-12.1));
#143902=CARTESIAN_POINT('Origin',(0.,-18.2,-19.1));
#143903=CARTESIAN_POINT('',(-2.,-18.2,-19.1));
#143904=CARTESIAN_POINT('Origin',(0.,-18.2,-19.1));
#143905=CARTESIAN_POINT('',(-2.,-18.2,-19.1));
#143906=CARTESIAN_POINT('Origin',(5.65685424949373,-12.5431457505076,-16.7000000000401));
#143907=CARTESIAN_POINT('',(8.95833898688851,-14.9742357383029,-17.5000000000039));
#143908=CARTESIAN_POINT('',(9.07509596432602,-10.3,-17.4885302101201));
#143909=CARTESIAN_POINT('Ctrl Pts',(8.95833898688868,-14.974235738303,-17.5000000000039));
#143910=CARTESIAN_POINT('Ctrl Pts',(8.96684937916237,-14.9626783996845,
-17.5000000000039));
#143911=CARTESIAN_POINT('Ctrl Pts',(8.97504674785079,-14.9511132665156,
-17.4998189890635));
#143912=CARTESIAN_POINT('Ctrl Pts',(9.09671999843394,-14.7737137436823,
-17.4948316381137));
#143913=CARTESIAN_POINT('Ctrl Pts',(9.17373133832194,-14.590460376238,-17.464473403876));
#143914=CARTESIAN_POINT('Ctrl Pts',(9.29933180973145,-14.2051637392862,
-17.3987460174418));
#143915=CARTESIAN_POINT('Ctrl Pts',(9.34518631085098,-14.0026171612565,
-17.3611498632386));
#143916=CARTESIAN_POINT('Ctrl Pts',(9.44789375510663,-13.3797508448848,
-17.2599642528778));
#143917=CARTESIAN_POINT('Ctrl Pts',(9.47008652427947,-12.9456743678109,
-17.2132322747989));
#143918=CARTESIAN_POINT('Ctrl Pts',(9.47008652427947,-12.5431457505076,
-17.2132322747989));
#143919=CARTESIAN_POINT('Ctrl Pts',(9.47008652427947,-12.1406171332043,
-17.2132322747989));
#143920=CARTESIAN_POINT('Ctrl Pts',(9.44789375510637,-11.7065406561306,
-17.2599642528782));
#143921=CARTESIAN_POINT('Ctrl Pts',(9.34518631085064,-11.0836743397588,
-17.3611498632388));
#143922=CARTESIAN_POINT('Ctrl Pts',(9.29933180973091,-10.8811277617293,
-17.3987460174422));
#143923=CARTESIAN_POINT('Ctrl Pts',(9.19248941207167,-10.5533740834192,
-17.4546572053516));
#143924=CARTESIAN_POINT('Ctrl Pts',(9.14049576625509,-10.4233085064875,
-17.4755557135403));
#143925=CARTESIAN_POINT('Ctrl Pts',(9.07509596432527,-10.3000000000004,
-17.4885302101202));
#143926=CARTESIAN_POINT('Ctrl Pts',(9.07509596432612,-10.3,-17.4885302101202));
#143927=CARTESIAN_POINT('Ctrl Pts',(7.63884118065615,-10.3,-16.2877402533004));
#143928=CARTESIAN_POINT('Ctrl Pts',(6.76061923425244,-10.3,-15.8999999999894));
#143929=CARTESIAN_POINT('',(2.22490186900091,-10.3,-17.5000000000152));
#143930=CARTESIAN_POINT('Ctrl Pts',(4.55308926471108,-10.3,-15.9000000000025));
#143931=CARTESIAN_POINT('Ctrl Pts',(3.67120009968434,-10.3,-16.2893593523261));
#143932=CARTESIAN_POINT('Ctrl Pts',(2.22490186900091,-10.3,-17.5000000000152));
#143933=CARTESIAN_POINT('Origin',(5.65685424949508,-12.5431457505076,-17.5000000000095));
#143934=CARTESIAN_POINT('Origin',(0.809946236563033,-10.3,-11.5097867863747));
#143935=CARTESIAN_POINT('',(0.809946236572127,-10.3,-16.9000000000176));
#143936=CARTESIAN_POINT('',(0.809946236572127,-10.3,-16.9000000000176));
#143937=CARTESIAN_POINT('',(0.809946236545172,-10.3,-0.922764272408981));
#143938=CARTESIAN_POINT('Origin',(1.40994623657213,-10.3,-16.9000000000166));
#143939=CARTESIAN_POINT('',(1.40994623657314,-10.3,-17.5000000000166));
#143940=CARTESIAN_POINT('',(1.40994623657314,-10.3,-17.5000000000166));
#143941=CARTESIAN_POINT('Origin',(1.40994623657213,-10.3,-16.9000000000166));
#143942=CARTESIAN_POINT('Origin',(-13.0020008006734,-10.3,-17.5000000000409));
#143943=CARTESIAN_POINT('',(8.95833898688851,-22.1864655136712,-17.5000000000039));
#143944=CARTESIAN_POINT('',(8.95833898688851,-10.3,-17.5000000000039));
#143945=CARTESIAN_POINT('',(1.52930216884256,-10.3,-17.5000000000164));
#143946=CARTESIAN_POINT('Origin',(5.65685424949508,-23.8568542494924,-17.5000000000094));
#143947=CARTESIAN_POINT('Origin',(5.65685424949238,-23.8568542494924,-15.8999999999905));
#143948=CARTESIAN_POINT('',(9.2027052186294,-22.8,-17.4479827960698));
#143949=CARTESIAN_POINT('',(9.20270521923383,-22.800000001014,-14.8591068129788));
#143950=CARTESIAN_POINT('',(9.20270521862939,-22.8,-15.8999999999905));
#143951=CARTESIAN_POINT('Ctrl Pts',(9.2027052186294,-22.8,-17.4479827960698));
#143952=CARTESIAN_POINT('Ctrl Pts',(9.19834579112383,-22.7853736877598,
-17.4499268294952));
#143953=CARTESIAN_POINT('Ctrl Pts',(9.19389700182971,-22.7707783400677,
-17.4518486125093));
#143954=CARTESIAN_POINT('Ctrl Pts',(9.12772044053632,-22.5583820195644,
-17.4794535144052));
#143955=CARTESIAN_POINT('Ctrl Pts',(9.04959436224867,-22.3668296543679,
-17.5000000000041));
#143956=CARTESIAN_POINT('Ctrl Pts',(8.95833898688636,-22.1864655136723,
-17.5000000000039));
#143957=CARTESIAN_POINT('',(8.72773006566549,-21.7929449196905,-14.5881859109889));
#143958=CARTESIAN_POINT('Ctrl Pts',(3.60994623656577,-20.7746200619886,
-13.1293002508268));
#143959=CARTESIAN_POINT('Ctrl Pts',(3.79140355647922,-20.6541144743078,
-13.2308379582684));
#143960=CARTESIAN_POINT('Ctrl Pts',(3.98575528452356,-20.5483144915821,
-13.3330605413595));
#143961=CARTESIAN_POINT('Ctrl Pts',(4.6518611362006,-20.2604272228388,-13.6577712706292));
#143962=CARTESIAN_POINT('Ctrl Pts',(5.16353509300209,-20.1568542494924,
-13.8653938802152));
#143963=CARTESIAN_POINT('Ctrl Pts',(6.10748558781039,-20.1568542494924,
-14.1743845031205));
#143964=CARTESIAN_POINT('Ctrl Pts',(6.59875708310373,-20.2447590781236,
-14.3012528646996));
#143965=CARTESIAN_POINT('Ctrl Pts',(7.51405499583234,-20.6187655438616,
-14.4783102296068));
#143966=CARTESIAN_POINT('Ctrl Pts',(7.93762194150675,-20.9052246256443,
-14.5301152590098));
#143967=CARTESIAN_POINT('Ctrl Pts',(8.43699112950463,-21.4043064481664,
-14.572534597221));
#143968=CARTESIAN_POINT('Ctrl Pts',(8.5915440810246,-21.5903147747047,-14.5820215238136));
#143969=CARTESIAN_POINT('Ctrl Pts',(8.72773006566549,-21.7929449196905,
-14.5881859109889));
#143970=CARTESIAN_POINT('Ctrl Pts',(9.20270521923383,-22.800000002028,-14.8591068129788));
#143971=CARTESIAN_POINT('Ctrl Pts',(9.19840087688139,-22.7855585059171,
-14.8525270133598));
#143972=CARTESIAN_POINT('Ctrl Pts',(9.19406217050678,-22.7713252500284,
-14.8461774792127));
#143973=CARTESIAN_POINT('Ctrl Pts',(9.09405266484628,-22.4499690063357,
-14.7054086990967));
#143974=CARTESIAN_POINT('Ctrl Pts',(8.92474937148254,-22.0860885247979,
-14.5971038865447));
#143975=CARTESIAN_POINT('Ctrl Pts',(8.72773006566549,-21.7929449196905,
-14.5881859109889));
#143976=CARTESIAN_POINT('Origin',(8.9583389868875,-10.3,-16.9000000000039));
#143977=CARTESIAN_POINT('',(9.5341197068668,-22.8,-16.7312500000035));
#143978=CARTESIAN_POINT('Origin',(8.9583389868875,-22.8,-16.9000000000039));
#143979=CARTESIAN_POINT('',(9.5341197068668,-10.3,-16.7312500000035));
#143980=CARTESIAN_POINT('',(9.5341197068668,-10.3,-16.7312500000035));
#143981=CARTESIAN_POINT('Origin',(8.9583389868875,-10.3,-16.9000000000039));
#143982=CARTESIAN_POINT('Origin',(8.89557956784908,-22.8,-16.359209486979));
#143983=CARTESIAN_POINT('',(9.30054298873711,-22.8,-15.1793622990701));
#143984=CARTESIAN_POINT('Origin',(8.70059915998578,-22.8,-15.1875721920774));
#143985=CARTESIAN_POINT('Origin',(15.1,-22.8,-15.1));
#143986=CARTESIAN_POINT('Origin',(-1.39005376342787,-10.3,-16.9000000000213));
#143987=CARTESIAN_POINT('Origin',(-1.39005376342787,-10.3,-16.9000000000213));
#143988=CARTESIAN_POINT('Origin',(15.1,-10.3,-15.1));
#143989=CARTESIAN_POINT('',(9.30054298873711,-10.3,-15.1793622990701));
#143990=CARTESIAN_POINT('Origin',(15.1,-10.3,-15.1));
#143991=CARTESIAN_POINT('',(9.30054298873711,-10.3,-15.1793622990701));
#143992=CARTESIAN_POINT('Origin',(8.70059915998578,-10.3,-15.1875721920774));
#143993=CARTESIAN_POINT('',(9.15685424949238,-10.3,-14.7979168401324));
#143994=CARTESIAN_POINT('',(8.72773006566549,-10.3967544991228,-14.5881859109889));
#143995=CARTESIAN_POINT('Ctrl Pts',(9.15685424949238,-10.3,-14.7979168401324));
#143996=CARTESIAN_POINT('Ctrl Pts',(9.13480845676445,-10.3,-14.7721029892919));
#143997=CARTESIAN_POINT('Ctrl Pts',(9.11081400901224,-10.3007417728394,
-14.7484812900472));
#143998=CARTESIAN_POINT('Ctrl Pts',(9.02751618170135,-10.3066884459713,
-14.6787793388689));
#143999=CARTESIAN_POINT('Ctrl Pts',(8.94804409342239,-10.3193411582955,
-14.6360996007727));
#144000=CARTESIAN_POINT('Ctrl Pts',(8.82976691205054,-10.3536628217986,
-14.599453582636));
#144001=CARTESIAN_POINT('Ctrl Pts',(8.77818765688933,-10.3727825306704,
-14.5904698473944));
#144002=CARTESIAN_POINT('Ctrl Pts',(8.72773006566549,-10.3967544991228,
-14.5881859109889));
#144003=CARTESIAN_POINT('Origin',(8.70059915998578,-10.3,-15.1875721920774));
#144004=CARTESIAN_POINT('',(8.72773006566549,-10.3,-14.5881859109889));
#144005=CARTESIAN_POINT('Origin',(8.15685424949238,-12.5431457505076,-17.5000000000052));
#144006=CARTESIAN_POINT('',(8.15685424949238,-11.3,-14.5481534330082));
#144007=CARTESIAN_POINT('',(8.15685424949238,-11.3,-13.3421101999983));
#144008=CARTESIAN_POINT('',(8.15685424949238,-11.3,-3.91787087922305));
#144009=CARTESIAN_POINT('',(8.15685424949238,-10.3,-14.5481534330082));
#144010=CARTESIAN_POINT('',(8.15685424949238,-21.1,-13.3421101999983));
#144011=CARTESIAN_POINT('Origin',(9.15685424949238,-11.3,-3.91787087922305));
#144012=CARTESIAN_POINT('',(9.15685424949238,-10.3,-13.3995808547945));
#144013=CARTESIAN_POINT('Ctrl Pts',(8.15685424949238,-11.3,-13.3421101999983));
#144014=CARTESIAN_POINT('Ctrl Pts',(8.15685424949238,-11.1743492779575,
-13.3421101999983));
#144015=CARTESIAN_POINT('Ctrl Pts',(8.18198270554795,-11.040386423148,-13.3448758442539));
#144016=CARTESIAN_POINT('Ctrl Pts',(8.28404532921617,-10.7940569805527,
-13.3549532338642));
#144017=CARTESIAN_POINT('Ctrl Pts',(8.36097444345056,-10.6816828441367,
-13.362131196164));
#144018=CARTESIAN_POINT('Ctrl Pts',(8.53841888019012,-10.5042052130985,
-13.3758933767352));
#144019=CARTESIAN_POINT('Ctrl Pts',(8.65080793814199,-10.4272469229557,
-13.3833767702998));
#144020=CARTESIAN_POINT('Ctrl Pts',(8.8971770787256,-10.3251417681012,-13.3947195510483));
#144021=CARTESIAN_POINT('Ctrl Pts',(9.03116520852081,-10.3,-13.3984496592208));
#144022=CARTESIAN_POINT('Ctrl Pts',(9.15685424949238,-10.3,-13.3995808547945));
#144023=CARTESIAN_POINT('',(9.15685424949238,-10.3,-3.91787087922305));
#144024=CARTESIAN_POINT('Ctrl Pts',(8.72773006566549,-10.3967544991228,
-14.5881859109889));
#144025=CARTESIAN_POINT('Ctrl Pts',(8.62263035139291,-10.4466864711768,
-14.5834286275394));
#144026=CARTESIAN_POINT('Ctrl Pts',(8.52719773482439,-10.5154313193455,
-14.5776230261749));
#144027=CARTESIAN_POINT('Ctrl Pts',(8.36097192174538,-10.6816820908159,
-14.566077401997));
#144028=CARTESIAN_POINT('Ctrl Pts',(8.28403667557063,-10.7940707929597,
-14.5596498341489));
#144029=CARTESIAN_POINT('Ctrl Pts',(8.181975807613,-11.0404101457541,-14.5506281907869));
#144030=CARTESIAN_POINT('Ctrl Pts',(8.15685424949238,-11.1743668352713,
-14.5481534330082));
#144031=CARTESIAN_POINT('Ctrl Pts',(8.15685424949238,-11.3,-14.5481534330082));
#144032=CARTESIAN_POINT('Origin',(3.15685424949238,-10.3,-17.5000000000137));
#144033=CARTESIAN_POINT('',(3.15685424949238,-11.3,-11.4163656902917));
#144034=CARTESIAN_POINT('',(3.15685424949238,-11.3,-12.8620372432944));
#144035=CARTESIAN_POINT('',(3.15685424949238,-11.3,-3.91787087922727));
#144036=CARTESIAN_POINT('',(3.15685424949238,-21.1,-11.4163656902917));
#144037=CARTESIAN_POINT('',(3.15685424949238,-10.3,-12.8620372432944));
#144038=CARTESIAN_POINT('Origin',(9.25,-10.3,-3.05000000003698));
#144039=CARTESIAN_POINT('',(2.15685424949238,-10.3,-12.1653597494959));
#144040=CARTESIAN_POINT('Ctrl Pts',(3.15685424949238,-11.3,-12.8620372432944));
#144041=CARTESIAN_POINT('Ctrl Pts',(3.15685424949238,-11.1762015590292,
-12.8620372432944));
#144042=CARTESIAN_POINT('Ctrl Pts',(3.13234244232117,-11.0457637590431,
-12.8469337261833));
#144043=CARTESIAN_POINT('Ctrl Pts',(3.03750402279937,-10.8094195852156,
-12.7870703131628));
#144044=CARTESIAN_POINT('Ctrl Pts',(2.96735248349465,-10.7034637280328,
-12.7422285875942));
#144045=CARTESIAN_POINT('Ctrl Pts',(2.79365250694672,-10.5158786289393,
-12.6276596027851));
#144046=CARTESIAN_POINT('Ctrl Pts',(2.67252340826556,-10.4319701706144,
-12.5454812826689));
#144047=CARTESIAN_POINT('Ctrl Pts',(2.41575853688544,-10.3241111824561,
-12.3623845936079));
#144048=CARTESIAN_POINT('Ctrl Pts',(2.28025089968914,-10.3,-12.2613812394894));
#144049=CARTESIAN_POINT('Ctrl Pts',(2.15685424949238,-10.3,-12.1653597494959));
#144050=CARTESIAN_POINT('Origin',(9.25,-10.3,-3.05000000003698));
#144051=CARTESIAN_POINT('Origin',(-1.39005376343553,-10.3,-12.3613777665656));
#144052=CARTESIAN_POINT('Origin',(-1.39005376343553,-10.3,-12.3613777665656));
#144053=CARTESIAN_POINT('Origin',(-3.15685424949238,-12.5431457505076,-17.5000000000243));
#144054=CARTESIAN_POINT('',(-3.15685424949238,-11.3,-11.4670924738648));
#144055=CARTESIAN_POINT('',(-3.15685424949238,-11.3,-3.9178708792326));
#144056=CARTESIAN_POINT('',(-3.15685424949238,-15.9,-11.4670924738648));
#144057=CARTESIAN_POINT('Origin',(-9.35,-15.9,-3.05000000003699));
#144058=CARTESIAN_POINT('Origin',(-9.35,-15.9,-3.05000000003699));
#144059=CARTESIAN_POINT('',(-2.15685424949238,-10.3,-10.6303135959217));
#144060=CARTESIAN_POINT('Origin',(-9.35,-10.3,-3.05000000003699));
#144061=CARTESIAN_POINT('Ctrl Pts',(-3.15685424949238,-11.3,-11.4670924738648));
#144062=CARTESIAN_POINT('Ctrl Pts',(-3.15685424949238,-11.1669531550595,
-11.4670924738648));
#144063=CARTESIAN_POINT('Ctrl Pts',(-3.12859247195756,-11.0286485309897,
-11.4464839092837));
#144064=CARTESIAN_POINT('Ctrl Pts',(-3.02305868401783,-10.7827027578499,
-11.3672511996362));
#144065=CARTESIAN_POINT('Ctrl Pts',(-2.94605369112082,-10.6749858792553,
-11.3085067616158));
#144066=CARTESIAN_POINT('Ctrl Pts',(-2.76593743750536,-10.4948696256399,
-11.1659256985317));
#144067=CARTESIAN_POINT('Ctrl Pts',(-2.64696217816639,-10.4182896302278,
-11.0686275519228));
#144068=CARTESIAN_POINT('Ctrl Pts',(-2.39997354427981,-10.3209637887529,
-10.8555260063351));
#144069=CARTESIAN_POINT('Ctrl Pts',(-2.27209385158697,-10.3,-10.7396672847383));
#144070=CARTESIAN_POINT('Ctrl Pts',(-2.15685424949238,-10.3,-10.6303135959217));
#144071=CARTESIAN_POINT('',(-8.15685424949239,-11.3,-13.4316618717243));
#144072=CARTESIAN_POINT('',(-8.15685424949239,-15.9,-13.4316618717243));
#144073=CARTESIAN_POINT('',(-9.15685424949239,-10.3,-13.4982149058982));
#144074=CARTESIAN_POINT('Ctrl Pts',(-9.15685424949239,-10.3,-13.4982149058982));
#144075=CARTESIAN_POINT('Ctrl Pts',(-9.03112180920881,-10.3,-13.4958906154084));
#144076=CARTESIAN_POINT('Ctrl Pts',(-8.89711190098953,-10.3251571822744,
-13.4909106549527));
#144077=CARTESIAN_POINT('Ctrl Pts',(-8.65072463395046,-10.4272930525798,
-13.4773072697496));
#144078=CARTESIAN_POINT('Ctrl Pts',(-8.53833784786347,-10.5042659905921,
-13.4688117245097));
#144079=CARTESIAN_POINT('Ctrl Pts',(-8.36093460719447,-10.6817429599976,
-13.4534691379964));
#144080=CARTESIAN_POINT('Ctrl Pts',(-8.28402699211168,-10.7940934369191,
-13.4456161349629));
#144081=CARTESIAN_POINT('Ctrl Pts',(-8.1819838951961,-11.0403913536937,
-13.4346459578849));
#144082=CARTESIAN_POINT('Ctrl Pts',(-8.15685424949239,-11.174347121187,
-13.4316618717243));
#144083=CARTESIAN_POINT('Ctrl Pts',(-8.15685424949239,-11.3,-13.4316618717243));
#144084=CARTESIAN_POINT('Origin',(-9.35,-10.3,-3.05000000003699));
#144085=CARTESIAN_POINT('Origin',(-8.15685424949238,-10.3,-17.5000000000328));
#144086=CARTESIAN_POINT('',(-8.15685424949239,-11.3,-3.91787087923682));
#144087=CARTESIAN_POINT('Origin',(9.25,-21.1,-3.05000000003699));
#144088=CARTESIAN_POINT('',(2.15685424949238,-10.3,-10.5872265033375));
#144089=CARTESIAN_POINT('Ctrl Pts',(2.15685424949238,-10.3,-10.5872265033375));
#144090=CARTESIAN_POINT('Ctrl Pts',(2.27216752689059,-10.3,-10.6957457157024));
#144091=CARTESIAN_POINT('Ctrl Pts',(2.4001077317982,-10.3209951024604,-10.8106623925262));
#144092=CARTESIAN_POINT('Ctrl Pts',(2.64710933942602,-10.4183692065858,
-11.0218717794871));
#144093=CARTESIAN_POINT('Ctrl Pts',(2.76603569567595,-10.4949678838105,
-11.1182210617341));
#144094=CARTESIAN_POINT('Ctrl Pts',(2.94615370539162,-10.6750858935261,
-11.259441539498));
#144095=CARTESIAN_POINT('Ctrl Pts',(3.02316861067196,-10.7828869566871,
-11.3176108509303));
#144096=CARTESIAN_POINT('Ctrl Pts',(3.12864992256832,-11.0288545184812,
-11.3960105022376));
#144097=CARTESIAN_POINT('Ctrl Pts',(3.15685424949238,-11.1670935229091,
-11.4163656902917));
#144098=CARTESIAN_POINT('Ctrl Pts',(3.15685424949238,-11.3,-11.4163656902917));
#144099=CARTESIAN_POINT('Origin',(9.25,-10.3,-3.05000000003699));
#144100=CARTESIAN_POINT('Origin',(9.25,-15.9,-3.05000000003699));
#144101=CARTESIAN_POINT('Origin',(9.25,-10.3,-3.05000000003699));
#144102=CARTESIAN_POINT('Origin',(2.15685424949238,-11.3,-3.91787087922727));
#144103=CARTESIAN_POINT('',(2.15685424949238,-10.3,-3.91787087922727));
#144104=CARTESIAN_POINT('Origin',(-2.15685424949238,-11.3,-3.9178708792326));
#144105=CARTESIAN_POINT('',(-2.15685424949238,-10.3,-3.9178708792326));
#144106=CARTESIAN_POINT('Origin',(-9.15685424949239,-11.3,-3.91787087923682));
#144107=CARTESIAN_POINT('',(-9.15685424949239,-10.3,-3.91787087923682));
#144108=CARTESIAN_POINT('Origin',(2.24865810106615,-10.3,9.66425824155912));
#144109=CARTESIAN_POINT('',(13.8193751525349,-10.3,-19.1000000000069));
#144110=CARTESIAN_POINT('Origin',(19.1,-24.4,-19.1));
#144111=CARTESIAN_POINT('',(9.54999999998871,-25.4,-19.1));
#144112=CARTESIAN_POINT('',(9.54999999998871,-25.4,-19.1));
#144113=CARTESIAN_POINT('',(9.54999999998871,-25.4,-19.1));
#144114=CARTESIAN_POINT('',(-69.9000013262034,-22.1,-19.1));
#144115=CARTESIAN_POINT('Origin',(11.2998162594733,-10.3,10.1607140398676));
#144116=CARTESIAN_POINT('',(10.69984250812,-11.3,10.1663263198865));
#144117=CARTESIAN_POINT('',(11.3890749660464,-10.5645232201992,9.56739044915099));
#144118=CARTESIAN_POINT('Ctrl Pts',(10.69984250812,-11.3,10.1663263198865));
#144119=CARTESIAN_POINT('Ctrl Pts',(10.6992150492722,-11.3,10.0992486193006));
#144120=CARTESIAN_POINT('Ctrl Pts',(10.7105416393666,-11.2859681238687,
10.0298809986402));
#144121=CARTESIAN_POINT('Ctrl Pts',(10.7531080502661,-11.2354954752618,
9.90483916612018));
#144122=CARTESIAN_POINT('Ctrl Pts',(10.78415813957,-11.1993829121916,9.84896825061679));
#144123=CARTESIAN_POINT('Ctrl Pts',(10.8663746357755,-11.1058434210861,
9.73764581751491));
#144124=CARTESIAN_POINT('Ctrl Pts',(10.9287151162477,-11.0366106450061,
9.68269383698243));
#144125=CARTESIAN_POINT('Ctrl Pts',(11.0648458019447,-10.8905755867573,
9.60303292733449));
#144126=CARTESIAN_POINT('Ctrl Pts',(11.1386925567721,-10.8137589718382,
9.57844696758312));
#144127=CARTESIAN_POINT('Ctrl Pts',(11.2085510069148,-10.7430780618347,
9.56769578241224));
#144128=CARTESIAN_POINT('Ctrl Pts',(11.2653388943385,-10.68562159734,9.55895615117352));
#144129=CARTESIAN_POINT('Ctrl Pts',(11.3269631854058,-10.6246068030101,
9.55804644650272));
#144130=CARTESIAN_POINT('Ctrl Pts',(11.3890749660464,-10.5645232201992,
9.56739044915099));
#144131=CARTESIAN_POINT('',(11.3890749660464,-10.3,9.56739044915099));
#144132=CARTESIAN_POINT('',(11.3890749660464,-10.3,9.56739044915099));
#144133=CARTESIAN_POINT('',(10.69984250812,-10.3,10.1663263198865));
#144134=CARTESIAN_POINT('Origin',(11.2998162594733,-10.3,10.1607140398676));
#144135=CARTESIAN_POINT('',(10.69984250812,-10.3,10.1663263198865));
#144136=CARTESIAN_POINT('Origin',(3.68732223444763,-10.3,7.75181077763493));
#144137=CARTESIAN_POINT('',(4.17484762952654,-11.3,8.10155209511566));
#144138=CARTESIAN_POINT('Ctrl Pts',(3.96202237101816,-10.5713843344211,
7.21838802318202));
#144139=CARTESIAN_POINT('Ctrl Pts',(4.01561068343958,-10.6292415447907,
7.24598474007845));
#144140=CARTESIAN_POINT('Ctrl Pts',(4.06327615070688,-10.6878073192481,
7.28094613908644));
#144141=CARTESIAN_POINT('Ctrl Pts',(4.15407930627617,-10.8137589718382,
7.36823076389991));
#144142=CARTESIAN_POINT('Ctrl Pts',(4.20033921266016,-10.8905755867573,
7.43082336471489));
#144143=CARTESIAN_POINT('Ctrl Pts',(4.26586151345588,-11.0366106450061,
7.57429549515384));
#144144=CARTESIAN_POINT('Ctrl Pts',(4.28524090449668,-11.1058434210861,
7.65510697251215));
#144145=CARTESIAN_POINT('Ctrl Pts',(4.28844947659775,-11.1993829121916,
7.79346137766468));
#144146=CARTESIAN_POINT('Ctrl Pts',(4.28170596499445,-11.2354954752618,
7.85702388466544));
#144147=CARTESIAN_POINT('Ctrl Pts',(4.24458994202194,-11.2859681238687,
7.98379044198844));
#144148=CARTESIAN_POINT('Ctrl Pts',(4.21394907908761,-11.3,8.04704623980883));
#144149=CARTESIAN_POINT('Ctrl Pts',(4.17484762952654,-11.3,8.10155209511565));
#144150=CARTESIAN_POINT('',(4.17484762952654,-10.3,8.10155209511566));
#144151=CARTESIAN_POINT('',(4.17484762952654,-10.3,8.10155209511566));
#144152=CARTESIAN_POINT('Origin',(3.68732223444763,-10.3,7.75181077763493));
#144153=CARTESIAN_POINT('Origin',(7.47499999999962,-14.8,14.199999999963));
#144154=CARTESIAN_POINT('',(7.64999999999965,-11.7199299841877,13.3321470759639));
#144155=CARTESIAN_POINT('',(7.41177157822234,-12.1000000000004,12.9825884501688));
#144156=CARTESIAN_POINT('Ctrl Pts',(7.64999999999965,-11.7199299841877,
13.3321470759639));
#144157=CARTESIAN_POINT('Ctrl Pts',(7.61868756556843,-11.7633272734221,
13.2935842063427));
#144158=CARTESIAN_POINT('Ctrl Pts',(7.58861560393998,-11.8067445070237,
13.2545025807997));
#144159=CARTESIAN_POINT('Ctrl Pts',(7.50520657393635,-11.9331277607182,
13.1393811397357));
#144160=CARTESIAN_POINT('Ctrl Pts',(7.455490303221,-12.0162549490882,13.0619591119168));
#144161=CARTESIAN_POINT('Ctrl Pts',(7.41177157822295,-12.1000000000003,
12.9825884501684));
#144162=CARTESIAN_POINT('',(7.29999999999962,-12.2182788550814,12.9928480087538));
#144163=CARTESIAN_POINT('Ctrl Pts',(7.41177157822255,-12.1000000000006,
12.9825884501688));
#144164=CARTESIAN_POINT('Ctrl Pts',(7.3743512628699,-12.1391578411027,12.9867811617336));
#144165=CARTESIAN_POINT('Ctrl Pts',(7.33707673963459,-12.1785907678552,
12.9901928882805));
#144166=CARTESIAN_POINT('Ctrl Pts',(7.29999999999961,-12.2182788550814,
12.9928480087538));
#144167=CARTESIAN_POINT('',(7.29999999999956,-12.5535531013342,15.9538461538416));
#144168=CARTESIAN_POINT('Origin',(7.29999999999959,-14.8,14.199999999963));
#144169=CARTESIAN_POINT('Ctrl Pts',(7.29999999999956,-12.5535531013342,
15.9538461538416));
#144170=CARTESIAN_POINT('Ctrl Pts',(7.29999999999956,-12.5814935453447,
15.9896341981098));
#144171=CARTESIAN_POINT('Ctrl Pts',(7.30941758154832,-12.6038504815788,
16.0316406923603));
#144172=CARTESIAN_POINT('Ctrl Pts',(7.34336734883734,-12.6320030732815,
16.1165268946216));
#144173=CARTESIAN_POINT('Ctrl Pts',(7.36769238401017,-12.6379779471448,
16.1594297908438));
#144174=CARTESIAN_POINT('Ctrl Pts',(7.43072186332663,-12.6386585391172,
16.2530509386545));
#144175=CARTESIAN_POINT('Ctrl Pts',(7.47734347162638,-12.6270638876253,
16.3079691869699));
#144176=CARTESIAN_POINT('Ctrl Pts',(7.57576120928368,-12.585316726708,16.4059033715659));
#144177=CARTESIAN_POINT('Ctrl Pts',(7.62758928926194,-12.5550504765137,
16.4488386620803));
#144178=CARTESIAN_POINT('Ctrl Pts',(7.67529068457363,-12.5213497005712,
16.482597821068));
#144179=CARTESIAN_POINT('Ctrl Pts',(7.7264149551059,-12.485230681931,16.5187794121043));
#144180=CARTESIAN_POINT('Ctrl Pts',(7.78179221084198,-12.4388020333086,
16.5507601268268));
#144181=CARTESIAN_POINT('Ctrl Pts',(7.87967710828239,-12.3400773625447,
16.5899436813847));
#144182=CARTESIAN_POINT('Ctrl Pts',(7.92296055726618,-12.2894858062932,
16.6));
#144183=CARTESIAN_POINT('Ctrl Pts',(7.9603418636975,-12.238262308539,16.6));
#144184=CARTESIAN_POINT('',(7.64999999999961,-12.1392658583161,15.9777777777737));
#144185=CARTESIAN_POINT('Ctrl Pts',(7.64999999999963,-12.1392658583161,
15.9777777777737));
#144186=CARTESIAN_POINT('Ctrl Pts',(7.64999999999963,-12.1647190199888,
16.0158725819284));
#144187=CARTESIAN_POINT('Ctrl Pts',(7.65945587523489,-12.1840248468099,
16.0598458438056));
#144188=CARTESIAN_POINT('Ctrl Pts',(7.6935871828228,-12.2057670409854,16.1474492768948));
#144189=CARTESIAN_POINT('Ctrl Pts',(7.71806257389703,-12.208379932636,16.1911133687284));
#144190=CARTESIAN_POINT('Ctrl Pts',(7.78149608588271,-12.2015215184701,
16.2853111664178));
#144191=CARTESIAN_POINT('Ctrl Pts',(7.82839529686648,-12.1853531341838,
16.3395239080143));
#144192=CARTESIAN_POINT('Ctrl Pts',(7.92745916770871,-12.1352560207032,
16.4343503422875));
#144193=CARTESIAN_POINT('Ctrl Pts',(7.97965638032824,-12.101215923928,16.4748711334417));
#144194=CARTESIAN_POINT('Ctrl Pts',(8.02770876399932,-12.0644749514664,
16.5058409981337));
#144195=CARTESIAN_POINT('Ctrl Pts',(8.07847474046147,-12.0256591591853,
16.5385597792197));
#144196=CARTESIAN_POINT('Ctrl Pts',(8.13347864575108,-11.9770409104891,
16.5663042200272));
#144197=CARTESIAN_POINT('Ctrl Pts',(8.22123438481492,-11.8859917604215,
16.5939479694972));
#144198=CARTESIAN_POINT('Ctrl Pts',(8.2555385114276,-11.8465704328685,16.6));
#144199=CARTESIAN_POINT('Ctrl Pts',(8.28666521865376,-11.8066740906056,
16.6));
#144200=CARTESIAN_POINT('Origin',(7.64999999999965,-14.8,14.199999999963));
#144201=CARTESIAN_POINT('Origin',(7.1,-24.4,10.2));
#144202=CARTESIAN_POINT('',(9.89635480722185,-12.1,10.0571721591311));
#144203=CARTESIAN_POINT('',(9.89635480722185,-17.7372583002031,10.0571721591311));
#144204=CARTESIAN_POINT('',(9.89635480722185,-10.3,10.0571721591311));
#144205=CARTESIAN_POINT('',(8.7218665882827,-12.1000000000115,12.4824435961951));
#144206=CARTESIAN_POINT('Origin',(7.1,-12.1,10.2));
#144207=CARTESIAN_POINT('Ctrl Pts',(9.32485954600978,-17.0248595463278,
11.9000000001556));
#144208=CARTESIAN_POINT('Ctrl Pts',(9.34001112247009,-17.0043603546528,
11.8801705122017));
#144209=CARTESIAN_POINT('Ctrl Pts',(9.35447849265797,-16.9836680437391,
11.8606864486227));
#144210=CARTESIAN_POINT('Ctrl Pts',(9.54024107063934,-16.703804134771,11.6040173789117));
#144211=CARTESIAN_POINT('Ctrl Pts',(9.64482709960529,-16.3646990093396,
11.3790747377687));
#144212=CARTESIAN_POINT('Ctrl Pts',(9.76404695970622,-15.608125281439,11.0770456465201));
#144213=CARTESIAN_POINT('Ctrl Pts',(9.78328157301077,-15.1913725392454,
10.999999999963));
#144214=CARTESIAN_POINT('Ctrl Pts',(9.78328157301077,-14.4086274607546,
10.999999999963));
#144215=CARTESIAN_POINT('Ctrl Pts',(9.76404695970622,-13.991874718561,11.0770456465201));
#144216=CARTESIAN_POINT('Ctrl Pts',(9.64482709960529,-13.2353009906604,
11.3790747377687));
#144217=CARTESIAN_POINT('Ctrl Pts',(9.54024107063934,-12.896195865229,11.6040173789117));
#144218=CARTESIAN_POINT('Ctrl Pts',(9.22419326738574,-12.4200484376874,
12.0407021866206));
#144219=CARTESIAN_POINT('Ctrl Pts',(8.98968945737333,-12.2245160908571,
12.2888237365864));
#144220=CARTESIAN_POINT('Ctrl Pts',(8.73475193252056,-12.1058672399844,
12.4732461679086));
#144221=CARTESIAN_POINT('Ctrl Pts',(8.72832975141059,-12.1029215104077,
12.4778509796025));
#144222=CARTESIAN_POINT('Ctrl Pts',(8.72186658827967,-12.1000000000216,
12.4824435961973));
#144223=CARTESIAN_POINT('Origin',(7.1,-17.7372583002031,10.2));
#144224=CARTESIAN_POINT('Origin',(7.1,-10.3,10.2));
#144225=CARTESIAN_POINT('Origin',(7.1,-10.3,10.2));
#144226=CARTESIAN_POINT('Origin',(7.1,-11.3,10.2));
#144227=CARTESIAN_POINT('Origin',(8.49999999999956,-12.238262308539,16.2));
#144228=CARTESIAN_POINT('',(8.49999999999956,-12.5535531013342,15.9538461538416));
#144229=CARTESIAN_POINT('Origin',(15.1,-10.3,-15.1000000000002));
#144230=CARTESIAN_POINT('',(4.67225419943745,-11.3140320785605,7.56083038410859));
#144231=CARTESIAN_POINT('',(4.67225419942505,-18.5232262216426,7.56083038411999));
#144232=CARTESIAN_POINT('',(4.67225419943745,-10.3,7.56083038410859));
#144233=CARTESIAN_POINT('',(4.65844715578268,-11.3,7.55447175239154));
#144234=CARTESIAN_POINT('Ctrl Pts',(4.65844715578268,-11.3,7.55447175239154));
#144235=CARTESIAN_POINT('Ctrl Pts',(4.66304985477283,-11.3046805476178,
7.55659315805736));
#144236=CARTESIAN_POINT('Ctrl Pts',(4.66765219994199,-11.3093579116597,
7.558712699977));
#144237=CARTESIAN_POINT('Ctrl Pts',(4.67225419943745,-11.3140320785604,
7.56083038410858));
#144238=CARTESIAN_POINT('Ctrl Pts',(4.20575266919785,-10.8312625177592,
7.34028723688267));
#144239=CARTESIAN_POINT('Ctrl Pts',(4.35718070025283,-10.9906489469993,
7.41380209013365));
#144240=CARTESIAN_POINT('Ctrl Pts',(4.5080049398014,-11.1470132508919,7.48513222572595));
#144241=CARTESIAN_POINT('Ctrl Pts',(4.65844715578268,-11.3,7.55447175239154));
#144242=CARTESIAN_POINT('Ctrl Pts',(4.20575266919785,-19.0059957824439,
7.34028723688266));
#144243=CARTESIAN_POINT('Ctrl Pts',(4.36181367819661,-18.8417328861054,
7.41605129519349));
#144244=CARTESIAN_POINT('Ctrl Pts',(4.51723285276396,-18.6806785743082,
7.48949481655117));
#144245=CARTESIAN_POINT('Ctrl Pts',(4.67225419943426,-18.5232262216458,
7.56083038410712));
#144246=CARTESIAN_POINT('Origin',(-2.356826353498,-10.3,7.0077344540968));
#144247=CARTESIAN_POINT('',(-2.6993491429948,-16.3017075537437,6.51511072479082));
#144248=CARTESIAN_POINT('',(-2.87773485737152,-16.5848708742773,7.30548322503002));
#144249=CARTESIAN_POINT('Ctrl Pts',(-2.69934914221477,-16.3017075545574,
6.51511072424847));
#144250=CARTESIAN_POINT('Ctrl Pts',(-2.74531797479244,-16.3670746844141,
6.54707299438395));
#144251=CARTESIAN_POINT('Ctrl Pts',(-2.78651988585169,-16.4308362330594,
6.58526323998097));
#144252=CARTESIAN_POINT('Ctrl Pts',(-2.85722586073441,-16.547448699515,
6.67196627688682));
#144253=CARTESIAN_POINT('Ctrl Pts',(-2.89124061589894,-16.6082776579722,
6.72661902786091));
#144254=CARTESIAN_POINT('Ctrl Pts',(-2.92845981168729,-16.6785516418896,
6.8221836431129));
#144255=CARTESIAN_POINT('Ctrl Pts',(-2.93858697485447,-16.6983485015077,
6.85634795597679));
#144256=CARTESIAN_POINT('Ctrl Pts',(-2.9527704395822,-16.7264359005426,
6.92887841593282));
#144257=CARTESIAN_POINT('Ctrl Pts',(-2.95682635349799,-16.7346748090408,
6.96726462231166));
#144258=CARTESIAN_POINT('Ctrl Pts',(-2.95682635349799,-16.7346748090408,
7.04820428588195));
#144259=CARTESIAN_POINT('Ctrl Pts',(-2.9527704395822,-16.7264359005426,
7.08659049226079));
#144260=CARTESIAN_POINT('Ctrl Pts',(-2.93858697485447,-16.6983485015077,
7.15912095221682));
#144261=CARTESIAN_POINT('Ctrl Pts',(-2.92845981168729,-16.6785516418896,
7.1932852650807));
#144262=CARTESIAN_POINT('Ctrl Pts',(-2.90488679928763,-16.6340431709469,
7.25381171689106));
#144263=CARTESIAN_POINT('Ctrl Pts',(-2.89191125967647,-16.6101294913542,
7.28068175067744));
#144264=CARTESIAN_POINT('Ctrl Pts',(-2.87773485721227,-16.5848708746402,
7.30548322530863));
#144265=CARTESIAN_POINT('',(-2.69934914434707,-10.3,6.51511072573106));
#144266=CARTESIAN_POINT('',(-2.69934914434707,-10.3,6.51511072573106));
#144267=CARTESIAN_POINT('',(-2.87773485773448,-10.3,7.30548322439503));
#144268=CARTESIAN_POINT('Origin',(-2.356826353498,-10.3,7.0077344540968));
#144269=CARTESIAN_POINT('',(-2.87773485773448,-10.3,7.30548322439503));
#144270=CARTESIAN_POINT('Origin',(-8.4775012782713,-10.3,10.5062825050979));
#144271=CARTESIAN_POINT('',(-4.07042440724209,-10.3,15.2158656557344));
#144272=CARTESIAN_POINT('Origin',(-8.4775012782713,-10.3,10.5062825050979));
#144273=CARTESIAN_POINT('',(-4.07042440724209,-15.4372006646508,15.2158656557344));
#144274=CARTESIAN_POINT('',(-4.07042440724209,-10.3,15.2158656557344));
#144275=CARTESIAN_POINT('',(-3.33223732524944,-14.0144660545858,14.3958530281318));
#144276=CARTESIAN_POINT('Ctrl Pts',(-4.07042440724209,-15.4372006646508,
15.2158656557344));
#144277=CARTESIAN_POINT('Ctrl Pts',(-4.03861146906795,-15.3625014535314,
15.1860961284658));
#144278=CARTESIAN_POINT('Ctrl Pts',(-4.0059205861772,-15.2886209362891,
15.1548999501354));
#144279=CARTESIAN_POINT('Ctrl Pts',(-3.77494925612046,-14.7841712702143,
14.929484770533));
#144280=CARTESIAN_POINT('Ctrl Pts',(-3.5505954637745,-14.3821453612863,
14.6847050369457));
#144281=CARTESIAN_POINT('Ctrl Pts',(-3.33223732524944,-14.0144660545858,
14.3958530281318));
#144282=CARTESIAN_POINT('',(-2.06491552545779,-13.264554338996,11.2));
#144283=CARTESIAN_POINT('Ctrl Pts',(-3.33223732524944,-14.0144660545858,
14.3958530281318));
#144284=CARTESIAN_POINT('Ctrl Pts',(-2.97652069716172,-13.7312686798221,
13.9252982629844));
#144285=CARTESIAN_POINT('Ctrl Pts',(-2.64594985001838,-13.5429439336592,
13.343649108976));
#144286=CARTESIAN_POINT('Ctrl Pts',(-2.23928412359358,-13.3371720517063,
12.2247807719029));
#144287=CARTESIAN_POINT('Ctrl Pts',(-2.12002313078455,-13.2876105243186,
11.7094036800094));
#144288=CARTESIAN_POINT('Ctrl Pts',(-2.06491552545779,-13.264554338996,
11.2));
#144289=CARTESIAN_POINT('',(-2.17171046614589,-15.7153121622159,9.14999999999999));
#144290=CARTESIAN_POINT('Ctrl Pts',(-2.06491552545779,-13.264554338996,
11.2));
#144291=CARTESIAN_POINT('Ctrl Pts',(-2.01806542640658,-13.7144020133522,
10.7669270561843));
#144292=CARTESIAN_POINT('Ctrl Pts',(-2.01903789024593,-14.176467536479,
10.3450743353087));
#144293=CARTESIAN_POINT('Ctrl Pts',(-2.06556093124264,-14.8558616960581,
9.77835970509417));
#144294=CARTESIAN_POINT('Ctrl Pts',(-2.09659729559528,-15.1499390919158,
9.54682356160579));
#144295=CARTESIAN_POINT('Ctrl Pts',(-2.14186392109874,-15.5009332716129,
9.29495491302226));
#144296=CARTESIAN_POINT('Ctrl Pts',(-2.15622982991206,-15.6061897771793,
9.22197442521173));
#144297=CARTESIAN_POINT('Ctrl Pts',(-2.17171046614589,-15.7153121622159,
9.14999999999999));
#144298=CARTESIAN_POINT('Ctrl Pts',(-2.17171046614589,-15.7153121622159,
9.14999999999999));
#144299=CARTESIAN_POINT('Ctrl Pts',(-2.21590083179177,-15.7539362010656,
8.94454486758705));
#144300=CARTESIAN_POINT('Ctrl Pts',(-2.26974837175159,-15.8029699038511,
8.74353599076851));
#144301=CARTESIAN_POINT('Ctrl Pts',(-2.42818675997411,-15.9610882759758,
8.24557800636064));
#144302=CARTESIAN_POINT('Ctrl Pts',(-2.54447355256091,-16.0886251879561,
7.96074874984413));
#144303=CARTESIAN_POINT('Ctrl Pts',(-2.73607614870722,-16.3511725332041,
7.56266001973146));
#144304=CARTESIAN_POINT('Ctrl Pts',(-2.80802393475142,-16.460664364867,
7.42744178898432));
#144305=CARTESIAN_POINT('Ctrl Pts',(-2.87773485721227,-16.5848708746402,
7.30548322530863));
#144306=CARTESIAN_POINT('Origin',(0.0177419354838726,-10.3,5.45105352468434));
#144307=CARTESIAN_POINT('',(-0.722791023811509,-16.12212292569,4.77903348316978));
#144308=CARTESIAN_POINT('Ctrl Pts',(0.753380028237917,-16.1330170457761,
4.77367874179883));
#144309=CARTESIAN_POINT('Ctrl Pts',(0.74409769330423,-16.1296337930307,
4.76359800165401));
#144310=CARTESIAN_POINT('Ctrl Pts',(0.734669071608476,-16.126268178292,
4.75377451472814));
#144311=CARTESIAN_POINT('Ctrl Pts',(0.637473178290217,-16.092336359572,
4.65650419393023));
#144312=CARTESIAN_POINT('Ctrl Pts',(0.526282739188228,-16.0602162963568,
4.57976205448264));
#144313=CARTESIAN_POINT('Ctrl Pts',(0.280340152199377,-16.0143519898035,
4.47698741133051));
#144314=CARTESIAN_POINT('Ctrl Pts',(0.145454989338261,-16.0011015187019,
4.45105352468434));
#144315=CARTESIAN_POINT('Ctrl Pts',(-0.109580731505419,-15.9990447121329,
4.45105352468434));
#144316=CARTESIAN_POINT('Ctrl Pts',(-0.244282057994744,-16.0100526854273,
4.4768451524154));
#144317=CARTESIAN_POINT('Ctrl Pts',(-0.490127096915344,-16.0516707912072,
4.57938413049508));
#144318=CARTESIAN_POINT('Ctrl Pts',(-0.601393492215431,-16.0817799830708,
4.65603999011667));
#144319=CARTESIAN_POINT('Ctrl Pts',(-0.700521533797108,-16.1144751009463,
4.75509513111577));
#144320=CARTESIAN_POINT('Ctrl Pts',(-0.7117644146194,-16.118287311821,4.76688270338414));
#144321=CARTESIAN_POINT('Ctrl Pts',(-0.72279102380988,-16.1221229257004,
4.77903348316799));
#144322=CARTESIAN_POINT('',(-0.722791023842917,-10.3,4.77903348320439));
#144323=CARTESIAN_POINT('Origin',(0.0177419354838726,-10.3,5.45105352468434));
#144324=CARTESIAN_POINT('',(-0.722791023842917,-10.3,4.77903348320439));
#144325=CARTESIAN_POINT('Origin',(-9.35,-10.3,-3.05000000003699));
#144326=CARTESIAN_POINT('',(-2.26762751619799,-15.8025293645632,6.19999999999999));
#144327=CARTESIAN_POINT('Ctrl Pts',(-2.69934914221477,-16.3017075545574,
6.51511072424847));
#144328=CARTESIAN_POINT('Ctrl Pts',(-2.5724485882362,-16.1212564853078,
6.42687637939889));
#144329=CARTESIAN_POINT('Ctrl Pts',(-2.42570115325786,-15.9520419899461,
6.32103095973219));
#144330=CARTESIAN_POINT('Ctrl Pts',(-2.26762751619799,-15.8025293645632,
6.19999999999999));
#144331=CARTESIAN_POINT('',(-1.02533784472924,-16.2535462234705,5.09999999999999));
#144332=CARTESIAN_POINT('Ctrl Pts',(-2.26762751619799,-15.8025293645632,
6.19999999999999));
#144333=CARTESIAN_POINT('Ctrl Pts',(-1.8764893960922,-15.8447934730179,
5.90052044765489));
#144334=CARTESIAN_POINT('Ctrl Pts',(-1.50140793289236,-15.9797824776671,
5.57275424042926));
#144335=CARTESIAN_POINT('Ctrl Pts',(-1.11481261265353,-16.1987537307299,
5.19064987199639));
#144336=CARTESIAN_POINT('Ctrl Pts',(-1.06975596859005,-16.2256644836538,
5.14537004597675));
#144337=CARTESIAN_POINT('Ctrl Pts',(-1.02533784472924,-16.2535462234705,
5.09999999999999));
#144338=CARTESIAN_POINT('Ctrl Pts',(-1.02533784472924,-16.2535462234705,
5.09999999999999));
#144339=CARTESIAN_POINT('Ctrl Pts',(-1.0092117726784,-16.2450514561352,
5.083528331078));
#144340=CARTESIAN_POINT('Ctrl Pts',(-0.993056266977858,-16.2367972149681,
5.0669287615527));
#144341=CARTESIAN_POINT('Ctrl Pts',(-0.892245880391997,-16.1868384475464,
4.96272194243645));
#144342=CARTESIAN_POINT('Ctrl Pts',(-0.807070308040803,-16.1514395348919,
4.87190509994976));
#144343=CARTESIAN_POINT('Ctrl Pts',(-0.722791023809883,-16.1221229257004,
4.77903348316799));
#144344=CARTESIAN_POINT('Origin',(-9.35,-10.3,-3.05000000003699));
#144345=CARTESIAN_POINT('Origin',(1.68452938230201E-16,-18.2,11.8));
#144346=CARTESIAN_POINT('',(4.15,-18.2,12.));
#144347=CARTESIAN_POINT('Origin',(1.9309146098219E-16,-18.2,12.));
#144348=CARTESIAN_POINT('',(3.75,-18.2,11.6));
#144349=CARTESIAN_POINT('',(3.95,-18.2,11.8));
#144350=CARTESIAN_POINT('Origin',(1.43814415478212E-16,-18.2,11.6));
#144351=CARTESIAN_POINT('Origin',(1.7735870188571E-16,-18.2,11.6));
#144352=CARTESIAN_POINT('',(2.4,-18.2,11.6));
#144353=CARTESIAN_POINT('Origin',(3.59031095959199E-16,-18.2,11.6));
#144354=CARTESIAN_POINT('Origin',(1.04273619012177E-16,-18.2,11.6));
#144355=CARTESIAN_POINT('',(4.15,-18.2,14.1));
#144356=CARTESIAN_POINT('',(4.15,-18.2,11.6));
#144357=CARTESIAN_POINT('Origin',(6.59385131324756E-16,-18.2,14.1));
#144358=CARTESIAN_POINT('Origin',(3.46711834583204E-16,-18.2,11.5));
#144359=CARTESIAN_POINT('',(2.1,-18.2,11.4));
#144360=CARTESIAN_POINT('',(2.25,-18.2,11.5));
#144361=CARTESIAN_POINT('Origin',(3.3439257320721E-16,-18.2,11.4));
#144362=CARTESIAN_POINT('Origin',(7.1,-24.4,10.2));
#144363=CARTESIAN_POINT('',(9.9,-25.4,10.2));
#144364=CARTESIAN_POINT('Origin',(7.1,-25.4,10.2));
#144365=CARTESIAN_POINT('',(9.9,-20.8,10.2));
#144366=CARTESIAN_POINT('',(9.9,-24.4,10.2));
#144367=CARTESIAN_POINT('Origin',(7.1,-20.8,10.2));
#144368=CARTESIAN_POINT('Origin',(8.49999999999959,-14.8,14.199999999963));
#144369=CARTESIAN_POINT('Ctrl Pts',(7.29999999999962,-12.2182788550814,
12.9928480087538));
#144370=CARTESIAN_POINT('Ctrl Pts',(7.23242869523073,-12.2160163080132,
12.9976868903941));
#144371=CARTESIAN_POINT('Ctrl Pts',(7.16556025075935,-12.2149468090407,
13.));
#144372=CARTESIAN_POINT('Ctrl Pts',(6.84067152517238,-12.2149468090407,
13.));
#144373=CARTESIAN_POINT('Ctrl Pts',(6.56105708740227,-12.231704090976,12.9613548244849));
#144374=CARTESIAN_POINT('Ctrl Pts',(6.03441613857713,-12.3138039205035,
12.8038566188284));
#144375=CARTESIAN_POINT('Ctrl Pts',(5.78755856457603,-12.3805717968042,
12.6851850087052));
#144376=CARTESIAN_POINT('Ctrl Pts',(5.55598060272308,-12.4860759700654,
12.5360460877507));
#144377=CARTESIAN_POINT('Ctrl Pts',(5.52791362209311,-12.4996785494448,
12.517261610228));
#144378=CARTESIAN_POINT('Ctrl Pts',(5.49999999999963,-12.5141521334422,
12.4978250586149));
#144379=CARTESIAN_POINT('Origin',(7.1,-24.4,10.2));
#144380=CARTESIAN_POINT('',(8.7,-20.8,10.2));
#144381=CARTESIAN_POINT('Origin',(7.1,-20.8,10.2));
#144382=CARTESIAN_POINT('',(8.7,-10.3,10.2));
#144383=CARTESIAN_POINT('',(8.7,-24.4,10.2));
#144384=CARTESIAN_POINT('Origin',(7.1,-10.3,10.2));
#144385=CARTESIAN_POINT('Origin',(11.4999886762478,-10.3,10.1900175708635));
#144386=CARTESIAN_POINT('',(11.5845457335763,-19.4622952671594,9.59600569888119));
#144387=CARTESIAN_POINT('',(11.5845457335763,-10.3,9.59600569888119));
#144388=CARTESIAN_POINT('Ctrl Pts',(11.5845457335763,-19.4622952671594,
9.59600569888118));
#144389=CARTESIAN_POINT('Ctrl Pts',(11.526887976094,-19.4062489738839,9.58779816880506));
#144390=CARTESIAN_POINT('Ctrl Pts',(11.4697992967847,-19.3496507368366,
9.58839463648441));
#144391=CARTESIAN_POINT('Ctrl Pts',(11.4168221802075,-19.2961572437437,
9.59580941378689));
#144392=CARTESIAN_POINT('Ctrl Pts',(11.3465401866327,-19.2251902002209,
9.60564621436044));
#144393=CARTESIAN_POINT('Ctrl Pts',(11.272077928651,-19.1480722446802,9.62936914383039));
#144394=CARTESIAN_POINT('Ctrl Pts',(11.1344342252255,-19.0015084112899,
9.70768993967275));
#144395=CARTESIAN_POINT('Ctrl Pts',(11.0711979486242,-18.9320481917235,
9.76216454706022));
#144396=CARTESIAN_POINT('Ctrl Pts',(10.9874224914153,-18.8381784329961,
9.87316070906256));
#144397=CARTESIAN_POINT('Ctrl Pts',(10.9556614086042,-18.8019424520368,
9.92903001551857));
#144398=CARTESIAN_POINT('Ctrl Pts',(10.9117741849865,-18.7513211403521,
10.0543325101422));
#144399=CARTESIAN_POINT('Ctrl Pts',(10.8998372689763,-18.7372583002031,
10.1239619024751));
#144400=CARTESIAN_POINT('Ctrl Pts',(10.8999902203958,-18.7372583002031,
10.1913788112003));
#144401=CARTESIAN_POINT('Origin',(13.7499999999997,-14.8,14.199999999963));
#144402=CARTESIAN_POINT('',(13.8999999999996,-14.8,11.899999999963));
#144403=CARTESIAN_POINT('Origin',(13.8999999999996,-14.8,14.199999999963));
#144404=CARTESIAN_POINT('',(13.5999999999997,-14.8,12.199999999963));
#144405=CARTESIAN_POINT('',(13.7499999999997,-14.8,12.049999999963));
#144406=CARTESIAN_POINT('Origin',(13.5999999999997,-14.8,14.199999999963));
#144407=CARTESIAN_POINT('Origin',(13.8999999999996,-14.8,14.199999999963));
#144408=CARTESIAN_POINT('',(8.49999999999959,-14.8,12.199999999963));
#144409=CARTESIAN_POINT('',(13.8999999999996,-14.8,12.199999999963));
#144410=CARTESIAN_POINT('Origin',(8.49999999999959,-14.8,14.199999999963));
#144411=CARTESIAN_POINT('Origin',(13.4954867544557,-19.9,8.99159012270411));
#144412=CARTESIAN_POINT('',(13.5220680886962,-10.3,8.59247430909859));
#144413=CARTESIAN_POINT('',(13.8952427952371,-10.3,8.97762202123065));
#144414=CARTESIAN_POINT('Origin',(13.4954867544557,-10.3,8.99159012270412));
#144415=CARTESIAN_POINT('',(13.8952427952371,-15.9,8.97762202123065));
#144416=CARTESIAN_POINT('',(13.8952427952371,-19.9,8.97762202123064));
#144417=CARTESIAN_POINT('',(13.5220680886962,-15.9,8.59247430909859));
#144418=CARTESIAN_POINT('Origin',(13.4954867544557,-15.9,8.99159012270412));
#144419=CARTESIAN_POINT('',(13.5220680886962,-19.9,8.59247430909859));
#144420=CARTESIAN_POINT('Origin',(9.25,-21.1,-3.05000000003699));
#144421=CARTESIAN_POINT('',(0.634274193548384,-10.3,2.68513459542314));
#144422=CARTESIAN_POINT('',(0.634274193548383,-15.9,2.68513459542314));
#144423=CARTESIAN_POINT('',(0.634274193548383,-15.7,2.68513459542314));
#144424=CARTESIAN_POINT('',(4.72983031395648,-10.3,6.26077687460528));
#144425=CARTESIAN_POINT('Origin',(9.25,-10.3,-3.05000000003699));
#144426=CARTESIAN_POINT('',(4.72983031395648,-15.9,6.26077687460528));
#144427=CARTESIAN_POINT('',(4.72983031395648,-15.7,6.26077687460528));
#144428=CARTESIAN_POINT('Origin',(9.25,-15.9,-3.05000000003699));
#144429=CARTESIAN_POINT('Origin',(0.0099462365591374,-15.7,3.10072405886228));
#144430=CARTESIAN_POINT('',(-0.616835877496162,-15.9,2.68884521563242));
#144431=CARTESIAN_POINT('',(-0.616835877496162,-10.3,2.68884521563242));
#144432=CARTESIAN_POINT('',(-0.616835877496162,-15.7,2.68884521563242));
#144433=CARTESIAN_POINT('Origin',(0.0099462365591374,-10.3,3.10072405886228));
#144434=CARTESIAN_POINT('Origin',(0.0099462365591374,-15.9,3.10072405886228));
#144435=CARTESIAN_POINT('Origin',(-5.41858467284464,-21.1,25.4463470699242));
#144436=CARTESIAN_POINT('',(-0.459727007153424,-10.3,16.7624694423079));
#144437=CARTESIAN_POINT('',(-0.459727007153423,-21.1,16.7624694423079));
#144438=CARTESIAN_POINT('Origin',(-5.41858467284464,-10.3,25.4463470699242));
#144439=CARTESIAN_POINT('Origin',(0.748897957688959,-10.3,17.4526448948953));
#144440=CARTESIAN_POINT('',(0.748897957688964,-10.3,17.4526448948953));
#144441=CARTESIAN_POINT('',(0.748897957688964,-10.3,17.4526448948953));
#144442=CARTESIAN_POINT('',(-0.362541436325646,-10.3,16.8179664718101));
#144443=CARTESIAN_POINT('Origin',(0.550543651061315,-10.3,17.8));
#144444=CARTESIAN_POINT('',(0.550543651061315,-10.3,18.2));
#144445=CARTESIAN_POINT('Origin',(0.550543651061315,-10.3,17.8));
#144446=CARTESIAN_POINT('',(0.550543651061315,-10.3,18.2));
#144447=CARTESIAN_POINT('Origin',(8.6,-19.9,-0.741996797474057));
#144448=CARTESIAN_POINT('',(6.1,-20.,-0.741996797474058));
#144449=CARTESIAN_POINT('',(6.09999999999987,-23.,-0.741996797474058));
#144450=CARTESIAN_POINT('',(7.99320388349507,-20.,1.68324514365152));
#144451=CARTESIAN_POINT('Origin',(8.6,-20.,-0.741996797474057));
#144452=CARTESIAN_POINT('',(7.99320388349492,-22.1690497294436,1.68324514365148));
#144453=CARTESIAN_POINT('',(7.99320388349507,-19.9,1.68324514365152));
#144454=CARTESIAN_POINT('',(7.14318637525862,-22.1759507871132,1.28967592783578));
#144455=CARTESIAN_POINT('Ctrl Pts',(7.14318637525862,-22.1759507871132,
1.28967592783578));
#144456=CARTESIAN_POINT('Ctrl Pts',(7.27634231486309,-22.1482114428875,
1.38515557109449));
#144457=CARTESIAN_POINT('Ctrl Pts',(7.41971691376916,-22.1341795264265,
1.46792856779323));
#144458=CARTESIAN_POINT('Ctrl Pts',(7.70527732150551,-22.1341795264265,
1.59720438867895));
#144459=CARTESIAN_POINT('Ctrl Pts',(7.84789476028797,-22.1458682109901,
1.64688876610433));
#144460=CARTESIAN_POINT('Ctrl Pts',(7.99320388349492,-22.1690497294436,
1.68324514365148));
#144461=CARTESIAN_POINT('',(6.10539366127889,-23.,-0.57786509787753));
#144462=CARTESIAN_POINT('Ctrl Pts',(6.10539366127889,-23.,-0.577865097877531));
#144463=CARTESIAN_POINT('Ctrl Pts',(6.11813237646687,-22.890355013293,-0.384251799939226));
#144464=CARTESIAN_POINT('Ctrl Pts',(6.15396251435404,-22.7894964256895,
-0.191486226472621));
#144465=CARTESIAN_POINT('Ctrl Pts',(6.29596367302553,-22.562167115317,0.272007126052555));
#144466=CARTESIAN_POINT('Ctrl Pts',(6.4444684430105,-22.4335682956343,0.56671497320216));
#144467=CARTESIAN_POINT('Ctrl Pts',(6.79236654041548,-22.2678733559761,
0.999597022742));
#144468=CARTESIAN_POINT('Ctrl Pts',(6.96001166618957,-22.2141101536678,
1.15833025953227));
#144469=CARTESIAN_POINT('Ctrl Pts',(7.14318637525862,-22.1759507871132,
1.28967592783578));
#144470=CARTESIAN_POINT('',(6.10539366127889,-23.,-0.57786509787753));
#144471=CARTESIAN_POINT('Origin',(3.34425313716315E-18,-18.2,18.2));
#144472=CARTESIAN_POINT('',(3.1,-18.2,18.2));
#144473=CARTESIAN_POINT('Origin',(3.34425313716343E-18,-18.2,18.2));
#144474=CARTESIAN_POINT('',(3.1,-18.2,16.1));
#144475=CARTESIAN_POINT('',(3.1,-18.2,18.2));
#144476=CARTESIAN_POINT('Origin',(8.48627692340407E-16,-18.2,16.1));
#144477=CARTESIAN_POINT('Origin',(6.1,-22.1,2.59986263839934));
#144478=CARTESIAN_POINT('',(6.1,-20.,-5.32716721908225));
#144479=CARTESIAN_POINT('',(6.09999999999996,-23.,-5.32716721908225));
#144480=CARTESIAN_POINT('',(6.1,-20.,1.07493131918839));
#144481=CARTESIAN_POINT('Origin',(8.6,-21.,-5.32716721908225));
#144482=CARTESIAN_POINT('',(7.74383561643836,-22.1349879358347,-7.67599299983325));
#144483=CARTESIAN_POINT('Ctrl Pts',(7.74383561643836,-22.1349879358347,
-7.67599299983324));
#144484=CARTESIAN_POINT('Ctrl Pts',(7.56929610419344,-22.1414472919843,
-7.61237205564362));
#144485=CARTESIAN_POINT('Ctrl Pts',(7.3994612412714,-22.1582279470408,-7.52800380534636));
#144486=CARTESIAN_POINT('Ctrl Pts',(6.96320155009549,-22.2327613073737,
-7.24588019257465));
#144487=CARTESIAN_POINT('Ctrl Pts',(6.72532955663053,-22.3135747988836,
-7.00860235960015));
#144488=CARTESIAN_POINT('Ctrl Pts',(6.55177992406772,-22.4120688591538,
-6.76062266678474));
#144489=CARTESIAN_POINT('Ctrl Pts',(6.36059256319116,-22.5205728021874,
-6.48744097045821));
#144490=CARTESIAN_POINT('Ctrl Pts',(6.22126616693759,-22.6644734037083,
-6.16555726477482));
#144491=CARTESIAN_POINT('Ctrl Pts',(6.13107715207365,-22.8859742655692,
-5.73441170350023));
#144492=CARTESIAN_POINT('Ctrl Pts',(6.11613067119341,-22.9421215186625,
-5.6292985619738));
#144493=CARTESIAN_POINT('Ctrl Pts',(6.10786135295693,-23.,-5.52527063630252));
#144494=CARTESIAN_POINT('',(7.74383561643836,-20.,-7.67599299983325));
#144495=CARTESIAN_POINT('',(7.74383561643836,-21.,-7.67599299983325));
#144496=CARTESIAN_POINT('Origin',(8.6,-20.,-5.32716721908225));
#144497=CARTESIAN_POINT('Origin',(-5.42954084321747,-21.1,-4.25000000003699));
#144498=CARTESIAN_POINT('',(-5.42954084321747,-20.,-3.65000000003699));
#144499=CARTESIAN_POINT('Origin',(-5.42954084321747,-20.,-4.25000000003699));
#144500=CARTESIAN_POINT('',(-5.42954084321747,-21.1,-3.65000000003699));
#144501=CARTESIAN_POINT('Origin',(9.25,-22.55,-3.05000000003699));
#144502=CARTESIAN_POINT('',(7.5030745174711,-23.,0.548367874220887));
#144503=CARTESIAN_POINT('Origin',(9.25,-23.,-3.05000000003699));
#144504=CARTESIAN_POINT('Origin',(9.25,-22.55,-3.05000000003699));
#144505=CARTESIAN_POINT('',(11.3899837160979,-22.1,-7.4580006460029));
#144506=CARTESIAN_POINT('',(10.9969254825289,-23.,-6.64836787429488));
#144507=CARTESIAN_POINT('',(8.05573019712722,-22.1,-7.8022331212071));
#144508=CARTESIAN_POINT('Origin',(9.25,-22.1,-3.05000000003699));
#144509=CARTESIAN_POINT('Ctrl Pts',(8.05573019725203,-22.0999999999764,
-7.80223312126278));
#144510=CARTESIAN_POINT('Ctrl Pts',(7.95316899134432,-22.1193813623634,
-7.75647475434377));
#144511=CARTESIAN_POINT('Ctrl Pts',(7.84883301855934,-22.1311021932522,
-7.7142653301181));
#144512=CARTESIAN_POINT('Ctrl Pts',(7.74383561643836,-22.1349879358347,
-7.67599299983325));
#144513=CARTESIAN_POINT('Origin',(-10.2709990938499,-21.1,-7.04521722430998));
#144514=CARTESIAN_POINT('Origin',(-10.2709990938499,-20.,-7.04521722430998));
#144515=CARTESIAN_POINT('Origin',(-9.35,-19.7,-3.05000000003699));
#144516=CARTESIAN_POINT('',(-10.9,-19.7,-3.05000000003699));
#144517=CARTESIAN_POINT('Origin',(-9.35,-19.7,-3.05000000003699));
#144518=CARTESIAN_POINT('Origin',(-8.47750127826606,-18.3,10.5062825051013));
#144519=CARTESIAN_POINT('',(-11.5275012782661,-18.3,10.5062825051013));
#144520=CARTESIAN_POINT('Origin',(-8.47750127826606,-18.3,10.5062825051013));
#144521=CARTESIAN_POINT('',(-6.47750127826606,-18.3,10.5062825051013));
#144522=CARTESIAN_POINT('Origin',(-8.47750127826606,-18.3,10.5062825051013));
#144523=CARTESIAN_POINT('Origin',(-9.35,-22.1,-3.05000000003699));
#144524=CARTESIAN_POINT('',(-10.9,-23.2,-3.05000000003699));
#144525=CARTESIAN_POINT('',(-10.9,-22.1,-3.05000000003699));
#144526=CARTESIAN_POINT('Origin',(-9.35,-23.2,-3.05000000003699));
#144527=CARTESIAN_POINT('Origin',(-8.47750127826606,-18.5,10.5062825051013));
#144528=CARTESIAN_POINT('',(-6.47750127826606,-24.4,10.5062825051013));
#144529=CARTESIAN_POINT('',(-6.47750127826606,-18.5,10.5062825051013));
#144530=CARTESIAN_POINT('Origin',(-8.47750127826606,-24.4,10.5062825051013));
#144531=CARTESIAN_POINT('Origin',(-0.100000000022575,-23.2,-0.450000000022577));
#144532=CARTESIAN_POINT('Origin',(-8.47750127826606,-24.4,10.5062825051013));
#144533=CARTESIAN_POINT('Origin',(15.1,-22.55,-15.1));
#144534=CARTESIAN_POINT('',(16.4999999999948,-23.,-5.80993508719201));
#144535=CARTESIAN_POINT('',(16.4999999999931,-22.1,-6.72119489704348));
#144536=CARTESIAN_POINT('Ctrl Pts',(16.4999999999948,-23.0000000000039,
-5.80993508718805));
#144537=CARTESIAN_POINT('Ctrl Pts',(16.4999999999939,-22.5267915597811,
-6.2884866616241));
#144538=CARTESIAN_POINT('Ctrl Pts',(16.4999999999931,-22.1,-6.72119489704349));
#144539=CARTESIAN_POINT('Origin',(15.1,-22.1,-15.1));
#144540=CARTESIAN_POINT('Origin',(15.1,-23.,-15.1));
#144541=CARTESIAN_POINT('Origin',(15.1,-15.7,-15.1));
#144542=CARTESIAN_POINT('Origin',(15.1,-10.3,-15.1));
#144543=CARTESIAN_POINT('Origin',(15.1,-15.9,-15.1));
#144544=CARTESIAN_POINT('Origin',(8.49999999999959,-14.8,14.199999999963));
#144545=CARTESIAN_POINT('',(8.49999999999962,-14.8,12.549999999963));
#144546=CARTESIAN_POINT('Origin',(8.49999999999959,-14.8,14.199999999963));
#144547=CARTESIAN_POINT('',(8.49999999999962,-14.8,12.549999999963));
#144548=CARTESIAN_POINT('Origin',(8.49999999999959,-14.8,14.199999999963));
#144549=CARTESIAN_POINT('Origin',(7.25435078580463E-16,-18.2,15.1));
#144550=CARTESIAN_POINT('',(3.625,-18.2,15.1));
#144551=CARTESIAN_POINT('Origin',(-2.57959738503056E-16,-18.2,6.59999999999999));
#144552=CARTESIAN_POINT('',(2.1,-18.2,6.59999999999999));
#144553=CARTESIAN_POINT('Origin',(-1.98514478612865E-16,-18.2,6.59999999999999));
#144554=CARTESIAN_POINT('',(1.2,-18.2,6.59999999999999));
#144555=CARTESIAN_POINT('Origin',(1.14718080875314E-15,-18.2,6.59999999999999));
#144556=CARTESIAN_POINT('Origin',(1.12870191668915E-15,-18.2,6.44999999999999));
#144557=CARTESIAN_POINT('',(-1.,-18.2,6.29999999999999));
#144558=CARTESIAN_POINT('',(1.,-18.2,6.29999999999999));
#144559=CARTESIAN_POINT('Origin',(1.11022302462516E-15,-18.2,6.29999999999999));
#144560=CARTESIAN_POINT('',(1.1,-18.2,6.44999999999999));
#144561=CARTESIAN_POINT('Origin',(1.11022302462516E-15,-18.2,6.29999999999999));
#144562=CARTESIAN_POINT('Origin',(7.1,-19.3686291501015,10.2));
#144563=CARTESIAN_POINT('',(5.32995029238257,-17.7372583002031,12.369544660191));
#144564=CARTESIAN_POINT('Origin',(7.1,-17.7372583002031,10.2));
#144565=CARTESIAN_POINT('Ctrl Pts',(5.32295533692169,-18.7372583002029,
13.5588855689683));
#144566=CARTESIAN_POINT('Ctrl Pts',(5.34297156764967,-18.5389449337303,
13.3451179243545));
#144567=CARTESIAN_POINT('Ctrl Pts',(5.350772928081,-18.3486971007653,13.1310218147186));
#144568=CARTESIAN_POINT('Ctrl Pts',(5.34926297347848,-18.0331996694862,
12.755024908149));
#144569=CARTESIAN_POINT('Ctrl Pts',(5.34159640421336,-17.8714005164436,
12.5521693415744));
#144570=CARTESIAN_POINT('Ctrl Pts',(5.32995029238257,-17.7372583002031,
12.369544660191));
#144571=CARTESIAN_POINT('Origin',(7.1,-19.3686291501015,10.2));
#144572=CARTESIAN_POINT('',(4.89412386071569,-17.7372583002031,8.47543905351648));
#144573=CARTESIAN_POINT('Ctrl Pts',(4.89412386071568,-17.7372583002031,
8.47543905351647));
#144574=CARTESIAN_POINT('Ctrl Pts',(4.93436452953714,-17.7372583002031,
8.42396744193725));
#144575=CARTESIAN_POINT('Ctrl Pts',(4.9669696527347,-17.7511306117407,8.36381545146218));
#144576=CARTESIAN_POINT('Ctrl Pts',(5.00922761570301,-17.8008285638029,
8.24239426982826));
#144577=CARTESIAN_POINT('Ctrl Pts',(5.01915235870633,-17.8362967472096,
8.18107382133259));
#144578=CARTESIAN_POINT('Ctrl Pts',(5.0239204625628,-17.9281186662182,8.04624688172536));
#144579=CARTESIAN_POINT('Ctrl Pts',(5.01003668161719,-17.9961660277199,
7.96621461494606));
#144580=CARTESIAN_POINT('Ctrl Pts',(4.95550714282828,-18.139449903377,7.82176351540889));
#144581=CARTESIAN_POINT('Ctrl Pts',(4.91473826352193,-18.2147014671034,
7.75740612148749));
#144582=CARTESIAN_POINT('Ctrl Pts',(4.86860064468514,-18.2838984063394,
7.70583542702161));
#144583=CARTESIAN_POINT('Ctrl Pts',(4.81723293471555,-18.3609394066135,
7.64841875613479));
#144584=CARTESIAN_POINT('Ctrl Pts',(4.75012706774148,-18.444132170492,7.59666483773002));
#144585=CARTESIAN_POINT('Ctrl Pts',(4.67225419943427,-18.5232262216458,
7.56083038410712));
#144586=CARTESIAN_POINT('',(4.30011215770157,-17.7372583002031,10.1749386642522));
#144587=CARTESIAN_POINT('Ctrl Pts',(4.30011215770158,-17.7372583002031,
10.1749386642522));
#144588=CARTESIAN_POINT('Ctrl Pts',(4.19159461984128,-17.8468421420048,
10.0553192575359));
#144589=CARTESIAN_POINT('Ctrl Pts',(4.08369135164002,-17.9632436979253,
9.9388527734317));
#144590=CARTESIAN_POINT('Ctrl Pts',(3.78934767167766,-18.2915555175059,
9.63507652193826));
#144591=CARTESIAN_POINT('Ctrl Pts',(3.60197212932834,-18.5118359362721,
9.45659171009935));
#144592=CARTESIAN_POINT('Ctrl Pts',(3.40807692379815,-18.7372583002031,
9.30016445979934));
#144593=CARTESIAN_POINT('Origin',(7.1,-17.7372583002031,10.2));
#144594=CARTESIAN_POINT('Origin',(7.1,-19.3686291501015,10.2));
#144595=CARTESIAN_POINT('',(10.6037224484923,-18.5232262216426,9.43639346681366));
#144596=CARTESIAN_POINT('Ctrl Pts',(10.6037224531807,-18.5232262260405,
9.4363934676728));
#144597=CARTESIAN_POINT('Ctrl Pts',(10.5194042997935,-18.4441321735666,
9.42094222224999));
#144598=CARTESIAN_POINT('Ctrl Pts',(10.4347432389821,-18.3609394080404,
9.42470659861854));
#144599=CARTESIAN_POINT('Ctrl Pts',(10.3597035517405,-18.2838984063394,
9.4421525517822));
#144600=CARTESIAN_POINT('Ctrl Pts',(10.2923041596806,-18.2147014671034,
9.4578222151345));
#144601=CARTESIAN_POINT('Ctrl Pts',(10.2219460850893,-18.139449903377,9.4870406513017));
#144602=CARTESIAN_POINT('Ctrl Pts',(10.0942809753824,-17.9961660277199,
9.57388079479276));
#144603=CARTESIAN_POINT('Ctrl Pts',(10.0369085244781,-17.9281186662182,
9.63138144675786));
#144604=CARTESIAN_POINT('Ctrl Pts',(9.96329423056347,-17.8362967472096,
9.74443884010165));
#144605=CARTESIAN_POINT('Ctrl Pts',(9.93615995461258,-17.8008285638029,
9.80031753904868));
#144606=CARTESIAN_POINT('Ctrl Pts',(9.90092737860809,-17.7511306117407,
9.92396018691622));
#144607=CARTESIAN_POINT('Ctrl Pts',(9.89302208195365,-17.7372583002031,
9.9919223992231));
#144608=CARTESIAN_POINT('Ctrl Pts',(9.89635480722185,-17.7372583002031,
10.0571721591311));
#144609=CARTESIAN_POINT('Ctrl Pts',(10.6037224484923,-18.5232262216426,
9.43639346681366));
#144610=CARTESIAN_POINT('Ctrl Pts',(10.9243634589968,-18.8240012734338,
9.4951507156968));
#144611=CARTESIAN_POINT('Ctrl Pts',(11.2507529726933,-19.1378316080336,
9.54849059868016));
#144612=CARTESIAN_POINT('Ctrl Pts',(11.5845457335763,-19.4622952671594,
9.59600569888119));
#144613=CARTESIAN_POINT('Origin',(7.1,-20.8,10.2));
#144614=CARTESIAN_POINT('Origin',(3.56597033699713E-16,-18.2,11.6));
#144615=CARTESIAN_POINT('',(2.1,-18.2,11.6));
#144616=CARTESIAN_POINT('Origin',(1.04273619012177E-16,-18.2,11.6));
#144617=CARTESIAN_POINT('',(4.4846606338756,-15.2827548956307,11.2));
#144618=CARTESIAN_POINT('Ctrl Pts',(4.48466063387559,-15.2827548956307,
11.2));
#144619=CARTESIAN_POINT('Ctrl Pts',(4.54827264874599,-15.3805452042008,
11.366367006649));
#144620=CARTESIAN_POINT('Ctrl Pts',(4.62296913595049,-15.5030834282367,
11.5130892578383));
#144621=CARTESIAN_POINT('Ctrl Pts',(4.80528294110503,-15.8368475963683,
11.8187844172933));
#144622=CARTESIAN_POINT('Ctrl Pts',(4.93705801232801,-16.1205392330633,
11.9835651254983));
#144623=CARTESIAN_POINT('Ctrl Pts',(5.12599278618915,-16.6428387391747,
12.19077642575));
#144624=CARTESIAN_POINT('Ctrl Pts',(5.21110280172174,-16.9473520403291,
12.2682274318723));
#144625=CARTESIAN_POINT('Ctrl Pts',(5.29517632124998,-17.4195096846515,
12.3410243821726));
#144626=CARTESIAN_POINT('Ctrl Pts',(5.3162453081633,-17.5794015851531,12.3583632801737));
#144627=CARTESIAN_POINT('Ctrl Pts',(5.32995029238257,-17.7372583002031,
12.369544660191));
#144628=CARTESIAN_POINT('Origin',(1.54557770421648E-17,-18.2,11.2));
#144629=CARTESIAN_POINT('Origin',(7.25077700072151E-16,-18.2,14.3958530281318));
#144630=CARTESIAN_POINT('Origin',(1.54557770421648E-17,-18.2,11.2));
#144631=CARTESIAN_POINT('Origin',(3.56597033699713E-16,-18.2,11.6));
#144632=CARTESIAN_POINT('Origin',(8.45923926665497E-17,-18.2,9.14999999999999));
#144633=CARTESIAN_POINT('Origin',(-2.42923399597872E-16,-18.2,6.19999999999999));
#144634=CARTESIAN_POINT('Origin',(-2.42923399597872E-16,-18.2,6.19999999999999));
#144635=CARTESIAN_POINT('Origin',(1.17797896219313E-15,-18.2,5.64999999999999));
#144636=CARTESIAN_POINT('Ctrl Pts',(2.3,-20.5664319132398,6.19999999999999));
#144637=CARTESIAN_POINT('Ctrl Pts',(2.27958604839685,-20.5471301887928,
6.17193081654566));
#144638=CARTESIAN_POINT('Ctrl Pts',(2.2595024242038,-20.5281396051547,6.14431583328021));
#144639=CARTESIAN_POINT('Origin',(1.17797896219313E-15,-18.2,5.64999999999999));
#144640=CARTESIAN_POINT('Origin',(1.11022302462516E-15,-18.2,5.09999999999999));
#144641=CARTESIAN_POINT('Origin',(1.11022302462516E-15,-18.2,-19.1));
#144642=CARTESIAN_POINT('Origin',(-5.536176502776,-10.3,16.5874694585077));
#144643=CARTESIAN_POINT('',(-4.16287082888301,-15.6648219347062,15.302374052251));
#144644=CARTESIAN_POINT('',(-4.16287082888302,-10.3,15.302374052251));
#144645=CARTESIAN_POINT('',(-4.16287082888302,-10.3,15.302374052251));
#144646=CARTESIAN_POINT('Origin',(4.4806864735526,-18.2,7.21401033669983));
#144647=CARTESIAN_POINT('',(-1.73395719574401,-10.3,13.0294745722009));
#144648=CARTESIAN_POINT('Origin',(-3.65042002992564,-10.3,15.85));
#144649=CARTESIAN_POINT('',(-4.18196358468572,-17.1622932649853,16.3791138340594));
#144650=CARTESIAN_POINT('Ctrl Pts',(-4.18187625800635,-17.1623114267662,
16.3792076522946));
#144651=CARTESIAN_POINT('Ctrl Pts',(-4.19394811587314,-17.1587260110058,
16.3670919708574));
#144652=CARTESIAN_POINT('Ctrl Pts',(-4.21680216810472,-17.1442366946548,
16.3422127058649));
#144653=CARTESIAN_POINT('Ctrl Pts',(-4.24674448939413,-17.1067250534971,
16.305735840826));
#144654=CARTESIAN_POINT('Ctrl Pts',(-4.28111161194148,-17.0288513854137,
16.2575852802216));
#144655=CARTESIAN_POINT('Ctrl Pts',(-4.3164940870397,-16.8690652334165,
16.197184839744));
#144656=CARTESIAN_POINT('Ctrl Pts',(-4.33114148592674,-16.682242226022,
16.164479258454));
#144657=CARTESIAN_POINT('Ctrl Pts',(-4.33276019641122,-16.4943822165373,
16.1612288892188));
#144658=CARTESIAN_POINT('Ctrl Pts',(-4.32419391032616,-16.3065945433838,
16.1795042852215));
#144659=CARTESIAN_POINT('Ctrl Pts',(-4.29214178574177,-16.075454478799,
16.2446281088384));
#144660=CARTESIAN_POINT('Ctrl Pts',(-4.15704520376224,-15.7158195120752,
16.4317690537223));
#144661=CARTESIAN_POINT('Ctrl Pts',(-3.89740878663184,-15.4677167334541,
16.6));
#144662=CARTESIAN_POINT('Ctrl Pts',(-3.65042002992564,-15.3215437309242,
16.6));
#144663=CARTESIAN_POINT('Ctrl Pts',(-4.16287082888297,-15.6648219347062,
15.302374052251));
#144664=CARTESIAN_POINT('Ctrl Pts',(-4.25484771496768,-15.9027259587502,
15.3884430724526));
#144665=CARTESIAN_POINT('Ctrl Pts',(-4.3183020446404,-16.1518334302826,
15.4924169890107));
#144666=CARTESIAN_POINT('Ctrl Pts',(-4.39472128107487,-16.6187968527348,
15.7017962064845));
#144667=CARTESIAN_POINT('Ctrl Pts',(-4.41570619245039,-16.912665600934,
15.8343457381435));
#144668=CARTESIAN_POINT('Ctrl Pts',(-4.38320717254138,-17.174369879551,
16.0121523282015));
#144669=CARTESIAN_POINT('Ctrl Pts',(-4.37587758335711,-17.2167793786262,
16.0437248374513));
#144670=CARTESIAN_POINT('Ctrl Pts',(-4.35929935835897,-17.2687407400561,
16.0956008187188));
#144671=CARTESIAN_POINT('Ctrl Pts',(-4.35285886199348,-17.2840306332906,
16.1136122575154));
#144672=CARTESIAN_POINT('Ctrl Pts',(-4.33744597327384,-17.3076885865545,
16.1515317596741));
#144673=CARTESIAN_POINT('Ctrl Pts',(-4.32848093244943,-17.3160588866582,
16.1714414131769));
#144674=CARTESIAN_POINT('Ctrl Pts',(-4.31735930687918,-17.3183300903997,
16.1930626777379));
#144675=CARTESIAN_POINT('Ctrl Pts',(-4.31061548133341,-17.3197072813252,
16.2061731745225));
#144676=CARTESIAN_POINT('Ctrl Pts',(-4.30342160786703,-17.3186208202269,
16.2191885665456));
#144677=CARTESIAN_POINT('Ctrl Pts',(-4.28859108025688,-17.3118976847781,
16.2442727939903));
#144678=CARTESIAN_POINT('Ctrl Pts',(-4.28095308507075,-17.3062247464623,
16.2563311027636));
#144679=CARTESIAN_POINT('Ctrl Pts',(-4.25810464024748,-17.2846822200441,
16.2904427701345));
#144680=CARTESIAN_POINT('Ctrl Pts',(-4.24290182089397,-17.2638318647245,
16.3103432232216));
#144681=CARTESIAN_POINT('Ctrl Pts',(-4.2135428425112,-17.2188943338578,
16.3459997875122));
#144682=CARTESIAN_POINT('Ctrl Pts',(-4.19780490989408,-17.1914425505379,
16.3631997645882));
#144683=CARTESIAN_POINT('Ctrl Pts',(-4.18196358468572,-17.1622932649853,
16.3791138340594));
#144684=CARTESIAN_POINT('Origin',(-3.65042002992564,-10.3,15.85));
#144685=CARTESIAN_POINT('Origin',(11.2999999999996,-10.3,12.6));
#144686=CARTESIAN_POINT('',(11.7999999999996,-11.8066740905561,12.6));
#144687=CARTESIAN_POINT('',(11.8999999999998,-11.8066740905561,12.6));
#144688=CARTESIAN_POINT('',(13.8999999999996,-11.8066740905561,12.6000000000001));
#144689=CARTESIAN_POINT('',(11.7999999999996,-10.3,12.6));
#144690=CARTESIAN_POINT('',(11.7999999999996,-10.3,12.6));
#144691=CARTESIAN_POINT('',(11.8999999999996,-10.3,12.6));
#144692=CARTESIAN_POINT('',(11.2999999999996,-10.3,12.6));
#144693=CARTESIAN_POINT('',(11.8999999999996,-10.3,12.6));
#144694=CARTESIAN_POINT('Origin',(11.2999999999996,-10.3,16.6));
#144695=CARTESIAN_POINT('',(11.2999999999996,-10.3,16.2));
#144696=CARTESIAN_POINT('',(11.2999999999996,-11.8066740906056,16.2));
#144697=CARTESIAN_POINT('',(11.2999999999996,-10.3,16.2));
#144698=CARTESIAN_POINT('',(11.2999999999996,-10.3,13.1));
#144699=CARTESIAN_POINT('',(11.2999999999996,-10.3,16.6));
#144700=CARTESIAN_POINT('',(11.2999999999996,-11.3721726997876,13.1));
#144701=CARTESIAN_POINT('',(11.2999999999996,-10.3,13.1));
#144702=CARTESIAN_POINT('Origin',(11.2999999999996,-14.8,14.199999999963));
#144703=CARTESIAN_POINT('Origin',(11.7999999999996,-10.3,13.1));
#144704=CARTESIAN_POINT('Ctrl Pts',(11.2999999999996,-11.3721726997876,
13.1));
#144705=CARTESIAN_POINT('Ctrl Pts',(11.2999999999996,-11.4587530856937,
12.950109792686));
#144706=CARTESIAN_POINT('Ctrl Pts',(11.4173949896311,-11.6750919324497,
12.702604689212));
#144707=CARTESIAN_POINT('Ctrl Pts',(11.6819358373965,-11.8066740905561,
12.6));
#144708=CARTESIAN_POINT('Ctrl Pts',(11.7999999999996,-11.8066740905561,
12.6));
#144709=CARTESIAN_POINT('Origin',(11.7999999999996,-10.3,13.1));
#144710=CARTESIAN_POINT('Origin',(11.8999999999997,-14.8,14.199999999963));
#144711=CARTESIAN_POINT('',(11.8999999999998,-12.1392658582721,12.4222222222182));
#144712=CARTESIAN_POINT('Origin',(11.8999999999998,-11.8066740905561,12.2000000000001));
#144713=CARTESIAN_POINT('Origin',(11.8999999999997,-14.8,14.199999999963));
#144714=CARTESIAN_POINT('Origin',(13.8999999999996,-14.8,14.199999999963));
#144715=CARTESIAN_POINT('',(10.8999999999996,-11.7530423998112,13.2222222222181));
#144716=CARTESIAN_POINT('',(10.8999999999996,-12.1392658583161,15.9777777777737));
#144717=CARTESIAN_POINT('Origin',(10.8999999999996,-14.8,14.199999999963));
#144718=CARTESIAN_POINT('',(11.7999999999996,-12.1392658582721,12.4222222222181));
#144719=CARTESIAN_POINT('Ctrl Pts',(11.7999999999996,-12.1392658582721,
12.4222222222181));
#144720=CARTESIAN_POINT('Ctrl Pts',(11.587484507314,-12.1392658582721,12.4222222222181));
#144721=CARTESIAN_POINT('Ctrl Pts',(11.1113109813363,-12.0223039399553,
12.5863897249574));
#144722=CARTESIAN_POINT('Ctrl Pts',(10.8999999999996,-11.8300027428388,
12.9823978905158));
#144723=CARTESIAN_POINT('Ctrl Pts',(10.8999999999996,-11.7530423998112,
13.2222222222181));
#144724=CARTESIAN_POINT('',(13.8999999999996,-12.1392658582721,12.4222222222182));
#144725=CARTESIAN_POINT('Ctrl Pts',(8.72186658824407,-12.1000000000251,
12.4824435961918));
#144726=CARTESIAN_POINT('Ctrl Pts',(8.70882337879446,-12.0731544895491,
12.5246447594989));
#144727=CARTESIAN_POINT('Ctrl Pts',(8.69229019349259,-12.0478221085961,
12.5666605881537));
#144728=CARTESIAN_POINT('Ctrl Pts',(8.6341741057584,-11.9787672316304,12.6870768342024));
#144729=CARTESIAN_POINT('Ctrl Pts',(8.57970250797918,-11.9362210326303,
12.7697041881164));
#144730=CARTESIAN_POINT('Ctrl Pts',(8.44647017591476,-11.86550775675,12.9210429686623));
#144731=CARTESIAN_POINT('Ctrl Pts',(8.36788263061954,-11.8370629769507,
12.9897769287426));
#144732=CARTESIAN_POINT('Ctrl Pts',(8.13014000727059,-11.770919657986,13.1608510380605));
#144733=CARTESIAN_POINT('Ctrl Pts',(7.93448701836192,-11.7429091928131,
13.2523731799822));
#144734=CARTESIAN_POINT('Ctrl Pts',(7.70170765487302,-11.7236773606694,
13.3189227526333));
#144735=CARTESIAN_POINT('Ctrl Pts',(7.67591374269582,-11.7217258906158,
13.3257732799122));
#144736=CARTESIAN_POINT('Ctrl Pts',(7.64999999999965,-11.7199299841877,
13.3321470759639));
#144737=CARTESIAN_POINT('',(13.8999999999996,-12.1392658583161,15.9777777777737));
#144738=CARTESIAN_POINT('Origin',(13.8999999999996,-11.8066740906056,16.2));
#144739=CARTESIAN_POINT('Origin',(10.8999999999996,-11.8066740906056,16.2));
#144740=CARTESIAN_POINT('Origin',(11.8999999999998,-11.8066740905561,12.2000000000001));
#144741=CARTESIAN_POINT('Origin',(11.8999999999997,-11.8066740905561,12.2));
#144742=CARTESIAN_POINT('Origin',(11.8999999999998,-11.8066740905561,12.2000000000001));
#144743=CARTESIAN_POINT('Origin',(11.8999999999997,-10.3,12.2));
#144744=CARTESIAN_POINT('Origin',(11.8999999999997,-10.3,12.2));
#144745=CARTESIAN_POINT('Origin',(10.8999999999996,-11.8066740906056,16.2));
#144746=CARTESIAN_POINT('Origin',(10.8999999999996,-11.8066740906056,16.2));
#144747=CARTESIAN_POINT('Origin',(10.8999999999996,-11.8066740906056,16.2));
#144748=CARTESIAN_POINT('Origin',(13.8999999999996,-11.8066740905561,12.2000000000001));
#144749=CARTESIAN_POINT('Origin',(11.7999999999996,-11.8066740905561,12.2));
#144750=CARTESIAN_POINT('Ctrl Pts',(11.7999999999996,-11.8066740905561,
12.6));
#144751=CARTESIAN_POINT('Ctrl Pts',(11.6819358373965,-11.8066740905561,
12.6));
#144752=CARTESIAN_POINT('Ctrl Pts',(11.4173949896311,-11.6750919324497,
12.702604689212));
#144753=CARTESIAN_POINT('Ctrl Pts',(11.2999999999996,-11.4587530856937,
12.950109792686));
#144754=CARTESIAN_POINT('Ctrl Pts',(11.2999999999996,-11.3721726997876,
13.1));
#144755=CARTESIAN_POINT('Ctrl Pts',(11.7999999999996,-11.8721251143289,
12.6));
#144756=CARTESIAN_POINT('Ctrl Pts',(11.6716366670667,-11.8721251143289,
12.6));
#144757=CARTESIAN_POINT('Ctrl Pts',(11.3853622217568,-11.7474710537238,
12.7239006626482));
#144758=CARTESIAN_POINT('Ctrl Pts',(11.2901909346614,-11.5500696929581,
12.9883381875986));
#144759=CARTESIAN_POINT('Ctrl Pts',(11.2999999999996,-11.471884154085,13.1319977029522));
#144760=CARTESIAN_POINT('Ctrl Pts',(11.7999999999996,-12.0029536410931,
12.5672054150641));
#144761=CARTESIAN_POINT('Ctrl Pts',(11.6432129484504,-12.0029536410931,
12.5672054150641));
#144762=CARTESIAN_POINT('Ctrl Pts',(11.2939898772465,-11.8923755833045,
12.7224346897746));
#144763=CARTESIAN_POINT('Ctrl Pts',(11.1953517025113,-11.732454125104,13.0376950947528));
#144764=CARTESIAN_POINT('Ctrl Pts',(11.2132967619966,-11.670485809188,13.1957295661626));
#144765=CARTESIAN_POINT('Ctrl Pts',(11.7999999999996,-12.102904178399,12.4766434014566));
#144766=CARTESIAN_POINT('Ctrl Pts',(11.6060763489285,-12.1029041783991,
12.4766434014566));
#144767=CARTESIAN_POINT('Ctrl Pts',(11.172110277341,-11.9919204949165,12.6401816400886));
#144768=CARTESIAN_POINT('Ctrl Pts',(10.9985531508785,-11.8206425682432,
13.0109145504288));
#144769=CARTESIAN_POINT('Ctrl Pts',(11.0047197551193,-11.7530423998112,
13.2222222222181));
#144770=CARTESIAN_POINT('Ctrl Pts',(11.7999999999996,-12.1392658582721,
12.4222222222181));
#144771=CARTESIAN_POINT('Ctrl Pts',(11.587484507314,-12.1392658582721,12.4222222222181));
#144772=CARTESIAN_POINT('Ctrl Pts',(11.1113109813363,-12.0223039399553,
12.5863897249574));
#144773=CARTESIAN_POINT('Ctrl Pts',(10.8999999999996,-11.8300027428388,
12.9823978905158));
#144774=CARTESIAN_POINT('Ctrl Pts',(10.8999999999996,-11.7530423998112,
13.2222222222181));
#144775=CARTESIAN_POINT('Origin',(10.8999999999996,-11.3721726997876,13.1));
#144776=CARTESIAN_POINT('Origin',(10.8999999999996,-14.8,14.199999999963));
#144777=CARTESIAN_POINT('Origin',(10.8999999999996,-10.3,16.2));
#144778=CARTESIAN_POINT('Origin',(10.8999999999996,-10.3,16.2));
#144779=CARTESIAN_POINT('Origin',(7.1,-24.4,10.2));
#144780=CARTESIAN_POINT('',(4.89412386071569,-12.1,8.47543905351648));
#144781=CARTESIAN_POINT('',(4.89412386071569,-10.3,8.47543905351648));
#144782=CARTESIAN_POINT('Ctrl Pts',(4.30011215770157,-17.7372583002031,
10.1749386642522));
#144783=CARTESIAN_POINT('Ctrl Pts',(4.30001128733287,-17.6309935487308,
10.1862080443775));
#144784=CARTESIAN_POINT('Ctrl Pts',(4.29993438568727,-17.5236929545511,
10.2015325229438));
#144785=CARTESIAN_POINT('Ctrl Pts',(4.30043239221638,-17.1514858680764,
10.2686927199916));
#144786=CARTESIAN_POINT('Ctrl Pts',(4.30231487297464,-16.8903956938801,
10.3420198077238));
#144787=CARTESIAN_POINT('Ctrl Pts',(4.31743469546803,-16.3800007039129,
10.5281842790581));
#144788=CARTESIAN_POINT('Ctrl Pts',(4.33744031191061,-16.0600796813261,
10.6822846029848));
#144789=CARTESIAN_POINT('Ctrl Pts',(4.39372574524066,-15.6586384458731,
10.9243170138561));
#144790=CARTESIAN_POINT('Ctrl Pts',(4.42716844435502,-15.4866311493459,
11.0416565744492));
#144791=CARTESIAN_POINT('Ctrl Pts',(4.47109045903957,-15.3281474321327,
11.1639384262309));
#144792=CARTESIAN_POINT('Ctrl Pts',(4.47769342258432,-15.3054612836516,
11.1817783780378));
#144793=CARTESIAN_POINT('Ctrl Pts',(4.4846606338756,-15.2827548956307,11.2));
#144794=CARTESIAN_POINT('Origin',(7.1,-12.1,10.2));
#144795=CARTESIAN_POINT('Origin',(4.42143611658333,-10.3,8.10589027927001));
#144796=CARTESIAN_POINT('Ctrl Pts',(4.67225419943745,-11.3140320785605,
7.56083038410858));
#144797=CARTESIAN_POINT('Ctrl Pts',(4.75012706774333,-11.3931261297133,
7.59666483773142));
#144798=CARTESIAN_POINT('Ctrl Pts',(4.81723293471625,-11.4763188935906,
7.64841875613557));
#144799=CARTESIAN_POINT('Ctrl Pts',(4.86860064468514,-11.5533598938637,
7.70583542702161));
#144800=CARTESIAN_POINT('Ctrl Pts',(4.91473826352193,-11.6225568330996,
7.75740612148749));
#144801=CARTESIAN_POINT('Ctrl Pts',(4.95550714282828,-11.6978083968261,
7.82176351540889));
#144802=CARTESIAN_POINT('Ctrl Pts',(5.01003668161719,-11.8410922724832,
7.96621461494606));
#144803=CARTESIAN_POINT('Ctrl Pts',(5.0239204625628,-11.9091396339848,8.04624688172536));
#144804=CARTESIAN_POINT('Ctrl Pts',(5.01915235870633,-12.0009615529934,
8.18107382133259));
#144805=CARTESIAN_POINT('Ctrl Pts',(5.00922761570301,-12.0364297364002,
8.24239426982826));
#144806=CARTESIAN_POINT('Ctrl Pts',(4.9669696527347,-12.0861276884624,8.36381545146218));
#144807=CARTESIAN_POINT('Ctrl Pts',(4.93436452953714,-12.1,8.42396744193725));
#144808=CARTESIAN_POINT('Ctrl Pts',(4.89412386071568,-12.1,8.47543905351647));
#144809=CARTESIAN_POINT('Origin',(15.1,-10.3,-15.1000000000002));
#144810=CARTESIAN_POINT('',(11.7798591918362,-10.3,9.6230212796182));
#144811=CARTESIAN_POINT('',(11.7798591918362,-10.3,9.6230212796182));
#144812=CARTESIAN_POINT('Origin',(15.1,-10.3,-15.1000000000002));
#144813=CARTESIAN_POINT('',(10.6037224484923,-11.3140320785605,9.43639346681366));
#144814=CARTESIAN_POINT('Ctrl Pts',(10.6037224484923,-11.3140320785605,
9.43639346681366));
#144815=CARTESIAN_POINT('Ctrl Pts',(10.608707598078,-11.309355793944,9.43730699211245));
#144816=CARTESIAN_POINT('Ctrl Pts',(10.6136918678395,-11.3046784029656,
9.43821878587495));
#144817=CARTESIAN_POINT('Ctrl Pts',(10.618675187344,-11.3,9.43912883747022));
#144818=CARTESIAN_POINT('Ctrl Pts',(10.8716162365519,-11.0625357648361,
9.48532081956795));
#144819=CARTESIAN_POINT('Ctrl Pts',(11.1281188708098,-10.8169580561747,
9.52813260756565));
#144820=CARTESIAN_POINT('Ctrl Pts',(11.3890749660464,-10.5645232201992,
9.56739044915099));
#144821=CARTESIAN_POINT('',(10.6037224484923,-10.3,9.43639346681366));
#144822=CARTESIAN_POINT('Origin',(7.1,-11.7,10.2));
#144823=CARTESIAN_POINT('Ctrl Pts',(9.89635480722185,-12.1,10.0571721591311));
#144824=CARTESIAN_POINT('Ctrl Pts',(9.89302208195365,-12.1,9.99192239922311));
#144825=CARTESIAN_POINT('Ctrl Pts',(9.90092737860809,-12.0861276884624,
9.92396018691622));
#144826=CARTESIAN_POINT('Ctrl Pts',(9.93615995461258,-12.0364297364002,
9.80031753904868));
#144827=CARTESIAN_POINT('Ctrl Pts',(9.96329423056347,-12.0009615529934,
9.74443884010165));
#144828=CARTESIAN_POINT('Ctrl Pts',(10.0369085244781,-11.9091396339848,
9.63138144675786));
#144829=CARTESIAN_POINT('Ctrl Pts',(10.0942809753824,-11.8410922724832,
9.57388079479276));
#144830=CARTESIAN_POINT('Ctrl Pts',(10.2219460850893,-11.6978083968261,
9.48704065130171));
#144831=CARTESIAN_POINT('Ctrl Pts',(10.2923041596806,-11.6225568330996,
9.4578222151345));
#144832=CARTESIAN_POINT('Ctrl Pts',(10.3597035517405,-11.5533598938637,
9.4421525517822));
#144833=CARTESIAN_POINT('Ctrl Pts',(10.4347432375913,-11.4763188935906,
9.4247065989419));
#144834=CARTESIAN_POINT('Ctrl Pts',(10.5194042966525,-11.3931261297133,
9.42094222236673));
#144835=CARTESIAN_POINT('Ctrl Pts',(10.6037224484923,-11.3140320785605,
9.43639346681366));
#144836=CARTESIAN_POINT('Origin',(10.4955736944837,-10.3,10.0265661932306));
#144837=CARTESIAN_POINT('Ctrl Pts',(-4.15558608030974,-17.0949638327396,
16.3958525879769));
#144838=CARTESIAN_POINT('Ctrl Pts',(-4.15558499113943,-17.0949600091324,
16.3958530281318));
#144839=CARTESIAN_POINT('Ctrl Pts',(-4.15225602908945,-17.082431601768,
16.3958530281318));
#144840=CARTESIAN_POINT('Ctrl Pts',(-4.14264067399083,-17.0470960648441,
16.3958530281318));
#144841=CARTESIAN_POINT('Ctrl Pts',(-4.12242181413037,-16.9757326797749,
16.3958530281318));
#144842=CARTESIAN_POINT('Ctrl Pts',(-4.07716739275611,-16.8287774262104,
16.3958530281318));
#144843=CARTESIAN_POINT('Ctrl Pts',(-4.0172093385339,-16.6621227828839,
16.3958530281318));
#144844=CARTESIAN_POINT('Ctrl Pts',(-3.9509934453542,-16.5015111868501,
16.3958530281318));
#144845=CARTESIAN_POINT('Ctrl Pts',(-3.88102031079464,-16.3453037878245,
16.3958530281318));
#144846=CARTESIAN_POINT('Ctrl Pts',(-3.7880821209169,-16.1604212714353,
16.3958530281318));
#144847=CARTESIAN_POINT('Ctrl Pts',(-3.62588443732701,-15.8785354637891,
16.3958530281318));
#144848=CARTESIAN_POINT('Ctrl Pts',(-3.48316325575844,-15.6727047931632,
16.3958530281318));
#144849=CARTESIAN_POINT('Ctrl Pts',(-3.37654926102705,-15.5374983403089,
16.3958530281318));
#144850=CARTESIAN_POINT('Ctrl Pts',(-4.15864956755341,-17.106484576438,
16.3958530281318));
#144851=CARTESIAN_POINT('Ctrl Pts',(-4.16166551294798,-17.1061109850393,
16.3930613132255));
#144852=CARTESIAN_POINT('Ctrl Pts',(-4.1640449424804,-17.0929074595252,
16.3888332106743));
#144853=CARTESIAN_POINT('Ctrl Pts',(-4.16285653706035,-17.0565722710498,
16.3842705686255));
#144854=CARTESIAN_POINT('Ctrl Pts',(-4.1546283879313,-16.9836856368366,
16.3802789513044));
#144855=CARTESIAN_POINT('Ctrl Pts',(-4.12819280007378,-16.8338876916016,
16.3795050583179));
#144856=CARTESIAN_POINT('Ctrl Pts',(-4.084909445423,-16.6638724411723,16.3868078748572));
#144857=CARTESIAN_POINT('Ctrl Pts',(-4.03044710954714,-16.500694908825,
16.3993030153564));
#144858=CARTESIAN_POINT('Ctrl Pts',(-3.96829324310505,-16.3426975171319,
16.4144180987784));
#144859=CARTESIAN_POINT('Ctrl Pts',(-3.87688666777836,-16.1572121716626,
16.436082235871));
#144860=CARTESIAN_POINT('Ctrl Pts',(-3.69817616932894,-15.8750570428302,
16.4661169180521));
#144861=CARTESIAN_POINT('Ctrl Pts',(-3.52791761123353,-15.6602065606675,
16.472559675109));
#144862=CARTESIAN_POINT('Ctrl Pts',(-3.40369690428402,-15.516091679354,
16.4574186477821));
#144863=CARTESIAN_POINT('Ctrl Pts',(-4.16407740090863,-17.1297201895698,
16.3950704330864));
#144864=CARTESIAN_POINT('Ctrl Pts',(-4.17309867009879,-17.1286064742394,
16.3866195493542));
#144865=CARTESIAN_POINT('Ctrl Pts',(-4.18636378592173,-17.1141977739953,
16.3731958794539));
#144866=CARTESIAN_POINT('Ctrl Pts',(-4.2007971294629,-17.0762147421848,
16.3573798048861));
#144867=CARTESIAN_POINT('Ctrl Pts',(-4.21449765860984,-17.00093000886,16.3407443488439));
#144868=CARTESIAN_POINT('Ctrl Pts',(-4.22313388349631,-16.8464676114765,
16.3272957665252));
#144869=CARTESIAN_POINT('Ctrl Pts',(-4.21459807528536,-16.6696778592131,
16.3338317080614));
#144870=CARTESIAN_POINT('Ctrl Pts',(-4.19048552821278,-16.4985546366527,
16.356892527142));
#144871=CARTESIAN_POINT('Ctrl Pts',(-4.15397606217355,-16.3321688812547,
16.390284419557));
#144872=CARTESIAN_POINT('Ctrl Pts',(-4.08234299653493,-16.135908034094,
16.4481217202394));
#144873=CARTESIAN_POINT('Ctrl Pts',(-3.89286548876974,-15.8363272941988,
16.5528979639547));
#144874=CARTESIAN_POINT('Ctrl Pts',(-3.65781260387296,-15.6050158945688,
16.5971927661982));
#144875=CARTESIAN_POINT('Ctrl Pts',(-3.484171134057,-15.4526355429943,16.5617031069992));
#144876=CARTESIAN_POINT('Ctrl Pts',(-4.16805924125643,-17.1531430391027,
16.3927289346864));
#144877=CARTESIAN_POINT('Ctrl Pts',(-4.18298182306529,-17.1512963280167,
16.3785132377752));
#144878=CARTESIAN_POINT('Ctrl Pts',(-4.20588345022822,-17.1358278214066,
16.3545595711711));
#144879=CARTESIAN_POINT('Ctrl Pts',(-4.23261434468994,-17.0965546016377,
16.3238807136553));
#144880=CARTESIAN_POINT('Ctrl Pts',(-4.26155471740868,-17.0195426579297,
16.2870832365073));
#144881=CARTESIAN_POINT('Ctrl Pts',(-4.29142198289111,-16.8615280733557,
16.2438785345673));
#144882=CARTESIAN_POINT('Ctrl Pts',(-4.30284255427461,-16.6780413458487,
16.2257886933808));
#144883=CARTESIAN_POINT('Ctrl Pts',(-4.30015587581447,-16.495765620729,
16.2332149212329));
#144884=CARTESIAN_POINT('Ctrl Pts',(-4.28596701049521,-16.3151284088004,
16.2588392704518));
#144885=CARTESIAN_POINT('Ctrl Pts',(-4.24322921026512,-16.0956649254156,
16.3252794120497));
#144886=CARTESIAN_POINT('Ctrl Pts',(-4.08618086693028,-15.7561566065747,
16.4925437736698));
#144887=CARTESIAN_POINT('Ctrl Pts',(-3.82169923706759,-15.5135583824825,
16.6184335132367));
#144888=CARTESIAN_POINT('Ctrl Pts',(-3.59497510060098,-15.3652635777075,
16.6));
#144889=CARTESIAN_POINT('Ctrl Pts',(-4.16968069936174,-17.1648544705749,
16.3911731305015));
#144890=CARTESIAN_POINT('Ctrl Pts',(-4.18751555020898,-17.1626412633014,
16.3740604246625));
#144891=CARTESIAN_POINT('Ctrl Pts',(-4.21488136238738,-17.1466430737096,
16.344552703831));
#144892=CARTESIAN_POINT('Ctrl Pts',(-4.24674448939413,-17.1067250534971,
16.305735840826));
#144893=CARTESIAN_POINT('Ctrl Pts',(-4.28111161194148,-17.0288513854137,
16.2575852802216));
#144894=CARTESIAN_POINT('Ctrl Pts',(-4.3164940870397,-16.8690652334165,
16.197184839744));
#144895=CARTESIAN_POINT('Ctrl Pts',(-4.33114148592674,-16.682242226022,
16.164479258454));
#144896=CARTESIAN_POINT('Ctrl Pts',(-4.33276019641122,-16.4943822165373,
16.1612288892188));
#144897=CARTESIAN_POINT('Ctrl Pts',(-4.32419391032616,-16.3065945433838,
16.1795042852215));
#144898=CARTESIAN_POINT('Ctrl Pts',(-4.29214178574177,-16.075454478799,
16.2446281088384));
#144899=CARTESIAN_POINT('Ctrl Pts',(-4.15704520376224,-15.7158195120752,
16.4317690537223));
#144900=CARTESIAN_POINT('Ctrl Pts',(-3.89740878663184,-15.4677167334541,
16.6));
#144901=CARTESIAN_POINT('Ctrl Pts',(-3.65042002992564,-15.3215437309242,
16.6));
#144902=CARTESIAN_POINT('',(-4.15558499113943,-17.0949600091324,16.3958530281318));
#144903=CARTESIAN_POINT('Ctrl Pts',(-4.18187625800635,-17.1623114267662,
16.3792076522946));
#144904=CARTESIAN_POINT('Ctrl Pts',(-4.17634967961608,-17.1520585558519,
16.3847557199795));
#144905=CARTESIAN_POINT('Ctrl Pts',(-4.17124056639269,-17.14091999511,16.3890221165494));
#144906=CARTESIAN_POINT('Ctrl Pts',(-4.16669365147873,-17.1291585903885,
16.3918453420656));
#144907=CARTESIAN_POINT('Ctrl Pts',(-4.1624355815674,-17.1181443346773,
16.3944892207946));
#144908=CARTESIAN_POINT('Ctrl Pts',(-4.15869481542099,-17.1066547384278,
16.3958530346329));
#144909=CARTESIAN_POINT('Ctrl Pts',(-4.15558608030974,-17.0949638327396,
16.3958525879769));
#144910=CARTESIAN_POINT('',(-3.37654926102705,-15.5374983403089,16.3958530281318));
#144911=CARTESIAN_POINT('Origin',(-3.65042002992564,-15.3215437309242,16.2));
#144912=CARTESIAN_POINT('Origin',(8.85953015492336E-16,-18.2,16.3958530281318));
#144913=CARTESIAN_POINT('Origin',(1.07729948100197E-15,-18.2,16.2));
#144914=CARTESIAN_POINT('Origin',(8.85953015492336E-16,-18.2,16.3958530281318));
#144915=CARTESIAN_POINT('Origin',(17.5,-22.1,11.6));
#144916=CARTESIAN_POINT('',(16.3999999999996,-22.1,11.6));
#144917=CARTESIAN_POINT('',(16.3999999999996,-22.1,11.6));
#144918=CARTESIAN_POINT('',(16.9,-22.1,11.6));
#144919=CARTESIAN_POINT('',(8.74999999998871,-22.1,11.6));
#144920=CARTESIAN_POINT('',(16.9,-22.1,11.6));
#144921=CARTESIAN_POINT('Origin',(16.9,-22.1,11.));
#144922=CARTESIAN_POINT('Origin',(16.9,-22.1,11.));
#144923=CARTESIAN_POINT('Origin',(16.3999999999996,-22.1,15.7));
#144924=CARTESIAN_POINT('',(14.742553191489,-22.1,11.9499506567302));
#144925=CARTESIAN_POINT('',(14.742553191489,-22.1,11.9499506567302));
#144926=CARTESIAN_POINT('Origin',(16.3999999999996,-22.1,15.7));
#144927=CARTESIAN_POINT('Origin',(11.6999999999997,-10.3,10.2176829561026));
#144928=CARTESIAN_POINT('Origin',(11.6999999999997,-10.3,10.2176829561026));
#144929=CARTESIAN_POINT('Origin',(0.,-24.4,18.2));
#144930=CARTESIAN_POINT('',(-9.16862915008378,-25.4,18.2));
#144931=CARTESIAN_POINT('',(-9.16862915008378,-24.4,18.2));
#144932=CARTESIAN_POINT('',(12.8999999999995,-25.4,18.2));
#144933=CARTESIAN_POINT('',(-1.12865534254263E-11,-25.4,18.2));
#144934=CARTESIAN_POINT('',(12.8999999999995,-10.3,18.2));
#144935=CARTESIAN_POINT('',(12.8999999999995,-22.15,18.2));
#144936=CARTESIAN_POINT('',(-5.79396237474835,-10.3,18.2));
#144937=CARTESIAN_POINT('Origin',(12.8999999999995,-22.15,17.2));
#144938=CARTESIAN_POINT('',(13.8999999999995,-25.4,17.2));
#144939=CARTESIAN_POINT('Origin',(12.8999999999995,-25.4,17.2));
#144940=CARTESIAN_POINT('',(13.8999999999997,-10.3,17.2));
#144941=CARTESIAN_POINT('',(13.8999999999995,-22.15,17.2));
#144942=CARTESIAN_POINT('Origin',(12.8999999999995,-10.3,17.2));
#144943=CARTESIAN_POINT('Origin',(16.3999999999996,-22.15,15.7));
#144944=CARTESIAN_POINT('',(16.3999999999996,-25.4,13.2));
#144945=CARTESIAN_POINT('',(13.8999999999996,-25.4,15.6999999999999));
#144946=CARTESIAN_POINT('Origin',(16.3999999999996,-25.4,15.7));
#144947=CARTESIAN_POINT('',(16.3999999999996,-22.1,13.2));
#144948=CARTESIAN_POINT('',(16.3999999999996,-22.15,13.2));
#144949=CARTESIAN_POINT('',(13.8999999999996,-22.1,15.6999999999999));
#144950=CARTESIAN_POINT('Origin',(16.3999999999996,-22.1,15.7));
#144951=CARTESIAN_POINT('',(13.8999999999996,-22.15,15.6999999999999));
#144952=CARTESIAN_POINT('Origin',(19.1,-24.4,13.2));
#144953=CARTESIAN_POINT('',(18.1,-25.4,13.2));
#144954=CARTESIAN_POINT('',(9.54999999998872,-25.4,13.2));
#144955=CARTESIAN_POINT('',(18.1,-22.1,13.2));
#144956=CARTESIAN_POINT('',(18.1,-24.4,13.2));
#144957=CARTESIAN_POINT('',(9.54999999998872,-22.1,13.2));
#144958=CARTESIAN_POINT('Origin',(18.1,-24.4,12.2));
#144959=CARTESIAN_POINT('',(19.1,-25.4,12.2));
#144960=CARTESIAN_POINT('Origin',(18.1,-25.4,12.2));
#144961=CARTESIAN_POINT('',(19.1,-22.1,12.2));
#144962=CARTESIAN_POINT('',(19.1,-24.4,12.2));
#144963=CARTESIAN_POINT('Origin',(18.1,-22.1,12.2));
#144964=CARTESIAN_POINT('Origin',(15.1,-22.55,-15.1));
#144965=CARTESIAN_POINT('',(17.5765623826223,-22.1,3.02656238258888));
#144966=CARTESIAN_POINT('',(16.7650854557587,-23.,2.2150854557252));
#144967=CARTESIAN_POINT('Ctrl Pts',(17.5765623826223,-22.1,3.02656238258888));
#144968=CARTESIAN_POINT('Ctrl Pts',(17.1605923305092,-22.568450440311,2.61059233047568));
#144969=CARTESIAN_POINT('Ctrl Pts',(16.7650854557587,-23.,2.21508545572519));
#144970=CARTESIAN_POINT('Origin',(15.1,-23.,-15.1));
#144971=CARTESIAN_POINT('',(9.9082087163681,-22.1,2.44283125131488));
#144972=CARTESIAN_POINT('Ctrl Pts',(7.99320388349492,-22.1690497294436,
1.68324514365148));
#144973=CARTESIAN_POINT('Ctrl Pts',(8.26898312988902,-22.2130454645242,
1.75224517737468));
#144974=CARTESIAN_POINT('Ctrl Pts',(8.54092388752982,-22.2349444050467,
1.83645502172102));
#144975=CARTESIAN_POINT('Ctrl Pts',(9.18093316499991,-22.2349444050467,
2.07300875877398));
#144976=CARTESIAN_POINT('Ctrl Pts',(9.55380073243788,-22.1895443581543,
2.24456092434208));
#144977=CARTESIAN_POINT('Ctrl Pts',(9.9082087163681,-22.1,2.44283125131488));
#144978=CARTESIAN_POINT('Origin',(15.1,-22.1,-15.1));
#144979=CARTESIAN_POINT('Origin',(-2.25752749827279E-11,-22.1,-0.450000000022577));
#144980=CARTESIAN_POINT('Origin',(6.1,-22.1,-12.1857384988752));
#144981=CARTESIAN_POINT('',(16.4999999999912,-22.1,-7.7186291501247));
#144982=CARTESIAN_POINT('',(16.4999999999906,-22.1,-8.05000000002406));
#144983=CARTESIAN_POINT('Origin',(17.2999999999912,-22.1,-7.71862915012621));
#144984=CARTESIAN_POINT('Origin',(14.4999999999996,-22.1,11.401162947959));
#144985=CARTESIAN_POINT('',(13.8999999999996,-22.1,11.401162947959));
#144986=CARTESIAN_POINT('',(13.8999999999996,-22.1,11.401162947959));
#144987=CARTESIAN_POINT('Origin',(14.4999999999996,-22.1,11.401162947959));
#144988=CARTESIAN_POINT('Origin',(-13.9260346165329,-15.9,10.3798528337676));
#144989=CARTESIAN_POINT('Origin',(-13.9260346165329,-15.7,10.3798528337676));
#144990=CARTESIAN_POINT('Origin',(-12.3362327337785,-22.8,13.1010255664155));
#144991=CARTESIAN_POINT('',(-9.07157287523651,-15.7,16.3656854249499));
#144992=CARTESIAN_POINT('',(-9.07157287523651,-16.55,16.3656854249499));
#144993=CARTESIAN_POINT('',(-11.0195632919613,-15.7,14.4176950082296));
#144994=CARTESIAN_POINT('Origin',(-8.50588745028793,-16.55,15.8));
#144995=CARTESIAN_POINT('Origin',(-8.50588745028793,-15.7,15.8));
#144996=CARTESIAN_POINT('Origin',(-4.89034568556533,-10.3,14.3396641393448));
#144997=CARTESIAN_POINT('',(-7.07515042368407,-15.7,16.3841343442657));
#144998=CARTESIAN_POINT('',(-4.89034568556533,-15.7,14.3396641393448));
#144999=CARTESIAN_POINT('',(-7.07515042368407,-15.7,16.3841343442657));
#145000=CARTESIAN_POINT('',(-7.07515042368407,-10.3,16.3841343442657));
#145001=CARTESIAN_POINT('',(-7.07515042368407,-10.3,16.3841343442657));
#145002=CARTESIAN_POINT('',(-4.89034568556533,-10.3,14.3396641393448));
#145003=CARTESIAN_POINT('',(-1.82100242629958,-10.3,11.4674711544254));
#145004=CARTESIAN_POINT('',(-4.89034568556533,-21.1,14.3396641393448));
#145005=CARTESIAN_POINT('Origin',(-7.62176460923847,-10.3,15.8));
#145006=CARTESIAN_POINT('Origin',(-7.62176460923847,-15.7,15.8));
#145007=CARTESIAN_POINT('Origin',(-7.62176460923847,-10.3,15.8));
#145008=CARTESIAN_POINT('Origin',(-16.5000000000123,-24.4,1.94999999997646));
#145009=CARTESIAN_POINT('',(-16.5000000000305,-20.,-7.71862915012594));
#145010=CARTESIAN_POINT('',(-16.5000000000089,-20.,3.77623615174464));
#145011=CARTESIAN_POINT('',(-16.5000000000195,-20.,-1.85000000003706));
#145012=CARTESIAN_POINT('',(-16.5000000000305,-25.4,-7.71862915012594));
#145013=CARTESIAN_POINT('',(-16.5000000000305,-24.4,-7.71862915012594));
#145014=CARTESIAN_POINT('',(-16.4999999999955,-25.4,10.8686291501049));
#145015=CARTESIAN_POINT('',(-16.5000000000146,-25.4,0.749999999992473));
#145016=CARTESIAN_POINT('',(-16.4999999999955,-24.4,10.8686291501049));
#145017=CARTESIAN_POINT('',(-16.5000000000054,-15.9,5.6354763829797));
#145018=CARTESIAN_POINT('',(-16.5000000000054,-22.8,5.6354763829797));
#145019=CARTESIAN_POINT('',(-16.5000000000089,-15.9,3.77623615174464));
#145020=CARTESIAN_POINT('',(-16.4999999999949,-15.9,11.2000000000031));
#145021=CARTESIAN_POINT('',(-16.5000000000089,-19.9,3.77623615174464));
#145022=CARTESIAN_POINT('Origin',(-15.6999999999955,-24.4,10.8686291501034));
#145023=CARTESIAN_POINT('',(-16.2656854249441,-25.4,11.4343145750533));
#145024=CARTESIAN_POINT('Origin',(-15.6999999999955,-25.4,10.8686291501034));
#145025=CARTESIAN_POINT('',(-16.2656854249441,-24.4,11.4343145750533));
#145026=CARTESIAN_POINT('Origin',(-10.6033654998821,-24.4,17.0966345001022));
#145027=CARTESIAN_POINT('',(-9.73431457503237,-25.4,17.9656854249499));
#145028=CARTESIAN_POINT('',(-9.73431457503237,-24.4,17.9656854249499));
#145029=CARTESIAN_POINT('',(-12.3391827499422,-25.4,15.3608172500461));
#145030=CARTESIAN_POINT('Origin',(-9.16862915008378,-24.4,17.4));
#145031=CARTESIAN_POINT('Origin',(-9.16862915008378,-25.4,17.4));
#145032=CARTESIAN_POINT('Origin',(-2.25752749827279E-11,-22.1,-0.450000000022577));
#145033=CARTESIAN_POINT('',(18.8656854249492,-22.1,4.31568542491577));
#145034=CARTESIAN_POINT('',(19.1,-22.1,4.88137084986501));
#145035=CARTESIAN_POINT('Origin',(18.3,-22.1,4.881370849865));
#145036=CARTESIAN_POINT('',(11.7750000000018,-22.1,-2.77500000003169));
#145037=CARTESIAN_POINT('Origin',(6.09999999999969,-22.1,9.2499999999633));
#145038=CARTESIAN_POINT('',(13.8999999999997,-22.1,6.04557695250827));
#145039=CARTESIAN_POINT('',(19.1,-22.1,-19.1));
#145040=CARTESIAN_POINT('Origin',(19.1,-24.4,18.2));
#145041=CARTESIAN_POINT('',(19.1,-25.4,4.881370849865));
#145042=CARTESIAN_POINT('',(19.1,-24.4,4.881370849865));
#145043=CARTESIAN_POINT('',(19.1,-25.4,8.87499999998871));
#145044=CARTESIAN_POINT('Origin',(18.3,-24.4,4.881370849865));
#145045=CARTESIAN_POINT('',(18.8656854249492,-25.4,4.31568542491577));
#145046=CARTESIAN_POINT('Origin',(18.3,-25.4,4.881370849865));
#145047=CARTESIAN_POINT('',(18.8656854249492,-24.4,4.31568542491577));
#145048=CARTESIAN_POINT('Origin',(17.2999999999912,-24.4,-7.71862915012621));
#145049=CARTESIAN_POINT('',(16.4999999999912,-25.4,-7.7186291501247));
#145050=CARTESIAN_POINT('',(16.4999999999912,-24.4,-7.7186291501247));
#145051=CARTESIAN_POINT('Origin',(17.2999999999912,-25.4,-7.71862915012621));
#145052=CARTESIAN_POINT('Origin',(-8.47750127826606,-21.1,10.5062825051013));
#145053=CARTESIAN_POINT('',(-4.68280159094393,-15.7,6.87823147417057));
#145054=CARTESIAN_POINT('',(-4.68280159094394,-10.3,6.87823147417058));
#145055=CARTESIAN_POINT('',(-4.68280159094394,-15.7,6.87823147417058));
#145056=CARTESIAN_POINT('Origin',(-8.47750127826606,-15.7,10.5062825051013));
#145057=CARTESIAN_POINT('Origin',(-8.47750127826606,-10.3,10.5062825051013));
#145058=CARTESIAN_POINT('Origin',(2.24865810106615,-10.3,9.66425824155912));
#145059=CARTESIAN_POINT('',(-4.57640302989081,-10.3,6.24598149558596));
#145060=CARTESIAN_POINT('Origin',(-4.39368161476701,-10.3,6.60180853848062));
#145061=CARTESIAN_POINT('',(13.8999999999997,-10.3,9.24999999996345));
#145062=CARTESIAN_POINT('',(13.8999999999997,-10.3,7.8549175970337));
#145063=CARTESIAN_POINT('Origin',(6.09999999999969,-10.3,9.2499999999633));
#145064=CARTESIAN_POINT('Origin',(-9.35,-10.3,-3.05000000003699));
#145065=CARTESIAN_POINT('Origin',(-4.39368161476701,-15.7,6.60180853848062));
#145066=CARTESIAN_POINT('',(-4.57640302989081,-15.7,6.24598149558596));
#145067=CARTESIAN_POINT('',(-4.57640302989081,-15.7,6.24598149558596));
#145068=CARTESIAN_POINT('Origin',(-4.39368161476701,-15.7,6.60180853848062));
#145069=CARTESIAN_POINT('Origin',(-9.35,-15.7,-3.05000000003699));
#145070=CARTESIAN_POINT('',(-9.43222590492927,-15.7,7.39967649737471));
#145071=CARTESIAN_POINT('',(-7.92889383452772,-15.7,7.30292022888666));
#145072=CARTESIAN_POINT('Ctrl Pts',(-9.43222590492927,-15.7,7.39967649737471));
#145073=CARTESIAN_POINT('Ctrl Pts',(-9.19930785473307,-15.7701742479532,
7.40150927157174));
#145074=CARTESIAN_POINT('Ctrl Pts',(-8.95201593280048,-15.8156689756711,
7.39600675444461));
#145075=CARTESIAN_POINT('Ctrl Pts',(-8.40561223809871,-15.8156689756711,
7.36083955244824));
#145076=CARTESIAN_POINT('Ctrl Pts',(-8.15965523600794,-15.7701742479532,
7.33459597284539));
#145077=CARTESIAN_POINT('Ctrl Pts',(-7.92889383452772,-15.7,7.30292022888666));
#145078=CARTESIAN_POINT('Origin',(-9.35,-15.7,-3.05000000003699));
#145079=CARTESIAN_POINT('',(-11.4725028070433,-15.9,7.18217874322649));
#145080=CARTESIAN_POINT('Origin',(-9.35,-15.9,-3.05000000003699));
#145081=CARTESIAN_POINT('',(-11.4725028070433,-15.7,7.18217874322649));
#145082=CARTESIAN_POINT('',(-11.4725028070433,-15.7,7.18217874322649));
#145083=CARTESIAN_POINT('Origin',(-9.35,-15.7,-3.05000000003699));
#145084=CARTESIAN_POINT('Origin',(-11.5537469336287,-15.7,7.57384108746624));
#145085=CARTESIAN_POINT('Origin',(-11.5537469336287,-15.7,7.57384108746624));
#145086=CARTESIAN_POINT('Origin',(-11.5537469336287,-15.9,7.57384108746624));
#145087=CARTESIAN_POINT('Origin',(-8.47750127826606,-24.4,10.5062825051013));
#145088=CARTESIAN_POINT('',(-5.42750127826606,-15.9,10.5062825051013));
#145089=CARTESIAN_POINT('',(-11.5275012782661,-15.9,10.5062825051013));
#145090=CARTESIAN_POINT('Origin',(-8.47750127826606,-15.9,10.5062825051013));
#145091=CARTESIAN_POINT('Origin',(-8.47750127826606,-15.9,10.5062825051013));
#145092=CARTESIAN_POINT('',(-11.5275012782661,-24.4,10.5062825051013));
#145093=CARTESIAN_POINT('Origin',(-8.85961065987377,-15.7,11.5466726141172));
#145094=CARTESIAN_POINT('',(-5.22750127826606,-15.7,10.5062825051013));
#145095=CARTESIAN_POINT('Origin',(-8.47750127826606,-15.7,10.5062825051013));
#145096=CARTESIAN_POINT('Origin',(-8.47750127826606,-15.7,10.5062825051013));
#145097=CARTESIAN_POINT('Origin',(-8.47750127826606,-15.8,10.5062825051013));
#145098=CARTESIAN_POINT('',(-5.32750127826606,-15.8,10.5062825051013));
#145099=CARTESIAN_POINT('Origin',(-13.5133325473166,-19.9,5.36110350072047));
#145100=CARTESIAN_POINT('',(-10.7906143361206,-20.,0.645217224236));
#145101=CARTESIAN_POINT('',(-10.7906143361206,-21.1,0.645217224236));
#145102=CARTESIAN_POINT('',(-13.0883185289381,-20.,4.62495762695992));
#145103=CARTESIAN_POINT('',(-11.4476530870906,-20.,1.78324172345756));
#145104=CARTESIAN_POINT('',(-13.0883185289381,-19.9,4.62495762695993));
#145105=CARTESIAN_POINT('Origin',(-2.6403124237551,-20.,-0.450000000022575));
#145106=CARTESIAN_POINT('',(-0.00257311493774171,-20.,-4.50827945559669));
#145107=CARTESIAN_POINT('Origin',(-0.00257311493774171,-20.,-4.70827945559669));
#145108=CARTESIAN_POINT('',(-0.0974268850622617,-20.,-4.50827945559669));
#145109=CARTESIAN_POINT('',(8.27360890601114,-20.,-4.50827945559669));
#145110=CARTESIAN_POINT('Origin',(-0.0974268850622617,-20.,-4.70827945559669));
#145111=CARTESIAN_POINT('',(-0.600000000789417,-20.,-5.79545078503888));
#145112=CARTESIAN_POINT('Origin',(-1.20000000078942,-20.,-5.79545078503888));
#145113=CARTESIAN_POINT('',(-0.600000000789417,-20.,-4.25000000003699));
#145114=CARTESIAN_POINT('',(-0.600000000789418,-20.,-0.0326255494647287));
#145115=CARTESIAN_POINT('',(-1.20000000078942,-20.,-3.65000000003699));
#145116=CARTESIAN_POINT('Origin',(-1.20000000078942,-20.,-4.25000000003699));
#145117=CARTESIAN_POINT('',(-1.31220842229031,-20.,-3.65000000003699));
#145118=CARTESIAN_POINT('Origin',(-5.42954084321747,-20.,-1.85000000003699));
#145119=CARTESIAN_POINT('',(-0.0620826661477014,-20.,-1.80272960390294));
#145120=CARTESIAN_POINT('Origin',(-0.0620826661477014,-20.,-1.60272960390294));
#145121=CARTESIAN_POINT('',(-0.037917333852302,-20.,-1.80272960390294));
#145122=CARTESIAN_POINT('',(8.27360890601114,-20.,-1.80272960390295));
#145123=CARTESIAN_POINT('Origin',(-0.037917333852302,-20.,-1.60272960390295));
#145124=CARTESIAN_POINT('',(1.19999999921058,-20.,-2.45000000003699));
#145125=CARTESIAN_POINT('Origin',(1.19999999921058,-20.,-1.85000000003699));
#145126=CARTESIAN_POINT('',(4.3,-20.,-2.45000000003699));
#145127=CARTESIAN_POINT('',(-4.29148370813747,-20.,-2.45000000003699));
#145128=CARTESIAN_POINT('',(4.9,-20.,-1.85000000003699));
#145129=CARTESIAN_POINT('Origin',(4.3,-20.,-1.85000000003699));
#145130=CARTESIAN_POINT('',(4.9,-20.,-0.741996797474059));
#145131=CARTESIAN_POINT('',(4.9,-20.,-2.88858360955241));
#145132=CARTESIAN_POINT('Origin',(8.6,-20.,-0.741996797474057));
#145133=CARTESIAN_POINT('',(13.7548828365128,-20.,7.75241235336064));
#145134=CARTESIAN_POINT('Origin',(13.3623247423326,-20.,7.82921171985308));
#145135=CARTESIAN_POINT('Origin',(6.09999999999969,-20.,9.2499999999633));
#145136=CARTESIAN_POINT('Origin',(6.1,-20.,-12.1857384988752));
#145137=CARTESIAN_POINT('Origin',(-12.5687032866674,-19.9,4.92495762695992));
#145138=CARTESIAN_POINT('Origin',(-12.5687032866674,-20.,4.92495762695992));
#145139=CARTESIAN_POINT('Origin',(0.,-18.2,-19.1));
#145140=CARTESIAN_POINT('Origin',(0.,-18.2,1.41228796703553));
#145141=CARTESIAN_POINT('Origin',(0.,-18.2,0.728598564603416));
#145142=CARTESIAN_POINT('',(-1.,-18.2,-19.1));
#145143=CARTESIAN_POINT('Origin',(19.1875302357774,-18.9150528379807,-5.20109977862422));
#145144=CARTESIAN_POINT('',(0.192158240549244,-19.225912103606,-4.66267573655754));
#145145=CARTESIAN_POINT('Origin',(-7.13578540802763E-18,-17.9401923788647,
-6.889607624103));
#145146=CARTESIAN_POINT('',(-0.0974268850622617,-19.3150528379807,-4.50827945559669));
#145147=CARTESIAN_POINT('Origin',(-0.0974268850622617,-19.1995827841427,
-4.70827945559669));
#145148=CARTESIAN_POINT('',(-0.00257311493774059,-19.3150528379807,-4.50827945559669));
#145149=CARTESIAN_POINT('',(19.1875302357774,-19.3150528379807,-4.50827945559669));
#145150=CARTESIAN_POINT('Origin',(-0.00257311493774171,-19.1995827841427,
-4.70827945559669));
#145151=CARTESIAN_POINT('Origin',(19.1875302357774,-16.3150528379807,-1.80272960390295));
#145152=CARTESIAN_POINT('',(-0.0620826661477025,-15.9,-1.80272960390294));
#145153=CARTESIAN_POINT('',(-0.0620826661477025,-16.3150528379807,-1.80272960390294));
#145154=CARTESIAN_POINT('',(-0.0620826661477026,-19.9,-1.80272960390294));
#145155=CARTESIAN_POINT('',(-0.0379173338523009,-15.9,-1.80272960390294));
#145156=CARTESIAN_POINT('',(8.03659089635399,-15.9,-1.80272960390294));
#145157=CARTESIAN_POINT('',(-0.037917333852302,-16.3150528379807,-1.80272960390294));
#145158=CARTESIAN_POINT('',(-0.0379173338523009,-21.1,-1.80272960390294));
#145159=CARTESIAN_POINT('',(19.1875302357774,-16.3150528379807,-1.80272960390295));
#145160=CARTESIAN_POINT('Origin',(19.1875302357774,-15.8150528379807,-4.50827945559669));
#145161=CARTESIAN_POINT('',(-0.0974268850622617,-16.3150528379807,-4.50827945559669));
#145162=CARTESIAN_POINT('',(-0.0974268850622628,-15.9,-4.50827945559669));
#145163=CARTESIAN_POINT('',(-0.0974268850622628,-19.9,-4.50827945559669));
#145164=CARTESIAN_POINT('',(-0.00257311493774059,-16.3150528379807,-4.50827945559669));
#145165=CARTESIAN_POINT('',(19.1875302357774,-16.3150528379807,-4.50827945559669));
#145166=CARTESIAN_POINT('',(-0.00257311493774171,-15.9,-4.50827945559669));
#145167=CARTESIAN_POINT('',(-0.00257311493774168,-21.1,-4.50827945559669));
#145168=CARTESIAN_POINT('',(8.03659089635399,-15.9,-4.50827945559669));
#145169=CARTESIAN_POINT('Origin',(19.1875302357774,-16.3150528379807,-4.50827945559669));
#145170=CARTESIAN_POINT('Origin',(4.54783644736696E-17,-18.4457456132867,
-7.55122409562988));
#145171=CARTESIAN_POINT('Origin',(-0.00257311493774171,-16.4550943456226,
-4.70827945559669));
#145172=CARTESIAN_POINT('Origin',(-0.0974268850622628,-16.4550943456226,
-4.70827945559669));
#145173=CARTESIAN_POINT('Origin',(19.1875302357774,-19.3150528379807,-4.50827945559669));
#145174=CARTESIAN_POINT('',(-0.00257311493774168,-21.1,-4.50827945559669));
#145175=CARTESIAN_POINT('',(-0.0974268850622617,-19.9,-4.50827945559669));
#145176=CARTESIAN_POINT('Origin',(-0.0974268850622617,-19.9,-4.70827945559669));
#145177=CARTESIAN_POINT('Origin',(-0.00257311493774171,-21.1,-4.70827945559669));
#145178=CARTESIAN_POINT('Ctrl Pts',(0.192159868891087,-19.2258247671933,
-4.6628270076618));
#145179=CARTESIAN_POINT('Ctrl Pts',(0.192955152312465,-19.2238679775077,
-4.66621855530548));
#145180=CARTESIAN_POINT('Ctrl Pts',(0.193667594328148,-19.2219578017748,
-4.6696565646564));
#145181=CARTESIAN_POINT('Ctrl Pts',(0.194292330138919,-19.2200994892544,
-4.67313792326465));
#145182=CARTESIAN_POINT('Origin',(-0.00257311493774171,-21.1,-4.70827945559669));
#145183=CARTESIAN_POINT('Origin',(-0.00257311493774171,-15.9,-4.70827945559669));
#145184=CARTESIAN_POINT('Origin',(-0.0974268850622628,-19.9,-4.70827945559669));
#145185=CARTESIAN_POINT('Origin',(-0.0974268850622628,-15.9,-4.70827945559669));
#145186=CARTESIAN_POINT('Origin',(-0.0379173338523009,-21.1,-1.60272960390294));
#145187=CARTESIAN_POINT('Origin',(-0.0379173338523009,-15.9,-1.60272960390294));
#145188=CARTESIAN_POINT('Origin',(-0.0379173338523009,-16.4550943456226,
-1.60272960390294));
#145189=CARTESIAN_POINT('Origin',(-0.0620826661477025,-19.9,-1.60272960390294));
#145190=CARTESIAN_POINT('Origin',(-0.0620826661477025,-15.9,-1.60272960390294));
#145191=CARTESIAN_POINT('Origin',(-0.0620826661477025,-16.4550943456226,
-1.60272960390294));
#145192=CARTESIAN_POINT('Origin',(19.1875302357774,-19.9150528379807,-1.80272960390295));
#145193=CARTESIAN_POINT('',(-0.0620826661477025,-19.3150528379807,-1.80272960390294));
#145194=CARTESIAN_POINT('',(-0.0620826661477014,-19.9,-1.80272960390294));
#145195=CARTESIAN_POINT('',(-0.037917333852302,-19.3150528379807,-1.80272960390294));
#145196=CARTESIAN_POINT('',(19.1875302357774,-19.3150528379807,-1.80272960390295));
#145197=CARTESIAN_POINT('',(-0.037917333852302,-21.1,-1.80272960390295));
#145198=CARTESIAN_POINT('Origin',(-0.0620826661477014,-19.9,-1.60272960390294));
#145199=CARTESIAN_POINT('Origin',(-0.0620826661477014,-19.1995827841427,
-1.60272960390294));
#145200=CARTESIAN_POINT('Origin',(-0.037917333852302,-21.1,-1.60272960390295));
#145201=CARTESIAN_POINT('',(0.154550859259101,-19.2309727753312,-1.65709866349047));
#145202=CARTESIAN_POINT('Ctrl Pts',(0.159700282405874,-19.2185167914062,
-1.63346006998121));
#145203=CARTESIAN_POINT('Ctrl Pts',(0.158439401477663,-19.2223797827423,
-1.64154567165289));
#145204=CARTESIAN_POINT('Ctrl Pts',(0.156704150703268,-19.2265376018115,
-1.64941336612285));
#145205=CARTESIAN_POINT('Ctrl Pts',(0.1545517600316,-19.2309315391986,-1.65702724041366));
#145206=CARTESIAN_POINT('Origin',(-0.037917333852302,-19.1995827841427,
-1.60272960390295));
#145207=CARTESIAN_POINT('Origin',(19.1875302357774,-19.3150528379807,-1.80272960390295));
#145208=CARTESIAN_POINT('Origin',(-4.41432195622002E-17,-17.9401923788647,
0.578598564603414));
#145209=CARTESIAN_POINT('Ctrl Pts',(0.239413492381404,-19.2179565118977,
-1.63455383389902));
#145210=CARTESIAN_POINT('Ctrl Pts',(0.0329622508010724,-19.256639091472,
-1.70155402708951));
#145211=CARTESIAN_POINT('Ctrl Pts',(-0.182855485725863,-19.2442944946718,
-1.68017255823251));
#145212=CARTESIAN_POINT('Ctrl Pts',(-0.38354942837159,-19.1823235458498,
-1.57283572627961));
#145213=CARTESIAN_POINT('Ctrl Pts',(0.220025619949421,-19.1920879531095,
-1.58974817575931));
#145214=CARTESIAN_POINT('Ctrl Pts',(0.0304801589848503,-19.2302536493785,
-1.6557966353406));
#145215=CARTESIAN_POINT('Ctrl Pts',(-0.168404518381573,-19.2180965784821,
-1.63469104263094));
#145216=CARTESIAN_POINT('Ctrl Pts',(-0.35222244035206,-19.1569603036518,
-1.52890530214794));
#145217=CARTESIAN_POINT('Ctrl Pts',(0.200667423514428,-19.1798032977788,
-1.53719128952209));
#145218=CARTESIAN_POINT('Ctrl Pts',(0.0279861671460582,-19.2149481765117,
-1.60369891136253));
#145219=CARTESIAN_POINT('Ctrl Pts',(-0.15394211994542,-19.2036985468328,
-1.58245502005562));
#145220=CARTESIAN_POINT('Ctrl Pts',(-0.320960312691724,-19.1474811411372,
-1.4759254735363));
#145221=CARTESIAN_POINT('Ctrl Pts',(0.184164224908773,-19.1828954869485,
-1.48455383389902));
#145222=CARTESIAN_POINT('Ctrl Pts',(0.0253555775392867,-19.2126513173903,
-1.55155402708952));
#145223=CARTESIAN_POINT('Ctrl Pts',(-0.140658065942972,-19.2031554736978,
-1.53017255823251));
#145224=CARTESIAN_POINT('Ctrl Pts',(-0.295038021824301,-19.1554855130655,
-1.42283572627961));
#145225=CARTESIAN_POINT('Ctrl Pts',(-0.445894921065382,-19.1613302577989,
-4.77453477474201));
#145226=CARTESIAN_POINT('Ctrl Pts',(-0.210103453700173,-19.2474288217223,
-4.62540768756798));
#145227=CARTESIAN_POINT('Ctrl Pts',(0.0508640605567958,-19.2632280647536,
-4.59804259591671));
#145228=CARTESIAN_POINT('Ctrl Pts',(0.295320308048652,-19.2062041938388,
-4.69681083758541));
#145229=CARTESIAN_POINT('Ctrl Pts',(-0.409289944973037,-19.1362684546969,
-4.81794309104411));
#145230=CARTESIAN_POINT('Ctrl Pts',(-0.193645890390995,-19.2212017125735,
-4.67099311891243));
#145231=CARTESIAN_POINT('Ctrl Pts',(0.0470734714362628,-19.2367613684955,
-4.64397201463185));
#145232=CARTESIAN_POINT('Ctrl Pts',(0.271337754375829,-19.180501426813,
-4.7413293359692));
#145233=CARTESIAN_POINT('Ctrl Pts',(-0.37277385892892,-19.1284635659547,
-4.8711741434902));
#145234=CARTESIAN_POINT('Ctrl Pts',(-0.177157130011096,-19.2064969954954,
-4.72318393045555));
#145235=CARTESIAN_POINT('Ctrl Pts',(0.0432613162406244,-19.2209198881668,
-4.69598856904055));
#145236=CARTESIAN_POINT('Ctrl Pts',(0.247395954893676,-19.1691370458623,
-4.79402523679034));
#145237=CARTESIAN_POINT('Ctrl Pts',(-0.342996093127217,-19.1393368299494,
-4.92453477474201));
#145238=CARTESIAN_POINT('Ctrl Pts',(-0.161618041307826,-19.2055664945059,
-4.77540768756798));
#145239=CARTESIAN_POINT('Ctrl Pts',(0.0391262004283044,-19.2177197583761,
-4.74804259591671));
#145240=CARTESIAN_POINT('Ctrl Pts',(0.227169467729732,-19.1738552422878,
-4.84681083758542));
#145241=CARTESIAN_POINT('Origin',(0.,-18.2,-7.039607624103));
#145242=CARTESIAN_POINT('Ctrl Pts',(-0.605214914090967,-17.2952175137768,
-5.90809968361399));
#145243=CARTESIAN_POINT('Ctrl Pts',(-0.623018660594374,-17.3333600838434,
-5.96257291902663));
#145244=CARTESIAN_POINT('Ctrl Pts',(-0.648851205478286,-17.3868815961198,
-6.03900956010202));
#145245=CARTESIAN_POINT('Ctrl Pts',(-0.678920665712354,-17.4468307073562,
-6.12462576382018));
#145246=CARTESIAN_POINT('Ctrl Pts',(-0.689573580943891,-17.4676466969021,
-6.15435407779857));
#145247=CARTESIAN_POINT('Ctrl Pts',(-0.689576769163932,-17.4676488696199,
-6.15435513352118));
#145248=CARTESIAN_POINT('Ctrl Pts',(-0.55385925080104,-17.3273362577698,
-5.95397000382664));
#145249=CARTESIAN_POINT('Ctrl Pts',(-0.579124049415806,-17.3542551168377,
-6.00899666937624));
#145250=CARTESIAN_POINT('Ctrl Pts',(-0.618927029183115,-17.3956063549456,
-6.08234407992258));
#145251=CARTESIAN_POINT('Ctrl Pts',(-0.669540381817794,-17.4504718858759,
-6.15513440299772));
#145252=CARTESIAN_POINT('Ctrl Pts',(-0.690350066847747,-17.4737712704258,
-6.17528093750827));
#145253=CARTESIAN_POINT('Ctrl Pts',(-0.694897793055846,-17.478047099637,
-6.16920739223372));
#145254=CARTESIAN_POINT('Ctrl Pts',(-0.502781108682595,-17.3345631845704,
-6.01690035049276));
#145255=CARTESIAN_POINT('Ctrl Pts',(-0.539605351320391,-17.3562694270032,
-6.06711859772466));
#145256=CARTESIAN_POINT('Ctrl Pts',(-0.594604834126566,-17.393599725971,
-6.131228060911));
#145257=CARTESIAN_POINT('Ctrl Pts',(-0.663199682814476,-17.4507778603678,
-6.18690214327408));
#145258=CARTESIAN_POINT('Ctrl Pts',(-0.692581332696088,-17.4785619697096,
-6.19661963035754));
#145259=CARTESIAN_POINT('Ctrl Pts',(-0.701612310120372,-17.4873509901404,
-6.1843296238416));
#145260=CARTESIAN_POINT('Ctrl Pts',(-0.465549933916129,-17.3149783849924,
-6.0801726145193));
#145261=CARTESIAN_POINT('Ctrl Pts',(-0.511817975000622,-17.3393168679221,
-6.12535925716751));
#145262=CARTESIAN_POINT('Ctrl Pts',(-0.578223751373194,-17.3811061564651,
-6.18014514262514));
#145263=CARTESIAN_POINT('Ctrl Pts',(-0.66000814405107,-17.4476866284114,
-6.21866263408644));
#145264=CARTESIAN_POINT('Ctrl Pts',(-0.696213461155708,-17.4819138991659,
-6.21795888300343));
#145265=CARTESIAN_POINT('Ctrl Pts',(-0.709597871030093,-17.4953931156811,
-6.19945217637467));
#145266=CARTESIAN_POINT('',(-0.465549933916128,-17.3149783849924,-6.0801726145193));
#145267=CARTESIAN_POINT('Ctrl Pts',(-0.707067566378144,-17.4928576526749,
-6.20267384590878));
#145268=CARTESIAN_POINT('Ctrl Pts',(-0.693980570416363,-17.4798073798581,
-6.21798592469554));
#145269=CARTESIAN_POINT('Ctrl Pts',(-0.658926778537658,-17.4468062914195,
-6.218153350034));
#145270=CARTESIAN_POINT('Ctrl Pts',(-0.578223751373194,-17.3811061564651,
-6.18014514262514));
#145271=CARTESIAN_POINT('Ctrl Pts',(-0.511817975000622,-17.3393168679221,
-6.12535925716751));
#145272=CARTESIAN_POINT('Ctrl Pts',(-0.465549933916129,-17.3149783849924,
-6.0801726145193));
#145273=CARTESIAN_POINT('Origin',(-0.605214914090966,-17.0494719004901,
-6.0801726145193));
#145274=CARTESIAN_POINT('Ctrl Pts',(0.838117322977332,-17.4519854043201,
-6.13198743401459));
#145275=CARTESIAN_POINT('Ctrl Pts',(0.669902960334304,-17.3101168025864,
-5.92937807322927));
#145276=CARTESIAN_POINT('Ctrl Pts',(0.191478511893925,-17.080317816636,
-5.6011911094929));
#145277=CARTESIAN_POINT('Ctrl Pts',(-0.345547509129884,-17.1586240778992,
-5.71302404043138));
#145278=CARTESIAN_POINT('Ctrl Pts',(-0.605214914090966,-17.2952175137768,
-5.90809968361399));
#145279=CARTESIAN_POINT('Ctrl Pts',(0.764181235176186,-17.4808267723045,
-6.17317717621315));
#145280=CARTESIAN_POINT('Ctrl Pts',(0.613605800021816,-17.3417952320759,
-5.97506916075729));
#145281=CARTESIAN_POINT('Ctrl Pts',(0.176871355450469,-17.1164577820709,
-5.65299097316032));
#145282=CARTESIAN_POINT('Ctrl Pts',(-0.317987318062742,-17.1933294614096,
-5.76290031980275));
#145283=CARTESIAN_POINT('Ctrl Pts',(-0.553859250801039,-17.3273362577698,
-5.95397000382664));
#145284=CARTESIAN_POINT('Ctrl Pts',(0.691003313955543,-17.4746156005897,
-6.23828151084433));
#145285=CARTESIAN_POINT('Ctrl Pts',(0.557421428927607,-17.3481757435076,
-6.03813220065825));
#145286=CARTESIAN_POINT('Ctrl Pts',(0.162193315798326,-17.1406373153018,
-5.71309101023175));
#145287=CARTESIAN_POINT('Ctrl Pts',(-0.29035089633337,-17.2118747949918,
-5.82396153717806));
#145288=CARTESIAN_POINT('Ctrl Pts',(-0.502781108682595,-17.3345631845704,
-6.01690035049276));
#145289=CARTESIAN_POINT('Ctrl Pts',(0.644705633059487,-17.4355690700257,
-6.3040603649199));
#145290=CARTESIAN_POINT('Ctrl Pts',(0.515309969487927,-17.3264393763844,
-6.10145100413458));
#145291=CARTESIAN_POINT('Ctrl Pts',(0.147291162995327,-17.1496709256533,
-5.77326404039821));
#145292=CARTESIAN_POINT('Ctrl Pts',(-0.265805776253758,-17.2099065112404,
-5.88509697133669));
#145293=CARTESIAN_POINT('Ctrl Pts',(-0.465549933916129,-17.3149783849924,
-6.0801726145193));
#145294=CARTESIAN_POINT('Origin',(0.,-18.2,-7.72329702653519));
#145295=CARTESIAN_POINT('Origin',(19.1875302357774,-17.3150528379807,-0.374581597160819));
#145296=CARTESIAN_POINT('Origin',(3.02518007237845E-18,-18.4457456132867,
1.24021503613021));
#145297=CARTESIAN_POINT('Ctrl Pts',(-0.914382087390238,-17.5216755952362,
-0.0794937182387867));
#145298=CARTESIAN_POINT('Ctrl Pts',(-0.683643791787282,-17.293356355078,
-0.405567385971643));
#145299=CARTESIAN_POINT('Ctrl Pts',(-0.125022675737884,-17.054213772593,
-0.747098388474721));
#145300=CARTESIAN_POINT('Ctrl Pts',(0.448115403944561,-17.2013730333212,
-0.536933183592055));
#145301=CARTESIAN_POINT('Ctrl Pts',(0.658073755029969,-17.3246127340343,
-0.360928650667152));
#145302=CARTESIAN_POINT('Ctrl Pts',(-0.832254441336071,-17.5489810332648,
-0.0404975113449715));
#145303=CARTESIAN_POINT('Ctrl Pts',(-0.627393047499884,-17.3253518030282,
-0.359056762504974));
#145304=CARTESIAN_POINT('Ctrl Pts',(-0.115018286391046,-17.0908909725833,
-0.694774811887389));
#145305=CARTESIAN_POINT('Ctrl Pts',(0.41157768336954,-17.235251291275,-0.488248529886861));
#145306=CARTESIAN_POINT('Ctrl Pts',(0.601833509913226,-17.3561346296068,
-0.315910718336575));
#145307=CARTESIAN_POINT('Ctrl Pts',(-0.751191480614262,-17.5364962027232,
0.0256067422309708));
#145308=CARTESIAN_POINT('Ctrl Pts',(-0.570929837813018,-17.3337638916996,
-0.296314833667629));
#145309=CARTESIAN_POINT('Ctrl Pts',(-0.105131601746012,-17.1167802483211,
-0.634963805784064));
#145310=CARTESIAN_POINT('Ctrl Pts',(0.375028796817523,-17.2503715095973,
-0.426620170382907));
#145311=CARTESIAN_POINT('Ctrl Pts',(0.545941211667053,-17.3609108659448,
-0.252580344646373));
#145312=CARTESIAN_POINT('Ctrl Pts',(-0.703370836454029,-17.4891769091919,
0.0925792126665251));
#145313=CARTESIAN_POINT('Ctrl Pts',(-0.525879839836371,-17.3135467244548,
-0.233494455066332));
#145314=CARTESIAN_POINT('Ctrl Pts',(-0.096171289029141,-17.1295908917741,
-0.575025457569408));
#145315=CARTESIAN_POINT('Ctrl Pts',(0.344704156880431,-17.2427903231035,
-0.364860252686742));
#145316=CARTESIAN_POINT('Ctrl Pts',(0.506210580792283,-17.3375900928828,
-0.188855719761839));
#145317=CARTESIAN_POINT('Origin',(13.3623247423326,-19.9,7.82921171985308));
#145318=CARTESIAN_POINT('',(13.7548828365128,-15.9,7.75241235336064));
#145319=CARTESIAN_POINT('Origin',(13.3623247423326,-15.9,7.82921171985308));
#145320=CARTESIAN_POINT('',(13.7548828365128,-19.9,7.75241235336064));
#145321=CARTESIAN_POINT('Origin',(1.19999999921058,-19.9,-1.85000000003699));
#145322=CARTESIAN_POINT('',(1.19999999921058,-19.9,-2.45000000003699));
#145323=CARTESIAN_POINT('Origin',(4.3,-19.9,-1.85000000003699));
#145324=CARTESIAN_POINT('',(4.9,-19.9,-1.85000000003699));
#145325=CARTESIAN_POINT('',(4.3,-19.9,-2.45000000003699));
#145326=CARTESIAN_POINT('Origin',(-5.94265499251984,-19.9,-2.45000000003699));
#145327=CARTESIAN_POINT('Origin',(-10.2709990938499,-21.1,0.945217224235999));
#145328=CARTESIAN_POINT('Origin',(-10.2709990938499,-20.,0.945217224235999));
#145329=CARTESIAN_POINT('Origin',(-15.3000000000043,-22.8,6.20189169841846));
#145330=CARTESIAN_POINT('',(-14.9000000000043,-15.9,6.20189169841771));
#145331=CARTESIAN_POINT('',(-14.9000000000043,-22.8,6.20189169841771));
#145332=CARTESIAN_POINT('',(-15.0836363636405,-15.9,5.86545927302008));
#145333=CARTESIAN_POINT('Origin',(-15.3000000000043,-15.9,6.20189169841846));
#145334=CARTESIAN_POINT('',(-15.0836363636405,-22.8,5.86545927302008));
#145335=CARTESIAN_POINT('Origin',(-9.35,-22.8,-3.05000000003699));
#145336=CARTESIAN_POINT('',(-15.8545454545506,-15.9,5.31964087814201));
#145337=CARTESIAN_POINT('',(-15.8545454545506,-22.8,5.31964087814201));
#145338=CARTESIAN_POINT('Origin',(-9.35,-15.9,-3.05000000003699));
#145339=CARTESIAN_POINT('Origin',(-16.1000000000054,-22.8,5.63547638297895));
#145340=CARTESIAN_POINT('Origin',(-16.1000000000054,-15.9,5.63547638297895));
#145341=CARTESIAN_POINT('Origin',(-3.1143484430694,-15.9,-8.60653400714346));
#145342=CARTESIAN_POINT('Origin',(-16.1000000000089,-15.9,3.77623615174389));
#145343=CARTESIAN_POINT('',(-14.9000000000142,-15.9,0.96536214654126));
#145344=CARTESIAN_POINT('Origin',(6.09999999999969,-15.9,9.2499999999633));
#145345=CARTESIAN_POINT('Origin',(-16.1000000000089,-19.9,3.77623615174389));
#145346=CARTESIAN_POINT('Origin',(-16.1000000000089,-20.,3.77623615174389));
#145347=CARTESIAN_POINT('Origin',(-5.42954084321747,-21.1,-1.85000000003699));
#145348=CARTESIAN_POINT('Origin',(0.0158955791744741,-19.9,-3.65000000003699));
#145349=CARTESIAN_POINT('',(-1.20000000078942,-19.9,-3.65000000003699));
#145350=CARTESIAN_POINT('Origin',(-1.20000000078942,-19.9,-4.25000000003699));
#145351=CARTESIAN_POINT('',(-0.600000000789417,-19.9,-4.25000000003699));
#145352=CARTESIAN_POINT('Origin',(-0.600000000789418,-19.9,0.384748901093117));
#145353=CARTESIAN_POINT('',(-0.600000000789417,-19.9,-5.79545078503888));
#145354=CARTESIAN_POINT('Origin',(-1.20000000078942,-19.9,-5.79545078503888));
#145355=CARTESIAN_POINT('Origin',(6.1,-21.,-12.1857384988752));
#145356=CARTESIAN_POINT('Origin',(8.6,-19.9,-0.741996797474057));
#145357=CARTESIAN_POINT('',(4.9,-19.9,-0.741996797474059));
#145358=CARTESIAN_POINT('Origin',(4.9,-19.9,-5.32716721908225));
#145359=CARTESIAN_POINT('Origin',(6.09999999999969,-19.9,9.2499999999633));
#145360=CARTESIAN_POINT('',(13.8999999999997,-19.9,9.24999999996345));
#145361=CARTESIAN_POINT('Origin',(13.8999999999998,-19.9,1.44999999996345));
#145362=CARTESIAN_POINT('',(13.8999999999998,-25.4,0.499999999970565));
#145363=CARTESIAN_POINT('Origin',(-14.8999999999961,-22.8,10.5372583002038));
#145364=CARTESIAN_POINT('',(-14.8999999999968,-22.8,10.2058874503056));
#145365=CARTESIAN_POINT('Origin',(-14.0999999999968,-22.8,10.2058874503041));
#145366=CARTESIAN_POINT('Origin',(7.94152002157416E-16,-18.2,15.6578006787879));
#145367=CARTESIAN_POINT('Origin',(2.10864821770493E-16,-18.2,10.175));
#145368=CARTESIAN_POINT('Origin',(3.04851216033843,-24.4,10.2415765003998));
#145369=CARTESIAN_POINT('Origin',(2.3,-22.8,6.19999999999999));
#145370=CARTESIAN_POINT('Origin',(16.5000000000094,-24.4,1.94999999997594));
#145371=CARTESIAN_POINT('',(16.7343145750595,-25.4,2.18431457502608));
#145372=CARTESIAN_POINT('',(11.7750000000018,-25.4,-2.77500000003169));
#145373=CARTESIAN_POINT('',(16.7343145750595,-23.,2.18431457502608));
#145374=CARTESIAN_POINT('',(16.7343145750595,-24.4,2.18431457502608));
#145375=CARTESIAN_POINT('',(16.7650854557587,-23.,2.2150854557252));
#145376=CARTESIAN_POINT('Origin',(17.3000000000088,-24.4,1.61862915007684));
#145377=CARTESIAN_POINT('',(16.5000000000088,-25.4,1.61862915007834));
#145378=CARTESIAN_POINT('Origin',(17.3000000000088,-25.4,1.61862915007684));
#145379=CARTESIAN_POINT('',(16.5000000000088,-23.,1.61862915007834));
#145380=CARTESIAN_POINT('',(16.5000000000088,-24.,1.61862915007834));
#145381=CARTESIAN_POINT('Origin',(17.3000000000088,-23.,1.61862915007684));
#145382=CARTESIAN_POINT('Origin',(16.4999999999906,-24.4,-8.05000000002406));
#145383=CARTESIAN_POINT('',(16.4999999999977,-25.4,-4.25000000003885));
#145384=CARTESIAN_POINT('',(16.5000000000088,-23.,1.61862915007834));
#145385=CARTESIAN_POINT('Origin',(9.25,-23.,-3.05000000003699));
#145386=CARTESIAN_POINT('Origin',(15.8325427278768,-23.,-1.75748667391245));
#145387=CARTESIAN_POINT('Origin',(0.,-18.2,-19.1));
#145388=CARTESIAN_POINT('',(-1.,-18.2,-19.1));
#145389=CARTESIAN_POINT('Origin',(-2.25752749827279E-11,-25.4,-0.450000000022578));
#145390=CARTESIAN_POINT('Origin',(-17.3000000000305,-25.4,-7.71862915012444));
#145391=CARTESIAN_POINT('Origin',(-17.3000000000305,-24.4,-7.71862915012444));
#145392=CARTESIAN_POINT('Origin',(-17.3000000000305,-20.,-7.71862915012444));
#145393=CARTESIAN_POINT('Origin',(-16.0596875762449,-20.,-5.65000000005141));
#145394=CARTESIAN_POINT('Origin',(-14.5525630318579,-19.9,-10.8611035007945));
#145395=CARTESIAN_POINT('',(-13.6127165965579,-20.,-9.23324172354236));
#145396=CARTESIAN_POINT('Origin',(-16.0596875762449,-20.,-5.65000000005141));
#145397=CARTESIAN_POINT('Origin',(-3.1143484430694,-15.9,-8.60653400714346));
#459195=UNCERTAINTY_MEASURE_WITH_UNIT(LENGTH_MEASURE(0.01),#459243,
'DISTANCE_ACCURACY_VALUE',
'Maximum model space distance between geometric entities at asserted c
onnectivities');
#459216=UNCERTAINTY_MEASURE_WITH_UNIT(LENGTH_MEASURE(0.01),#459243,
'DISTANCE_ACCURACY_VALUE',
'Maximum model space distance between geometric entities at asserted c
onnectivities');
#459221=(
GEOMETRIC_REPRESENTATION_CONTEXT(3)
GLOBAL_UNCERTAINTY_ASSIGNED_CONTEXT((#459195))
GLOBAL_UNIT_ASSIGNED_CONTEXT((#459243,#459245,#459246))
REPRESENTATION_CONTEXT('','3D')
);
#459242=(
GEOMETRIC_REPRESENTATION_CONTEXT(3)
GLOBAL_UNCERTAINTY_ASSIGNED_CONTEXT((#459216))
GLOBAL_UNIT_ASSIGNED_CONTEXT((#459243,#459245,#459246))
REPRESENTATION_CONTEXT('','3D')
);
#459243=(
LENGTH_UNIT()
NAMED_UNIT(*)
SI_UNIT(.MILLI.,.METRE.)
);
#459245=(
NAMED_UNIT(*)
PLANE_ANGLE_UNIT()
SI_UNIT($,.RADIAN.)
);
#459246=(
NAMED_UNIT(*)
SI_UNIT($,.STERADIAN.)
SOLID_ANGLE_UNIT()
);
#459251=SHAPE_DEFINITION_REPRESENTATION(#459276,#459332);
#459276=PRODUCT_DEFINITION_SHAPE('',$,#459358);
#459332=SHAPE_REPRESENTATION('',(#95341),#459221);
#459353=PRODUCT_DEFINITION_CONTEXT('part definition',#459430,'design');
#459358=PRODUCT_DEFINITION('Extruder Housing and Cover',
'Extruder Housing and Cover',#459383,#459353);
#459383=PRODUCT_DEFINITION_FORMATION('',$,#459436);
#459430=APPLICATION_CONTEXT(
'Core Data for Automotive Mechanical Design Process');
#459431=PRODUCT_CONTEXT('part definition',#459430,'mechanical');
#459436=PRODUCT('Extruder Housing and Cover',
'Extruder Housing and Cover',$,(#459431));
#459499=COLOUR_RGB('Dark Blue',0.08,0.2,0.34);
#459500=FILL_AREA_STYLE_COLOUR('',#459499);
#459501=FILL_AREA_STYLE('',(#459500));
#459502=SURFACE_STYLE_FILL_AREA(#459501);
#459503=SURFACE_SIDE_STYLE('',(#459502));
#459504=SURFACE_STYLE_USAGE(.BOTH.,#459503);
#459505=PRESENTATION_STYLE_ASSIGNMENT((#459504));
ENDSEC;
END-ISO-10303-21;
